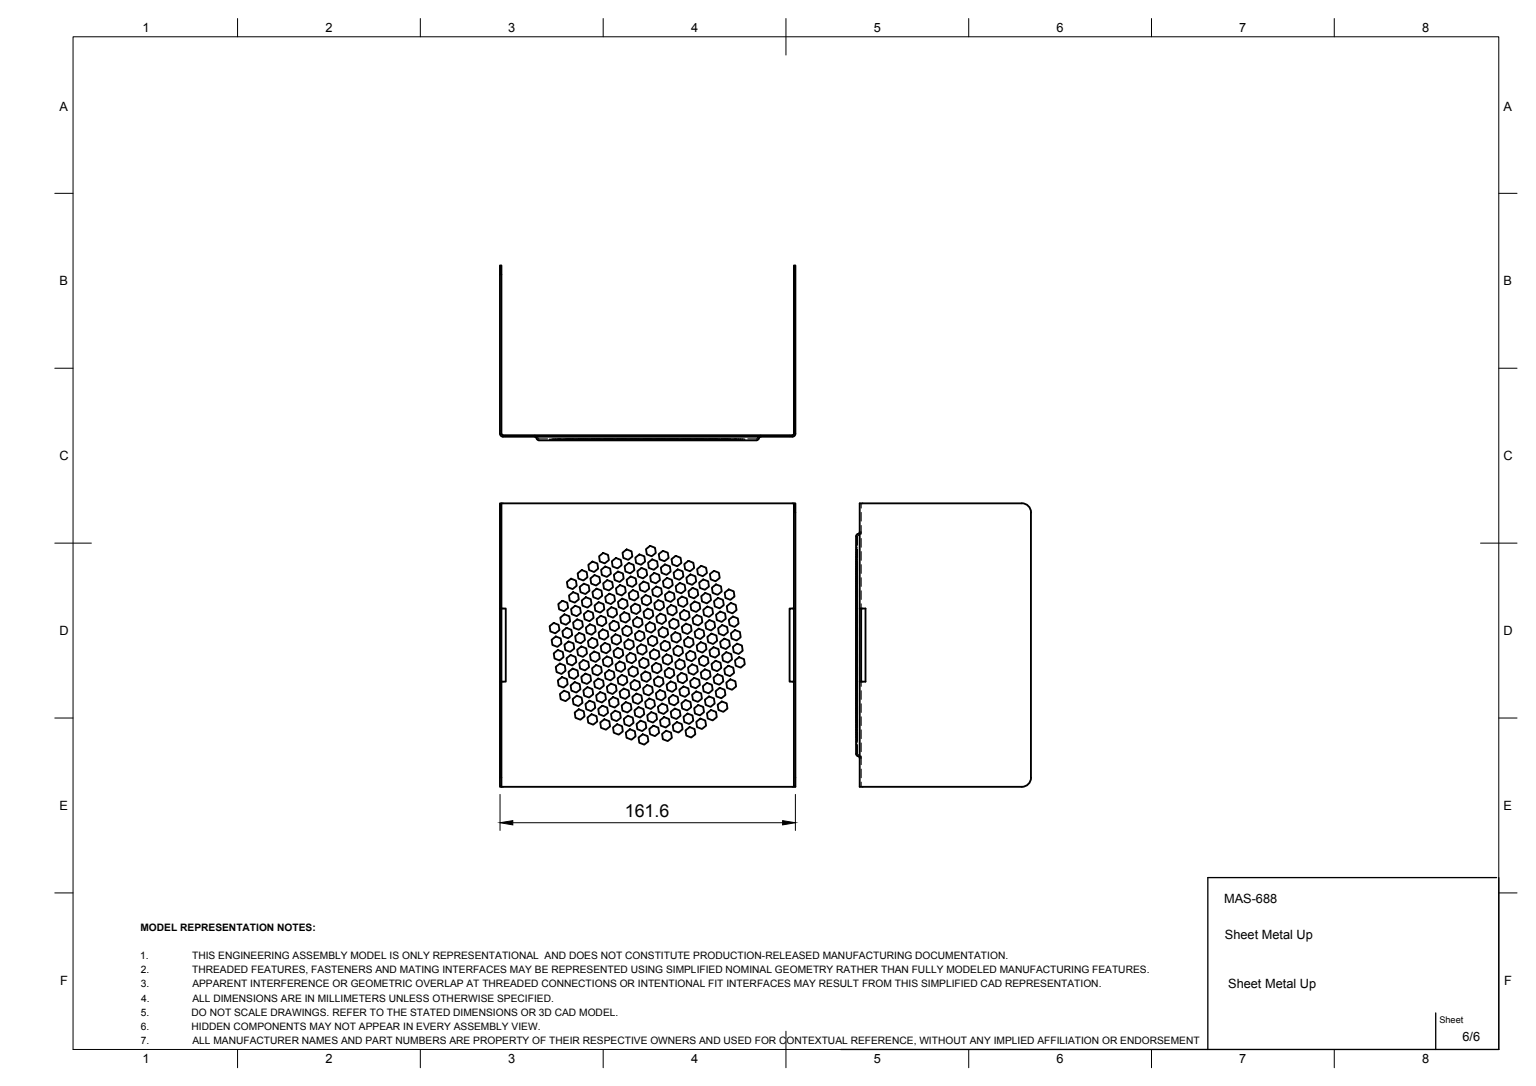
ISO-10303-21;
HEADER;
/* Generated by software containing ST-Developer
 * from STEP Tools, Inc. (www.steptools.com) 
 */

FILE_DESCRIPTION(
/* description */ ('STEP AP214'),
/* implementation_level */ '2;1');

FILE_NAME(
/* name */ 'Sheet Metal Up.step',
/* time_stamp */ '2026-11-14T03:58:36-08:00',
/* author */ (''),
/* organization */ (''),
/* preprocessor_version */ 'ST-DEVELOPER v20.2',
/* originating_system */ 'Autodesk Translation Framework v15.17.0.0',
/* authorisation */ '');

FILE_SCHEMA (('AUTOMOTIVE_DESIGN { 1 0 10303 214 3 1 1 }'));
ENDSEC;

DATA;
#10=MECHANICAL_DESIGN_GEOMETRIC_PRESENTATION_REPRESENTATION('',(#44),#65304);
#36=SHAPE_REPRESENTATION_RELATIONSHIP('SRR','None',#65327,#40);
#40=ADVANCED_BREP_SHAPE_REPRESENTATION('',(#47),#65303);
#44=STYLED_ITEM('',(#65356),#47);
#47=MANIFOLD_SOLID_BREP('Body1',#39937);
#255=FACE_BOUND('',#5203,.T.);
#256=FACE_BOUND('',#5205,.T.);
#257=FACE_BOUND('',#5251,.T.);
#258=FACE_BOUND('',#5252,.T.);
#259=FACE_BOUND('',#5253,.T.);
#260=FACE_BOUND('',#5254,.T.);
#261=FACE_BOUND('',#5255,.T.);
#262=FACE_BOUND('',#5256,.T.);
#263=FACE_BOUND('',#5257,.T.);
#264=FACE_BOUND('',#5258,.T.);
#265=FACE_BOUND('',#5259,.T.);
#266=FACE_BOUND('',#5260,.T.);
#267=FACE_BOUND('',#5261,.T.);
#268=FACE_BOUND('',#5262,.T.);
#269=FACE_BOUND('',#5263,.T.);
#270=FACE_BOUND('',#5264,.T.);
#271=FACE_BOUND('',#5265,.T.);
#272=FACE_BOUND('',#5266,.T.);
#273=FACE_BOUND('',#5267,.T.);
#274=FACE_BOUND('',#5268,.T.);
#275=FACE_BOUND('',#5269,.T.);
#276=FACE_BOUND('',#5270,.T.);
#277=FACE_BOUND('',#5271,.T.);
#278=FACE_BOUND('',#5272,.T.);
#279=FACE_BOUND('',#5273,.T.);
#280=FACE_BOUND('',#5274,.T.);
#281=FACE_BOUND('',#5275,.T.);
#282=FACE_BOUND('',#5276,.T.);
#283=FACE_BOUND('',#5277,.T.);
#284=FACE_BOUND('',#5278,.T.);
#285=FACE_BOUND('',#5279,.T.);
#286=FACE_BOUND('',#5280,.T.);
#287=FACE_BOUND('',#5281,.T.);
#288=FACE_BOUND('',#5282,.T.);
#289=FACE_BOUND('',#5283,.T.);
#290=FACE_BOUND('',#5284,.T.);
#291=FACE_BOUND('',#5285,.T.);
#292=FACE_BOUND('',#5286,.T.);
#293=FACE_BOUND('',#5287,.T.);
#294=FACE_BOUND('',#5288,.T.);
#295=FACE_BOUND('',#5289,.T.);
#296=FACE_BOUND('',#5290,.T.);
#297=FACE_BOUND('',#5291,.T.);
#298=FACE_BOUND('',#5292,.T.);
#299=FACE_BOUND('',#5293,.T.);
#300=FACE_BOUND('',#5294,.T.);
#301=FACE_BOUND('',#5295,.T.);
#302=FACE_BOUND('',#5296,.T.);
#303=FACE_BOUND('',#5297,.T.);
#304=FACE_BOUND('',#5298,.T.);
#305=FACE_BOUND('',#5299,.T.);
#306=FACE_BOUND('',#5300,.T.);
#307=FACE_BOUND('',#5301,.T.);
#308=FACE_BOUND('',#5302,.T.);
#309=FACE_BOUND('',#5303,.T.);
#310=FACE_BOUND('',#5304,.T.);
#311=FACE_BOUND('',#5305,.T.);
#312=FACE_BOUND('',#5306,.T.);
#313=FACE_BOUND('',#5307,.T.);
#314=FACE_BOUND('',#5308,.T.);
#315=FACE_BOUND('',#5309,.T.);
#316=FACE_BOUND('',#5310,.T.);
#317=FACE_BOUND('',#5311,.T.);
#318=FACE_BOUND('',#5312,.T.);
#319=FACE_BOUND('',#5313,.T.);
#320=FACE_BOUND('',#5314,.T.);
#321=FACE_BOUND('',#5315,.T.);
#322=FACE_BOUND('',#5316,.T.);
#323=FACE_BOUND('',#5317,.T.);
#324=FACE_BOUND('',#5318,.T.);
#325=FACE_BOUND('',#5319,.T.);
#326=FACE_BOUND('',#5320,.T.);
#327=FACE_BOUND('',#5321,.T.);
#328=FACE_BOUND('',#5322,.T.);
#329=FACE_BOUND('',#5323,.T.);
#330=FACE_BOUND('',#5324,.T.);
#331=FACE_BOUND('',#5325,.T.);
#332=FACE_BOUND('',#5326,.T.);
#333=FACE_BOUND('',#5327,.T.);
#334=FACE_BOUND('',#5328,.T.);
#335=FACE_BOUND('',#5329,.T.);
#336=FACE_BOUND('',#5330,.T.);
#337=FACE_BOUND('',#5331,.T.);
#338=FACE_BOUND('',#5332,.T.);
#339=FACE_BOUND('',#5333,.T.);
#340=FACE_BOUND('',#5334,.T.);
#341=FACE_BOUND('',#5335,.T.);
#342=FACE_BOUND('',#5336,.T.);
#343=FACE_BOUND('',#5337,.T.);
#344=FACE_BOUND('',#5338,.T.);
#345=FACE_BOUND('',#5339,.T.);
#346=FACE_BOUND('',#5340,.T.);
#347=FACE_BOUND('',#5341,.T.);
#348=FACE_BOUND('',#5342,.T.);
#349=FACE_BOUND('',#5343,.T.);
#350=FACE_BOUND('',#5344,.T.);
#351=FACE_BOUND('',#5345,.T.);
#352=FACE_BOUND('',#5346,.T.);
#353=FACE_BOUND('',#5347,.T.);
#354=FACE_BOUND('',#5348,.T.);
#355=FACE_BOUND('',#5349,.T.);
#356=FACE_BOUND('',#5350,.T.);
#357=FACE_BOUND('',#5351,.T.);
#358=FACE_BOUND('',#5352,.T.);
#359=FACE_BOUND('',#5353,.T.);
#360=FACE_BOUND('',#5354,.T.);
#361=FACE_BOUND('',#5355,.T.);
#362=FACE_BOUND('',#5356,.T.);
#363=FACE_BOUND('',#5357,.T.);
#364=FACE_BOUND('',#5358,.T.);
#365=FACE_BOUND('',#5359,.T.);
#366=FACE_BOUND('',#5360,.T.);
#367=FACE_BOUND('',#5361,.T.);
#368=FACE_BOUND('',#5362,.T.);
#369=FACE_BOUND('',#5363,.T.);
#370=FACE_BOUND('',#5364,.T.);
#371=FACE_BOUND('',#5365,.T.);
#372=FACE_BOUND('',#5366,.T.);
#373=FACE_BOUND('',#5367,.T.);
#374=FACE_BOUND('',#5368,.T.);
#375=FACE_BOUND('',#5369,.T.);
#376=FACE_BOUND('',#5370,.T.);
#377=FACE_BOUND('',#5371,.T.);
#378=FACE_BOUND('',#5372,.T.);
#379=FACE_BOUND('',#5373,.T.);
#380=FACE_BOUND('',#5374,.T.);
#381=FACE_BOUND('',#5375,.T.);
#382=FACE_BOUND('',#5376,.T.);
#383=FACE_BOUND('',#5377,.T.);
#384=FACE_BOUND('',#5378,.T.);
#385=FACE_BOUND('',#5379,.T.);
#386=FACE_BOUND('',#5380,.T.);
#387=FACE_BOUND('',#5381,.T.);
#388=FACE_BOUND('',#5382,.T.);
#389=FACE_BOUND('',#5383,.T.);
#390=FACE_BOUND('',#5384,.T.);
#391=FACE_BOUND('',#5385,.T.);
#392=FACE_BOUND('',#5386,.T.);
#393=FACE_BOUND('',#5387,.T.);
#394=FACE_BOUND('',#5388,.T.);
#395=FACE_BOUND('',#5389,.T.);
#396=FACE_BOUND('',#5390,.T.);
#397=FACE_BOUND('',#5391,.T.);
#398=FACE_BOUND('',#5392,.T.);
#399=FACE_BOUND('',#5393,.T.);
#400=FACE_BOUND('',#5394,.T.);
#401=FACE_BOUND('',#5395,.T.);
#402=FACE_BOUND('',#5396,.T.);
#403=FACE_BOUND('',#5397,.T.);
#404=FACE_BOUND('',#5398,.T.);
#405=FACE_BOUND('',#5399,.T.);
#406=FACE_BOUND('',#5400,.T.);
#407=FACE_BOUND('',#5401,.T.);
#408=FACE_BOUND('',#5402,.T.);
#409=FACE_BOUND('',#5403,.T.);
#410=FACE_BOUND('',#5404,.T.);
#411=FACE_BOUND('',#5405,.T.);
#412=FACE_BOUND('',#5406,.T.);
#413=FACE_BOUND('',#5407,.T.);
#414=FACE_BOUND('',#5408,.T.);
#415=FACE_BOUND('',#5409,.T.);
#416=FACE_BOUND('',#5410,.T.);
#417=FACE_BOUND('',#5411,.T.);
#418=FACE_BOUND('',#5412,.T.);
#419=FACE_BOUND('',#5413,.T.);
#420=FACE_BOUND('',#5414,.T.);
#421=FACE_BOUND('',#5415,.T.);
#422=FACE_BOUND('',#5416,.T.);
#423=FACE_BOUND('',#5417,.T.);
#424=FACE_BOUND('',#5418,.T.);
#425=FACE_BOUND('',#5419,.T.);
#426=FACE_BOUND('',#5420,.T.);
#427=FACE_BOUND('',#5421,.T.);
#428=FACE_BOUND('',#5422,.T.);
#429=FACE_BOUND('',#5423,.T.);
#430=FACE_BOUND('',#5424,.T.);
#431=FACE_BOUND('',#5425,.T.);
#432=FACE_BOUND('',#5426,.T.);
#433=FACE_BOUND('',#5427,.T.);
#434=FACE_BOUND('',#5428,.T.);
#435=FACE_BOUND('',#5429,.T.);
#436=FACE_BOUND('',#5430,.T.);
#437=FACE_BOUND('',#5431,.T.);
#438=FACE_BOUND('',#5432,.T.);
#439=FACE_BOUND('',#5433,.T.);
#440=FACE_BOUND('',#5434,.T.);
#441=FACE_BOUND('',#5435,.T.);
#442=FACE_BOUND('',#5436,.T.);
#443=FACE_BOUND('',#5438,.T.);
#444=FACE_BOUND('',#5439,.T.);
#445=FACE_BOUND('',#5440,.T.);
#446=FACE_BOUND('',#5441,.T.);
#447=FACE_BOUND('',#5442,.T.);
#448=FACE_BOUND('',#5443,.T.);
#449=FACE_BOUND('',#5444,.T.);
#450=FACE_BOUND('',#5445,.T.);
#451=FACE_BOUND('',#5446,.T.);
#452=FACE_BOUND('',#5447,.T.);
#453=FACE_BOUND('',#5448,.T.);
#454=FACE_BOUND('',#5449,.T.);
#455=FACE_BOUND('',#5450,.T.);
#456=FACE_BOUND('',#5451,.T.);
#457=FACE_BOUND('',#5452,.T.);
#458=FACE_BOUND('',#5453,.T.);
#459=FACE_BOUND('',#5454,.T.);
#460=FACE_BOUND('',#5455,.T.);
#461=FACE_BOUND('',#5456,.T.);
#462=FACE_BOUND('',#5457,.T.);
#463=FACE_BOUND('',#5458,.T.);
#464=FACE_BOUND('',#5459,.T.);
#465=FACE_BOUND('',#5460,.T.);
#466=FACE_BOUND('',#5461,.T.);
#467=FACE_BOUND('',#5462,.T.);
#468=FACE_BOUND('',#5463,.T.);
#469=FACE_BOUND('',#5464,.T.);
#470=FACE_BOUND('',#5465,.T.);
#471=FACE_BOUND('',#5466,.T.);
#472=FACE_BOUND('',#5467,.T.);
#473=FACE_BOUND('',#5468,.T.);
#474=FACE_BOUND('',#5469,.T.);
#475=FACE_BOUND('',#5470,.T.);
#476=FACE_BOUND('',#5471,.T.);
#477=FACE_BOUND('',#5472,.T.);
#478=FACE_BOUND('',#5473,.T.);
#479=FACE_BOUND('',#5474,.T.);
#480=FACE_BOUND('',#5475,.T.);
#481=FACE_BOUND('',#5476,.T.);
#482=FACE_BOUND('',#5477,.T.);
#483=FACE_BOUND('',#5478,.T.);
#484=FACE_BOUND('',#5479,.T.);
#485=FACE_BOUND('',#5480,.T.);
#486=FACE_BOUND('',#5481,.T.);
#487=FACE_BOUND('',#5482,.T.);
#488=FACE_BOUND('',#5483,.T.);
#489=FACE_BOUND('',#5484,.T.);
#490=FACE_BOUND('',#5485,.T.);
#491=FACE_BOUND('',#5486,.T.);
#492=FACE_BOUND('',#5487,.T.);
#493=FACE_BOUND('',#5488,.T.);
#494=FACE_BOUND('',#5489,.T.);
#495=FACE_BOUND('',#5490,.T.);
#496=FACE_BOUND('',#5491,.T.);
#497=FACE_BOUND('',#5492,.T.);
#498=FACE_BOUND('',#5493,.T.);
#499=FACE_BOUND('',#5494,.T.);
#500=FACE_BOUND('',#5495,.T.);
#501=FACE_BOUND('',#5496,.T.);
#502=FACE_BOUND('',#5497,.T.);
#503=FACE_BOUND('',#5498,.T.);
#504=FACE_BOUND('',#5499,.T.);
#505=FACE_BOUND('',#5500,.T.);
#506=FACE_BOUND('',#5501,.T.);
#507=FACE_BOUND('',#5502,.T.);
#508=FACE_BOUND('',#5503,.T.);
#509=FACE_BOUND('',#5504,.T.);
#510=FACE_BOUND('',#5505,.T.);
#511=FACE_BOUND('',#5506,.T.);
#512=FACE_BOUND('',#5507,.T.);
#513=FACE_BOUND('',#5508,.T.);
#514=FACE_BOUND('',#5509,.T.);
#515=FACE_BOUND('',#5510,.T.);
#516=FACE_BOUND('',#5511,.T.);
#517=FACE_BOUND('',#5512,.T.);
#518=FACE_BOUND('',#5513,.T.);
#519=FACE_BOUND('',#5514,.T.);
#520=FACE_BOUND('',#5515,.T.);
#521=FACE_BOUND('',#5516,.T.);
#522=FACE_BOUND('',#5517,.T.);
#523=FACE_BOUND('',#5518,.T.);
#524=FACE_BOUND('',#5519,.T.);
#525=FACE_BOUND('',#5520,.T.);
#526=FACE_BOUND('',#5521,.T.);
#527=FACE_BOUND('',#5522,.T.);
#528=FACE_BOUND('',#5523,.T.);
#529=FACE_BOUND('',#5524,.T.);
#530=FACE_BOUND('',#5525,.T.);
#531=FACE_BOUND('',#5526,.T.);
#532=FACE_BOUND('',#5527,.T.);
#533=FACE_BOUND('',#5528,.T.);
#534=FACE_BOUND('',#5529,.T.);
#535=FACE_BOUND('',#5530,.T.);
#536=FACE_BOUND('',#5531,.T.);
#537=FACE_BOUND('',#5532,.T.);
#538=FACE_BOUND('',#5533,.T.);
#539=FACE_BOUND('',#5534,.T.);
#540=FACE_BOUND('',#5535,.T.);
#541=FACE_BOUND('',#5536,.T.);
#542=FACE_BOUND('',#5537,.T.);
#543=FACE_BOUND('',#5538,.T.);
#544=FACE_BOUND('',#5539,.T.);
#545=FACE_BOUND('',#5540,.T.);
#546=FACE_BOUND('',#5541,.T.);
#547=FACE_BOUND('',#5542,.T.);
#548=FACE_BOUND('',#5543,.T.);
#549=FACE_BOUND('',#5544,.T.);
#550=FACE_BOUND('',#5545,.T.);
#551=FACE_BOUND('',#5546,.T.);
#552=FACE_BOUND('',#5547,.T.);
#553=FACE_BOUND('',#5548,.T.);
#554=FACE_BOUND('',#5549,.T.);
#555=FACE_BOUND('',#5550,.T.);
#556=FACE_BOUND('',#5551,.T.);
#557=FACE_BOUND('',#5552,.T.);
#558=FACE_BOUND('',#5553,.T.);
#559=FACE_BOUND('',#5554,.T.);
#560=FACE_BOUND('',#5555,.T.);
#561=FACE_BOUND('',#5556,.T.);
#562=FACE_BOUND('',#5557,.T.);
#563=FACE_BOUND('',#5558,.T.);
#564=FACE_BOUND('',#5559,.T.);
#565=FACE_BOUND('',#5560,.T.);
#566=FACE_BOUND('',#5561,.T.);
#567=FACE_BOUND('',#5562,.T.);
#568=FACE_BOUND('',#5563,.T.);
#569=FACE_BOUND('',#5564,.T.);
#570=FACE_BOUND('',#5565,.T.);
#571=FACE_BOUND('',#5566,.T.);
#572=FACE_BOUND('',#5567,.T.);
#573=FACE_BOUND('',#5568,.T.);
#574=FACE_BOUND('',#5569,.T.);
#575=FACE_BOUND('',#5570,.T.);
#576=FACE_BOUND('',#5571,.T.);
#577=FACE_BOUND('',#5572,.T.);
#578=FACE_BOUND('',#5573,.T.);
#579=FACE_BOUND('',#5574,.T.);
#580=FACE_BOUND('',#5575,.T.);
#581=FACE_BOUND('',#5576,.T.);
#582=FACE_BOUND('',#5577,.T.);
#583=FACE_BOUND('',#5578,.T.);
#584=FACE_BOUND('',#5579,.T.);
#585=FACE_BOUND('',#5580,.T.);
#586=FACE_BOUND('',#5581,.T.);
#587=FACE_BOUND('',#5582,.T.);
#588=FACE_BOUND('',#5583,.T.);
#589=FACE_BOUND('',#5584,.T.);
#590=FACE_BOUND('',#5585,.T.);
#591=FACE_BOUND('',#5586,.T.);
#592=FACE_BOUND('',#5587,.T.);
#593=FACE_BOUND('',#5588,.T.);
#594=FACE_BOUND('',#5589,.T.);
#595=FACE_BOUND('',#5590,.T.);
#596=FACE_BOUND('',#5591,.T.);
#597=FACE_BOUND('',#5592,.T.);
#598=FACE_BOUND('',#5593,.T.);
#599=FACE_BOUND('',#5594,.T.);
#600=FACE_BOUND('',#5595,.T.);
#601=FACE_BOUND('',#5596,.T.);
#602=FACE_BOUND('',#5597,.T.);
#603=FACE_BOUND('',#5598,.T.);
#604=FACE_BOUND('',#5599,.T.);
#605=FACE_BOUND('',#5600,.T.);
#606=FACE_BOUND('',#5601,.T.);
#607=FACE_BOUND('',#5602,.T.);
#608=FACE_BOUND('',#5603,.T.);
#609=FACE_BOUND('',#5604,.T.);
#610=FACE_BOUND('',#5605,.T.);
#611=FACE_BOUND('',#5606,.T.);
#612=FACE_BOUND('',#5607,.T.);
#613=FACE_BOUND('',#5608,.T.);
#614=FACE_BOUND('',#5609,.T.);
#615=FACE_BOUND('',#5610,.T.);
#616=FACE_BOUND('',#5611,.T.);
#617=FACE_BOUND('',#5612,.T.);
#618=FACE_BOUND('',#5613,.T.);
#619=FACE_BOUND('',#5614,.T.);
#620=FACE_BOUND('',#5615,.T.);
#621=FACE_BOUND('',#5616,.T.);
#622=FACE_BOUND('',#5617,.T.);
#623=FACE_BOUND('',#5618,.T.);
#624=FACE_BOUND('',#5619,.T.);
#625=FACE_BOUND('',#5620,.T.);
#626=FACE_BOUND('',#5621,.T.);
#627=FACE_BOUND('',#5622,.T.);
#628=FACE_BOUND('',#5623,.T.);
#1029=PLANE('',#41322);
#1030=PLANE('',#41323);
#1031=PLANE('',#41324);
#1032=PLANE('',#41325);
#1033=PLANE('',#41326);
#1034=PLANE('',#41327);
#1035=PLANE('',#41328);
#1036=PLANE('',#41329);
#1037=PLANE('',#41330);
#1038=PLANE('',#41331);
#1039=PLANE('',#41332);
#1040=PLANE('',#41335);
#1041=PLANE('',#41340);
#1042=PLANE('',#41343);
#1043=PLANE('',#41351);
#1044=PLANE('',#41355);
#1045=PLANE('',#41356);
#1046=PLANE('',#41357);
#1047=PLANE('',#41358);
#1048=PLANE('',#41359);
#1049=PLANE('',#41360);
#1050=PLANE('',#41361);
#1051=PLANE('',#41362);
#1052=PLANE('',#41365);
#1053=PLANE('',#41370);
#1054=PLANE('',#41373);
#1055=PLANE('',#41381);
#1056=PLANE('',#41385);
#1057=PLANE('',#41386);
#1058=PLANE('',#41387);
#1059=PLANE('',#41388);
#1060=PLANE('',#41389);
#1061=PLANE('',#41390);
#1062=PLANE('',#41391);
#1063=PLANE('',#41392);
#1064=PLANE('',#41393);
#1065=PLANE('',#41394);
#1066=PLANE('',#41395);
#1067=PLANE('',#41396);
#1068=PLANE('',#41397);
#1069=PLANE('',#41398);
#1070=PLANE('',#41399);
#1071=PLANE('',#41400);
#1072=PLANE('',#41401);
#1073=PLANE('',#41402);
#1074=PLANE('',#41403);
#1075=PLANE('',#41404);
#1076=PLANE('',#41405);
#1077=PLANE('',#41406);
#1078=PLANE('',#41407);
#1079=PLANE('',#41408);
#1080=PLANE('',#41409);
#1081=PLANE('',#41410);
#1082=PLANE('',#41411);
#1083=PLANE('',#41412);
#1084=PLANE('',#41413);
#1085=PLANE('',#41414);
#1086=PLANE('',#41415);
#1087=PLANE('',#41416);
#1088=PLANE('',#41417);
#1089=PLANE('',#41418);
#1090=PLANE('',#41419);
#1091=PLANE('',#41420);
#1092=PLANE('',#41421);
#1093=PLANE('',#41422);
#1094=PLANE('',#41423);
#1095=PLANE('',#41424);
#1096=PLANE('',#41425);
#1097=PLANE('',#41426);
#1098=PLANE('',#41427);
#1099=PLANE('',#41428);
#1100=PLANE('',#41429);
#1101=PLANE('',#41430);
#1102=PLANE('',#41431);
#1103=PLANE('',#41432);
#1104=PLANE('',#41433);
#1105=PLANE('',#41434);
#1106=PLANE('',#41435);
#1107=PLANE('',#41436);
#1108=PLANE('',#41437);
#1109=PLANE('',#41438);
#1110=PLANE('',#41439);
#1111=PLANE('',#41440);
#1112=PLANE('',#41441);
#1113=PLANE('',#41442);
#1114=PLANE('',#41443);
#1115=PLANE('',#41444);
#1116=PLANE('',#41445);
#1117=PLANE('',#41446);
#1118=PLANE('',#41447);
#1119=PLANE('',#41448);
#1120=PLANE('',#41449);
#1121=PLANE('',#41450);
#1122=PLANE('',#41451);
#1123=PLANE('',#41452);
#1124=PLANE('',#41453);
#1125=PLANE('',#41454);
#1126=PLANE('',#41455);
#1127=PLANE('',#41456);
#1128=PLANE('',#41457);
#1129=PLANE('',#41458);
#1130=PLANE('',#41459);
#1131=PLANE('',#41460);
#1132=PLANE('',#41461);
#1133=PLANE('',#41462);
#1134=PLANE('',#41463);
#1135=PLANE('',#41464);
#1136=PLANE('',#41465);
#1137=PLANE('',#41466);
#1138=PLANE('',#41467);
#1139=PLANE('',#41468);
#1140=PLANE('',#41469);
#1141=PLANE('',#41470);
#1142=PLANE('',#41471);
#1143=PLANE('',#41472);
#1144=PLANE('',#41473);
#1145=PLANE('',#41474);
#1146=PLANE('',#41475);
#1147=PLANE('',#41476);
#1148=PLANE('',#41477);
#1149=PLANE('',#41478);
#1150=PLANE('',#41479);
#1151=PLANE('',#41480);
#1152=PLANE('',#41481);
#1153=PLANE('',#41482);
#1154=PLANE('',#41483);
#1155=PLANE('',#41484);
#1156=PLANE('',#41485);
#1157=PLANE('',#41486);
#1158=PLANE('',#41487);
#1159=PLANE('',#41488);
#1160=PLANE('',#41489);
#1161=PLANE('',#41490);
#1162=PLANE('',#41491);
#1163=PLANE('',#41492);
#1164=PLANE('',#41493);
#1165=PLANE('',#41494);
#1166=PLANE('',#41495);
#1167=PLANE('',#41496);
#1168=PLANE('',#41497);
#1169=PLANE('',#41498);
#1170=PLANE('',#41499);
#1171=PLANE('',#41500);
#1172=PLANE('',#41501);
#1173=PLANE('',#41502);
#1174=PLANE('',#41503);
#1175=PLANE('',#41504);
#1176=PLANE('',#41505);
#1177=PLANE('',#41506);
#1178=PLANE('',#41507);
#1179=PLANE('',#41508);
#1180=PLANE('',#41509);
#1181=PLANE('',#41510);
#1182=PLANE('',#41511);
#1183=PLANE('',#41512);
#1184=PLANE('',#41513);
#1185=PLANE('',#41514);
#1186=PLANE('',#41515);
#1187=PLANE('',#41516);
#1188=PLANE('',#41517);
#1189=PLANE('',#41518);
#1190=PLANE('',#41519);
#1191=PLANE('',#41520);
#1192=PLANE('',#41521);
#1193=PLANE('',#41522);
#1194=PLANE('',#41523);
#1195=PLANE('',#41524);
#1196=PLANE('',#41525);
#1197=PLANE('',#41526);
#1198=PLANE('',#41527);
#1199=PLANE('',#41528);
#1200=PLANE('',#41529);
#1201=PLANE('',#41530);
#1202=PLANE('',#41531);
#1203=PLANE('',#41532);
#1204=PLANE('',#41533);
#1205=PLANE('',#41534);
#1206=PLANE('',#41535);
#1207=PLANE('',#41536);
#1208=PLANE('',#41537);
#1209=PLANE('',#41538);
#1210=PLANE('',#41539);
#1211=PLANE('',#41540);
#1212=PLANE('',#41541);
#1213=PLANE('',#41542);
#1214=PLANE('',#41543);
#1215=PLANE('',#41544);
#1216=PLANE('',#41545);
#1217=PLANE('',#41546);
#1218=PLANE('',#41547);
#1219=PLANE('',#41548);
#1220=PLANE('',#41549);
#1221=PLANE('',#41550);
#1222=PLANE('',#41551);
#1223=PLANE('',#41552);
#1224=PLANE('',#41553);
#1225=PLANE('',#41554);
#1226=PLANE('',#41555);
#1227=PLANE('',#41556);
#1228=PLANE('',#41557);
#1229=PLANE('',#41558);
#1230=PLANE('',#41559);
#1231=PLANE('',#41560);
#1232=PLANE('',#41561);
#1233=PLANE('',#41562);
#1234=PLANE('',#41563);
#1235=PLANE('',#41564);
#1236=PLANE('',#41565);
#1237=PLANE('',#41566);
#1238=PLANE('',#41567);
#1239=PLANE('',#41568);
#1240=PLANE('',#41569);
#1241=PLANE('',#41570);
#1242=PLANE('',#41571);
#1243=PLANE('',#41572);
#1244=PLANE('',#41573);
#1245=PLANE('',#41574);
#1246=PLANE('',#41575);
#1247=PLANE('',#41576);
#1248=PLANE('',#41577);
#1249=PLANE('',#41578);
#1250=PLANE('',#41579);
#1251=PLANE('',#41580);
#1252=PLANE('',#41581);
#1253=PLANE('',#41582);
#1254=PLANE('',#41583);
#1255=PLANE('',#41584);
#1256=PLANE('',#41585);
#1257=PLANE('',#41586);
#1258=PLANE('',#41587);
#1259=PLANE('',#41588);
#1260=PLANE('',#41589);
#1261=PLANE('',#41590);
#1262=PLANE('',#41591);
#1263=PLANE('',#41592);
#1264=PLANE('',#41593);
#1265=PLANE('',#41594);
#1266=PLANE('',#41595);
#1267=PLANE('',#41596);
#1268=PLANE('',#41597);
#1269=PLANE('',#41598);
#1270=PLANE('',#41599);
#1271=PLANE('',#41600);
#1272=PLANE('',#41601);
#1273=PLANE('',#41602);
#1274=PLANE('',#41603);
#1275=PLANE('',#41604);
#1276=PLANE('',#41605);
#1277=PLANE('',#41606);
#1278=PLANE('',#41607);
#1279=PLANE('',#41608);
#1280=PLANE('',#41609);
#1281=PLANE('',#41610);
#1282=PLANE('',#41611);
#1283=PLANE('',#41612);
#1284=PLANE('',#41613);
#1285=PLANE('',#41614);
#1286=PLANE('',#41615);
#1287=PLANE('',#41616);
#1288=PLANE('',#41617);
#1289=PLANE('',#41618);
#1290=PLANE('',#41619);
#1291=PLANE('',#41620);
#1292=PLANE('',#41621);
#1293=PLANE('',#41622);
#1294=PLANE('',#41623);
#1295=PLANE('',#41624);
#1296=PLANE('',#41625);
#1297=PLANE('',#41626);
#1298=PLANE('',#41627);
#1299=PLANE('',#41628);
#1300=PLANE('',#41629);
#1301=PLANE('',#41630);
#1302=PLANE('',#41631);
#1303=PLANE('',#41632);
#1304=PLANE('',#41633);
#1305=PLANE('',#41634);
#1306=PLANE('',#41635);
#1307=PLANE('',#41636);
#1308=PLANE('',#41637);
#1309=PLANE('',#41638);
#1310=PLANE('',#41639);
#1311=PLANE('',#41640);
#1312=PLANE('',#41641);
#1313=PLANE('',#41642);
#1314=PLANE('',#41643);
#1315=PLANE('',#41644);
#1316=PLANE('',#41645);
#1317=PLANE('',#41646);
#1318=PLANE('',#41647);
#1319=PLANE('',#41648);
#1320=PLANE('',#41649);
#1321=PLANE('',#41650);
#1322=PLANE('',#41651);
#1323=PLANE('',#41652);
#1324=PLANE('',#41653);
#1325=PLANE('',#41654);
#1326=PLANE('',#41655);
#1327=PLANE('',#41656);
#1328=PLANE('',#41657);
#1329=PLANE('',#41658);
#1330=PLANE('',#41659);
#1331=PLANE('',#41660);
#1332=PLANE('',#41661);
#1333=PLANE('',#41662);
#1334=PLANE('',#41663);
#1335=PLANE('',#41664);
#1336=PLANE('',#41665);
#1337=PLANE('',#41666);
#1338=PLANE('',#41667);
#1339=PLANE('',#41668);
#1340=PLANE('',#41669);
#1341=PLANE('',#41670);
#1342=PLANE('',#41671);
#1343=PLANE('',#41672);
#1344=PLANE('',#41673);
#1345=PLANE('',#41674);
#1346=PLANE('',#41675);
#1347=PLANE('',#41676);
#1348=PLANE('',#41677);
#1349=PLANE('',#41678);
#1350=PLANE('',#41679);
#1351=PLANE('',#41680);
#1352=PLANE('',#41681);
#1353=PLANE('',#41682);
#1354=PLANE('',#41683);
#1355=PLANE('',#41684);
#1356=PLANE('',#41685);
#1357=PLANE('',#41686);
#1358=PLANE('',#41687);
#1359=PLANE('',#41688);
#1360=PLANE('',#41689);
#1361=PLANE('',#41690);
#1362=PLANE('',#41691);
#1363=PLANE('',#41692);
#1364=PLANE('',#41693);
#1365=PLANE('',#41694);
#1366=PLANE('',#41695);
#1367=PLANE('',#41696);
#1368=PLANE('',#41697);
#1369=PLANE('',#41698);
#1370=PLANE('',#41699);
#1371=PLANE('',#41700);
#1372=PLANE('',#41701);
#1373=PLANE('',#41702);
#1374=PLANE('',#41703);
#1375=PLANE('',#41704);
#1376=PLANE('',#41705);
#1377=PLANE('',#41706);
#1378=PLANE('',#41707);
#1379=PLANE('',#41708);
#1380=PLANE('',#41709);
#1381=PLANE('',#41710);
#1382=PLANE('',#41711);
#1383=PLANE('',#41712);
#1384=PLANE('',#41713);
#1385=PLANE('',#41714);
#1386=PLANE('',#41715);
#1387=PLANE('',#41716);
#1388=PLANE('',#41717);
#1389=PLANE('',#41718);
#1390=PLANE('',#41719);
#1391=PLANE('',#41720);
#1392=PLANE('',#41721);
#1393=PLANE('',#41722);
#1394=PLANE('',#41723);
#1395=PLANE('',#41724);
#1396=PLANE('',#41725);
#1397=PLANE('',#41726);
#1398=PLANE('',#41727);
#1399=PLANE('',#41728);
#1400=PLANE('',#41729);
#1401=PLANE('',#41730);
#1402=PLANE('',#41731);
#1403=PLANE('',#41732);
#1404=PLANE('',#41733);
#1405=PLANE('',#41734);
#1406=PLANE('',#41735);
#1407=PLANE('',#41736);
#1408=PLANE('',#41737);
#1409=PLANE('',#41738);
#1410=PLANE('',#41739);
#1411=PLANE('',#41740);
#1412=PLANE('',#41741);
#1413=PLANE('',#41742);
#1414=PLANE('',#41743);
#1415=PLANE('',#41744);
#1416=PLANE('',#41745);
#1417=PLANE('',#41746);
#1418=PLANE('',#41747);
#1419=PLANE('',#41748);
#1420=PLANE('',#41749);
#1421=PLANE('',#41750);
#1422=PLANE('',#41751);
#1423=PLANE('',#41752);
#1424=PLANE('',#41753);
#1425=PLANE('',#41754);
#1426=PLANE('',#41755);
#1427=PLANE('',#41756);
#1428=PLANE('',#41757);
#1429=PLANE('',#41758);
#1430=PLANE('',#41759);
#1431=PLANE('',#41760);
#1432=PLANE('',#41761);
#1433=PLANE('',#41762);
#1434=PLANE('',#41763);
#1435=PLANE('',#41764);
#1436=PLANE('',#41765);
#1437=PLANE('',#41766);
#1438=PLANE('',#41767);
#1439=PLANE('',#41768);
#1440=PLANE('',#41769);
#1441=PLANE('',#41770);
#1442=PLANE('',#41771);
#1443=PLANE('',#41772);
#1444=PLANE('',#41773);
#1445=PLANE('',#41774);
#1446=PLANE('',#41775);
#1447=PLANE('',#41776);
#1448=PLANE('',#41777);
#1449=PLANE('',#41778);
#1450=PLANE('',#41779);
#1451=PLANE('',#41780);
#1452=PLANE('',#41781);
#1453=PLANE('',#41782);
#1454=PLANE('',#41783);
#1455=PLANE('',#41784);
#1456=PLANE('',#41785);
#1457=PLANE('',#41786);
#1458=PLANE('',#41787);
#1459=PLANE('',#41788);
#1460=PLANE('',#41789);
#1461=PLANE('',#41790);
#1462=PLANE('',#41791);
#1463=PLANE('',#41792);
#1464=PLANE('',#41793);
#1465=PLANE('',#41794);
#1466=PLANE('',#41795);
#1467=PLANE('',#41796);
#1468=PLANE('',#41797);
#1469=PLANE('',#41798);
#1470=PLANE('',#41799);
#1471=PLANE('',#41800);
#1472=PLANE('',#41801);
#1473=PLANE('',#41802);
#1474=PLANE('',#41803);
#1475=PLANE('',#41804);
#1476=PLANE('',#41805);
#1477=PLANE('',#41806);
#1478=PLANE('',#41807);
#1479=PLANE('',#41808);
#1480=PLANE('',#41809);
#1481=PLANE('',#41810);
#1482=PLANE('',#41811);
#1483=PLANE('',#41812);
#1484=PLANE('',#41813);
#1485=PLANE('',#41814);
#1486=PLANE('',#41815);
#1487=PLANE('',#41816);
#1488=PLANE('',#41817);
#1489=PLANE('',#41818);
#1490=PLANE('',#41819);
#1491=PLANE('',#41820);
#1492=PLANE('',#41821);
#1493=PLANE('',#41822);
#1494=PLANE('',#41823);
#1495=PLANE('',#41824);
#1496=PLANE('',#41825);
#1497=PLANE('',#41826);
#1498=PLANE('',#41827);
#1499=PLANE('',#41828);
#1500=PLANE('',#41829);
#1501=PLANE('',#41830);
#1502=PLANE('',#41831);
#1503=PLANE('',#41832);
#1504=PLANE('',#41833);
#1505=PLANE('',#41834);
#1506=PLANE('',#41835);
#1507=PLANE('',#41836);
#1508=PLANE('',#41837);
#1509=PLANE('',#41838);
#1510=PLANE('',#41839);
#1511=PLANE('',#41840);
#1512=PLANE('',#41841);
#1513=PLANE('',#41842);
#1514=PLANE('',#41843);
#1515=PLANE('',#41844);
#1516=PLANE('',#41845);
#1517=PLANE('',#41846);
#1518=PLANE('',#41847);
#1519=PLANE('',#41848);
#1520=PLANE('',#41849);
#1521=PLANE('',#41850);
#1522=PLANE('',#41851);
#1523=PLANE('',#41852);
#1524=PLANE('',#41853);
#1525=PLANE('',#41854);
#1526=PLANE('',#41855);
#1527=PLANE('',#41856);
#1528=PLANE('',#41857);
#1529=PLANE('',#41858);
#1530=PLANE('',#41859);
#1531=PLANE('',#41860);
#1532=PLANE('',#41861);
#1533=PLANE('',#41862);
#1534=PLANE('',#41863);
#1535=PLANE('',#41864);
#1536=PLANE('',#41865);
#1537=PLANE('',#41866);
#1538=PLANE('',#41867);
#1539=PLANE('',#41868);
#1540=PLANE('',#41869);
#1541=PLANE('',#41870);
#1542=PLANE('',#41871);
#1543=PLANE('',#41872);
#1544=PLANE('',#41873);
#1545=PLANE('',#41874);
#1546=PLANE('',#41875);
#1547=PLANE('',#41876);
#1548=PLANE('',#41877);
#1549=PLANE('',#41878);
#1550=PLANE('',#41879);
#1551=PLANE('',#41880);
#1552=PLANE('',#41881);
#1553=PLANE('',#41882);
#1554=PLANE('',#41883);
#1555=PLANE('',#41884);
#1556=PLANE('',#41885);
#1557=PLANE('',#41886);
#1558=PLANE('',#41887);
#1559=PLANE('',#41888);
#1560=PLANE('',#41889);
#1561=PLANE('',#41890);
#1562=PLANE('',#41891);
#1563=PLANE('',#41892);
#1564=PLANE('',#41893);
#1565=PLANE('',#41894);
#1566=PLANE('',#41895);
#1567=PLANE('',#41896);
#1568=PLANE('',#41897);
#1569=PLANE('',#41898);
#1570=PLANE('',#41899);
#1571=PLANE('',#41900);
#1572=PLANE('',#41901);
#1573=PLANE('',#41902);
#1574=PLANE('',#41903);
#1575=PLANE('',#41904);
#1576=PLANE('',#41905);
#1577=PLANE('',#41906);
#1578=PLANE('',#41907);
#1579=PLANE('',#41908);
#1580=PLANE('',#41909);
#1581=PLANE('',#41910);
#1582=PLANE('',#41911);
#1583=PLANE('',#41912);
#1584=PLANE('',#41913);
#1585=PLANE('',#41914);
#1586=PLANE('',#41915);
#1587=PLANE('',#41916);
#1588=PLANE('',#41917);
#1589=PLANE('',#41918);
#1590=PLANE('',#41919);
#1591=PLANE('',#41920);
#1592=PLANE('',#41921);
#1593=PLANE('',#41922);
#1594=PLANE('',#41923);
#1595=PLANE('',#41924);
#1596=PLANE('',#41925);
#1597=PLANE('',#41926);
#1598=PLANE('',#41927);
#1599=PLANE('',#41928);
#1600=PLANE('',#41929);
#1601=PLANE('',#41930);
#1602=PLANE('',#41931);
#1603=PLANE('',#41932);
#1604=PLANE('',#41933);
#1605=PLANE('',#41934);
#1606=PLANE('',#41935);
#1607=PLANE('',#41936);
#1608=PLANE('',#41937);
#1609=PLANE('',#41938);
#1610=PLANE('',#41939);
#1611=PLANE('',#41940);
#1612=PLANE('',#41941);
#1613=PLANE('',#41942);
#1614=PLANE('',#41943);
#1615=PLANE('',#41944);
#1616=PLANE('',#41945);
#1617=PLANE('',#41946);
#1618=PLANE('',#41947);
#1619=PLANE('',#41948);
#1620=PLANE('',#41949);
#1621=PLANE('',#41950);
#1622=PLANE('',#41951);
#1623=PLANE('',#41952);
#1624=PLANE('',#41953);
#1625=PLANE('',#41954);
#1626=PLANE('',#41955);
#1627=PLANE('',#41956);
#1628=PLANE('',#41957);
#1629=PLANE('',#41958);
#1630=PLANE('',#41959);
#1631=PLANE('',#41960);
#1632=PLANE('',#41961);
#1633=PLANE('',#41962);
#1634=PLANE('',#41963);
#1635=PLANE('',#41964);
#1636=PLANE('',#41965);
#1637=PLANE('',#41966);
#1638=PLANE('',#41967);
#1639=PLANE('',#41968);
#1640=PLANE('',#41969);
#1641=PLANE('',#41970);
#1642=PLANE('',#41971);
#1643=PLANE('',#41972);
#1644=PLANE('',#41973);
#1645=PLANE('',#41974);
#1646=PLANE('',#41975);
#1647=PLANE('',#41976);
#1648=PLANE('',#41977);
#1649=PLANE('',#41978);
#1650=PLANE('',#41979);
#1651=PLANE('',#41980);
#1652=PLANE('',#41981);
#1653=PLANE('',#41982);
#1654=PLANE('',#41983);
#1655=PLANE('',#41984);
#1656=PLANE('',#41985);
#1657=PLANE('',#41986);
#1658=PLANE('',#41987);
#1659=PLANE('',#41988);
#1660=PLANE('',#41989);
#1661=PLANE('',#41990);
#1662=PLANE('',#41991);
#1663=PLANE('',#41992);
#1664=PLANE('',#41993);
#1665=PLANE('',#41994);
#1666=PLANE('',#41995);
#1667=PLANE('',#41996);
#1668=PLANE('',#41997);
#1669=PLANE('',#41998);
#1670=PLANE('',#41999);
#1671=PLANE('',#42000);
#1672=PLANE('',#42001);
#1673=PLANE('',#42002);
#1674=PLANE('',#42003);
#1675=PLANE('',#42004);
#1676=PLANE('',#42005);
#1677=PLANE('',#42006);
#1678=PLANE('',#42007);
#1679=PLANE('',#42008);
#1680=PLANE('',#42009);
#1681=PLANE('',#42010);
#1682=PLANE('',#42011);
#1683=PLANE('',#42012);
#1684=PLANE('',#42013);
#1685=PLANE('',#42014);
#1686=PLANE('',#42015);
#1687=PLANE('',#42016);
#1688=PLANE('',#42017);
#1689=PLANE('',#42018);
#1690=PLANE('',#42019);
#1691=PLANE('',#42020);
#1692=PLANE('',#42021);
#1693=PLANE('',#42022);
#1694=PLANE('',#42023);
#1695=PLANE('',#42024);
#1696=PLANE('',#42025);
#1697=PLANE('',#42026);
#1698=PLANE('',#42027);
#1699=PLANE('',#42028);
#1700=PLANE('',#42029);
#1701=PLANE('',#42030);
#1702=PLANE('',#42031);
#1703=PLANE('',#42032);
#1704=PLANE('',#42033);
#1705=PLANE('',#42034);
#1706=PLANE('',#42035);
#1707=PLANE('',#42036);
#1708=PLANE('',#42037);
#1709=PLANE('',#42038);
#1710=PLANE('',#42039);
#1711=PLANE('',#42040);
#1712=PLANE('',#42041);
#1713=PLANE('',#42042);
#1714=PLANE('',#42043);
#1715=PLANE('',#42044);
#1716=PLANE('',#42045);
#1717=PLANE('',#42046);
#1718=PLANE('',#42047);
#1719=PLANE('',#42048);
#1720=PLANE('',#42049);
#1721=PLANE('',#42050);
#1722=PLANE('',#42051);
#1723=PLANE('',#42052);
#1724=PLANE('',#42053);
#1725=PLANE('',#42054);
#1726=PLANE('',#42055);
#1727=PLANE('',#42056);
#1728=PLANE('',#42057);
#1729=PLANE('',#42058);
#1730=PLANE('',#42059);
#1731=PLANE('',#42060);
#1732=PLANE('',#42061);
#1733=PLANE('',#42062);
#1734=PLANE('',#42063);
#1735=PLANE('',#42064);
#1736=PLANE('',#42065);
#1737=PLANE('',#42066);
#1738=PLANE('',#42067);
#1739=PLANE('',#42068);
#1740=PLANE('',#42069);
#1741=PLANE('',#42070);
#1742=PLANE('',#42071);
#1743=PLANE('',#42072);
#1744=PLANE('',#42073);
#1745=PLANE('',#42074);
#1746=PLANE('',#42075);
#1747=PLANE('',#42076);
#1748=PLANE('',#42077);
#1749=PLANE('',#42078);
#1750=PLANE('',#42079);
#1751=PLANE('',#42080);
#1752=PLANE('',#42081);
#1753=PLANE('',#42082);
#1754=PLANE('',#42083);
#1755=PLANE('',#42084);
#1756=PLANE('',#42085);
#1757=PLANE('',#42086);
#1758=PLANE('',#42087);
#1759=PLANE('',#42088);
#1760=PLANE('',#42089);
#1761=PLANE('',#42090);
#1762=PLANE('',#42091);
#1763=PLANE('',#42092);
#1764=PLANE('',#42093);
#1765=PLANE('',#42094);
#1766=PLANE('',#42095);
#1767=PLANE('',#42096);
#1768=PLANE('',#42097);
#1769=PLANE('',#42098);
#1770=PLANE('',#42099);
#1771=PLANE('',#42100);
#1772=PLANE('',#42101);
#1773=PLANE('',#42102);
#1774=PLANE('',#42103);
#1775=PLANE('',#42104);
#1776=PLANE('',#42105);
#1777=PLANE('',#42106);
#1778=PLANE('',#42107);
#1779=PLANE('',#42108);
#1780=PLANE('',#42109);
#1781=PLANE('',#42110);
#1782=PLANE('',#42111);
#1783=PLANE('',#42112);
#1784=PLANE('',#42113);
#1785=PLANE('',#42114);
#1786=PLANE('',#42115);
#1787=PLANE('',#42116);
#1788=PLANE('',#42117);
#1789=PLANE('',#42118);
#1790=PLANE('',#42119);
#1791=PLANE('',#42120);
#1792=PLANE('',#42121);
#1793=PLANE('',#42122);
#1794=PLANE('',#42123);
#1795=PLANE('',#42124);
#1796=PLANE('',#42125);
#1797=PLANE('',#42126);
#1798=PLANE('',#42127);
#1799=PLANE('',#42128);
#1800=PLANE('',#42129);
#1801=PLANE('',#42130);
#1802=PLANE('',#42131);
#1803=PLANE('',#42132);
#1804=PLANE('',#42133);
#1805=PLANE('',#42134);
#1806=PLANE('',#42135);
#1807=PLANE('',#42136);
#1808=PLANE('',#42137);
#1809=PLANE('',#42138);
#1810=PLANE('',#42139);
#1811=PLANE('',#42140);
#1812=PLANE('',#42141);
#1813=PLANE('',#42142);
#1814=PLANE('',#42143);
#1815=PLANE('',#42144);
#1816=PLANE('',#42145);
#1817=PLANE('',#42146);
#1818=PLANE('',#42147);
#1819=PLANE('',#42148);
#1820=PLANE('',#42149);
#1821=PLANE('',#42150);
#1822=PLANE('',#42151);
#1823=PLANE('',#42152);
#1824=PLANE('',#42153);
#1825=PLANE('',#42154);
#1826=PLANE('',#42155);
#1827=PLANE('',#42156);
#1828=PLANE('',#42157);
#1829=PLANE('',#42158);
#1830=PLANE('',#42159);
#1831=PLANE('',#42160);
#1832=PLANE('',#42161);
#1833=PLANE('',#42162);
#1834=PLANE('',#42163);
#1835=PLANE('',#42164);
#1836=PLANE('',#42165);
#1837=PLANE('',#42166);
#1838=PLANE('',#42167);
#1839=PLANE('',#42168);
#1840=PLANE('',#42169);
#1841=PLANE('',#42170);
#1842=PLANE('',#42171);
#1843=PLANE('',#42172);
#1844=PLANE('',#42173);
#1845=PLANE('',#42174);
#1846=PLANE('',#42175);
#1847=PLANE('',#42176);
#1848=PLANE('',#42177);
#1849=PLANE('',#42178);
#1850=PLANE('',#42179);
#1851=PLANE('',#42180);
#1852=PLANE('',#42181);
#1853=PLANE('',#42182);
#1854=PLANE('',#42183);
#1855=PLANE('',#42184);
#1856=PLANE('',#42185);
#1857=PLANE('',#42186);
#1858=PLANE('',#42187);
#1859=PLANE('',#42188);
#1860=PLANE('',#42189);
#1861=PLANE('',#42190);
#1862=PLANE('',#42191);
#1863=PLANE('',#42192);
#1864=PLANE('',#42193);
#1865=PLANE('',#42194);
#1866=PLANE('',#42195);
#1867=PLANE('',#42196);
#1868=PLANE('',#42197);
#1869=PLANE('',#42198);
#1870=PLANE('',#42199);
#1871=PLANE('',#42200);
#1872=PLANE('',#42201);
#1873=PLANE('',#42202);
#1874=PLANE('',#42203);
#1875=PLANE('',#42204);
#1876=PLANE('',#42205);
#1877=PLANE('',#42206);
#1878=PLANE('',#42207);
#1879=PLANE('',#42208);
#1880=PLANE('',#42209);
#1881=PLANE('',#42210);
#1882=PLANE('',#42211);
#1883=PLANE('',#42212);
#1884=PLANE('',#42213);
#1885=PLANE('',#42214);
#1886=PLANE('',#42215);
#1887=PLANE('',#42216);
#1888=PLANE('',#42217);
#1889=PLANE('',#42218);
#1890=PLANE('',#42219);
#1891=PLANE('',#42220);
#1892=PLANE('',#42221);
#1893=PLANE('',#42222);
#1894=PLANE('',#42223);
#1895=PLANE('',#42224);
#1896=PLANE('',#42225);
#1897=PLANE('',#42226);
#1898=PLANE('',#42227);
#1899=PLANE('',#42228);
#1900=PLANE('',#42229);
#1901=PLANE('',#42230);
#1902=PLANE('',#42231);
#1903=PLANE('',#42232);
#1904=PLANE('',#42233);
#1905=PLANE('',#42234);
#1906=PLANE('',#42235);
#1907=PLANE('',#42236);
#1908=PLANE('',#42237);
#1909=PLANE('',#42238);
#1910=PLANE('',#42239);
#1911=PLANE('',#42240);
#1912=PLANE('',#42241);
#1913=PLANE('',#42242);
#1914=PLANE('',#42243);
#1915=PLANE('',#42244);
#1916=PLANE('',#42245);
#1917=PLANE('',#42246);
#1918=PLANE('',#42247);
#1919=PLANE('',#42248);
#1920=PLANE('',#42249);
#1921=PLANE('',#42250);
#1922=PLANE('',#42251);
#1923=PLANE('',#42252);
#1924=PLANE('',#42253);
#1925=PLANE('',#42254);
#1926=PLANE('',#42255);
#1927=PLANE('',#42256);
#1928=PLANE('',#42257);
#1929=PLANE('',#42258);
#1930=PLANE('',#42259);
#1931=PLANE('',#42260);
#1932=PLANE('',#42261);
#1933=PLANE('',#42262);
#1934=PLANE('',#42263);
#1935=PLANE('',#42264);
#1936=PLANE('',#42265);
#1937=PLANE('',#42266);
#1938=PLANE('',#42267);
#1939=PLANE('',#42268);
#1940=PLANE('',#42269);
#1941=PLANE('',#42270);
#1942=PLANE('',#42271);
#1943=PLANE('',#42272);
#1944=PLANE('',#42273);
#1945=PLANE('',#42274);
#1946=PLANE('',#42275);
#1947=PLANE('',#42276);
#1948=PLANE('',#42277);
#1949=PLANE('',#42278);
#1950=PLANE('',#42279);
#1951=PLANE('',#42280);
#1952=PLANE('',#42281);
#1953=PLANE('',#42282);
#1954=PLANE('',#42283);
#1955=PLANE('',#42284);
#1956=PLANE('',#42285);
#1957=PLANE('',#42286);
#1958=PLANE('',#42287);
#1959=PLANE('',#42288);
#1960=PLANE('',#42289);
#1961=PLANE('',#42290);
#1962=PLANE('',#42291);
#1963=PLANE('',#42292);
#1964=PLANE('',#42293);
#1965=PLANE('',#42294);
#1966=PLANE('',#42295);
#1967=PLANE('',#42296);
#1968=PLANE('',#42297);
#1969=PLANE('',#42298);
#1970=PLANE('',#42299);
#1971=PLANE('',#42300);
#1972=PLANE('',#42301);
#1973=PLANE('',#42302);
#1974=PLANE('',#42303);
#1975=PLANE('',#42304);
#1976=PLANE('',#42305);
#1977=PLANE('',#42306);
#1978=PLANE('',#42307);
#1979=PLANE('',#42308);
#1980=PLANE('',#42309);
#1981=PLANE('',#42310);
#1982=PLANE('',#42311);
#1983=PLANE('',#42312);
#1984=PLANE('',#42313);
#1985=PLANE('',#42314);
#1986=PLANE('',#42315);
#1987=PLANE('',#42316);
#1988=PLANE('',#42317);
#1989=PLANE('',#42318);
#1990=PLANE('',#42319);
#1991=PLANE('',#42320);
#1992=PLANE('',#42321);
#1993=PLANE('',#42322);
#1994=PLANE('',#42323);
#1995=PLANE('',#42324);
#1996=PLANE('',#42325);
#1997=PLANE('',#42326);
#1998=PLANE('',#42327);
#1999=PLANE('',#42328);
#2000=PLANE('',#42329);
#2001=PLANE('',#42330);
#2002=PLANE('',#42331);
#2003=PLANE('',#42332);
#2004=PLANE('',#42333);
#2005=PLANE('',#42334);
#2006=PLANE('',#42335);
#2007=PLANE('',#42336);
#2008=PLANE('',#42337);
#2009=PLANE('',#42338);
#2010=PLANE('',#42339);
#2011=PLANE('',#42340);
#2012=PLANE('',#42341);
#2013=PLANE('',#42342);
#2014=PLANE('',#42343);
#2015=PLANE('',#42344);
#2016=PLANE('',#42345);
#2017=PLANE('',#42346);
#2018=PLANE('',#42347);
#2019=PLANE('',#42348);
#2020=PLANE('',#42349);
#2021=PLANE('',#42350);
#2022=PLANE('',#42351);
#2023=PLANE('',#42352);
#2024=PLANE('',#42353);
#2025=PLANE('',#42354);
#2026=PLANE('',#42355);
#2027=PLANE('',#42356);
#2028=PLANE('',#42357);
#2029=PLANE('',#42358);
#2030=PLANE('',#42359);
#2031=PLANE('',#42360);
#2032=PLANE('',#42361);
#2033=PLANE('',#42362);
#2034=PLANE('',#42363);
#2035=PLANE('',#42364);
#2036=PLANE('',#42365);
#2037=PLANE('',#42366);
#2038=PLANE('',#42367);
#2039=PLANE('',#42368);
#2040=PLANE('',#42369);
#2041=PLANE('',#42370);
#2042=PLANE('',#42371);
#2043=PLANE('',#42372);
#2044=PLANE('',#42373);
#2045=PLANE('',#42374);
#2046=PLANE('',#42375);
#2047=PLANE('',#42376);
#2048=PLANE('',#42377);
#2049=PLANE('',#42378);
#2050=PLANE('',#42379);
#2051=PLANE('',#42380);
#2052=PLANE('',#42381);
#2053=PLANE('',#42382);
#2054=PLANE('',#42383);
#2055=PLANE('',#42384);
#2056=PLANE('',#42385);
#2057=PLANE('',#42386);
#2058=PLANE('',#42387);
#2059=PLANE('',#42388);
#2060=PLANE('',#42389);
#2061=PLANE('',#42390);
#2062=PLANE('',#42391);
#2063=PLANE('',#42392);
#2064=PLANE('',#42393);
#2065=PLANE('',#42394);
#2066=PLANE('',#42395);
#2067=PLANE('',#42396);
#2068=PLANE('',#42397);
#2069=PLANE('',#42398);
#2070=PLANE('',#42399);
#2071=PLANE('',#42400);
#2072=PLANE('',#42401);
#2073=PLANE('',#42402);
#2074=PLANE('',#42403);
#2075=PLANE('',#42404);
#2076=PLANE('',#42405);
#2077=PLANE('',#42406);
#2078=PLANE('',#42407);
#2079=PLANE('',#42408);
#2080=PLANE('',#42409);
#2081=PLANE('',#42410);
#2082=PLANE('',#42411);
#2083=PLANE('',#42412);
#2084=PLANE('',#42413);
#2085=PLANE('',#42414);
#2086=PLANE('',#42415);
#2087=PLANE('',#42416);
#2088=PLANE('',#42417);
#2089=PLANE('',#42418);
#2090=PLANE('',#42419);
#2091=PLANE('',#42420);
#2092=PLANE('',#42421);
#2093=PLANE('',#42422);
#2094=PLANE('',#42423);
#2095=PLANE('',#42424);
#2096=PLANE('',#42425);
#2097=PLANE('',#42426);
#2098=PLANE('',#42427);
#2099=PLANE('',#42428);
#2100=PLANE('',#42429);
#2101=PLANE('',#42430);
#2102=PLANE('',#42431);
#2103=PLANE('',#42432);
#2104=PLANE('',#42433);
#2105=PLANE('',#42434);
#2106=PLANE('',#42435);
#2107=PLANE('',#42436);
#2108=PLANE('',#42437);
#2109=PLANE('',#42438);
#2110=PLANE('',#42439);
#2111=PLANE('',#42440);
#2112=PLANE('',#42441);
#2113=PLANE('',#42442);
#2114=PLANE('',#42443);
#2115=PLANE('',#42444);
#2116=PLANE('',#42445);
#2117=PLANE('',#42446);
#2118=PLANE('',#42447);
#2119=PLANE('',#42448);
#2120=PLANE('',#42449);
#2121=PLANE('',#42450);
#2122=PLANE('',#42451);
#2123=PLANE('',#42452);
#2124=PLANE('',#42453);
#2125=PLANE('',#42454);
#2126=PLANE('',#42455);
#2127=PLANE('',#42456);
#2128=PLANE('',#42457);
#2129=PLANE('',#42458);
#2130=PLANE('',#42459);
#2131=PLANE('',#42460);
#2132=PLANE('',#42461);
#2133=PLANE('',#42462);
#2134=PLANE('',#42463);
#2135=PLANE('',#42464);
#2136=PLANE('',#42465);
#2137=PLANE('',#42466);
#2138=PLANE('',#42467);
#2139=PLANE('',#42468);
#2140=PLANE('',#42469);
#2141=PLANE('',#42470);
#2142=PLANE('',#42471);
#2143=PLANE('',#42472);
#2144=PLANE('',#42473);
#2145=PLANE('',#42474);
#2146=PLANE('',#42475);
#2147=PLANE('',#42476);
#2148=PLANE('',#42477);
#2149=PLANE('',#42478);
#2150=PLANE('',#42479);
#2151=PLANE('',#42480);
#2152=PLANE('',#42481);
#2153=PLANE('',#42482);
#2154=PLANE('',#42483);
#2155=PLANE('',#42484);
#2156=PLANE('',#42485);
#2157=PLANE('',#42486);
#2158=PLANE('',#42487);
#2159=PLANE('',#42488);
#2160=PLANE('',#42489);
#2161=PLANE('',#42490);
#2162=PLANE('',#42491);
#2163=PLANE('',#42492);
#2164=PLANE('',#42493);
#2165=PLANE('',#42494);
#2166=PLANE('',#42495);
#2167=PLANE('',#42496);
#2168=PLANE('',#42497);
#2169=PLANE('',#42498);
#2170=PLANE('',#42499);
#2171=PLANE('',#42500);
#2172=PLANE('',#42501);
#2173=PLANE('',#42502);
#2174=PLANE('',#42503);
#2175=PLANE('',#42504);
#2176=PLANE('',#42505);
#2177=PLANE('',#42506);
#2178=PLANE('',#42507);
#2179=PLANE('',#42508);
#2180=PLANE('',#42509);
#2189=TOROIDAL_SURFACE('',#41308,59.5,0.5);
#2190=TOROIDAL_SURFACE('',#41312,61.9494897427832,1.2);
#2191=TOROIDAL_SURFACE('',#41316,59.5,1.3);
#2192=TOROIDAL_SURFACE('',#41319,61.9494897427832,2.);
#3077=FACE_OUTER_BOUND('',#5198,.T.);
#3078=FACE_OUTER_BOUND('',#5199,.T.);
#3079=FACE_OUTER_BOUND('',#5200,.T.);
#3080=FACE_OUTER_BOUND('',#5201,.T.);
#3081=FACE_OUTER_BOUND('',#5202,.T.);
#3082=FACE_OUTER_BOUND('',#5204,.T.);
#3083=FACE_OUTER_BOUND('',#5206,.T.);
#3084=FACE_OUTER_BOUND('',#5207,.T.);
#3085=FACE_OUTER_BOUND('',#5208,.T.);
#3086=FACE_OUTER_BOUND('',#5209,.T.);
#3087=FACE_OUTER_BOUND('',#5210,.T.);
#3088=FACE_OUTER_BOUND('',#5211,.T.);
#3089=FACE_OUTER_BOUND('',#5212,.T.);
#3090=FACE_OUTER_BOUND('',#5213,.T.);
#3091=FACE_OUTER_BOUND('',#5214,.T.);
#3092=FACE_OUTER_BOUND('',#5215,.T.);
#3093=FACE_OUTER_BOUND('',#5216,.T.);
#3094=FACE_OUTER_BOUND('',#5217,.T.);
#3095=FACE_OUTER_BOUND('',#5218,.T.);
#3096=FACE_OUTER_BOUND('',#5219,.T.);
#3097=FACE_OUTER_BOUND('',#5220,.T.);
#3098=FACE_OUTER_BOUND('',#5221,.T.);
#3099=FACE_OUTER_BOUND('',#5222,.T.);
#3100=FACE_OUTER_BOUND('',#5223,.T.);
#3101=FACE_OUTER_BOUND('',#5224,.T.);
#3102=FACE_OUTER_BOUND('',#5225,.T.);
#3103=FACE_OUTER_BOUND('',#5226,.T.);
#3104=FACE_OUTER_BOUND('',#5227,.T.);
#3105=FACE_OUTER_BOUND('',#5228,.T.);
#3106=FACE_OUTER_BOUND('',#5229,.T.);
#3107=FACE_OUTER_BOUND('',#5230,.T.);
#3108=FACE_OUTER_BOUND('',#5231,.T.);
#3109=FACE_OUTER_BOUND('',#5232,.T.);
#3110=FACE_OUTER_BOUND('',#5233,.T.);
#3111=FACE_OUTER_BOUND('',#5234,.T.);
#3112=FACE_OUTER_BOUND('',#5235,.T.);
#3113=FACE_OUTER_BOUND('',#5236,.T.);
#3114=FACE_OUTER_BOUND('',#5237,.T.);
#3115=FACE_OUTER_BOUND('',#5238,.T.);
#3116=FACE_OUTER_BOUND('',#5239,.T.);
#3117=FACE_OUTER_BOUND('',#5240,.T.);
#3118=FACE_OUTER_BOUND('',#5241,.T.);
#3119=FACE_OUTER_BOUND('',#5242,.T.);
#3120=FACE_OUTER_BOUND('',#5243,.T.);
#3121=FACE_OUTER_BOUND('',#5244,.T.);
#3122=FACE_OUTER_BOUND('',#5245,.T.);
#3123=FACE_OUTER_BOUND('',#5246,.T.);
#3124=FACE_OUTER_BOUND('',#5247,.T.);
#3125=FACE_OUTER_BOUND('',#5248,.T.);
#3126=FACE_OUTER_BOUND('',#5249,.T.);
#3127=FACE_OUTER_BOUND('',#5250,.T.);
#3128=FACE_OUTER_BOUND('',#5437,.T.);
#3129=FACE_OUTER_BOUND('',#5624,.T.);
#3130=FACE_OUTER_BOUND('',#5625,.T.);
#3131=FACE_OUTER_BOUND('',#5626,.T.);
#3132=FACE_OUTER_BOUND('',#5627,.T.);
#3133=FACE_OUTER_BOUND('',#5628,.T.);
#3134=FACE_OUTER_BOUND('',#5629,.T.);
#3135=FACE_OUTER_BOUND('',#5630,.T.);
#3136=FACE_OUTER_BOUND('',#5631,.T.);
#3137=FACE_OUTER_BOUND('',#5632,.T.);
#3138=FACE_OUTER_BOUND('',#5633,.T.);
#3139=FACE_OUTER_BOUND('',#5634,.T.);
#3140=FACE_OUTER_BOUND('',#5635,.T.);
#3141=FACE_OUTER_BOUND('',#5636,.T.);
#3142=FACE_OUTER_BOUND('',#5637,.T.);
#3143=FACE_OUTER_BOUND('',#5638,.T.);
#3144=FACE_OUTER_BOUND('',#5639,.T.);
#3145=FACE_OUTER_BOUND('',#5640,.T.);
#3146=FACE_OUTER_BOUND('',#5641,.T.);
#3147=FACE_OUTER_BOUND('',#5642,.T.);
#3148=FACE_OUTER_BOUND('',#5643,.T.);
#3149=FACE_OUTER_BOUND('',#5644,.T.);
#3150=FACE_OUTER_BOUND('',#5645,.T.);
#3151=FACE_OUTER_BOUND('',#5646,.T.);
#3152=FACE_OUTER_BOUND('',#5647,.T.);
#3153=FACE_OUTER_BOUND('',#5648,.T.);
#3154=FACE_OUTER_BOUND('',#5649,.T.);
#3155=FACE_OUTER_BOUND('',#5650,.T.);
#3156=FACE_OUTER_BOUND('',#5651,.T.);
#3157=FACE_OUTER_BOUND('',#5652,.T.);
#3158=FACE_OUTER_BOUND('',#5653,.T.);
#3159=FACE_OUTER_BOUND('',#5654,.T.);
#3160=FACE_OUTER_BOUND('',#5655,.T.);
#3161=FACE_OUTER_BOUND('',#5656,.T.);
#3162=FACE_OUTER_BOUND('',#5657,.T.);
#3163=FACE_OUTER_BOUND('',#5658,.T.);
#3164=FACE_OUTER_BOUND('',#5659,.T.);
#3165=FACE_OUTER_BOUND('',#5660,.T.);
#3166=FACE_OUTER_BOUND('',#5661,.T.);
#3167=FACE_OUTER_BOUND('',#5662,.T.);
#3168=FACE_OUTER_BOUND('',#5663,.T.);
#3169=FACE_OUTER_BOUND('',#5664,.T.);
#3170=FACE_OUTER_BOUND('',#5665,.T.);
#3171=FACE_OUTER_BOUND('',#5666,.T.);
#3172=FACE_OUTER_BOUND('',#5667,.T.);
#3173=FACE_OUTER_BOUND('',#5668,.T.);
#3174=FACE_OUTER_BOUND('',#5669,.T.);
#3175=FACE_OUTER_BOUND('',#5670,.T.);
#3176=FACE_OUTER_BOUND('',#5671,.T.);
#3177=FACE_OUTER_BOUND('',#5672,.T.);
#3178=FACE_OUTER_BOUND('',#5673,.T.);
#3179=FACE_OUTER_BOUND('',#5674,.T.);
#3180=FACE_OUTER_BOUND('',#5675,.T.);
#3181=FACE_OUTER_BOUND('',#5676,.T.);
#3182=FACE_OUTER_BOUND('',#5677,.T.);
#3183=FACE_OUTER_BOUND('',#5678,.T.);
#3184=FACE_OUTER_BOUND('',#5679,.T.);
#3185=FACE_OUTER_BOUND('',#5680,.T.);
#3186=FACE_OUTER_BOUND('',#5681,.T.);
#3187=FACE_OUTER_BOUND('',#5682,.T.);
#3188=FACE_OUTER_BOUND('',#5683,.T.);
#3189=FACE_OUTER_BOUND('',#5684,.T.);
#3190=FACE_OUTER_BOUND('',#5685,.T.);
#3191=FACE_OUTER_BOUND('',#5686,.T.);
#3192=FACE_OUTER_BOUND('',#5687,.T.);
#3193=FACE_OUTER_BOUND('',#5688,.T.);
#3194=FACE_OUTER_BOUND('',#5689,.T.);
#3195=FACE_OUTER_BOUND('',#5690,.T.);
#3196=FACE_OUTER_BOUND('',#5691,.T.);
#3197=FACE_OUTER_BOUND('',#5692,.T.);
#3198=FACE_OUTER_BOUND('',#5693,.T.);
#3199=FACE_OUTER_BOUND('',#5694,.T.);
#3200=FACE_OUTER_BOUND('',#5695,.T.);
#3201=FACE_OUTER_BOUND('',#5696,.T.);
#3202=FACE_OUTER_BOUND('',#5697,.T.);
#3203=FACE_OUTER_BOUND('',#5698,.T.);
#3204=FACE_OUTER_BOUND('',#5699,.T.);
#3205=FACE_OUTER_BOUND('',#5700,.T.);
#3206=FACE_OUTER_BOUND('',#5701,.T.);
#3207=FACE_OUTER_BOUND('',#5702,.T.);
#3208=FACE_OUTER_BOUND('',#5703,.T.);
#3209=FACE_OUTER_BOUND('',#5704,.T.);
#3210=FACE_OUTER_BOUND('',#5705,.T.);
#3211=FACE_OUTER_BOUND('',#5706,.T.);
#3212=FACE_OUTER_BOUND('',#5707,.T.);
#3213=FACE_OUTER_BOUND('',#5708,.T.);
#3214=FACE_OUTER_BOUND('',#5709,.T.);
#3215=FACE_OUTER_BOUND('',#5710,.T.);
#3216=FACE_OUTER_BOUND('',#5711,.T.);
#3217=FACE_OUTER_BOUND('',#5712,.T.);
#3218=FACE_OUTER_BOUND('',#5713,.T.);
#3219=FACE_OUTER_BOUND('',#5714,.T.);
#3220=FACE_OUTER_BOUND('',#5715,.T.);
#3221=FACE_OUTER_BOUND('',#5716,.T.);
#3222=FACE_OUTER_BOUND('',#5717,.T.);
#3223=FACE_OUTER_BOUND('',#5718,.T.);
#3224=FACE_OUTER_BOUND('',#5719,.T.);
#3225=FACE_OUTER_BOUND('',#5720,.T.);
#3226=FACE_OUTER_BOUND('',#5721,.T.);
#3227=FACE_OUTER_BOUND('',#5722,.T.);
#3228=FACE_OUTER_BOUND('',#5723,.T.);
#3229=FACE_OUTER_BOUND('',#5724,.T.);
#3230=FACE_OUTER_BOUND('',#5725,.T.);
#3231=FACE_OUTER_BOUND('',#5726,.T.);
#3232=FACE_OUTER_BOUND('',#5727,.T.);
#3233=FACE_OUTER_BOUND('',#5728,.T.);
#3234=FACE_OUTER_BOUND('',#5729,.T.);
#3235=FACE_OUTER_BOUND('',#5730,.T.);
#3236=FACE_OUTER_BOUND('',#5731,.T.);
#3237=FACE_OUTER_BOUND('',#5732,.T.);
#3238=FACE_OUTER_BOUND('',#5733,.T.);
#3239=FACE_OUTER_BOUND('',#5734,.T.);
#3240=FACE_OUTER_BOUND('',#5735,.T.);
#3241=FACE_OUTER_BOUND('',#5736,.T.);
#3242=FACE_OUTER_BOUND('',#5737,.T.);
#3243=FACE_OUTER_BOUND('',#5738,.T.);
#3244=FACE_OUTER_BOUND('',#5739,.T.);
#3245=FACE_OUTER_BOUND('',#5740,.T.);
#3246=FACE_OUTER_BOUND('',#5741,.T.);
#3247=FACE_OUTER_BOUND('',#5742,.T.);
#3248=FACE_OUTER_BOUND('',#5743,.T.);
#3249=FACE_OUTER_BOUND('',#5744,.T.);
#3250=FACE_OUTER_BOUND('',#5745,.T.);
#3251=FACE_OUTER_BOUND('',#5746,.T.);
#3252=FACE_OUTER_BOUND('',#5747,.T.);
#3253=FACE_OUTER_BOUND('',#5748,.T.);
#3254=FACE_OUTER_BOUND('',#5749,.T.);
#3255=FACE_OUTER_BOUND('',#5750,.T.);
#3256=FACE_OUTER_BOUND('',#5751,.T.);
#3257=FACE_OUTER_BOUND('',#5752,.T.);
#3258=FACE_OUTER_BOUND('',#5753,.T.);
#3259=FACE_OUTER_BOUND('',#5754,.T.);
#3260=FACE_OUTER_BOUND('',#5755,.T.);
#3261=FACE_OUTER_BOUND('',#5756,.T.);
#3262=FACE_OUTER_BOUND('',#5757,.T.);
#3263=FACE_OUTER_BOUND('',#5758,.T.);
#3264=FACE_OUTER_BOUND('',#5759,.T.);
#3265=FACE_OUTER_BOUND('',#5760,.T.);
#3266=FACE_OUTER_BOUND('',#5761,.T.);
#3267=FACE_OUTER_BOUND('',#5762,.T.);
#3268=FACE_OUTER_BOUND('',#5763,.T.);
#3269=FACE_OUTER_BOUND('',#5764,.T.);
#3270=FACE_OUTER_BOUND('',#5765,.T.);
#3271=FACE_OUTER_BOUND('',#5766,.T.);
#3272=FACE_OUTER_BOUND('',#5767,.T.);
#3273=FACE_OUTER_BOUND('',#5768,.T.);
#3274=FACE_OUTER_BOUND('',#5769,.T.);
#3275=FACE_OUTER_BOUND('',#5770,.T.);
#3276=FACE_OUTER_BOUND('',#5771,.T.);
#3277=FACE_OUTER_BOUND('',#5772,.T.);
#3278=FACE_OUTER_BOUND('',#5773,.T.);
#3279=FACE_OUTER_BOUND('',#5774,.T.);
#3280=FACE_OUTER_BOUND('',#5775,.T.);
#3281=FACE_OUTER_BOUND('',#5776,.T.);
#3282=FACE_OUTER_BOUND('',#5777,.T.);
#3283=FACE_OUTER_BOUND('',#5778,.T.);
#3284=FACE_OUTER_BOUND('',#5779,.T.);
#3285=FACE_OUTER_BOUND('',#5780,.T.);
#3286=FACE_OUTER_BOUND('',#5781,.T.);
#3287=FACE_OUTER_BOUND('',#5782,.T.);
#3288=FACE_OUTER_BOUND('',#5783,.T.);
#3289=FACE_OUTER_BOUND('',#5784,.T.);
#3290=FACE_OUTER_BOUND('',#5785,.T.);
#3291=FACE_OUTER_BOUND('',#5786,.T.);
#3292=FACE_OUTER_BOUND('',#5787,.T.);
#3293=FACE_OUTER_BOUND('',#5788,.T.);
#3294=FACE_OUTER_BOUND('',#5789,.T.);
#3295=FACE_OUTER_BOUND('',#5790,.T.);
#3296=FACE_OUTER_BOUND('',#5791,.T.);
#3297=FACE_OUTER_BOUND('',#5792,.T.);
#3298=FACE_OUTER_BOUND('',#5793,.T.);
#3299=FACE_OUTER_BOUND('',#5794,.T.);
#3300=FACE_OUTER_BOUND('',#5795,.T.);
#3301=FACE_OUTER_BOUND('',#5796,.T.);
#3302=FACE_OUTER_BOUND('',#5797,.T.);
#3303=FACE_OUTER_BOUND('',#5798,.T.);
#3304=FACE_OUTER_BOUND('',#5799,.T.);
#3305=FACE_OUTER_BOUND('',#5800,.T.);
#3306=FACE_OUTER_BOUND('',#5801,.T.);
#3307=FACE_OUTER_BOUND('',#5802,.T.);
#3308=FACE_OUTER_BOUND('',#5803,.T.);
#3309=FACE_OUTER_BOUND('',#5804,.T.);
#3310=FACE_OUTER_BOUND('',#5805,.T.);
#3311=FACE_OUTER_BOUND('',#5806,.T.);
#3312=FACE_OUTER_BOUND('',#5807,.T.);
#3313=FACE_OUTER_BOUND('',#5808,.T.);
#3314=FACE_OUTER_BOUND('',#5809,.T.);
#3315=FACE_OUTER_BOUND('',#5810,.T.);
#3316=FACE_OUTER_BOUND('',#5811,.T.);
#3317=FACE_OUTER_BOUND('',#5812,.T.);
#3318=FACE_OUTER_BOUND('',#5813,.T.);
#3319=FACE_OUTER_BOUND('',#5814,.T.);
#3320=FACE_OUTER_BOUND('',#5815,.T.);
#3321=FACE_OUTER_BOUND('',#5816,.T.);
#3322=FACE_OUTER_BOUND('',#5817,.T.);
#3323=FACE_OUTER_BOUND('',#5818,.T.);
#3324=FACE_OUTER_BOUND('',#5819,.T.);
#3325=FACE_OUTER_BOUND('',#5820,.T.);
#3326=FACE_OUTER_BOUND('',#5821,.T.);
#3327=FACE_OUTER_BOUND('',#5822,.T.);
#3328=FACE_OUTER_BOUND('',#5823,.T.);
#3329=FACE_OUTER_BOUND('',#5824,.T.);
#3330=FACE_OUTER_BOUND('',#5825,.T.);
#3331=FACE_OUTER_BOUND('',#5826,.T.);
#3332=FACE_OUTER_BOUND('',#5827,.T.);
#3333=FACE_OUTER_BOUND('',#5828,.T.);
#3334=FACE_OUTER_BOUND('',#5829,.T.);
#3335=FACE_OUTER_BOUND('',#5830,.T.);
#3336=FACE_OUTER_BOUND('',#5831,.T.);
#3337=FACE_OUTER_BOUND('',#5832,.T.);
#3338=FACE_OUTER_BOUND('',#5833,.T.);
#3339=FACE_OUTER_BOUND('',#5834,.T.);
#3340=FACE_OUTER_BOUND('',#5835,.T.);
#3341=FACE_OUTER_BOUND('',#5836,.T.);
#3342=FACE_OUTER_BOUND('',#5837,.T.);
#3343=FACE_OUTER_BOUND('',#5838,.T.);
#3344=FACE_OUTER_BOUND('',#5839,.T.);
#3345=FACE_OUTER_BOUND('',#5840,.T.);
#3346=FACE_OUTER_BOUND('',#5841,.T.);
#3347=FACE_OUTER_BOUND('',#5842,.T.);
#3348=FACE_OUTER_BOUND('',#5843,.T.);
#3349=FACE_OUTER_BOUND('',#5844,.T.);
#3350=FACE_OUTER_BOUND('',#5845,.T.);
#3351=FACE_OUTER_BOUND('',#5846,.T.);
#3352=FACE_OUTER_BOUND('',#5847,.T.);
#3353=FACE_OUTER_BOUND('',#5848,.T.);
#3354=FACE_OUTER_BOUND('',#5849,.T.);
#3355=FACE_OUTER_BOUND('',#5850,.T.);
#3356=FACE_OUTER_BOUND('',#5851,.T.);
#3357=FACE_OUTER_BOUND('',#5852,.T.);
#3358=FACE_OUTER_BOUND('',#5853,.T.);
#3359=FACE_OUTER_BOUND('',#5854,.T.);
#3360=FACE_OUTER_BOUND('',#5855,.T.);
#3361=FACE_OUTER_BOUND('',#5856,.T.);
#3362=FACE_OUTER_BOUND('',#5857,.T.);
#3363=FACE_OUTER_BOUND('',#5858,.T.);
#3364=FACE_OUTER_BOUND('',#5859,.T.);
#3365=FACE_OUTER_BOUND('',#5860,.T.);
#3366=FACE_OUTER_BOUND('',#5861,.T.);
#3367=FACE_OUTER_BOUND('',#5862,.T.);
#3368=FACE_OUTER_BOUND('',#5863,.T.);
#3369=FACE_OUTER_BOUND('',#5864,.T.);
#3370=FACE_OUTER_BOUND('',#5865,.T.);
#3371=FACE_OUTER_BOUND('',#5866,.T.);
#3372=FACE_OUTER_BOUND('',#5867,.T.);
#3373=FACE_OUTER_BOUND('',#5868,.T.);
#3374=FACE_OUTER_BOUND('',#5869,.T.);
#3375=FACE_OUTER_BOUND('',#5870,.T.);
#3376=FACE_OUTER_BOUND('',#5871,.T.);
#3377=FACE_OUTER_BOUND('',#5872,.T.);
#3378=FACE_OUTER_BOUND('',#5873,.T.);
#3379=FACE_OUTER_BOUND('',#5874,.T.);
#3380=FACE_OUTER_BOUND('',#5875,.T.);
#3381=FACE_OUTER_BOUND('',#5876,.T.);
#3382=FACE_OUTER_BOUND('',#5877,.T.);
#3383=FACE_OUTER_BOUND('',#5878,.T.);
#3384=FACE_OUTER_BOUND('',#5879,.T.);
#3385=FACE_OUTER_BOUND('',#5880,.T.);
#3386=FACE_OUTER_BOUND('',#5881,.T.);
#3387=FACE_OUTER_BOUND('',#5882,.T.);
#3388=FACE_OUTER_BOUND('',#5883,.T.);
#3389=FACE_OUTER_BOUND('',#5884,.T.);
#3390=FACE_OUTER_BOUND('',#5885,.T.);
#3391=FACE_OUTER_BOUND('',#5886,.T.);
#3392=FACE_OUTER_BOUND('',#5887,.T.);
#3393=FACE_OUTER_BOUND('',#5888,.T.);
#3394=FACE_OUTER_BOUND('',#5889,.T.);
#3395=FACE_OUTER_BOUND('',#5890,.T.);
#3396=FACE_OUTER_BOUND('',#5891,.T.);
#3397=FACE_OUTER_BOUND('',#5892,.T.);
#3398=FACE_OUTER_BOUND('',#5893,.T.);
#3399=FACE_OUTER_BOUND('',#5894,.T.);
#3400=FACE_OUTER_BOUND('',#5895,.T.);
#3401=FACE_OUTER_BOUND('',#5896,.T.);
#3402=FACE_OUTER_BOUND('',#5897,.T.);
#3403=FACE_OUTER_BOUND('',#5898,.T.);
#3404=FACE_OUTER_BOUND('',#5899,.T.);
#3405=FACE_OUTER_BOUND('',#5900,.T.);
#3406=FACE_OUTER_BOUND('',#5901,.T.);
#3407=FACE_OUTER_BOUND('',#5902,.T.);
#3408=FACE_OUTER_BOUND('',#5903,.T.);
#3409=FACE_OUTER_BOUND('',#5904,.T.);
#3410=FACE_OUTER_BOUND('',#5905,.T.);
#3411=FACE_OUTER_BOUND('',#5906,.T.);
#3412=FACE_OUTER_BOUND('',#5907,.T.);
#3413=FACE_OUTER_BOUND('',#5908,.T.);
#3414=FACE_OUTER_BOUND('',#5909,.T.);
#3415=FACE_OUTER_BOUND('',#5910,.T.);
#3416=FACE_OUTER_BOUND('',#5911,.T.);
#3417=FACE_OUTER_BOUND('',#5912,.T.);
#3418=FACE_OUTER_BOUND('',#5913,.T.);
#3419=FACE_OUTER_BOUND('',#5914,.T.);
#3420=FACE_OUTER_BOUND('',#5915,.T.);
#3421=FACE_OUTER_BOUND('',#5916,.T.);
#3422=FACE_OUTER_BOUND('',#5917,.T.);
#3423=FACE_OUTER_BOUND('',#5918,.T.);
#3424=FACE_OUTER_BOUND('',#5919,.T.);
#3425=FACE_OUTER_BOUND('',#5920,.T.);
#3426=FACE_OUTER_BOUND('',#5921,.T.);
#3427=FACE_OUTER_BOUND('',#5922,.T.);
#3428=FACE_OUTER_BOUND('',#5923,.T.);
#3429=FACE_OUTER_BOUND('',#5924,.T.);
#3430=FACE_OUTER_BOUND('',#5925,.T.);
#3431=FACE_OUTER_BOUND('',#5926,.T.);
#3432=FACE_OUTER_BOUND('',#5927,.T.);
#3433=FACE_OUTER_BOUND('',#5928,.T.);
#3434=FACE_OUTER_BOUND('',#5929,.T.);
#3435=FACE_OUTER_BOUND('',#5930,.T.);
#3436=FACE_OUTER_BOUND('',#5931,.T.);
#3437=FACE_OUTER_BOUND('',#5932,.T.);
#3438=FACE_OUTER_BOUND('',#5933,.T.);
#3439=FACE_OUTER_BOUND('',#5934,.T.);
#3440=FACE_OUTER_BOUND('',#5935,.T.);
#3441=FACE_OUTER_BOUND('',#5936,.T.);
#3442=FACE_OUTER_BOUND('',#5937,.T.);
#3443=FACE_OUTER_BOUND('',#5938,.T.);
#3444=FACE_OUTER_BOUND('',#5939,.T.);
#3445=FACE_OUTER_BOUND('',#5940,.T.);
#3446=FACE_OUTER_BOUND('',#5941,.T.);
#3447=FACE_OUTER_BOUND('',#5942,.T.);
#3448=FACE_OUTER_BOUND('',#5943,.T.);
#3449=FACE_OUTER_BOUND('',#5944,.T.);
#3450=FACE_OUTER_BOUND('',#5945,.T.);
#3451=FACE_OUTER_BOUND('',#5946,.T.);
#3452=FACE_OUTER_BOUND('',#5947,.T.);
#3453=FACE_OUTER_BOUND('',#5948,.T.);
#3454=FACE_OUTER_BOUND('',#5949,.T.);
#3455=FACE_OUTER_BOUND('',#5950,.T.);
#3456=FACE_OUTER_BOUND('',#5951,.T.);
#3457=FACE_OUTER_BOUND('',#5952,.T.);
#3458=FACE_OUTER_BOUND('',#5953,.T.);
#3459=FACE_OUTER_BOUND('',#5954,.T.);
#3460=FACE_OUTER_BOUND('',#5955,.T.);
#3461=FACE_OUTER_BOUND('',#5956,.T.);
#3462=FACE_OUTER_BOUND('',#5957,.T.);
#3463=FACE_OUTER_BOUND('',#5958,.T.);
#3464=FACE_OUTER_BOUND('',#5959,.T.);
#3465=FACE_OUTER_BOUND('',#5960,.T.);
#3466=FACE_OUTER_BOUND('',#5961,.T.);
#3467=FACE_OUTER_BOUND('',#5962,.T.);
#3468=FACE_OUTER_BOUND('',#5963,.T.);
#3469=FACE_OUTER_BOUND('',#5964,.T.);
#3470=FACE_OUTER_BOUND('',#5965,.T.);
#3471=FACE_OUTER_BOUND('',#5966,.T.);
#3472=FACE_OUTER_BOUND('',#5967,.T.);
#3473=FACE_OUTER_BOUND('',#5968,.T.);
#3474=FACE_OUTER_BOUND('',#5969,.T.);
#3475=FACE_OUTER_BOUND('',#5970,.T.);
#3476=FACE_OUTER_BOUND('',#5971,.T.);
#3477=FACE_OUTER_BOUND('',#5972,.T.);
#3478=FACE_OUTER_BOUND('',#5973,.T.);
#3479=FACE_OUTER_BOUND('',#5974,.T.);
#3480=FACE_OUTER_BOUND('',#5975,.T.);
#3481=FACE_OUTER_BOUND('',#5976,.T.);
#3482=FACE_OUTER_BOUND('',#5977,.T.);
#3483=FACE_OUTER_BOUND('',#5978,.T.);
#3484=FACE_OUTER_BOUND('',#5979,.T.);
#3485=FACE_OUTER_BOUND('',#5980,.T.);
#3486=FACE_OUTER_BOUND('',#5981,.T.);
#3487=FACE_OUTER_BOUND('',#5982,.T.);
#3488=FACE_OUTER_BOUND('',#5983,.T.);
#3489=FACE_OUTER_BOUND('',#5984,.T.);
#3490=FACE_OUTER_BOUND('',#5985,.T.);
#3491=FACE_OUTER_BOUND('',#5986,.T.);
#3492=FACE_OUTER_BOUND('',#5987,.T.);
#3493=FACE_OUTER_BOUND('',#5988,.T.);
#3494=FACE_OUTER_BOUND('',#5989,.T.);
#3495=FACE_OUTER_BOUND('',#5990,.T.);
#3496=FACE_OUTER_BOUND('',#5991,.T.);
#3497=FACE_OUTER_BOUND('',#5992,.T.);
#3498=FACE_OUTER_BOUND('',#5993,.T.);
#3499=FACE_OUTER_BOUND('',#5994,.T.);
#3500=FACE_OUTER_BOUND('',#5995,.T.);
#3501=FACE_OUTER_BOUND('',#5996,.T.);
#3502=FACE_OUTER_BOUND('',#5997,.T.);
#3503=FACE_OUTER_BOUND('',#5998,.T.);
#3504=FACE_OUTER_BOUND('',#5999,.T.);
#3505=FACE_OUTER_BOUND('',#6000,.T.);
#3506=FACE_OUTER_BOUND('',#6001,.T.);
#3507=FACE_OUTER_BOUND('',#6002,.T.);
#3508=FACE_OUTER_BOUND('',#6003,.T.);
#3509=FACE_OUTER_BOUND('',#6004,.T.);
#3510=FACE_OUTER_BOUND('',#6005,.T.);
#3511=FACE_OUTER_BOUND('',#6006,.T.);
#3512=FACE_OUTER_BOUND('',#6007,.T.);
#3513=FACE_OUTER_BOUND('',#6008,.T.);
#3514=FACE_OUTER_BOUND('',#6009,.T.);
#3515=FACE_OUTER_BOUND('',#6010,.T.);
#3516=FACE_OUTER_BOUND('',#6011,.T.);
#3517=FACE_OUTER_BOUND('',#6012,.T.);
#3518=FACE_OUTER_BOUND('',#6013,.T.);
#3519=FACE_OUTER_BOUND('',#6014,.T.);
#3520=FACE_OUTER_BOUND('',#6015,.T.);
#3521=FACE_OUTER_BOUND('',#6016,.T.);
#3522=FACE_OUTER_BOUND('',#6017,.T.);
#3523=FACE_OUTER_BOUND('',#6018,.T.);
#3524=FACE_OUTER_BOUND('',#6019,.T.);
#3525=FACE_OUTER_BOUND('',#6020,.T.);
#3526=FACE_OUTER_BOUND('',#6021,.T.);
#3527=FACE_OUTER_BOUND('',#6022,.T.);
#3528=FACE_OUTER_BOUND('',#6023,.T.);
#3529=FACE_OUTER_BOUND('',#6024,.T.);
#3530=FACE_OUTER_BOUND('',#6025,.T.);
#3531=FACE_OUTER_BOUND('',#6026,.T.);
#3532=FACE_OUTER_BOUND('',#6027,.T.);
#3533=FACE_OUTER_BOUND('',#6028,.T.);
#3534=FACE_OUTER_BOUND('',#6029,.T.);
#3535=FACE_OUTER_BOUND('',#6030,.T.);
#3536=FACE_OUTER_BOUND('',#6031,.T.);
#3537=FACE_OUTER_BOUND('',#6032,.T.);
#3538=FACE_OUTER_BOUND('',#6033,.T.);
#3539=FACE_OUTER_BOUND('',#6034,.T.);
#3540=FACE_OUTER_BOUND('',#6035,.T.);
#3541=FACE_OUTER_BOUND('',#6036,.T.);
#3542=FACE_OUTER_BOUND('',#6037,.T.);
#3543=FACE_OUTER_BOUND('',#6038,.T.);
#3544=FACE_OUTER_BOUND('',#6039,.T.);
#3545=FACE_OUTER_BOUND('',#6040,.T.);
#3546=FACE_OUTER_BOUND('',#6041,.T.);
#3547=FACE_OUTER_BOUND('',#6042,.T.);
#3548=FACE_OUTER_BOUND('',#6043,.T.);
#3549=FACE_OUTER_BOUND('',#6044,.T.);
#3550=FACE_OUTER_BOUND('',#6045,.T.);
#3551=FACE_OUTER_BOUND('',#6046,.T.);
#3552=FACE_OUTER_BOUND('',#6047,.T.);
#3553=FACE_OUTER_BOUND('',#6048,.T.);
#3554=FACE_OUTER_BOUND('',#6049,.T.);
#3555=FACE_OUTER_BOUND('',#6050,.T.);
#3556=FACE_OUTER_BOUND('',#6051,.T.);
#3557=FACE_OUTER_BOUND('',#6052,.T.);
#3558=FACE_OUTER_BOUND('',#6053,.T.);
#3559=FACE_OUTER_BOUND('',#6054,.T.);
#3560=FACE_OUTER_BOUND('',#6055,.T.);
#3561=FACE_OUTER_BOUND('',#6056,.T.);
#3562=FACE_OUTER_BOUND('',#6057,.T.);
#3563=FACE_OUTER_BOUND('',#6058,.T.);
#3564=FACE_OUTER_BOUND('',#6059,.T.);
#3565=FACE_OUTER_BOUND('',#6060,.T.);
#3566=FACE_OUTER_BOUND('',#6061,.T.);
#3567=FACE_OUTER_BOUND('',#6062,.T.);
#3568=FACE_OUTER_BOUND('',#6063,.T.);
#3569=FACE_OUTER_BOUND('',#6064,.T.);
#3570=FACE_OUTER_BOUND('',#6065,.T.);
#3571=FACE_OUTER_BOUND('',#6066,.T.);
#3572=FACE_OUTER_BOUND('',#6067,.T.);
#3573=FACE_OUTER_BOUND('',#6068,.T.);
#3574=FACE_OUTER_BOUND('',#6069,.T.);
#3575=FACE_OUTER_BOUND('',#6070,.T.);
#3576=FACE_OUTER_BOUND('',#6071,.T.);
#3577=FACE_OUTER_BOUND('',#6072,.T.);
#3578=FACE_OUTER_BOUND('',#6073,.T.);
#3579=FACE_OUTER_BOUND('',#6074,.T.);
#3580=FACE_OUTER_BOUND('',#6075,.T.);
#3581=FACE_OUTER_BOUND('',#6076,.T.);
#3582=FACE_OUTER_BOUND('',#6077,.T.);
#3583=FACE_OUTER_BOUND('',#6078,.T.);
#3584=FACE_OUTER_BOUND('',#6079,.T.);
#3585=FACE_OUTER_BOUND('',#6080,.T.);
#3586=FACE_OUTER_BOUND('',#6081,.T.);
#3587=FACE_OUTER_BOUND('',#6082,.T.);
#3588=FACE_OUTER_BOUND('',#6083,.T.);
#3589=FACE_OUTER_BOUND('',#6084,.T.);
#3590=FACE_OUTER_BOUND('',#6085,.T.);
#3591=FACE_OUTER_BOUND('',#6086,.T.);
#3592=FACE_OUTER_BOUND('',#6087,.T.);
#3593=FACE_OUTER_BOUND('',#6088,.T.);
#3594=FACE_OUTER_BOUND('',#6089,.T.);
#3595=FACE_OUTER_BOUND('',#6090,.T.);
#3596=FACE_OUTER_BOUND('',#6091,.T.);
#3597=FACE_OUTER_BOUND('',#6092,.T.);
#3598=FACE_OUTER_BOUND('',#6093,.T.);
#3599=FACE_OUTER_BOUND('',#6094,.T.);
#3600=FACE_OUTER_BOUND('',#6095,.T.);
#3601=FACE_OUTER_BOUND('',#6096,.T.);
#3602=FACE_OUTER_BOUND('',#6097,.T.);
#3603=FACE_OUTER_BOUND('',#6098,.T.);
#3604=FACE_OUTER_BOUND('',#6099,.T.);
#3605=FACE_OUTER_BOUND('',#6100,.T.);
#3606=FACE_OUTER_BOUND('',#6101,.T.);
#3607=FACE_OUTER_BOUND('',#6102,.T.);
#3608=FACE_OUTER_BOUND('',#6103,.T.);
#3609=FACE_OUTER_BOUND('',#6104,.T.);
#3610=FACE_OUTER_BOUND('',#6105,.T.);
#3611=FACE_OUTER_BOUND('',#6106,.T.);
#3612=FACE_OUTER_BOUND('',#6107,.T.);
#3613=FACE_OUTER_BOUND('',#6108,.T.);
#3614=FACE_OUTER_BOUND('',#6109,.T.);
#3615=FACE_OUTER_BOUND('',#6110,.T.);
#3616=FACE_OUTER_BOUND('',#6111,.T.);
#3617=FACE_OUTER_BOUND('',#6112,.T.);
#3618=FACE_OUTER_BOUND('',#6113,.T.);
#3619=FACE_OUTER_BOUND('',#6114,.T.);
#3620=FACE_OUTER_BOUND('',#6115,.T.);
#3621=FACE_OUTER_BOUND('',#6116,.T.);
#3622=FACE_OUTER_BOUND('',#6117,.T.);
#3623=FACE_OUTER_BOUND('',#6118,.T.);
#3624=FACE_OUTER_BOUND('',#6119,.T.);
#3625=FACE_OUTER_BOUND('',#6120,.T.);
#3626=FACE_OUTER_BOUND('',#6121,.T.);
#3627=FACE_OUTER_BOUND('',#6122,.T.);
#3628=FACE_OUTER_BOUND('',#6123,.T.);
#3629=FACE_OUTER_BOUND('',#6124,.T.);
#3630=FACE_OUTER_BOUND('',#6125,.T.);
#3631=FACE_OUTER_BOUND('',#6126,.T.);
#3632=FACE_OUTER_BOUND('',#6127,.T.);
#3633=FACE_OUTER_BOUND('',#6128,.T.);
#3634=FACE_OUTER_BOUND('',#6129,.T.);
#3635=FACE_OUTER_BOUND('',#6130,.T.);
#3636=FACE_OUTER_BOUND('',#6131,.T.);
#3637=FACE_OUTER_BOUND('',#6132,.T.);
#3638=FACE_OUTER_BOUND('',#6133,.T.);
#3639=FACE_OUTER_BOUND('',#6134,.T.);
#3640=FACE_OUTER_BOUND('',#6135,.T.);
#3641=FACE_OUTER_BOUND('',#6136,.T.);
#3642=FACE_OUTER_BOUND('',#6137,.T.);
#3643=FACE_OUTER_BOUND('',#6138,.T.);
#3644=FACE_OUTER_BOUND('',#6139,.T.);
#3645=FACE_OUTER_BOUND('',#6140,.T.);
#3646=FACE_OUTER_BOUND('',#6141,.T.);
#3647=FACE_OUTER_BOUND('',#6142,.T.);
#3648=FACE_OUTER_BOUND('',#6143,.T.);
#3649=FACE_OUTER_BOUND('',#6144,.T.);
#3650=FACE_OUTER_BOUND('',#6145,.T.);
#3651=FACE_OUTER_BOUND('',#6146,.T.);
#3652=FACE_OUTER_BOUND('',#6147,.T.);
#3653=FACE_OUTER_BOUND('',#6148,.T.);
#3654=FACE_OUTER_BOUND('',#6149,.T.);
#3655=FACE_OUTER_BOUND('',#6150,.T.);
#3656=FACE_OUTER_BOUND('',#6151,.T.);
#3657=FACE_OUTER_BOUND('',#6152,.T.);
#3658=FACE_OUTER_BOUND('',#6153,.T.);
#3659=FACE_OUTER_BOUND('',#6154,.T.);
#3660=FACE_OUTER_BOUND('',#6155,.T.);
#3661=FACE_OUTER_BOUND('',#6156,.T.);
#3662=FACE_OUTER_BOUND('',#6157,.T.);
#3663=FACE_OUTER_BOUND('',#6158,.T.);
#3664=FACE_OUTER_BOUND('',#6159,.T.);
#3665=FACE_OUTER_BOUND('',#6160,.T.);
#3666=FACE_OUTER_BOUND('',#6161,.T.);
#3667=FACE_OUTER_BOUND('',#6162,.T.);
#3668=FACE_OUTER_BOUND('',#6163,.T.);
#3669=FACE_OUTER_BOUND('',#6164,.T.);
#3670=FACE_OUTER_BOUND('',#6165,.T.);
#3671=FACE_OUTER_BOUND('',#6166,.T.);
#3672=FACE_OUTER_BOUND('',#6167,.T.);
#3673=FACE_OUTER_BOUND('',#6168,.T.);
#3674=FACE_OUTER_BOUND('',#6169,.T.);
#3675=FACE_OUTER_BOUND('',#6170,.T.);
#3676=FACE_OUTER_BOUND('',#6171,.T.);
#3677=FACE_OUTER_BOUND('',#6172,.T.);
#3678=FACE_OUTER_BOUND('',#6173,.T.);
#3679=FACE_OUTER_BOUND('',#6174,.T.);
#3680=FACE_OUTER_BOUND('',#6175,.T.);
#3681=FACE_OUTER_BOUND('',#6176,.T.);
#3682=FACE_OUTER_BOUND('',#6177,.T.);
#3683=FACE_OUTER_BOUND('',#6178,.T.);
#3684=FACE_OUTER_BOUND('',#6179,.T.);
#3685=FACE_OUTER_BOUND('',#6180,.T.);
#3686=FACE_OUTER_BOUND('',#6181,.T.);
#3687=FACE_OUTER_BOUND('',#6182,.T.);
#3688=FACE_OUTER_BOUND('',#6183,.T.);
#3689=FACE_OUTER_BOUND('',#6184,.T.);
#3690=FACE_OUTER_BOUND('',#6185,.T.);
#3691=FACE_OUTER_BOUND('',#6186,.T.);
#3692=FACE_OUTER_BOUND('',#6187,.T.);
#3693=FACE_OUTER_BOUND('',#6188,.T.);
#3694=FACE_OUTER_BOUND('',#6189,.T.);
#3695=FACE_OUTER_BOUND('',#6190,.T.);
#3696=FACE_OUTER_BOUND('',#6191,.T.);
#3697=FACE_OUTER_BOUND('',#6192,.T.);
#3698=FACE_OUTER_BOUND('',#6193,.T.);
#3699=FACE_OUTER_BOUND('',#6194,.T.);
#3700=FACE_OUTER_BOUND('',#6195,.T.);
#3701=FACE_OUTER_BOUND('',#6196,.T.);
#3702=FACE_OUTER_BOUND('',#6197,.T.);
#3703=FACE_OUTER_BOUND('',#6198,.T.);
#3704=FACE_OUTER_BOUND('',#6199,.T.);
#3705=FACE_OUTER_BOUND('',#6200,.T.);
#3706=FACE_OUTER_BOUND('',#6201,.T.);
#3707=FACE_OUTER_BOUND('',#6202,.T.);
#3708=FACE_OUTER_BOUND('',#6203,.T.);
#3709=FACE_OUTER_BOUND('',#6204,.T.);
#3710=FACE_OUTER_BOUND('',#6205,.T.);
#3711=FACE_OUTER_BOUND('',#6206,.T.);
#3712=FACE_OUTER_BOUND('',#6207,.T.);
#3713=FACE_OUTER_BOUND('',#6208,.T.);
#3714=FACE_OUTER_BOUND('',#6209,.T.);
#3715=FACE_OUTER_BOUND('',#6210,.T.);
#3716=FACE_OUTER_BOUND('',#6211,.T.);
#3717=FACE_OUTER_BOUND('',#6212,.T.);
#3718=FACE_OUTER_BOUND('',#6213,.T.);
#3719=FACE_OUTER_BOUND('',#6214,.T.);
#3720=FACE_OUTER_BOUND('',#6215,.T.);
#3721=FACE_OUTER_BOUND('',#6216,.T.);
#3722=FACE_OUTER_BOUND('',#6217,.T.);
#3723=FACE_OUTER_BOUND('',#6218,.T.);
#3724=FACE_OUTER_BOUND('',#6219,.T.);
#3725=FACE_OUTER_BOUND('',#6220,.T.);
#3726=FACE_OUTER_BOUND('',#6221,.T.);
#3727=FACE_OUTER_BOUND('',#6222,.T.);
#3728=FACE_OUTER_BOUND('',#6223,.T.);
#3729=FACE_OUTER_BOUND('',#6224,.T.);
#3730=FACE_OUTER_BOUND('',#6225,.T.);
#3731=FACE_OUTER_BOUND('',#6226,.T.);
#3732=FACE_OUTER_BOUND('',#6227,.T.);
#3733=FACE_OUTER_BOUND('',#6228,.T.);
#3734=FACE_OUTER_BOUND('',#6229,.T.);
#3735=FACE_OUTER_BOUND('',#6230,.T.);
#3736=FACE_OUTER_BOUND('',#6231,.T.);
#3737=FACE_OUTER_BOUND('',#6232,.T.);
#3738=FACE_OUTER_BOUND('',#6233,.T.);
#3739=FACE_OUTER_BOUND('',#6234,.T.);
#3740=FACE_OUTER_BOUND('',#6235,.T.);
#3741=FACE_OUTER_BOUND('',#6236,.T.);
#3742=FACE_OUTER_BOUND('',#6237,.T.);
#3743=FACE_OUTER_BOUND('',#6238,.T.);
#3744=FACE_OUTER_BOUND('',#6239,.T.);
#3745=FACE_OUTER_BOUND('',#6240,.T.);
#3746=FACE_OUTER_BOUND('',#6241,.T.);
#3747=FACE_OUTER_BOUND('',#6242,.T.);
#3748=FACE_OUTER_BOUND('',#6243,.T.);
#3749=FACE_OUTER_BOUND('',#6244,.T.);
#3750=FACE_OUTER_BOUND('',#6245,.T.);
#3751=FACE_OUTER_BOUND('',#6246,.T.);
#3752=FACE_OUTER_BOUND('',#6247,.T.);
#3753=FACE_OUTER_BOUND('',#6248,.T.);
#3754=FACE_OUTER_BOUND('',#6249,.T.);
#3755=FACE_OUTER_BOUND('',#6250,.T.);
#3756=FACE_OUTER_BOUND('',#6251,.T.);
#3757=FACE_OUTER_BOUND('',#6252,.T.);
#3758=FACE_OUTER_BOUND('',#6253,.T.);
#3759=FACE_OUTER_BOUND('',#6254,.T.);
#3760=FACE_OUTER_BOUND('',#6255,.T.);
#3761=FACE_OUTER_BOUND('',#6256,.T.);
#3762=FACE_OUTER_BOUND('',#6257,.T.);
#3763=FACE_OUTER_BOUND('',#6258,.T.);
#3764=FACE_OUTER_BOUND('',#6259,.T.);
#3765=FACE_OUTER_BOUND('',#6260,.T.);
#3766=FACE_OUTER_BOUND('',#6261,.T.);
#3767=FACE_OUTER_BOUND('',#6262,.T.);
#3768=FACE_OUTER_BOUND('',#6263,.T.);
#3769=FACE_OUTER_BOUND('',#6264,.T.);
#3770=FACE_OUTER_BOUND('',#6265,.T.);
#3771=FACE_OUTER_BOUND('',#6266,.T.);
#3772=FACE_OUTER_BOUND('',#6267,.T.);
#3773=FACE_OUTER_BOUND('',#6268,.T.);
#3774=FACE_OUTER_BOUND('',#6269,.T.);
#3775=FACE_OUTER_BOUND('',#6270,.T.);
#3776=FACE_OUTER_BOUND('',#6271,.T.);
#3777=FACE_OUTER_BOUND('',#6272,.T.);
#3778=FACE_OUTER_BOUND('',#6273,.T.);
#3779=FACE_OUTER_BOUND('',#6274,.T.);
#3780=FACE_OUTER_BOUND('',#6275,.T.);
#3781=FACE_OUTER_BOUND('',#6276,.T.);
#3782=FACE_OUTER_BOUND('',#6277,.T.);
#3783=FACE_OUTER_BOUND('',#6278,.T.);
#3784=FACE_OUTER_BOUND('',#6279,.T.);
#3785=FACE_OUTER_BOUND('',#6280,.T.);
#3786=FACE_OUTER_BOUND('',#6281,.T.);
#3787=FACE_OUTER_BOUND('',#6282,.T.);
#3788=FACE_OUTER_BOUND('',#6283,.T.);
#3789=FACE_OUTER_BOUND('',#6284,.T.);
#3790=FACE_OUTER_BOUND('',#6285,.T.);
#3791=FACE_OUTER_BOUND('',#6286,.T.);
#3792=FACE_OUTER_BOUND('',#6287,.T.);
#3793=FACE_OUTER_BOUND('',#6288,.T.);
#3794=FACE_OUTER_BOUND('',#6289,.T.);
#3795=FACE_OUTER_BOUND('',#6290,.T.);
#3796=FACE_OUTER_BOUND('',#6291,.T.);
#3797=FACE_OUTER_BOUND('',#6292,.T.);
#3798=FACE_OUTER_BOUND('',#6293,.T.);
#3799=FACE_OUTER_BOUND('',#6294,.T.);
#3800=FACE_OUTER_BOUND('',#6295,.T.);
#3801=FACE_OUTER_BOUND('',#6296,.T.);
#3802=FACE_OUTER_BOUND('',#6297,.T.);
#3803=FACE_OUTER_BOUND('',#6298,.T.);
#3804=FACE_OUTER_BOUND('',#6299,.T.);
#3805=FACE_OUTER_BOUND('',#6300,.T.);
#3806=FACE_OUTER_BOUND('',#6301,.T.);
#3807=FACE_OUTER_BOUND('',#6302,.T.);
#3808=FACE_OUTER_BOUND('',#6303,.T.);
#3809=FACE_OUTER_BOUND('',#6304,.T.);
#3810=FACE_OUTER_BOUND('',#6305,.T.);
#3811=FACE_OUTER_BOUND('',#6306,.T.);
#3812=FACE_OUTER_BOUND('',#6307,.T.);
#3813=FACE_OUTER_BOUND('',#6308,.T.);
#3814=FACE_OUTER_BOUND('',#6309,.T.);
#3815=FACE_OUTER_BOUND('',#6310,.T.);
#3816=FACE_OUTER_BOUND('',#6311,.T.);
#3817=FACE_OUTER_BOUND('',#6312,.T.);
#3818=FACE_OUTER_BOUND('',#6313,.T.);
#3819=FACE_OUTER_BOUND('',#6314,.T.);
#3820=FACE_OUTER_BOUND('',#6315,.T.);
#3821=FACE_OUTER_BOUND('',#6316,.T.);
#3822=FACE_OUTER_BOUND('',#6317,.T.);
#3823=FACE_OUTER_BOUND('',#6318,.T.);
#3824=FACE_OUTER_BOUND('',#6319,.T.);
#3825=FACE_OUTER_BOUND('',#6320,.T.);
#3826=FACE_OUTER_BOUND('',#6321,.T.);
#3827=FACE_OUTER_BOUND('',#6322,.T.);
#3828=FACE_OUTER_BOUND('',#6323,.T.);
#3829=FACE_OUTER_BOUND('',#6324,.T.);
#3830=FACE_OUTER_BOUND('',#6325,.T.);
#3831=FACE_OUTER_BOUND('',#6326,.T.);
#3832=FACE_OUTER_BOUND('',#6327,.T.);
#3833=FACE_OUTER_BOUND('',#6328,.T.);
#3834=FACE_OUTER_BOUND('',#6329,.T.);
#3835=FACE_OUTER_BOUND('',#6330,.T.);
#3836=FACE_OUTER_BOUND('',#6331,.T.);
#3837=FACE_OUTER_BOUND('',#6332,.T.);
#3838=FACE_OUTER_BOUND('',#6333,.T.);
#3839=FACE_OUTER_BOUND('',#6334,.T.);
#3840=FACE_OUTER_BOUND('',#6335,.T.);
#3841=FACE_OUTER_BOUND('',#6336,.T.);
#3842=FACE_OUTER_BOUND('',#6337,.T.);
#3843=FACE_OUTER_BOUND('',#6338,.T.);
#3844=FACE_OUTER_BOUND('',#6339,.T.);
#3845=FACE_OUTER_BOUND('',#6340,.T.);
#3846=FACE_OUTER_BOUND('',#6341,.T.);
#3847=FACE_OUTER_BOUND('',#6342,.T.);
#3848=FACE_OUTER_BOUND('',#6343,.T.);
#3849=FACE_OUTER_BOUND('',#6344,.T.);
#3850=FACE_OUTER_BOUND('',#6345,.T.);
#3851=FACE_OUTER_BOUND('',#6346,.T.);
#3852=FACE_OUTER_BOUND('',#6347,.T.);
#3853=FACE_OUTER_BOUND('',#6348,.T.);
#3854=FACE_OUTER_BOUND('',#6349,.T.);
#3855=FACE_OUTER_BOUND('',#6350,.T.);
#3856=FACE_OUTER_BOUND('',#6351,.T.);
#3857=FACE_OUTER_BOUND('',#6352,.T.);
#3858=FACE_OUTER_BOUND('',#6353,.T.);
#3859=FACE_OUTER_BOUND('',#6354,.T.);
#3860=FACE_OUTER_BOUND('',#6355,.T.);
#3861=FACE_OUTER_BOUND('',#6356,.T.);
#3862=FACE_OUTER_BOUND('',#6357,.T.);
#3863=FACE_OUTER_BOUND('',#6358,.T.);
#3864=FACE_OUTER_BOUND('',#6359,.T.);
#3865=FACE_OUTER_BOUND('',#6360,.T.);
#3866=FACE_OUTER_BOUND('',#6361,.T.);
#3867=FACE_OUTER_BOUND('',#6362,.T.);
#3868=FACE_OUTER_BOUND('',#6363,.T.);
#3869=FACE_OUTER_BOUND('',#6364,.T.);
#3870=FACE_OUTER_BOUND('',#6365,.T.);
#3871=FACE_OUTER_BOUND('',#6366,.T.);
#3872=FACE_OUTER_BOUND('',#6367,.T.);
#3873=FACE_OUTER_BOUND('',#6368,.T.);
#3874=FACE_OUTER_BOUND('',#6369,.T.);
#3875=FACE_OUTER_BOUND('',#6370,.T.);
#3876=FACE_OUTER_BOUND('',#6371,.T.);
#3877=FACE_OUTER_BOUND('',#6372,.T.);
#3878=FACE_OUTER_BOUND('',#6373,.T.);
#3879=FACE_OUTER_BOUND('',#6374,.T.);
#3880=FACE_OUTER_BOUND('',#6375,.T.);
#3881=FACE_OUTER_BOUND('',#6376,.T.);
#3882=FACE_OUTER_BOUND('',#6377,.T.);
#3883=FACE_OUTER_BOUND('',#6378,.T.);
#3884=FACE_OUTER_BOUND('',#6379,.T.);
#3885=FACE_OUTER_BOUND('',#6380,.T.);
#3886=FACE_OUTER_BOUND('',#6381,.T.);
#3887=FACE_OUTER_BOUND('',#6382,.T.);
#3888=FACE_OUTER_BOUND('',#6383,.T.);
#3889=FACE_OUTER_BOUND('',#6384,.T.);
#3890=FACE_OUTER_BOUND('',#6385,.T.);
#3891=FACE_OUTER_BOUND('',#6386,.T.);
#3892=FACE_OUTER_BOUND('',#6387,.T.);
#3893=FACE_OUTER_BOUND('',#6388,.T.);
#3894=FACE_OUTER_BOUND('',#6389,.T.);
#3895=FACE_OUTER_BOUND('',#6390,.T.);
#3896=FACE_OUTER_BOUND('',#6391,.T.);
#3897=FACE_OUTER_BOUND('',#6392,.T.);
#3898=FACE_OUTER_BOUND('',#6393,.T.);
#3899=FACE_OUTER_BOUND('',#6394,.T.);
#3900=FACE_OUTER_BOUND('',#6395,.T.);
#3901=FACE_OUTER_BOUND('',#6396,.T.);
#3902=FACE_OUTER_BOUND('',#6397,.T.);
#3903=FACE_OUTER_BOUND('',#6398,.T.);
#3904=FACE_OUTER_BOUND('',#6399,.T.);
#3905=FACE_OUTER_BOUND('',#6400,.T.);
#3906=FACE_OUTER_BOUND('',#6401,.T.);
#3907=FACE_OUTER_BOUND('',#6402,.T.);
#3908=FACE_OUTER_BOUND('',#6403,.T.);
#3909=FACE_OUTER_BOUND('',#6404,.T.);
#3910=FACE_OUTER_BOUND('',#6405,.T.);
#3911=FACE_OUTER_BOUND('',#6406,.T.);
#3912=FACE_OUTER_BOUND('',#6407,.T.);
#3913=FACE_OUTER_BOUND('',#6408,.T.);
#3914=FACE_OUTER_BOUND('',#6409,.T.);
#3915=FACE_OUTER_BOUND('',#6410,.T.);
#3916=FACE_OUTER_BOUND('',#6411,.T.);
#3917=FACE_OUTER_BOUND('',#6412,.T.);
#3918=FACE_OUTER_BOUND('',#6413,.T.);
#3919=FACE_OUTER_BOUND('',#6414,.T.);
#3920=FACE_OUTER_BOUND('',#6415,.T.);
#3921=FACE_OUTER_BOUND('',#6416,.T.);
#3922=FACE_OUTER_BOUND('',#6417,.T.);
#3923=FACE_OUTER_BOUND('',#6418,.T.);
#3924=FACE_OUTER_BOUND('',#6419,.T.);
#3925=FACE_OUTER_BOUND('',#6420,.T.);
#3926=FACE_OUTER_BOUND('',#6421,.T.);
#3927=FACE_OUTER_BOUND('',#6422,.T.);
#3928=FACE_OUTER_BOUND('',#6423,.T.);
#3929=FACE_OUTER_BOUND('',#6424,.T.);
#3930=FACE_OUTER_BOUND('',#6425,.T.);
#3931=FACE_OUTER_BOUND('',#6426,.T.);
#3932=FACE_OUTER_BOUND('',#6427,.T.);
#3933=FACE_OUTER_BOUND('',#6428,.T.);
#3934=FACE_OUTER_BOUND('',#6429,.T.);
#3935=FACE_OUTER_BOUND('',#6430,.T.);
#3936=FACE_OUTER_BOUND('',#6431,.T.);
#3937=FACE_OUTER_BOUND('',#6432,.T.);
#3938=FACE_OUTER_BOUND('',#6433,.T.);
#3939=FACE_OUTER_BOUND('',#6434,.T.);
#3940=FACE_OUTER_BOUND('',#6435,.T.);
#3941=FACE_OUTER_BOUND('',#6436,.T.);
#3942=FACE_OUTER_BOUND('',#6437,.T.);
#3943=FACE_OUTER_BOUND('',#6438,.T.);
#3944=FACE_OUTER_BOUND('',#6439,.T.);
#3945=FACE_OUTER_BOUND('',#6440,.T.);
#3946=FACE_OUTER_BOUND('',#6441,.T.);
#3947=FACE_OUTER_BOUND('',#6442,.T.);
#3948=FACE_OUTER_BOUND('',#6443,.T.);
#3949=FACE_OUTER_BOUND('',#6444,.T.);
#3950=FACE_OUTER_BOUND('',#6445,.T.);
#3951=FACE_OUTER_BOUND('',#6446,.T.);
#3952=FACE_OUTER_BOUND('',#6447,.T.);
#3953=FACE_OUTER_BOUND('',#6448,.T.);
#3954=FACE_OUTER_BOUND('',#6449,.T.);
#3955=FACE_OUTER_BOUND('',#6450,.T.);
#3956=FACE_OUTER_BOUND('',#6451,.T.);
#3957=FACE_OUTER_BOUND('',#6452,.T.);
#3958=FACE_OUTER_BOUND('',#6453,.T.);
#3959=FACE_OUTER_BOUND('',#6454,.T.);
#3960=FACE_OUTER_BOUND('',#6455,.T.);
#3961=FACE_OUTER_BOUND('',#6456,.T.);
#3962=FACE_OUTER_BOUND('',#6457,.T.);
#3963=FACE_OUTER_BOUND('',#6458,.T.);
#3964=FACE_OUTER_BOUND('',#6459,.T.);
#3965=FACE_OUTER_BOUND('',#6460,.T.);
#3966=FACE_OUTER_BOUND('',#6461,.T.);
#3967=FACE_OUTER_BOUND('',#6462,.T.);
#3968=FACE_OUTER_BOUND('',#6463,.T.);
#3969=FACE_OUTER_BOUND('',#6464,.T.);
#3970=FACE_OUTER_BOUND('',#6465,.T.);
#3971=FACE_OUTER_BOUND('',#6466,.T.);
#3972=FACE_OUTER_BOUND('',#6467,.T.);
#3973=FACE_OUTER_BOUND('',#6468,.T.);
#3974=FACE_OUTER_BOUND('',#6469,.T.);
#3975=FACE_OUTER_BOUND('',#6470,.T.);
#3976=FACE_OUTER_BOUND('',#6471,.T.);
#3977=FACE_OUTER_BOUND('',#6472,.T.);
#3978=FACE_OUTER_BOUND('',#6473,.T.);
#3979=FACE_OUTER_BOUND('',#6474,.T.);
#3980=FACE_OUTER_BOUND('',#6475,.T.);
#3981=FACE_OUTER_BOUND('',#6476,.T.);
#3982=FACE_OUTER_BOUND('',#6477,.T.);
#3983=FACE_OUTER_BOUND('',#6478,.T.);
#3984=FACE_OUTER_BOUND('',#6479,.T.);
#3985=FACE_OUTER_BOUND('',#6480,.T.);
#3986=FACE_OUTER_BOUND('',#6481,.T.);
#3987=FACE_OUTER_BOUND('',#6482,.T.);
#3988=FACE_OUTER_BOUND('',#6483,.T.);
#3989=FACE_OUTER_BOUND('',#6484,.T.);
#3990=FACE_OUTER_BOUND('',#6485,.T.);
#3991=FACE_OUTER_BOUND('',#6486,.T.);
#3992=FACE_OUTER_BOUND('',#6487,.T.);
#3993=FACE_OUTER_BOUND('',#6488,.T.);
#3994=FACE_OUTER_BOUND('',#6489,.T.);
#3995=FACE_OUTER_BOUND('',#6490,.T.);
#3996=FACE_OUTER_BOUND('',#6491,.T.);
#3997=FACE_OUTER_BOUND('',#6492,.T.);
#3998=FACE_OUTER_BOUND('',#6493,.T.);
#3999=FACE_OUTER_BOUND('',#6494,.T.);
#4000=FACE_OUTER_BOUND('',#6495,.T.);
#4001=FACE_OUTER_BOUND('',#6496,.T.);
#4002=FACE_OUTER_BOUND('',#6497,.T.);
#4003=FACE_OUTER_BOUND('',#6498,.T.);
#4004=FACE_OUTER_BOUND('',#6499,.T.);
#4005=FACE_OUTER_BOUND('',#6500,.T.);
#4006=FACE_OUTER_BOUND('',#6501,.T.);
#4007=FACE_OUTER_BOUND('',#6502,.T.);
#4008=FACE_OUTER_BOUND('',#6503,.T.);
#4009=FACE_OUTER_BOUND('',#6504,.T.);
#4010=FACE_OUTER_BOUND('',#6505,.T.);
#4011=FACE_OUTER_BOUND('',#6506,.T.);
#4012=FACE_OUTER_BOUND('',#6507,.T.);
#4013=FACE_OUTER_BOUND('',#6508,.T.);
#4014=FACE_OUTER_BOUND('',#6509,.T.);
#4015=FACE_OUTER_BOUND('',#6510,.T.);
#4016=FACE_OUTER_BOUND('',#6511,.T.);
#4017=FACE_OUTER_BOUND('',#6512,.T.);
#4018=FACE_OUTER_BOUND('',#6513,.T.);
#4019=FACE_OUTER_BOUND('',#6514,.T.);
#4020=FACE_OUTER_BOUND('',#6515,.T.);
#4021=FACE_OUTER_BOUND('',#6516,.T.);
#4022=FACE_OUTER_BOUND('',#6517,.T.);
#4023=FACE_OUTER_BOUND('',#6518,.T.);
#4024=FACE_OUTER_BOUND('',#6519,.T.);
#4025=FACE_OUTER_BOUND('',#6520,.T.);
#4026=FACE_OUTER_BOUND('',#6521,.T.);
#4027=FACE_OUTER_BOUND('',#6522,.T.);
#4028=FACE_OUTER_BOUND('',#6523,.T.);
#4029=FACE_OUTER_BOUND('',#6524,.T.);
#4030=FACE_OUTER_BOUND('',#6525,.T.);
#4031=FACE_OUTER_BOUND('',#6526,.T.);
#4032=FACE_OUTER_BOUND('',#6527,.T.);
#4033=FACE_OUTER_BOUND('',#6528,.T.);
#4034=FACE_OUTER_BOUND('',#6529,.T.);
#4035=FACE_OUTER_BOUND('',#6530,.T.);
#4036=FACE_OUTER_BOUND('',#6531,.T.);
#4037=FACE_OUTER_BOUND('',#6532,.T.);
#4038=FACE_OUTER_BOUND('',#6533,.T.);
#4039=FACE_OUTER_BOUND('',#6534,.T.);
#4040=FACE_OUTER_BOUND('',#6535,.T.);
#4041=FACE_OUTER_BOUND('',#6536,.T.);
#4042=FACE_OUTER_BOUND('',#6537,.T.);
#4043=FACE_OUTER_BOUND('',#6538,.T.);
#4044=FACE_OUTER_BOUND('',#6539,.T.);
#4045=FACE_OUTER_BOUND('',#6540,.T.);
#4046=FACE_OUTER_BOUND('',#6541,.T.);
#4047=FACE_OUTER_BOUND('',#6542,.T.);
#4048=FACE_OUTER_BOUND('',#6543,.T.);
#4049=FACE_OUTER_BOUND('',#6544,.T.);
#4050=FACE_OUTER_BOUND('',#6545,.T.);
#4051=FACE_OUTER_BOUND('',#6546,.T.);
#4052=FACE_OUTER_BOUND('',#6547,.T.);
#4053=FACE_OUTER_BOUND('',#6548,.T.);
#4054=FACE_OUTER_BOUND('',#6549,.T.);
#4055=FACE_OUTER_BOUND('',#6550,.T.);
#4056=FACE_OUTER_BOUND('',#6551,.T.);
#4057=FACE_OUTER_BOUND('',#6552,.T.);
#4058=FACE_OUTER_BOUND('',#6553,.T.);
#4059=FACE_OUTER_BOUND('',#6554,.T.);
#4060=FACE_OUTER_BOUND('',#6555,.T.);
#4061=FACE_OUTER_BOUND('',#6556,.T.);
#4062=FACE_OUTER_BOUND('',#6557,.T.);
#4063=FACE_OUTER_BOUND('',#6558,.T.);
#4064=FACE_OUTER_BOUND('',#6559,.T.);
#4065=FACE_OUTER_BOUND('',#6560,.T.);
#4066=FACE_OUTER_BOUND('',#6561,.T.);
#4067=FACE_OUTER_BOUND('',#6562,.T.);
#4068=FACE_OUTER_BOUND('',#6563,.T.);
#4069=FACE_OUTER_BOUND('',#6564,.T.);
#4070=FACE_OUTER_BOUND('',#6565,.T.);
#4071=FACE_OUTER_BOUND('',#6566,.T.);
#4072=FACE_OUTER_BOUND('',#6567,.T.);
#4073=FACE_OUTER_BOUND('',#6568,.T.);
#4074=FACE_OUTER_BOUND('',#6569,.T.);
#4075=FACE_OUTER_BOUND('',#6570,.T.);
#4076=FACE_OUTER_BOUND('',#6571,.T.);
#4077=FACE_OUTER_BOUND('',#6572,.T.);
#4078=FACE_OUTER_BOUND('',#6573,.T.);
#4079=FACE_OUTER_BOUND('',#6574,.T.);
#4080=FACE_OUTER_BOUND('',#6575,.T.);
#4081=FACE_OUTER_BOUND('',#6576,.T.);
#4082=FACE_OUTER_BOUND('',#6577,.T.);
#4083=FACE_OUTER_BOUND('',#6578,.T.);
#4084=FACE_OUTER_BOUND('',#6579,.T.);
#4085=FACE_OUTER_BOUND('',#6580,.T.);
#4086=FACE_OUTER_BOUND('',#6581,.T.);
#4087=FACE_OUTER_BOUND('',#6582,.T.);
#4088=FACE_OUTER_BOUND('',#6583,.T.);
#4089=FACE_OUTER_BOUND('',#6584,.T.);
#4090=FACE_OUTER_BOUND('',#6585,.T.);
#4091=FACE_OUTER_BOUND('',#6586,.T.);
#4092=FACE_OUTER_BOUND('',#6587,.T.);
#4093=FACE_OUTER_BOUND('',#6588,.T.);
#4094=FACE_OUTER_BOUND('',#6589,.T.);
#4095=FACE_OUTER_BOUND('',#6590,.T.);
#4096=FACE_OUTER_BOUND('',#6591,.T.);
#4097=FACE_OUTER_BOUND('',#6592,.T.);
#4098=FACE_OUTER_BOUND('',#6593,.T.);
#4099=FACE_OUTER_BOUND('',#6594,.T.);
#4100=FACE_OUTER_BOUND('',#6595,.T.);
#4101=FACE_OUTER_BOUND('',#6596,.T.);
#4102=FACE_OUTER_BOUND('',#6597,.T.);
#4103=FACE_OUTER_BOUND('',#6598,.T.);
#4104=FACE_OUTER_BOUND('',#6599,.T.);
#4105=FACE_OUTER_BOUND('',#6600,.T.);
#4106=FACE_OUTER_BOUND('',#6601,.T.);
#4107=FACE_OUTER_BOUND('',#6602,.T.);
#4108=FACE_OUTER_BOUND('',#6603,.T.);
#4109=FACE_OUTER_BOUND('',#6604,.T.);
#4110=FACE_OUTER_BOUND('',#6605,.T.);
#4111=FACE_OUTER_BOUND('',#6606,.T.);
#4112=FACE_OUTER_BOUND('',#6607,.T.);
#4113=FACE_OUTER_BOUND('',#6608,.T.);
#4114=FACE_OUTER_BOUND('',#6609,.T.);
#4115=FACE_OUTER_BOUND('',#6610,.T.);
#4116=FACE_OUTER_BOUND('',#6611,.T.);
#4117=FACE_OUTER_BOUND('',#6612,.T.);
#4118=FACE_OUTER_BOUND('',#6613,.T.);
#4119=FACE_OUTER_BOUND('',#6614,.T.);
#4120=FACE_OUTER_BOUND('',#6615,.T.);
#4121=FACE_OUTER_BOUND('',#6616,.T.);
#4122=FACE_OUTER_BOUND('',#6617,.T.);
#4123=FACE_OUTER_BOUND('',#6618,.T.);
#4124=FACE_OUTER_BOUND('',#6619,.T.);
#4125=FACE_OUTER_BOUND('',#6620,.T.);
#4126=FACE_OUTER_BOUND('',#6621,.T.);
#4127=FACE_OUTER_BOUND('',#6622,.T.);
#4128=FACE_OUTER_BOUND('',#6623,.T.);
#4129=FACE_OUTER_BOUND('',#6624,.T.);
#4130=FACE_OUTER_BOUND('',#6625,.T.);
#4131=FACE_OUTER_BOUND('',#6626,.T.);
#4132=FACE_OUTER_BOUND('',#6627,.T.);
#4133=FACE_OUTER_BOUND('',#6628,.T.);
#4134=FACE_OUTER_BOUND('',#6629,.T.);
#4135=FACE_OUTER_BOUND('',#6630,.T.);
#4136=FACE_OUTER_BOUND('',#6631,.T.);
#4137=FACE_OUTER_BOUND('',#6632,.T.);
#4138=FACE_OUTER_BOUND('',#6633,.T.);
#4139=FACE_OUTER_BOUND('',#6634,.T.);
#4140=FACE_OUTER_BOUND('',#6635,.T.);
#4141=FACE_OUTER_BOUND('',#6636,.T.);
#4142=FACE_OUTER_BOUND('',#6637,.T.);
#4143=FACE_OUTER_BOUND('',#6638,.T.);
#4144=FACE_OUTER_BOUND('',#6639,.T.);
#4145=FACE_OUTER_BOUND('',#6640,.T.);
#4146=FACE_OUTER_BOUND('',#6641,.T.);
#4147=FACE_OUTER_BOUND('',#6642,.T.);
#4148=FACE_OUTER_BOUND('',#6643,.T.);
#4149=FACE_OUTER_BOUND('',#6644,.T.);
#4150=FACE_OUTER_BOUND('',#6645,.T.);
#4151=FACE_OUTER_BOUND('',#6646,.T.);
#4152=FACE_OUTER_BOUND('',#6647,.T.);
#4153=FACE_OUTER_BOUND('',#6648,.T.);
#4154=FACE_OUTER_BOUND('',#6649,.T.);
#4155=FACE_OUTER_BOUND('',#6650,.T.);
#4156=FACE_OUTER_BOUND('',#6651,.T.);
#4157=FACE_OUTER_BOUND('',#6652,.T.);
#4158=FACE_OUTER_BOUND('',#6653,.T.);
#4159=FACE_OUTER_BOUND('',#6654,.T.);
#4160=FACE_OUTER_BOUND('',#6655,.T.);
#4161=FACE_OUTER_BOUND('',#6656,.T.);
#4162=FACE_OUTER_BOUND('',#6657,.T.);
#4163=FACE_OUTER_BOUND('',#6658,.T.);
#4164=FACE_OUTER_BOUND('',#6659,.T.);
#4165=FACE_OUTER_BOUND('',#6660,.T.);
#4166=FACE_OUTER_BOUND('',#6661,.T.);
#4167=FACE_OUTER_BOUND('',#6662,.T.);
#4168=FACE_OUTER_BOUND('',#6663,.T.);
#4169=FACE_OUTER_BOUND('',#6664,.T.);
#4170=FACE_OUTER_BOUND('',#6665,.T.);
#4171=FACE_OUTER_BOUND('',#6666,.T.);
#4172=FACE_OUTER_BOUND('',#6667,.T.);
#4173=FACE_OUTER_BOUND('',#6668,.T.);
#4174=FACE_OUTER_BOUND('',#6669,.T.);
#4175=FACE_OUTER_BOUND('',#6670,.T.);
#4176=FACE_OUTER_BOUND('',#6671,.T.);
#4177=FACE_OUTER_BOUND('',#6672,.T.);
#4178=FACE_OUTER_BOUND('',#6673,.T.);
#4179=FACE_OUTER_BOUND('',#6674,.T.);
#4180=FACE_OUTER_BOUND('',#6675,.T.);
#4181=FACE_OUTER_BOUND('',#6676,.T.);
#4182=FACE_OUTER_BOUND('',#6677,.T.);
#4183=FACE_OUTER_BOUND('',#6678,.T.);
#4184=FACE_OUTER_BOUND('',#6679,.T.);
#4185=FACE_OUTER_BOUND('',#6680,.T.);
#4186=FACE_OUTER_BOUND('',#6681,.T.);
#4187=FACE_OUTER_BOUND('',#6682,.T.);
#4188=FACE_OUTER_BOUND('',#6683,.T.);
#4189=FACE_OUTER_BOUND('',#6684,.T.);
#4190=FACE_OUTER_BOUND('',#6685,.T.);
#4191=FACE_OUTER_BOUND('',#6686,.T.);
#4192=FACE_OUTER_BOUND('',#6687,.T.);
#4193=FACE_OUTER_BOUND('',#6688,.T.);
#4194=FACE_OUTER_BOUND('',#6689,.T.);
#4195=FACE_OUTER_BOUND('',#6690,.T.);
#4196=FACE_OUTER_BOUND('',#6691,.T.);
#4197=FACE_OUTER_BOUND('',#6692,.T.);
#4198=FACE_OUTER_BOUND('',#6693,.T.);
#4199=FACE_OUTER_BOUND('',#6694,.T.);
#4200=FACE_OUTER_BOUND('',#6695,.T.);
#4201=FACE_OUTER_BOUND('',#6696,.T.);
#4202=FACE_OUTER_BOUND('',#6697,.T.);
#4203=FACE_OUTER_BOUND('',#6698,.T.);
#4204=FACE_OUTER_BOUND('',#6699,.T.);
#4205=FACE_OUTER_BOUND('',#6700,.T.);
#4206=FACE_OUTER_BOUND('',#6701,.T.);
#4207=FACE_OUTER_BOUND('',#6702,.T.);
#4208=FACE_OUTER_BOUND('',#6703,.T.);
#4209=FACE_OUTER_BOUND('',#6704,.T.);
#4210=FACE_OUTER_BOUND('',#6705,.T.);
#4211=FACE_OUTER_BOUND('',#6706,.T.);
#4212=FACE_OUTER_BOUND('',#6707,.T.);
#4213=FACE_OUTER_BOUND('',#6708,.T.);
#4214=FACE_OUTER_BOUND('',#6709,.T.);
#4215=FACE_OUTER_BOUND('',#6710,.T.);
#4216=FACE_OUTER_BOUND('',#6711,.T.);
#4217=FACE_OUTER_BOUND('',#6712,.T.);
#4218=FACE_OUTER_BOUND('',#6713,.T.);
#4219=FACE_OUTER_BOUND('',#6714,.T.);
#4220=FACE_OUTER_BOUND('',#6715,.T.);
#4221=FACE_OUTER_BOUND('',#6716,.T.);
#4222=FACE_OUTER_BOUND('',#6717,.T.);
#4223=FACE_OUTER_BOUND('',#6718,.T.);
#4224=FACE_OUTER_BOUND('',#6719,.T.);
#4225=FACE_OUTER_BOUND('',#6720,.T.);
#4226=FACE_OUTER_BOUND('',#6721,.T.);
#4227=FACE_OUTER_BOUND('',#6722,.T.);
#4228=FACE_OUTER_BOUND('',#6723,.T.);
#4229=FACE_OUTER_BOUND('',#6724,.T.);
#4230=FACE_OUTER_BOUND('',#6725,.T.);
#4231=FACE_OUTER_BOUND('',#6726,.T.);
#4232=FACE_OUTER_BOUND('',#6727,.T.);
#4233=FACE_OUTER_BOUND('',#6728,.T.);
#4234=FACE_OUTER_BOUND('',#6729,.T.);
#4235=FACE_OUTER_BOUND('',#6730,.T.);
#4236=FACE_OUTER_BOUND('',#6731,.T.);
#4237=FACE_OUTER_BOUND('',#6732,.T.);
#4238=FACE_OUTER_BOUND('',#6733,.T.);
#4239=FACE_OUTER_BOUND('',#6734,.T.);
#4240=FACE_OUTER_BOUND('',#6735,.T.);
#4241=FACE_OUTER_BOUND('',#6736,.T.);
#4242=FACE_OUTER_BOUND('',#6737,.T.);
#4243=FACE_OUTER_BOUND('',#6738,.T.);
#4244=FACE_OUTER_BOUND('',#6739,.T.);
#5198=EDGE_LOOP('',(#30779,#30780,#30781,#30782));
#5199=EDGE_LOOP('',(#30783,#30784,#30785,#30786));
#5200=EDGE_LOOP('',(#30787,#30788,#30789,#30790));
#5201=EDGE_LOOP('',(#30791,#30792,#30793,#30794));
#5202=EDGE_LOOP('',(#30795,#30796,#30797,#30798,#30799,#30800,#30801,#30802,
#30803,#30804,#30805,#30806));
#5203=EDGE_LOOP('',(#30807));
#5204=EDGE_LOOP('',(#30808,#30809,#30810,#30811,#30812,#30813,#30814,#30815,
#30816,#30817,#30818,#30819));
#5205=EDGE_LOOP('',(#30820));
#5206=EDGE_LOOP('',(#30821,#30822,#30823,#30824));
#5207=EDGE_LOOP('',(#30825,#30826,#30827,#30828));
#5208=EDGE_LOOP('',(#30829,#30830,#30831,#30832));
#5209=EDGE_LOOP('',(#30833,#30834,#30835,#30836));
#5210=EDGE_LOOP('',(#30837,#30838,#30839,#30840));
#5211=EDGE_LOOP('',(#30841,#30842,#30843,#30844));
#5212=EDGE_LOOP('',(#30845,#30846,#30847,#30848));
#5213=EDGE_LOOP('',(#30849,#30850,#30851,#30852));
#5214=EDGE_LOOP('',(#30853,#30854,#30855,#30856));
#5215=EDGE_LOOP('',(#30857,#30858,#30859,#30860));
#5216=EDGE_LOOP('',(#30861,#30862,#30863,#30864));
#5217=EDGE_LOOP('',(#30865,#30866,#30867,#30868));
#5218=EDGE_LOOP('',(#30869,#30870,#30871,#30872));
#5219=EDGE_LOOP('',(#30873,#30874,#30875,#30876));
#5220=EDGE_LOOP('',(#30877,#30878,#30879,#30880));
#5221=EDGE_LOOP('',(#30881,#30882,#30883,#30884));
#5222=EDGE_LOOP('',(#30885,#30886,#30887,#30888));
#5223=EDGE_LOOP('',(#30889,#30890,#30891,#30892));
#5224=EDGE_LOOP('',(#30893,#30894,#30895,#30896));
#5225=EDGE_LOOP('',(#30897,#30898,#30899,#30900));
#5226=EDGE_LOOP('',(#30901,#30902,#30903,#30904,#30905,#30906,#30907,#30908,
#30909,#30910));
#5227=EDGE_LOOP('',(#30911,#30912,#30913,#30914));
#5228=EDGE_LOOP('',(#30915,#30916,#30917,#30918,#30919,#30920,#30921,#30922,
#30923,#30924));
#5229=EDGE_LOOP('',(#30925,#30926,#30927,#30928));
#5230=EDGE_LOOP('',(#30929,#30930,#30931,#30932));
#5231=EDGE_LOOP('',(#30933,#30934,#30935,#30936));
#5232=EDGE_LOOP('',(#30937,#30938,#30939,#30940));
#5233=EDGE_LOOP('',(#30941,#30942,#30943,#30944));
#5234=EDGE_LOOP('',(#30945,#30946,#30947,#30948));
#5235=EDGE_LOOP('',(#30949,#30950,#30951,#30952));
#5236=EDGE_LOOP('',(#30953,#30954,#30955,#30956));
#5237=EDGE_LOOP('',(#30957,#30958,#30959,#30960));
#5238=EDGE_LOOP('',(#30961,#30962,#30963,#30964));
#5239=EDGE_LOOP('',(#30965,#30966,#30967,#30968));
#5240=EDGE_LOOP('',(#30969,#30970,#30971,#30972));
#5241=EDGE_LOOP('',(#30973,#30974,#30975,#30976));
#5242=EDGE_LOOP('',(#30977,#30978,#30979,#30980));
#5243=EDGE_LOOP('',(#30981,#30982,#30983,#30984));
#5244=EDGE_LOOP('',(#30985,#30986,#30987,#30988,#30989,#30990,#30991,#30992,
#30993,#30994));
#5245=EDGE_LOOP('',(#30995,#30996,#30997,#30998));
#5246=EDGE_LOOP('',(#30999,#31000,#31001,#31002,#31003,#31004,#31005,#31006,
#31007,#31008));
#5247=EDGE_LOOP('',(#31009,#31010,#31011,#31012));
#5248=EDGE_LOOP('',(#31013,#31014,#31015,#31016));
#5249=EDGE_LOOP('',(#31017,#31018,#31019,#31020));
#5250=EDGE_LOOP('',(#31021));
#5251=EDGE_LOOP('',(#31022,#31023,#31024,#31025,#31026,#31027));
#5252=EDGE_LOOP('',(#31028,#31029,#31030,#31031,#31032,#31033));
#5253=EDGE_LOOP('',(#31034,#31035,#31036,#31037,#31038,#31039));
#5254=EDGE_LOOP('',(#31040,#31041,#31042,#31043,#31044,#31045));
#5255=EDGE_LOOP('',(#31046,#31047,#31048,#31049,#31050,#31051));
#5256=EDGE_LOOP('',(#31052,#31053,#31054,#31055,#31056,#31057));
#5257=EDGE_LOOP('',(#31058,#31059,#31060,#31061,#31062,#31063));
#5258=EDGE_LOOP('',(#31064,#31065,#31066,#31067,#31068,#31069));
#5259=EDGE_LOOP('',(#31070,#31071,#31072,#31073,#31074,#31075));
#5260=EDGE_LOOP('',(#31076,#31077,#31078,#31079,#31080,#31081));
#5261=EDGE_LOOP('',(#31082,#31083,#31084,#31085,#31086,#31087));
#5262=EDGE_LOOP('',(#31088,#31089,#31090,#31091,#31092,#31093));
#5263=EDGE_LOOP('',(#31094,#31095,#31096,#31097,#31098,#31099));
#5264=EDGE_LOOP('',(#31100,#31101,#31102,#31103,#31104,#31105));
#5265=EDGE_LOOP('',(#31106,#31107,#31108,#31109,#31110,#31111));
#5266=EDGE_LOOP('',(#31112,#31113,#31114,#31115,#31116,#31117));
#5267=EDGE_LOOP('',(#31118,#31119,#31120,#31121,#31122,#31123));
#5268=EDGE_LOOP('',(#31124,#31125,#31126,#31127,#31128,#31129));
#5269=EDGE_LOOP('',(#31130,#31131,#31132,#31133,#31134,#31135));
#5270=EDGE_LOOP('',(#31136,#31137,#31138,#31139,#31140,#31141));
#5271=EDGE_LOOP('',(#31142,#31143,#31144,#31145,#31146,#31147));
#5272=EDGE_LOOP('',(#31148,#31149,#31150,#31151,#31152,#31153));
#5273=EDGE_LOOP('',(#31154,#31155,#31156,#31157,#31158,#31159));
#5274=EDGE_LOOP('',(#31160,#31161,#31162,#31163,#31164,#31165));
#5275=EDGE_LOOP('',(#31166,#31167,#31168,#31169,#31170,#31171));
#5276=EDGE_LOOP('',(#31172,#31173,#31174,#31175,#31176,#31177));
#5277=EDGE_LOOP('',(#31178,#31179,#31180,#31181,#31182,#31183));
#5278=EDGE_LOOP('',(#31184,#31185,#31186,#31187,#31188,#31189));
#5279=EDGE_LOOP('',(#31190,#31191,#31192,#31193,#31194,#31195));
#5280=EDGE_LOOP('',(#31196,#31197,#31198,#31199,#31200,#31201));
#5281=EDGE_LOOP('',(#31202,#31203,#31204,#31205,#31206,#31207));
#5282=EDGE_LOOP('',(#31208,#31209,#31210,#31211,#31212,#31213));
#5283=EDGE_LOOP('',(#31214,#31215,#31216,#31217,#31218,#31219));
#5284=EDGE_LOOP('',(#31220,#31221,#31222,#31223,#31224,#31225));
#5285=EDGE_LOOP('',(#31226,#31227,#31228,#31229,#31230,#31231));
#5286=EDGE_LOOP('',(#31232,#31233,#31234,#31235,#31236,#31237));
#5287=EDGE_LOOP('',(#31238,#31239,#31240,#31241,#31242,#31243));
#5288=EDGE_LOOP('',(#31244,#31245,#31246,#31247,#31248,#31249));
#5289=EDGE_LOOP('',(#31250,#31251,#31252,#31253,#31254,#31255));
#5290=EDGE_LOOP('',(#31256,#31257,#31258,#31259,#31260,#31261));
#5291=EDGE_LOOP('',(#31262,#31263,#31264,#31265,#31266,#31267));
#5292=EDGE_LOOP('',(#31268,#31269,#31270,#31271,#31272,#31273));
#5293=EDGE_LOOP('',(#31274,#31275,#31276,#31277,#31278,#31279));
#5294=EDGE_LOOP('',(#31280,#31281,#31282,#31283,#31284,#31285));
#5295=EDGE_LOOP('',(#31286,#31287,#31288,#31289,#31290,#31291));
#5296=EDGE_LOOP('',(#31292,#31293,#31294,#31295,#31296,#31297));
#5297=EDGE_LOOP('',(#31298,#31299,#31300,#31301,#31302,#31303));
#5298=EDGE_LOOP('',(#31304,#31305,#31306,#31307,#31308,#31309));
#5299=EDGE_LOOP('',(#31310,#31311,#31312,#31313,#31314,#31315));
#5300=EDGE_LOOP('',(#31316,#31317,#31318,#31319,#31320,#31321));
#5301=EDGE_LOOP('',(#31322,#31323,#31324,#31325,#31326,#31327));
#5302=EDGE_LOOP('',(#31328,#31329,#31330,#31331,#31332,#31333));
#5303=EDGE_LOOP('',(#31334,#31335,#31336,#31337,#31338,#31339));
#5304=EDGE_LOOP('',(#31340,#31341,#31342,#31343,#31344,#31345));
#5305=EDGE_LOOP('',(#31346,#31347,#31348,#31349,#31350,#31351));
#5306=EDGE_LOOP('',(#31352,#31353,#31354,#31355,#31356,#31357));
#5307=EDGE_LOOP('',(#31358,#31359,#31360,#31361,#31362,#31363));
#5308=EDGE_LOOP('',(#31364,#31365,#31366,#31367,#31368,#31369));
#5309=EDGE_LOOP('',(#31370,#31371,#31372,#31373,#31374,#31375));
#5310=EDGE_LOOP('',(#31376,#31377,#31378,#31379,#31380,#31381));
#5311=EDGE_LOOP('',(#31382,#31383,#31384,#31385,#31386,#31387));
#5312=EDGE_LOOP('',(#31388,#31389,#31390,#31391,#31392,#31393));
#5313=EDGE_LOOP('',(#31394,#31395,#31396,#31397,#31398,#31399));
#5314=EDGE_LOOP('',(#31400,#31401,#31402,#31403,#31404,#31405));
#5315=EDGE_LOOP('',(#31406,#31407,#31408,#31409,#31410,#31411));
#5316=EDGE_LOOP('',(#31412,#31413,#31414,#31415,#31416,#31417));
#5317=EDGE_LOOP('',(#31418,#31419,#31420,#31421,#31422,#31423));
#5318=EDGE_LOOP('',(#31424,#31425,#31426,#31427,#31428,#31429));
#5319=EDGE_LOOP('',(#31430,#31431,#31432,#31433,#31434,#31435));
#5320=EDGE_LOOP('',(#31436,#31437,#31438,#31439,#31440,#31441));
#5321=EDGE_LOOP('',(#31442,#31443,#31444,#31445,#31446,#31447));
#5322=EDGE_LOOP('',(#31448,#31449,#31450,#31451,#31452,#31453));
#5323=EDGE_LOOP('',(#31454,#31455,#31456,#31457,#31458,#31459));
#5324=EDGE_LOOP('',(#31460,#31461,#31462,#31463,#31464,#31465));
#5325=EDGE_LOOP('',(#31466,#31467,#31468,#31469,#31470,#31471));
#5326=EDGE_LOOP('',(#31472,#31473,#31474,#31475,#31476,#31477));
#5327=EDGE_LOOP('',(#31478,#31479,#31480,#31481,#31482,#31483));
#5328=EDGE_LOOP('',(#31484,#31485,#31486,#31487,#31488,#31489));
#5329=EDGE_LOOP('',(#31490,#31491,#31492,#31493,#31494,#31495));
#5330=EDGE_LOOP('',(#31496,#31497,#31498,#31499,#31500,#31501));
#5331=EDGE_LOOP('',(#31502,#31503,#31504,#31505,#31506,#31507));
#5332=EDGE_LOOP('',(#31508,#31509,#31510,#31511,#31512,#31513));
#5333=EDGE_LOOP('',(#31514,#31515,#31516,#31517,#31518,#31519));
#5334=EDGE_LOOP('',(#31520,#31521,#31522,#31523,#31524,#31525));
#5335=EDGE_LOOP('',(#31526,#31527,#31528,#31529,#31530,#31531));
#5336=EDGE_LOOP('',(#31532,#31533,#31534,#31535,#31536,#31537));
#5337=EDGE_LOOP('',(#31538,#31539,#31540,#31541,#31542,#31543));
#5338=EDGE_LOOP('',(#31544,#31545,#31546,#31547,#31548,#31549));
#5339=EDGE_LOOP('',(#31550,#31551,#31552,#31553,#31554,#31555));
#5340=EDGE_LOOP('',(#31556,#31557,#31558,#31559,#31560,#31561));
#5341=EDGE_LOOP('',(#31562,#31563,#31564,#31565,#31566,#31567));
#5342=EDGE_LOOP('',(#31568,#31569,#31570,#31571,#31572,#31573));
#5343=EDGE_LOOP('',(#31574,#31575,#31576,#31577,#31578,#31579));
#5344=EDGE_LOOP('',(#31580,#31581,#31582,#31583,#31584,#31585));
#5345=EDGE_LOOP('',(#31586,#31587,#31588,#31589,#31590,#31591));
#5346=EDGE_LOOP('',(#31592,#31593,#31594,#31595,#31596,#31597));
#5347=EDGE_LOOP('',(#31598,#31599,#31600,#31601,#31602,#31603));
#5348=EDGE_LOOP('',(#31604,#31605,#31606,#31607,#31608,#31609));
#5349=EDGE_LOOP('',(#31610,#31611,#31612,#31613,#31614,#31615));
#5350=EDGE_LOOP('',(#31616,#31617,#31618,#31619,#31620,#31621));
#5351=EDGE_LOOP('',(#31622,#31623,#31624,#31625,#31626,#31627));
#5352=EDGE_LOOP('',(#31628,#31629,#31630,#31631,#31632,#31633));
#5353=EDGE_LOOP('',(#31634,#31635,#31636,#31637,#31638,#31639));
#5354=EDGE_LOOP('',(#31640,#31641,#31642,#31643,#31644,#31645));
#5355=EDGE_LOOP('',(#31646,#31647,#31648,#31649,#31650,#31651));
#5356=EDGE_LOOP('',(#31652,#31653,#31654,#31655,#31656,#31657));
#5357=EDGE_LOOP('',(#31658,#31659,#31660,#31661,#31662,#31663));
#5358=EDGE_LOOP('',(#31664,#31665,#31666,#31667,#31668,#31669));
#5359=EDGE_LOOP('',(#31670,#31671,#31672,#31673,#31674,#31675));
#5360=EDGE_LOOP('',(#31676,#31677,#31678,#31679,#31680,#31681));
#5361=EDGE_LOOP('',(#31682,#31683,#31684,#31685,#31686,#31687));
#5362=EDGE_LOOP('',(#31688,#31689,#31690,#31691,#31692,#31693));
#5363=EDGE_LOOP('',(#31694,#31695,#31696,#31697,#31698,#31699));
#5364=EDGE_LOOP('',(#31700,#31701,#31702,#31703,#31704,#31705));
#5365=EDGE_LOOP('',(#31706,#31707,#31708,#31709,#31710,#31711));
#5366=EDGE_LOOP('',(#31712,#31713,#31714,#31715,#31716,#31717));
#5367=EDGE_LOOP('',(#31718,#31719,#31720,#31721,#31722,#31723));
#5368=EDGE_LOOP('',(#31724,#31725,#31726,#31727,#31728,#31729));
#5369=EDGE_LOOP('',(#31730,#31731,#31732,#31733,#31734,#31735));
#5370=EDGE_LOOP('',(#31736,#31737,#31738,#31739,#31740,#31741));
#5371=EDGE_LOOP('',(#31742,#31743,#31744,#31745,#31746,#31747));
#5372=EDGE_LOOP('',(#31748,#31749,#31750,#31751,#31752,#31753));
#5373=EDGE_LOOP('',(#31754,#31755,#31756,#31757,#31758,#31759));
#5374=EDGE_LOOP('',(#31760,#31761,#31762,#31763,#31764,#31765));
#5375=EDGE_LOOP('',(#31766,#31767,#31768,#31769,#31770,#31771));
#5376=EDGE_LOOP('',(#31772,#31773,#31774,#31775,#31776,#31777));
#5377=EDGE_LOOP('',(#31778,#31779,#31780,#31781,#31782,#31783));
#5378=EDGE_LOOP('',(#31784,#31785,#31786,#31787,#31788,#31789));
#5379=EDGE_LOOP('',(#31790,#31791,#31792,#31793,#31794,#31795));
#5380=EDGE_LOOP('',(#31796,#31797,#31798,#31799,#31800,#31801));
#5381=EDGE_LOOP('',(#31802,#31803,#31804,#31805,#31806,#31807));
#5382=EDGE_LOOP('',(#31808,#31809,#31810,#31811,#31812,#31813));
#5383=EDGE_LOOP('',(#31814,#31815,#31816,#31817,#31818,#31819));
#5384=EDGE_LOOP('',(#31820,#31821,#31822,#31823,#31824,#31825));
#5385=EDGE_LOOP('',(#31826,#31827,#31828,#31829,#31830,#31831));
#5386=EDGE_LOOP('',(#31832,#31833,#31834,#31835,#31836,#31837));
#5387=EDGE_LOOP('',(#31838,#31839,#31840,#31841,#31842,#31843));
#5388=EDGE_LOOP('',(#31844,#31845,#31846,#31847,#31848,#31849));
#5389=EDGE_LOOP('',(#31850,#31851,#31852,#31853,#31854,#31855));
#5390=EDGE_LOOP('',(#31856,#31857,#31858,#31859,#31860,#31861));
#5391=EDGE_LOOP('',(#31862,#31863,#31864,#31865,#31866,#31867));
#5392=EDGE_LOOP('',(#31868,#31869,#31870,#31871,#31872,#31873));
#5393=EDGE_LOOP('',(#31874,#31875,#31876,#31877,#31878,#31879));
#5394=EDGE_LOOP('',(#31880,#31881,#31882,#31883,#31884,#31885));
#5395=EDGE_LOOP('',(#31886,#31887,#31888,#31889,#31890,#31891));
#5396=EDGE_LOOP('',(#31892,#31893,#31894,#31895,#31896,#31897));
#5397=EDGE_LOOP('',(#31898,#31899,#31900,#31901,#31902,#31903));
#5398=EDGE_LOOP('',(#31904,#31905,#31906,#31907,#31908,#31909));
#5399=EDGE_LOOP('',(#31910,#31911,#31912,#31913,#31914,#31915));
#5400=EDGE_LOOP('',(#31916,#31917,#31918,#31919,#31920,#31921));
#5401=EDGE_LOOP('',(#31922,#31923,#31924,#31925,#31926,#31927));
#5402=EDGE_LOOP('',(#31928,#31929,#31930,#31931,#31932,#31933));
#5403=EDGE_LOOP('',(#31934,#31935,#31936,#31937,#31938,#31939));
#5404=EDGE_LOOP('',(#31940,#31941,#31942,#31943,#31944,#31945));
#5405=EDGE_LOOP('',(#31946,#31947,#31948,#31949,#31950,#31951));
#5406=EDGE_LOOP('',(#31952,#31953,#31954,#31955,#31956,#31957));
#5407=EDGE_LOOP('',(#31958,#31959,#31960,#31961,#31962,#31963));
#5408=EDGE_LOOP('',(#31964,#31965,#31966,#31967,#31968,#31969));
#5409=EDGE_LOOP('',(#31970,#31971,#31972,#31973,#31974,#31975));
#5410=EDGE_LOOP('',(#31976,#31977,#31978,#31979,#31980,#31981));
#5411=EDGE_LOOP('',(#31982,#31983,#31984,#31985,#31986,#31987));
#5412=EDGE_LOOP('',(#31988,#31989,#31990,#31991,#31992,#31993));
#5413=EDGE_LOOP('',(#31994,#31995,#31996,#31997,#31998,#31999));
#5414=EDGE_LOOP('',(#32000,#32001,#32002,#32003,#32004,#32005));
#5415=EDGE_LOOP('',(#32006,#32007,#32008,#32009,#32010,#32011));
#5416=EDGE_LOOP('',(#32012,#32013,#32014,#32015,#32016,#32017));
#5417=EDGE_LOOP('',(#32018,#32019,#32020,#32021,#32022,#32023));
#5418=EDGE_LOOP('',(#32024,#32025,#32026,#32027,#32028,#32029));
#5419=EDGE_LOOP('',(#32030,#32031,#32032,#32033,#32034,#32035));
#5420=EDGE_LOOP('',(#32036,#32037,#32038,#32039,#32040,#32041));
#5421=EDGE_LOOP('',(#32042,#32043,#32044,#32045,#32046,#32047));
#5422=EDGE_LOOP('',(#32048,#32049,#32050,#32051,#32052,#32053));
#5423=EDGE_LOOP('',(#32054,#32055,#32056,#32057,#32058,#32059));
#5424=EDGE_LOOP('',(#32060,#32061,#32062,#32063,#32064,#32065));
#5425=EDGE_LOOP('',(#32066,#32067,#32068,#32069,#32070,#32071));
#5426=EDGE_LOOP('',(#32072,#32073,#32074,#32075,#32076,#32077));
#5427=EDGE_LOOP('',(#32078,#32079,#32080,#32081,#32082,#32083));
#5428=EDGE_LOOP('',(#32084,#32085,#32086,#32087,#32088,#32089));
#5429=EDGE_LOOP('',(#32090,#32091,#32092,#32093,#32094,#32095));
#5430=EDGE_LOOP('',(#32096,#32097,#32098,#32099,#32100,#32101));
#5431=EDGE_LOOP('',(#32102,#32103,#32104,#32105,#32106,#32107));
#5432=EDGE_LOOP('',(#32108,#32109,#32110,#32111,#32112,#32113));
#5433=EDGE_LOOP('',(#32114,#32115,#32116,#32117,#32118,#32119));
#5434=EDGE_LOOP('',(#32120,#32121,#32122,#32123,#32124,#32125));
#5435=EDGE_LOOP('',(#32126,#32127,#32128,#32129,#32130,#32131));
#5436=EDGE_LOOP('',(#32132,#32133,#32134,#32135,#32136,#32137));
#5437=EDGE_LOOP('',(#32138));
#5438=EDGE_LOOP('',(#32139,#32140,#32141,#32142,#32143,#32144));
#5439=EDGE_LOOP('',(#32145,#32146,#32147,#32148,#32149,#32150));
#5440=EDGE_LOOP('',(#32151,#32152,#32153,#32154,#32155,#32156));
#5441=EDGE_LOOP('',(#32157,#32158,#32159,#32160,#32161,#32162));
#5442=EDGE_LOOP('',(#32163,#32164,#32165,#32166,#32167,#32168));
#5443=EDGE_LOOP('',(#32169,#32170,#32171,#32172,#32173,#32174));
#5444=EDGE_LOOP('',(#32175,#32176,#32177,#32178,#32179,#32180));
#5445=EDGE_LOOP('',(#32181,#32182,#32183,#32184,#32185,#32186));
#5446=EDGE_LOOP('',(#32187,#32188,#32189,#32190,#32191,#32192));
#5447=EDGE_LOOP('',(#32193,#32194,#32195,#32196,#32197,#32198));
#5448=EDGE_LOOP('',(#32199,#32200,#32201,#32202,#32203,#32204));
#5449=EDGE_LOOP('',(#32205,#32206,#32207,#32208,#32209,#32210));
#5450=EDGE_LOOP('',(#32211,#32212,#32213,#32214,#32215,#32216));
#5451=EDGE_LOOP('',(#32217,#32218,#32219,#32220,#32221,#32222));
#5452=EDGE_LOOP('',(#32223,#32224,#32225,#32226,#32227,#32228));
#5453=EDGE_LOOP('',(#32229,#32230,#32231,#32232,#32233,#32234));
#5454=EDGE_LOOP('',(#32235,#32236,#32237,#32238,#32239,#32240));
#5455=EDGE_LOOP('',(#32241,#32242,#32243,#32244,#32245,#32246));
#5456=EDGE_LOOP('',(#32247,#32248,#32249,#32250,#32251,#32252));
#5457=EDGE_LOOP('',(#32253,#32254,#32255,#32256,#32257,#32258));
#5458=EDGE_LOOP('',(#32259,#32260,#32261,#32262,#32263,#32264));
#5459=EDGE_LOOP('',(#32265,#32266,#32267,#32268,#32269,#32270));
#5460=EDGE_LOOP('',(#32271,#32272,#32273,#32274,#32275,#32276));
#5461=EDGE_LOOP('',(#32277,#32278,#32279,#32280,#32281,#32282));
#5462=EDGE_LOOP('',(#32283,#32284,#32285,#32286,#32287,#32288));
#5463=EDGE_LOOP('',(#32289,#32290,#32291,#32292,#32293,#32294));
#5464=EDGE_LOOP('',(#32295,#32296,#32297,#32298,#32299,#32300));
#5465=EDGE_LOOP('',(#32301,#32302,#32303,#32304,#32305,#32306));
#5466=EDGE_LOOP('',(#32307,#32308,#32309,#32310,#32311,#32312));
#5467=EDGE_LOOP('',(#32313,#32314,#32315,#32316,#32317,#32318));
#5468=EDGE_LOOP('',(#32319,#32320,#32321,#32322,#32323,#32324));
#5469=EDGE_LOOP('',(#32325,#32326,#32327,#32328,#32329,#32330));
#5470=EDGE_LOOP('',(#32331,#32332,#32333,#32334,#32335,#32336));
#5471=EDGE_LOOP('',(#32337,#32338,#32339,#32340,#32341,#32342));
#5472=EDGE_LOOP('',(#32343,#32344,#32345,#32346,#32347,#32348));
#5473=EDGE_LOOP('',(#32349,#32350,#32351,#32352,#32353,#32354));
#5474=EDGE_LOOP('',(#32355,#32356,#32357,#32358,#32359,#32360));
#5475=EDGE_LOOP('',(#32361,#32362,#32363,#32364,#32365,#32366));
#5476=EDGE_LOOP('',(#32367,#32368,#32369,#32370,#32371,#32372));
#5477=EDGE_LOOP('',(#32373,#32374,#32375,#32376,#32377,#32378));
#5478=EDGE_LOOP('',(#32379,#32380,#32381,#32382,#32383,#32384));
#5479=EDGE_LOOP('',(#32385,#32386,#32387,#32388,#32389,#32390));
#5480=EDGE_LOOP('',(#32391,#32392,#32393,#32394,#32395,#32396));
#5481=EDGE_LOOP('',(#32397,#32398,#32399,#32400,#32401,#32402));
#5482=EDGE_LOOP('',(#32403,#32404,#32405,#32406,#32407,#32408));
#5483=EDGE_LOOP('',(#32409,#32410,#32411,#32412,#32413,#32414));
#5484=EDGE_LOOP('',(#32415,#32416,#32417,#32418,#32419,#32420));
#5485=EDGE_LOOP('',(#32421,#32422,#32423,#32424,#32425,#32426));
#5486=EDGE_LOOP('',(#32427,#32428,#32429,#32430,#32431,#32432));
#5487=EDGE_LOOP('',(#32433,#32434,#32435,#32436,#32437,#32438));
#5488=EDGE_LOOP('',(#32439,#32440,#32441,#32442,#32443,#32444));
#5489=EDGE_LOOP('',(#32445,#32446,#32447,#32448,#32449,#32450));
#5490=EDGE_LOOP('',(#32451,#32452,#32453,#32454,#32455,#32456));
#5491=EDGE_LOOP('',(#32457,#32458,#32459,#32460,#32461,#32462));
#5492=EDGE_LOOP('',(#32463,#32464,#32465,#32466,#32467,#32468));
#5493=EDGE_LOOP('',(#32469,#32470,#32471,#32472,#32473,#32474));
#5494=EDGE_LOOP('',(#32475,#32476,#32477,#32478,#32479,#32480));
#5495=EDGE_LOOP('',(#32481,#32482,#32483,#32484,#32485,#32486));
#5496=EDGE_LOOP('',(#32487,#32488,#32489,#32490,#32491,#32492));
#5497=EDGE_LOOP('',(#32493,#32494,#32495,#32496,#32497,#32498));
#5498=EDGE_LOOP('',(#32499,#32500,#32501,#32502,#32503,#32504));
#5499=EDGE_LOOP('',(#32505,#32506,#32507,#32508,#32509,#32510));
#5500=EDGE_LOOP('',(#32511,#32512,#32513,#32514,#32515,#32516));
#5501=EDGE_LOOP('',(#32517,#32518,#32519,#32520,#32521,#32522));
#5502=EDGE_LOOP('',(#32523,#32524,#32525,#32526,#32527,#32528));
#5503=EDGE_LOOP('',(#32529,#32530,#32531,#32532,#32533,#32534));
#5504=EDGE_LOOP('',(#32535,#32536,#32537,#32538,#32539,#32540));
#5505=EDGE_LOOP('',(#32541,#32542,#32543,#32544,#32545,#32546));
#5506=EDGE_LOOP('',(#32547,#32548,#32549,#32550,#32551,#32552));
#5507=EDGE_LOOP('',(#32553,#32554,#32555,#32556,#32557,#32558));
#5508=EDGE_LOOP('',(#32559,#32560,#32561,#32562,#32563,#32564));
#5509=EDGE_LOOP('',(#32565,#32566,#32567,#32568,#32569,#32570));
#5510=EDGE_LOOP('',(#32571,#32572,#32573,#32574,#32575,#32576));
#5511=EDGE_LOOP('',(#32577,#32578,#32579,#32580,#32581,#32582));
#5512=EDGE_LOOP('',(#32583,#32584,#32585,#32586,#32587,#32588));
#5513=EDGE_LOOP('',(#32589,#32590,#32591,#32592,#32593,#32594));
#5514=EDGE_LOOP('',(#32595,#32596,#32597,#32598,#32599,#32600));
#5515=EDGE_LOOP('',(#32601,#32602,#32603,#32604,#32605,#32606));
#5516=EDGE_LOOP('',(#32607,#32608,#32609,#32610,#32611,#32612));
#5517=EDGE_LOOP('',(#32613,#32614,#32615,#32616,#32617,#32618));
#5518=EDGE_LOOP('',(#32619,#32620,#32621,#32622,#32623,#32624));
#5519=EDGE_LOOP('',(#32625,#32626,#32627,#32628,#32629,#32630));
#5520=EDGE_LOOP('',(#32631,#32632,#32633,#32634,#32635,#32636));
#5521=EDGE_LOOP('',(#32637,#32638,#32639,#32640,#32641,#32642));
#5522=EDGE_LOOP('',(#32643,#32644,#32645,#32646,#32647,#32648));
#5523=EDGE_LOOP('',(#32649,#32650,#32651,#32652,#32653,#32654));
#5524=EDGE_LOOP('',(#32655,#32656,#32657,#32658,#32659,#32660));
#5525=EDGE_LOOP('',(#32661,#32662,#32663,#32664,#32665,#32666));
#5526=EDGE_LOOP('',(#32667,#32668,#32669,#32670,#32671,#32672));
#5527=EDGE_LOOP('',(#32673,#32674,#32675,#32676,#32677,#32678));
#5528=EDGE_LOOP('',(#32679,#32680,#32681,#32682,#32683,#32684));
#5529=EDGE_LOOP('',(#32685,#32686,#32687,#32688,#32689,#32690));
#5530=EDGE_LOOP('',(#32691,#32692,#32693,#32694,#32695,#32696));
#5531=EDGE_LOOP('',(#32697,#32698,#32699,#32700,#32701,#32702));
#5532=EDGE_LOOP('',(#32703,#32704,#32705,#32706,#32707,#32708));
#5533=EDGE_LOOP('',(#32709,#32710,#32711,#32712,#32713,#32714));
#5534=EDGE_LOOP('',(#32715,#32716,#32717,#32718,#32719,#32720));
#5535=EDGE_LOOP('',(#32721,#32722,#32723,#32724,#32725,#32726));
#5536=EDGE_LOOP('',(#32727,#32728,#32729,#32730,#32731,#32732));
#5537=EDGE_LOOP('',(#32733,#32734,#32735,#32736,#32737,#32738));
#5538=EDGE_LOOP('',(#32739,#32740,#32741,#32742,#32743,#32744));
#5539=EDGE_LOOP('',(#32745,#32746,#32747,#32748,#32749,#32750));
#5540=EDGE_LOOP('',(#32751,#32752,#32753,#32754,#32755,#32756));
#5541=EDGE_LOOP('',(#32757,#32758,#32759,#32760,#32761,#32762));
#5542=EDGE_LOOP('',(#32763,#32764,#32765,#32766,#32767,#32768));
#5543=EDGE_LOOP('',(#32769,#32770,#32771,#32772,#32773,#32774));
#5544=EDGE_LOOP('',(#32775,#32776,#32777,#32778,#32779,#32780));
#5545=EDGE_LOOP('',(#32781,#32782,#32783,#32784,#32785,#32786));
#5546=EDGE_LOOP('',(#32787,#32788,#32789,#32790,#32791,#32792));
#5547=EDGE_LOOP('',(#32793,#32794,#32795,#32796,#32797,#32798));
#5548=EDGE_LOOP('',(#32799,#32800,#32801,#32802,#32803,#32804));
#5549=EDGE_LOOP('',(#32805,#32806,#32807,#32808,#32809,#32810));
#5550=EDGE_LOOP('',(#32811,#32812,#32813,#32814,#32815,#32816));
#5551=EDGE_LOOP('',(#32817,#32818,#32819,#32820,#32821,#32822));
#5552=EDGE_LOOP('',(#32823,#32824,#32825,#32826,#32827,#32828));
#5553=EDGE_LOOP('',(#32829,#32830,#32831,#32832,#32833,#32834));
#5554=EDGE_LOOP('',(#32835,#32836,#32837,#32838,#32839,#32840));
#5555=EDGE_LOOP('',(#32841,#32842,#32843,#32844,#32845,#32846));
#5556=EDGE_LOOP('',(#32847,#32848,#32849,#32850,#32851,#32852));
#5557=EDGE_LOOP('',(#32853,#32854,#32855,#32856,#32857,#32858));
#5558=EDGE_LOOP('',(#32859,#32860,#32861,#32862,#32863,#32864));
#5559=EDGE_LOOP('',(#32865,#32866,#32867,#32868,#32869,#32870));
#5560=EDGE_LOOP('',(#32871,#32872,#32873,#32874,#32875,#32876));
#5561=EDGE_LOOP('',(#32877,#32878,#32879,#32880,#32881,#32882));
#5562=EDGE_LOOP('',(#32883,#32884,#32885,#32886,#32887,#32888));
#5563=EDGE_LOOP('',(#32889,#32890,#32891,#32892,#32893,#32894));
#5564=EDGE_LOOP('',(#32895,#32896,#32897,#32898,#32899,#32900));
#5565=EDGE_LOOP('',(#32901,#32902,#32903,#32904,#32905,#32906));
#5566=EDGE_LOOP('',(#32907,#32908,#32909,#32910,#32911,#32912));
#5567=EDGE_LOOP('',(#32913,#32914,#32915,#32916,#32917,#32918));
#5568=EDGE_LOOP('',(#32919,#32920,#32921,#32922,#32923,#32924));
#5569=EDGE_LOOP('',(#32925,#32926,#32927,#32928,#32929,#32930));
#5570=EDGE_LOOP('',(#32931,#32932,#32933,#32934,#32935,#32936));
#5571=EDGE_LOOP('',(#32937,#32938,#32939,#32940,#32941,#32942));
#5572=EDGE_LOOP('',(#32943,#32944,#32945,#32946,#32947,#32948));
#5573=EDGE_LOOP('',(#32949,#32950,#32951,#32952,#32953,#32954));
#5574=EDGE_LOOP('',(#32955,#32956,#32957,#32958,#32959,#32960));
#5575=EDGE_LOOP('',(#32961,#32962,#32963,#32964,#32965,#32966));
#5576=EDGE_LOOP('',(#32967,#32968,#32969,#32970,#32971,#32972));
#5577=EDGE_LOOP('',(#32973,#32974,#32975,#32976,#32977,#32978));
#5578=EDGE_LOOP('',(#32979,#32980,#32981,#32982,#32983,#32984));
#5579=EDGE_LOOP('',(#32985,#32986,#32987,#32988,#32989,#32990));
#5580=EDGE_LOOP('',(#32991,#32992,#32993,#32994,#32995,#32996));
#5581=EDGE_LOOP('',(#32997,#32998,#32999,#33000,#33001,#33002));
#5582=EDGE_LOOP('',(#33003,#33004,#33005,#33006,#33007,#33008));
#5583=EDGE_LOOP('',(#33009,#33010,#33011,#33012,#33013,#33014));
#5584=EDGE_LOOP('',(#33015,#33016,#33017,#33018,#33019,#33020));
#5585=EDGE_LOOP('',(#33021,#33022,#33023,#33024,#33025,#33026));
#5586=EDGE_LOOP('',(#33027,#33028,#33029,#33030,#33031,#33032));
#5587=EDGE_LOOP('',(#33033,#33034,#33035,#33036,#33037,#33038));
#5588=EDGE_LOOP('',(#33039,#33040,#33041,#33042,#33043,#33044));
#5589=EDGE_LOOP('',(#33045,#33046,#33047,#33048,#33049,#33050));
#5590=EDGE_LOOP('',(#33051,#33052,#33053,#33054,#33055,#33056));
#5591=EDGE_LOOP('',(#33057,#33058,#33059,#33060,#33061,#33062));
#5592=EDGE_LOOP('',(#33063,#33064,#33065,#33066,#33067,#33068));
#5593=EDGE_LOOP('',(#33069,#33070,#33071,#33072,#33073,#33074));
#5594=EDGE_LOOP('',(#33075,#33076,#33077,#33078,#33079,#33080));
#5595=EDGE_LOOP('',(#33081,#33082,#33083,#33084,#33085,#33086));
#5596=EDGE_LOOP('',(#33087,#33088,#33089,#33090,#33091,#33092));
#5597=EDGE_LOOP('',(#33093,#33094,#33095,#33096,#33097,#33098));
#5598=EDGE_LOOP('',(#33099,#33100,#33101,#33102,#33103,#33104));
#5599=EDGE_LOOP('',(#33105,#33106,#33107,#33108,#33109,#33110));
#5600=EDGE_LOOP('',(#33111,#33112,#33113,#33114,#33115,#33116));
#5601=EDGE_LOOP('',(#33117,#33118,#33119,#33120,#33121,#33122));
#5602=EDGE_LOOP('',(#33123,#33124,#33125,#33126,#33127,#33128));
#5603=EDGE_LOOP('',(#33129,#33130,#33131,#33132,#33133,#33134));
#5604=EDGE_LOOP('',(#33135,#33136,#33137,#33138,#33139,#33140));
#5605=EDGE_LOOP('',(#33141,#33142,#33143,#33144,#33145,#33146));
#5606=EDGE_LOOP('',(#33147,#33148,#33149,#33150,#33151,#33152));
#5607=EDGE_LOOP('',(#33153,#33154,#33155,#33156,#33157,#33158));
#5608=EDGE_LOOP('',(#33159,#33160,#33161,#33162,#33163,#33164));
#5609=EDGE_LOOP('',(#33165,#33166,#33167,#33168,#33169,#33170));
#5610=EDGE_LOOP('',(#33171,#33172,#33173,#33174,#33175,#33176));
#5611=EDGE_LOOP('',(#33177,#33178,#33179,#33180,#33181,#33182));
#5612=EDGE_LOOP('',(#33183,#33184,#33185,#33186,#33187,#33188));
#5613=EDGE_LOOP('',(#33189,#33190,#33191,#33192,#33193,#33194));
#5614=EDGE_LOOP('',(#33195,#33196,#33197,#33198,#33199,#33200));
#5615=EDGE_LOOP('',(#33201,#33202,#33203,#33204,#33205,#33206));
#5616=EDGE_LOOP('',(#33207,#33208,#33209,#33210,#33211,#33212));
#5617=EDGE_LOOP('',(#33213,#33214,#33215,#33216,#33217,#33218));
#5618=EDGE_LOOP('',(#33219,#33220,#33221,#33222,#33223,#33224));
#5619=EDGE_LOOP('',(#33225,#33226,#33227,#33228,#33229,#33230));
#5620=EDGE_LOOP('',(#33231,#33232,#33233,#33234,#33235,#33236));
#5621=EDGE_LOOP('',(#33237,#33238,#33239,#33240,#33241,#33242));
#5622=EDGE_LOOP('',(#33243,#33244,#33245,#33246,#33247,#33248));
#5623=EDGE_LOOP('',(#33249,#33250,#33251,#33252,#33253,#33254));
#5624=EDGE_LOOP('',(#33255,#33256,#33257,#33258));
#5625=EDGE_LOOP('',(#33259,#33260,#33261,#33262));
#5626=EDGE_LOOP('',(#33263,#33264,#33265,#33266));
#5627=EDGE_LOOP('',(#33267,#33268,#33269,#33270));
#5628=EDGE_LOOP('',(#33271,#33272,#33273,#33274));
#5629=EDGE_LOOP('',(#33275,#33276,#33277,#33278));
#5630=EDGE_LOOP('',(#33279,#33280,#33281,#33282));
#5631=EDGE_LOOP('',(#33283,#33284,#33285,#33286));
#5632=EDGE_LOOP('',(#33287,#33288,#33289,#33290));
#5633=EDGE_LOOP('',(#33291,#33292,#33293,#33294));
#5634=EDGE_LOOP('',(#33295,#33296,#33297,#33298));
#5635=EDGE_LOOP('',(#33299,#33300,#33301,#33302));
#5636=EDGE_LOOP('',(#33303,#33304,#33305,#33306));
#5637=EDGE_LOOP('',(#33307,#33308,#33309,#33310));
#5638=EDGE_LOOP('',(#33311,#33312,#33313,#33314));
#5639=EDGE_LOOP('',(#33315,#33316,#33317,#33318));
#5640=EDGE_LOOP('',(#33319,#33320,#33321,#33322));
#5641=EDGE_LOOP('',(#33323,#33324,#33325,#33326));
#5642=EDGE_LOOP('',(#33327,#33328,#33329,#33330));
#5643=EDGE_LOOP('',(#33331,#33332,#33333,#33334));
#5644=EDGE_LOOP('',(#33335,#33336,#33337,#33338));
#5645=EDGE_LOOP('',(#33339,#33340,#33341,#33342));
#5646=EDGE_LOOP('',(#33343,#33344,#33345,#33346));
#5647=EDGE_LOOP('',(#33347,#33348,#33349,#33350));
#5648=EDGE_LOOP('',(#33351,#33352,#33353,#33354));
#5649=EDGE_LOOP('',(#33355,#33356,#33357,#33358));
#5650=EDGE_LOOP('',(#33359,#33360,#33361,#33362));
#5651=EDGE_LOOP('',(#33363,#33364,#33365,#33366));
#5652=EDGE_LOOP('',(#33367,#33368,#33369,#33370));
#5653=EDGE_LOOP('',(#33371,#33372,#33373,#33374));
#5654=EDGE_LOOP('',(#33375,#33376,#33377,#33378));
#5655=EDGE_LOOP('',(#33379,#33380,#33381,#33382));
#5656=EDGE_LOOP('',(#33383,#33384,#33385,#33386));
#5657=EDGE_LOOP('',(#33387,#33388,#33389,#33390));
#5658=EDGE_LOOP('',(#33391,#33392,#33393,#33394));
#5659=EDGE_LOOP('',(#33395,#33396,#33397,#33398));
#5660=EDGE_LOOP('',(#33399,#33400,#33401,#33402));
#5661=EDGE_LOOP('',(#33403,#33404,#33405,#33406));
#5662=EDGE_LOOP('',(#33407,#33408,#33409,#33410));
#5663=EDGE_LOOP('',(#33411,#33412,#33413,#33414));
#5664=EDGE_LOOP('',(#33415,#33416,#33417,#33418));
#5665=EDGE_LOOP('',(#33419,#33420,#33421,#33422));
#5666=EDGE_LOOP('',(#33423,#33424,#33425,#33426));
#5667=EDGE_LOOP('',(#33427,#33428,#33429,#33430));
#5668=EDGE_LOOP('',(#33431,#33432,#33433,#33434));
#5669=EDGE_LOOP('',(#33435,#33436,#33437,#33438));
#5670=EDGE_LOOP('',(#33439,#33440,#33441,#33442));
#5671=EDGE_LOOP('',(#33443,#33444,#33445,#33446));
#5672=EDGE_LOOP('',(#33447,#33448,#33449,#33450));
#5673=EDGE_LOOP('',(#33451,#33452,#33453,#33454));
#5674=EDGE_LOOP('',(#33455,#33456,#33457,#33458));
#5675=EDGE_LOOP('',(#33459,#33460,#33461,#33462));
#5676=EDGE_LOOP('',(#33463,#33464,#33465,#33466));
#5677=EDGE_LOOP('',(#33467,#33468,#33469,#33470));
#5678=EDGE_LOOP('',(#33471,#33472,#33473,#33474));
#5679=EDGE_LOOP('',(#33475,#33476,#33477,#33478));
#5680=EDGE_LOOP('',(#33479,#33480,#33481,#33482));
#5681=EDGE_LOOP('',(#33483,#33484,#33485,#33486));
#5682=EDGE_LOOP('',(#33487,#33488,#33489,#33490));
#5683=EDGE_LOOP('',(#33491,#33492,#33493,#33494));
#5684=EDGE_LOOP('',(#33495,#33496,#33497,#33498));
#5685=EDGE_LOOP('',(#33499,#33500,#33501,#33502));
#5686=EDGE_LOOP('',(#33503,#33504,#33505,#33506));
#5687=EDGE_LOOP('',(#33507,#33508,#33509,#33510));
#5688=EDGE_LOOP('',(#33511,#33512,#33513,#33514));
#5689=EDGE_LOOP('',(#33515,#33516,#33517,#33518));
#5690=EDGE_LOOP('',(#33519,#33520,#33521,#33522));
#5691=EDGE_LOOP('',(#33523,#33524,#33525,#33526));
#5692=EDGE_LOOP('',(#33527,#33528,#33529,#33530));
#5693=EDGE_LOOP('',(#33531,#33532,#33533,#33534));
#5694=EDGE_LOOP('',(#33535,#33536,#33537,#33538));
#5695=EDGE_LOOP('',(#33539,#33540,#33541,#33542));
#5696=EDGE_LOOP('',(#33543,#33544,#33545,#33546));
#5697=EDGE_LOOP('',(#33547,#33548,#33549,#33550));
#5698=EDGE_LOOP('',(#33551,#33552,#33553,#33554));
#5699=EDGE_LOOP('',(#33555,#33556,#33557,#33558));
#5700=EDGE_LOOP('',(#33559,#33560,#33561,#33562));
#5701=EDGE_LOOP('',(#33563,#33564,#33565,#33566));
#5702=EDGE_LOOP('',(#33567,#33568,#33569,#33570));
#5703=EDGE_LOOP('',(#33571,#33572,#33573,#33574));
#5704=EDGE_LOOP('',(#33575,#33576,#33577,#33578));
#5705=EDGE_LOOP('',(#33579,#33580,#33581,#33582));
#5706=EDGE_LOOP('',(#33583,#33584,#33585,#33586));
#5707=EDGE_LOOP('',(#33587,#33588,#33589,#33590));
#5708=EDGE_LOOP('',(#33591,#33592,#33593,#33594));
#5709=EDGE_LOOP('',(#33595,#33596,#33597,#33598));
#5710=EDGE_LOOP('',(#33599,#33600,#33601,#33602));
#5711=EDGE_LOOP('',(#33603,#33604,#33605,#33606));
#5712=EDGE_LOOP('',(#33607,#33608,#33609,#33610));
#5713=EDGE_LOOP('',(#33611,#33612,#33613,#33614));
#5714=EDGE_LOOP('',(#33615,#33616,#33617,#33618));
#5715=EDGE_LOOP('',(#33619,#33620,#33621,#33622));
#5716=EDGE_LOOP('',(#33623,#33624,#33625,#33626));
#5717=EDGE_LOOP('',(#33627,#33628,#33629,#33630));
#5718=EDGE_LOOP('',(#33631,#33632,#33633,#33634));
#5719=EDGE_LOOP('',(#33635,#33636,#33637,#33638));
#5720=EDGE_LOOP('',(#33639,#33640,#33641,#33642));
#5721=EDGE_LOOP('',(#33643,#33644,#33645,#33646));
#5722=EDGE_LOOP('',(#33647,#33648,#33649,#33650));
#5723=EDGE_LOOP('',(#33651,#33652,#33653,#33654));
#5724=EDGE_LOOP('',(#33655,#33656,#33657,#33658));
#5725=EDGE_LOOP('',(#33659,#33660,#33661,#33662));
#5726=EDGE_LOOP('',(#33663,#33664,#33665,#33666));
#5727=EDGE_LOOP('',(#33667,#33668,#33669,#33670));
#5728=EDGE_LOOP('',(#33671,#33672,#33673,#33674));
#5729=EDGE_LOOP('',(#33675,#33676,#33677,#33678));
#5730=EDGE_LOOP('',(#33679,#33680,#33681,#33682));
#5731=EDGE_LOOP('',(#33683,#33684,#33685,#33686));
#5732=EDGE_LOOP('',(#33687,#33688,#33689,#33690));
#5733=EDGE_LOOP('',(#33691,#33692,#33693,#33694));
#5734=EDGE_LOOP('',(#33695,#33696,#33697,#33698));
#5735=EDGE_LOOP('',(#33699,#33700,#33701,#33702));
#5736=EDGE_LOOP('',(#33703,#33704,#33705,#33706));
#5737=EDGE_LOOP('',(#33707,#33708,#33709,#33710));
#5738=EDGE_LOOP('',(#33711,#33712,#33713,#33714));
#5739=EDGE_LOOP('',(#33715,#33716,#33717,#33718));
#5740=EDGE_LOOP('',(#33719,#33720,#33721,#33722));
#5741=EDGE_LOOP('',(#33723,#33724,#33725,#33726));
#5742=EDGE_LOOP('',(#33727,#33728,#33729,#33730));
#5743=EDGE_LOOP('',(#33731,#33732,#33733,#33734));
#5744=EDGE_LOOP('',(#33735,#33736,#33737,#33738));
#5745=EDGE_LOOP('',(#33739,#33740,#33741,#33742));
#5746=EDGE_LOOP('',(#33743,#33744,#33745,#33746));
#5747=EDGE_LOOP('',(#33747,#33748,#33749,#33750));
#5748=EDGE_LOOP('',(#33751,#33752,#33753,#33754));
#5749=EDGE_LOOP('',(#33755,#33756,#33757,#33758));
#5750=EDGE_LOOP('',(#33759,#33760,#33761,#33762));
#5751=EDGE_LOOP('',(#33763,#33764,#33765,#33766));
#5752=EDGE_LOOP('',(#33767,#33768,#33769,#33770));
#5753=EDGE_LOOP('',(#33771,#33772,#33773,#33774));
#5754=EDGE_LOOP('',(#33775,#33776,#33777,#33778));
#5755=EDGE_LOOP('',(#33779,#33780,#33781,#33782));
#5756=EDGE_LOOP('',(#33783,#33784,#33785,#33786));
#5757=EDGE_LOOP('',(#33787,#33788,#33789,#33790));
#5758=EDGE_LOOP('',(#33791,#33792,#33793,#33794));
#5759=EDGE_LOOP('',(#33795,#33796,#33797,#33798));
#5760=EDGE_LOOP('',(#33799,#33800,#33801,#33802));
#5761=EDGE_LOOP('',(#33803,#33804,#33805,#33806));
#5762=EDGE_LOOP('',(#33807,#33808,#33809,#33810));
#5763=EDGE_LOOP('',(#33811,#33812,#33813,#33814));
#5764=EDGE_LOOP('',(#33815,#33816,#33817,#33818));
#5765=EDGE_LOOP('',(#33819,#33820,#33821,#33822));
#5766=EDGE_LOOP('',(#33823,#33824,#33825,#33826));
#5767=EDGE_LOOP('',(#33827,#33828,#33829,#33830));
#5768=EDGE_LOOP('',(#33831,#33832,#33833,#33834));
#5769=EDGE_LOOP('',(#33835,#33836,#33837,#33838));
#5770=EDGE_LOOP('',(#33839,#33840,#33841,#33842));
#5771=EDGE_LOOP('',(#33843,#33844,#33845,#33846));
#5772=EDGE_LOOP('',(#33847,#33848,#33849,#33850));
#5773=EDGE_LOOP('',(#33851,#33852,#33853,#33854));
#5774=EDGE_LOOP('',(#33855,#33856,#33857,#33858));
#5775=EDGE_LOOP('',(#33859,#33860,#33861,#33862));
#5776=EDGE_LOOP('',(#33863,#33864,#33865,#33866));
#5777=EDGE_LOOP('',(#33867,#33868,#33869,#33870));
#5778=EDGE_LOOP('',(#33871,#33872,#33873,#33874));
#5779=EDGE_LOOP('',(#33875,#33876,#33877,#33878));
#5780=EDGE_LOOP('',(#33879,#33880,#33881,#33882));
#5781=EDGE_LOOP('',(#33883,#33884,#33885,#33886));
#5782=EDGE_LOOP('',(#33887,#33888,#33889,#33890));
#5783=EDGE_LOOP('',(#33891,#33892,#33893,#33894));
#5784=EDGE_LOOP('',(#33895,#33896,#33897,#33898));
#5785=EDGE_LOOP('',(#33899,#33900,#33901,#33902));
#5786=EDGE_LOOP('',(#33903,#33904,#33905,#33906));
#5787=EDGE_LOOP('',(#33907,#33908,#33909,#33910));
#5788=EDGE_LOOP('',(#33911,#33912,#33913,#33914));
#5789=EDGE_LOOP('',(#33915,#33916,#33917,#33918));
#5790=EDGE_LOOP('',(#33919,#33920,#33921,#33922));
#5791=EDGE_LOOP('',(#33923,#33924,#33925,#33926));
#5792=EDGE_LOOP('',(#33927,#33928,#33929,#33930));
#5793=EDGE_LOOP('',(#33931,#33932,#33933,#33934));
#5794=EDGE_LOOP('',(#33935,#33936,#33937,#33938));
#5795=EDGE_LOOP('',(#33939,#33940,#33941,#33942));
#5796=EDGE_LOOP('',(#33943,#33944,#33945,#33946));
#5797=EDGE_LOOP('',(#33947,#33948,#33949,#33950));
#5798=EDGE_LOOP('',(#33951,#33952,#33953,#33954));
#5799=EDGE_LOOP('',(#33955,#33956,#33957,#33958));
#5800=EDGE_LOOP('',(#33959,#33960,#33961,#33962));
#5801=EDGE_LOOP('',(#33963,#33964,#33965,#33966));
#5802=EDGE_LOOP('',(#33967,#33968,#33969,#33970));
#5803=EDGE_LOOP('',(#33971,#33972,#33973,#33974));
#5804=EDGE_LOOP('',(#33975,#33976,#33977,#33978));
#5805=EDGE_LOOP('',(#33979,#33980,#33981,#33982));
#5806=EDGE_LOOP('',(#33983,#33984,#33985,#33986));
#5807=EDGE_LOOP('',(#33987,#33988,#33989,#33990));
#5808=EDGE_LOOP('',(#33991,#33992,#33993,#33994));
#5809=EDGE_LOOP('',(#33995,#33996,#33997,#33998));
#5810=EDGE_LOOP('',(#33999,#34000,#34001,#34002));
#5811=EDGE_LOOP('',(#34003,#34004,#34005,#34006));
#5812=EDGE_LOOP('',(#34007,#34008,#34009,#34010));
#5813=EDGE_LOOP('',(#34011,#34012,#34013,#34014));
#5814=EDGE_LOOP('',(#34015,#34016,#34017,#34018));
#5815=EDGE_LOOP('',(#34019,#34020,#34021,#34022));
#5816=EDGE_LOOP('',(#34023,#34024,#34025,#34026));
#5817=EDGE_LOOP('',(#34027,#34028,#34029,#34030));
#5818=EDGE_LOOP('',(#34031,#34032,#34033,#34034));
#5819=EDGE_LOOP('',(#34035,#34036,#34037,#34038));
#5820=EDGE_LOOP('',(#34039,#34040,#34041,#34042));
#5821=EDGE_LOOP('',(#34043,#34044,#34045,#34046));
#5822=EDGE_LOOP('',(#34047,#34048,#34049,#34050));
#5823=EDGE_LOOP('',(#34051,#34052,#34053,#34054));
#5824=EDGE_LOOP('',(#34055,#34056,#34057,#34058));
#5825=EDGE_LOOP('',(#34059,#34060,#34061,#34062));
#5826=EDGE_LOOP('',(#34063,#34064,#34065,#34066));
#5827=EDGE_LOOP('',(#34067,#34068,#34069,#34070));
#5828=EDGE_LOOP('',(#34071,#34072,#34073,#34074));
#5829=EDGE_LOOP('',(#34075,#34076,#34077,#34078));
#5830=EDGE_LOOP('',(#34079,#34080,#34081,#34082));
#5831=EDGE_LOOP('',(#34083,#34084,#34085,#34086));
#5832=EDGE_LOOP('',(#34087,#34088,#34089,#34090));
#5833=EDGE_LOOP('',(#34091,#34092,#34093,#34094));
#5834=EDGE_LOOP('',(#34095,#34096,#34097,#34098));
#5835=EDGE_LOOP('',(#34099,#34100,#34101,#34102));
#5836=EDGE_LOOP('',(#34103,#34104,#34105,#34106));
#5837=EDGE_LOOP('',(#34107,#34108,#34109,#34110));
#5838=EDGE_LOOP('',(#34111,#34112,#34113,#34114));
#5839=EDGE_LOOP('',(#34115,#34116,#34117,#34118));
#5840=EDGE_LOOP('',(#34119,#34120,#34121,#34122));
#5841=EDGE_LOOP('',(#34123,#34124,#34125,#34126));
#5842=EDGE_LOOP('',(#34127,#34128,#34129,#34130));
#5843=EDGE_LOOP('',(#34131,#34132,#34133,#34134));
#5844=EDGE_LOOP('',(#34135,#34136,#34137,#34138));
#5845=EDGE_LOOP('',(#34139,#34140,#34141,#34142));
#5846=EDGE_LOOP('',(#34143,#34144,#34145,#34146));
#5847=EDGE_LOOP('',(#34147,#34148,#34149,#34150));
#5848=EDGE_LOOP('',(#34151,#34152,#34153,#34154));
#5849=EDGE_LOOP('',(#34155,#34156,#34157,#34158));
#5850=EDGE_LOOP('',(#34159,#34160,#34161,#34162));
#5851=EDGE_LOOP('',(#34163,#34164,#34165,#34166));
#5852=EDGE_LOOP('',(#34167,#34168,#34169,#34170));
#5853=EDGE_LOOP('',(#34171,#34172,#34173,#34174));
#5854=EDGE_LOOP('',(#34175,#34176,#34177,#34178));
#5855=EDGE_LOOP('',(#34179,#34180,#34181,#34182));
#5856=EDGE_LOOP('',(#34183,#34184,#34185,#34186));
#5857=EDGE_LOOP('',(#34187,#34188,#34189,#34190));
#5858=EDGE_LOOP('',(#34191,#34192,#34193,#34194));
#5859=EDGE_LOOP('',(#34195,#34196,#34197,#34198));
#5860=EDGE_LOOP('',(#34199,#34200,#34201,#34202));
#5861=EDGE_LOOP('',(#34203,#34204,#34205,#34206));
#5862=EDGE_LOOP('',(#34207,#34208,#34209,#34210));
#5863=EDGE_LOOP('',(#34211,#34212,#34213,#34214));
#5864=EDGE_LOOP('',(#34215,#34216,#34217,#34218));
#5865=EDGE_LOOP('',(#34219,#34220,#34221,#34222));
#5866=EDGE_LOOP('',(#34223,#34224,#34225,#34226));
#5867=EDGE_LOOP('',(#34227,#34228,#34229,#34230));
#5868=EDGE_LOOP('',(#34231,#34232,#34233,#34234));
#5869=EDGE_LOOP('',(#34235,#34236,#34237,#34238));
#5870=EDGE_LOOP('',(#34239,#34240,#34241,#34242));
#5871=EDGE_LOOP('',(#34243,#34244,#34245,#34246));
#5872=EDGE_LOOP('',(#34247,#34248,#34249,#34250));
#5873=EDGE_LOOP('',(#34251,#34252,#34253,#34254));
#5874=EDGE_LOOP('',(#34255,#34256,#34257,#34258));
#5875=EDGE_LOOP('',(#34259,#34260,#34261,#34262));
#5876=EDGE_LOOP('',(#34263,#34264,#34265,#34266));
#5877=EDGE_LOOP('',(#34267,#34268,#34269,#34270));
#5878=EDGE_LOOP('',(#34271,#34272,#34273,#34274));
#5879=EDGE_LOOP('',(#34275,#34276,#34277,#34278));
#5880=EDGE_LOOP('',(#34279,#34280,#34281,#34282));
#5881=EDGE_LOOP('',(#34283,#34284,#34285,#34286));
#5882=EDGE_LOOP('',(#34287,#34288,#34289,#34290));
#5883=EDGE_LOOP('',(#34291,#34292,#34293,#34294));
#5884=EDGE_LOOP('',(#34295,#34296,#34297,#34298));
#5885=EDGE_LOOP('',(#34299,#34300,#34301,#34302));
#5886=EDGE_LOOP('',(#34303,#34304,#34305,#34306));
#5887=EDGE_LOOP('',(#34307,#34308,#34309,#34310));
#5888=EDGE_LOOP('',(#34311,#34312,#34313,#34314));
#5889=EDGE_LOOP('',(#34315,#34316,#34317,#34318));
#5890=EDGE_LOOP('',(#34319,#34320,#34321,#34322));
#5891=EDGE_LOOP('',(#34323,#34324,#34325,#34326));
#5892=EDGE_LOOP('',(#34327,#34328,#34329,#34330));
#5893=EDGE_LOOP('',(#34331,#34332,#34333,#34334));
#5894=EDGE_LOOP('',(#34335,#34336,#34337,#34338));
#5895=EDGE_LOOP('',(#34339,#34340,#34341,#34342));
#5896=EDGE_LOOP('',(#34343,#34344,#34345,#34346));
#5897=EDGE_LOOP('',(#34347,#34348,#34349,#34350));
#5898=EDGE_LOOP('',(#34351,#34352,#34353,#34354));
#5899=EDGE_LOOP('',(#34355,#34356,#34357,#34358));
#5900=EDGE_LOOP('',(#34359,#34360,#34361,#34362));
#5901=EDGE_LOOP('',(#34363,#34364,#34365,#34366));
#5902=EDGE_LOOP('',(#34367,#34368,#34369,#34370));
#5903=EDGE_LOOP('',(#34371,#34372,#34373,#34374));
#5904=EDGE_LOOP('',(#34375,#34376,#34377,#34378));
#5905=EDGE_LOOP('',(#34379,#34380,#34381,#34382));
#5906=EDGE_LOOP('',(#34383,#34384,#34385,#34386));
#5907=EDGE_LOOP('',(#34387,#34388,#34389,#34390));
#5908=EDGE_LOOP('',(#34391,#34392,#34393,#34394));
#5909=EDGE_LOOP('',(#34395,#34396,#34397,#34398));
#5910=EDGE_LOOP('',(#34399,#34400,#34401,#34402));
#5911=EDGE_LOOP('',(#34403,#34404,#34405,#34406));
#5912=EDGE_LOOP('',(#34407,#34408,#34409,#34410));
#5913=EDGE_LOOP('',(#34411,#34412,#34413,#34414));
#5914=EDGE_LOOP('',(#34415,#34416,#34417,#34418));
#5915=EDGE_LOOP('',(#34419,#34420,#34421,#34422));
#5916=EDGE_LOOP('',(#34423,#34424,#34425,#34426));
#5917=EDGE_LOOP('',(#34427,#34428,#34429,#34430));
#5918=EDGE_LOOP('',(#34431,#34432,#34433,#34434));
#5919=EDGE_LOOP('',(#34435,#34436,#34437,#34438));
#5920=EDGE_LOOP('',(#34439,#34440,#34441,#34442));
#5921=EDGE_LOOP('',(#34443,#34444,#34445,#34446));
#5922=EDGE_LOOP('',(#34447,#34448,#34449,#34450));
#5923=EDGE_LOOP('',(#34451,#34452,#34453,#34454));
#5924=EDGE_LOOP('',(#34455,#34456,#34457,#34458));
#5925=EDGE_LOOP('',(#34459,#34460,#34461,#34462));
#5926=EDGE_LOOP('',(#34463,#34464,#34465,#34466));
#5927=EDGE_LOOP('',(#34467,#34468,#34469,#34470));
#5928=EDGE_LOOP('',(#34471,#34472,#34473,#34474));
#5929=EDGE_LOOP('',(#34475,#34476,#34477,#34478));
#5930=EDGE_LOOP('',(#34479,#34480,#34481,#34482));
#5931=EDGE_LOOP('',(#34483,#34484,#34485,#34486));
#5932=EDGE_LOOP('',(#34487,#34488,#34489,#34490));
#5933=EDGE_LOOP('',(#34491,#34492,#34493,#34494));
#5934=EDGE_LOOP('',(#34495,#34496,#34497,#34498));
#5935=EDGE_LOOP('',(#34499,#34500,#34501,#34502));
#5936=EDGE_LOOP('',(#34503,#34504,#34505,#34506));
#5937=EDGE_LOOP('',(#34507,#34508,#34509,#34510));
#5938=EDGE_LOOP('',(#34511,#34512,#34513,#34514));
#5939=EDGE_LOOP('',(#34515,#34516,#34517,#34518));
#5940=EDGE_LOOP('',(#34519,#34520,#34521,#34522));
#5941=EDGE_LOOP('',(#34523,#34524,#34525,#34526));
#5942=EDGE_LOOP('',(#34527,#34528,#34529,#34530));
#5943=EDGE_LOOP('',(#34531,#34532,#34533,#34534));
#5944=EDGE_LOOP('',(#34535,#34536,#34537,#34538));
#5945=EDGE_LOOP('',(#34539,#34540,#34541,#34542));
#5946=EDGE_LOOP('',(#34543,#34544,#34545,#34546));
#5947=EDGE_LOOP('',(#34547,#34548,#34549,#34550));
#5948=EDGE_LOOP('',(#34551,#34552,#34553,#34554));
#5949=EDGE_LOOP('',(#34555,#34556,#34557,#34558));
#5950=EDGE_LOOP('',(#34559,#34560,#34561,#34562));
#5951=EDGE_LOOP('',(#34563,#34564,#34565,#34566));
#5952=EDGE_LOOP('',(#34567,#34568,#34569,#34570));
#5953=EDGE_LOOP('',(#34571,#34572,#34573,#34574));
#5954=EDGE_LOOP('',(#34575,#34576,#34577,#34578));
#5955=EDGE_LOOP('',(#34579,#34580,#34581,#34582));
#5956=EDGE_LOOP('',(#34583,#34584,#34585,#34586));
#5957=EDGE_LOOP('',(#34587,#34588,#34589,#34590));
#5958=EDGE_LOOP('',(#34591,#34592,#34593,#34594));
#5959=EDGE_LOOP('',(#34595,#34596,#34597,#34598));
#5960=EDGE_LOOP('',(#34599,#34600,#34601,#34602));
#5961=EDGE_LOOP('',(#34603,#34604,#34605,#34606));
#5962=EDGE_LOOP('',(#34607,#34608,#34609,#34610));
#5963=EDGE_LOOP('',(#34611,#34612,#34613,#34614));
#5964=EDGE_LOOP('',(#34615,#34616,#34617,#34618));
#5965=EDGE_LOOP('',(#34619,#34620,#34621,#34622));
#5966=EDGE_LOOP('',(#34623,#34624,#34625,#34626));
#5967=EDGE_LOOP('',(#34627,#34628,#34629,#34630));
#5968=EDGE_LOOP('',(#34631,#34632,#34633,#34634));
#5969=EDGE_LOOP('',(#34635,#34636,#34637,#34638));
#5970=EDGE_LOOP('',(#34639,#34640,#34641,#34642));
#5971=EDGE_LOOP('',(#34643,#34644,#34645,#34646));
#5972=EDGE_LOOP('',(#34647,#34648,#34649,#34650));
#5973=EDGE_LOOP('',(#34651,#34652,#34653,#34654));
#5974=EDGE_LOOP('',(#34655,#34656,#34657,#34658));
#5975=EDGE_LOOP('',(#34659,#34660,#34661,#34662));
#5976=EDGE_LOOP('',(#34663,#34664,#34665,#34666));
#5977=EDGE_LOOP('',(#34667,#34668,#34669,#34670));
#5978=EDGE_LOOP('',(#34671,#34672,#34673,#34674));
#5979=EDGE_LOOP('',(#34675,#34676,#34677,#34678));
#5980=EDGE_LOOP('',(#34679,#34680,#34681,#34682));
#5981=EDGE_LOOP('',(#34683,#34684,#34685,#34686));
#5982=EDGE_LOOP('',(#34687,#34688,#34689,#34690));
#5983=EDGE_LOOP('',(#34691,#34692,#34693,#34694));
#5984=EDGE_LOOP('',(#34695,#34696,#34697,#34698));
#5985=EDGE_LOOP('',(#34699,#34700,#34701,#34702));
#5986=EDGE_LOOP('',(#34703,#34704,#34705,#34706));
#5987=EDGE_LOOP('',(#34707,#34708,#34709,#34710));
#5988=EDGE_LOOP('',(#34711,#34712,#34713,#34714));
#5989=EDGE_LOOP('',(#34715,#34716,#34717,#34718));
#5990=EDGE_LOOP('',(#34719,#34720,#34721,#34722));
#5991=EDGE_LOOP('',(#34723,#34724,#34725,#34726));
#5992=EDGE_LOOP('',(#34727,#34728,#34729,#34730));
#5993=EDGE_LOOP('',(#34731,#34732,#34733,#34734));
#5994=EDGE_LOOP('',(#34735,#34736,#34737,#34738));
#5995=EDGE_LOOP('',(#34739,#34740,#34741,#34742));
#5996=EDGE_LOOP('',(#34743,#34744,#34745,#34746));
#5997=EDGE_LOOP('',(#34747,#34748,#34749,#34750));
#5998=EDGE_LOOP('',(#34751,#34752,#34753,#34754));
#5999=EDGE_LOOP('',(#34755,#34756,#34757,#34758));
#6000=EDGE_LOOP('',(#34759,#34760,#34761,#34762));
#6001=EDGE_LOOP('',(#34763,#34764,#34765,#34766));
#6002=EDGE_LOOP('',(#34767,#34768,#34769,#34770));
#6003=EDGE_LOOP('',(#34771,#34772,#34773,#34774));
#6004=EDGE_LOOP('',(#34775,#34776,#34777,#34778));
#6005=EDGE_LOOP('',(#34779,#34780,#34781,#34782));
#6006=EDGE_LOOP('',(#34783,#34784,#34785,#34786));
#6007=EDGE_LOOP('',(#34787,#34788,#34789,#34790));
#6008=EDGE_LOOP('',(#34791,#34792,#34793,#34794));
#6009=EDGE_LOOP('',(#34795,#34796,#34797,#34798));
#6010=EDGE_LOOP('',(#34799,#34800,#34801,#34802));
#6011=EDGE_LOOP('',(#34803,#34804,#34805,#34806));
#6012=EDGE_LOOP('',(#34807,#34808,#34809,#34810));
#6013=EDGE_LOOP('',(#34811,#34812,#34813,#34814));
#6014=EDGE_LOOP('',(#34815,#34816,#34817,#34818));
#6015=EDGE_LOOP('',(#34819,#34820,#34821,#34822));
#6016=EDGE_LOOP('',(#34823,#34824,#34825,#34826));
#6017=EDGE_LOOP('',(#34827,#34828,#34829,#34830));
#6018=EDGE_LOOP('',(#34831,#34832,#34833,#34834));
#6019=EDGE_LOOP('',(#34835,#34836,#34837,#34838));
#6020=EDGE_LOOP('',(#34839,#34840,#34841,#34842));
#6021=EDGE_LOOP('',(#34843,#34844,#34845,#34846));
#6022=EDGE_LOOP('',(#34847,#34848,#34849,#34850));
#6023=EDGE_LOOP('',(#34851,#34852,#34853,#34854));
#6024=EDGE_LOOP('',(#34855,#34856,#34857,#34858));
#6025=EDGE_LOOP('',(#34859,#34860,#34861,#34862));
#6026=EDGE_LOOP('',(#34863,#34864,#34865,#34866));
#6027=EDGE_LOOP('',(#34867,#34868,#34869,#34870));
#6028=EDGE_LOOP('',(#34871,#34872,#34873,#34874));
#6029=EDGE_LOOP('',(#34875,#34876,#34877,#34878));
#6030=EDGE_LOOP('',(#34879,#34880,#34881,#34882));
#6031=EDGE_LOOP('',(#34883,#34884,#34885,#34886));
#6032=EDGE_LOOP('',(#34887,#34888,#34889,#34890));
#6033=EDGE_LOOP('',(#34891,#34892,#34893,#34894));
#6034=EDGE_LOOP('',(#34895,#34896,#34897,#34898));
#6035=EDGE_LOOP('',(#34899,#34900,#34901,#34902));
#6036=EDGE_LOOP('',(#34903,#34904,#34905,#34906));
#6037=EDGE_LOOP('',(#34907,#34908,#34909,#34910));
#6038=EDGE_LOOP('',(#34911,#34912,#34913,#34914));
#6039=EDGE_LOOP('',(#34915,#34916,#34917,#34918));
#6040=EDGE_LOOP('',(#34919,#34920,#34921,#34922));
#6041=EDGE_LOOP('',(#34923,#34924,#34925,#34926));
#6042=EDGE_LOOP('',(#34927,#34928,#34929,#34930));
#6043=EDGE_LOOP('',(#34931,#34932,#34933,#34934));
#6044=EDGE_LOOP('',(#34935,#34936,#34937,#34938));
#6045=EDGE_LOOP('',(#34939,#34940,#34941,#34942));
#6046=EDGE_LOOP('',(#34943,#34944,#34945,#34946));
#6047=EDGE_LOOP('',(#34947,#34948,#34949,#34950));
#6048=EDGE_LOOP('',(#34951,#34952,#34953,#34954));
#6049=EDGE_LOOP('',(#34955,#34956,#34957,#34958));
#6050=EDGE_LOOP('',(#34959,#34960,#34961,#34962));
#6051=EDGE_LOOP('',(#34963,#34964,#34965,#34966));
#6052=EDGE_LOOP('',(#34967,#34968,#34969,#34970));
#6053=EDGE_LOOP('',(#34971,#34972,#34973,#34974));
#6054=EDGE_LOOP('',(#34975,#34976,#34977,#34978));
#6055=EDGE_LOOP('',(#34979,#34980,#34981,#34982));
#6056=EDGE_LOOP('',(#34983,#34984,#34985,#34986));
#6057=EDGE_LOOP('',(#34987,#34988,#34989,#34990));
#6058=EDGE_LOOP('',(#34991,#34992,#34993,#34994));
#6059=EDGE_LOOP('',(#34995,#34996,#34997,#34998));
#6060=EDGE_LOOP('',(#34999,#35000,#35001,#35002));
#6061=EDGE_LOOP('',(#35003,#35004,#35005,#35006));
#6062=EDGE_LOOP('',(#35007,#35008,#35009,#35010));
#6063=EDGE_LOOP('',(#35011,#35012,#35013,#35014));
#6064=EDGE_LOOP('',(#35015,#35016,#35017,#35018));
#6065=EDGE_LOOP('',(#35019,#35020,#35021,#35022));
#6066=EDGE_LOOP('',(#35023,#35024,#35025,#35026));
#6067=EDGE_LOOP('',(#35027,#35028,#35029,#35030));
#6068=EDGE_LOOP('',(#35031,#35032,#35033,#35034));
#6069=EDGE_LOOP('',(#35035,#35036,#35037,#35038));
#6070=EDGE_LOOP('',(#35039,#35040,#35041,#35042));
#6071=EDGE_LOOP('',(#35043,#35044,#35045,#35046));
#6072=EDGE_LOOP('',(#35047,#35048,#35049,#35050));
#6073=EDGE_LOOP('',(#35051,#35052,#35053,#35054));
#6074=EDGE_LOOP('',(#35055,#35056,#35057,#35058));
#6075=EDGE_LOOP('',(#35059,#35060,#35061,#35062));
#6076=EDGE_LOOP('',(#35063,#35064,#35065,#35066));
#6077=EDGE_LOOP('',(#35067,#35068,#35069,#35070));
#6078=EDGE_LOOP('',(#35071,#35072,#35073,#35074));
#6079=EDGE_LOOP('',(#35075,#35076,#35077,#35078));
#6080=EDGE_LOOP('',(#35079,#35080,#35081,#35082));
#6081=EDGE_LOOP('',(#35083,#35084,#35085,#35086));
#6082=EDGE_LOOP('',(#35087,#35088,#35089,#35090));
#6083=EDGE_LOOP('',(#35091,#35092,#35093,#35094));
#6084=EDGE_LOOP('',(#35095,#35096,#35097,#35098));
#6085=EDGE_LOOP('',(#35099,#35100,#35101,#35102));
#6086=EDGE_LOOP('',(#35103,#35104,#35105,#35106));
#6087=EDGE_LOOP('',(#35107,#35108,#35109,#35110));
#6088=EDGE_LOOP('',(#35111,#35112,#35113,#35114));
#6089=EDGE_LOOP('',(#35115,#35116,#35117,#35118));
#6090=EDGE_LOOP('',(#35119,#35120,#35121,#35122));
#6091=EDGE_LOOP('',(#35123,#35124,#35125,#35126));
#6092=EDGE_LOOP('',(#35127,#35128,#35129,#35130));
#6093=EDGE_LOOP('',(#35131,#35132,#35133,#35134));
#6094=EDGE_LOOP('',(#35135,#35136,#35137,#35138));
#6095=EDGE_LOOP('',(#35139,#35140,#35141,#35142));
#6096=EDGE_LOOP('',(#35143,#35144,#35145,#35146));
#6097=EDGE_LOOP('',(#35147,#35148,#35149,#35150));
#6098=EDGE_LOOP('',(#35151,#35152,#35153,#35154));
#6099=EDGE_LOOP('',(#35155,#35156,#35157,#35158));
#6100=EDGE_LOOP('',(#35159,#35160,#35161,#35162));
#6101=EDGE_LOOP('',(#35163,#35164,#35165,#35166));
#6102=EDGE_LOOP('',(#35167,#35168,#35169,#35170));
#6103=EDGE_LOOP('',(#35171,#35172,#35173,#35174));
#6104=EDGE_LOOP('',(#35175,#35176,#35177,#35178));
#6105=EDGE_LOOP('',(#35179,#35180,#35181,#35182));
#6106=EDGE_LOOP('',(#35183,#35184,#35185,#35186));
#6107=EDGE_LOOP('',(#35187,#35188,#35189,#35190));
#6108=EDGE_LOOP('',(#35191,#35192,#35193,#35194));
#6109=EDGE_LOOP('',(#35195,#35196,#35197,#35198));
#6110=EDGE_LOOP('',(#35199,#35200,#35201,#35202));
#6111=EDGE_LOOP('',(#35203,#35204,#35205,#35206));
#6112=EDGE_LOOP('',(#35207,#35208,#35209,#35210));
#6113=EDGE_LOOP('',(#35211,#35212,#35213,#35214));
#6114=EDGE_LOOP('',(#35215,#35216,#35217,#35218));
#6115=EDGE_LOOP('',(#35219,#35220,#35221,#35222));
#6116=EDGE_LOOP('',(#35223,#35224,#35225,#35226));
#6117=EDGE_LOOP('',(#35227,#35228,#35229,#35230));
#6118=EDGE_LOOP('',(#35231,#35232,#35233,#35234));
#6119=EDGE_LOOP('',(#35235,#35236,#35237,#35238));
#6120=EDGE_LOOP('',(#35239,#35240,#35241,#35242));
#6121=EDGE_LOOP('',(#35243,#35244,#35245,#35246));
#6122=EDGE_LOOP('',(#35247,#35248,#35249,#35250));
#6123=EDGE_LOOP('',(#35251,#35252,#35253,#35254));
#6124=EDGE_LOOP('',(#35255,#35256,#35257,#35258));
#6125=EDGE_LOOP('',(#35259,#35260,#35261,#35262));
#6126=EDGE_LOOP('',(#35263,#35264,#35265,#35266));
#6127=EDGE_LOOP('',(#35267,#35268,#35269,#35270));
#6128=EDGE_LOOP('',(#35271,#35272,#35273,#35274));
#6129=EDGE_LOOP('',(#35275,#35276,#35277,#35278));
#6130=EDGE_LOOP('',(#35279,#35280,#35281,#35282));
#6131=EDGE_LOOP('',(#35283,#35284,#35285,#35286));
#6132=EDGE_LOOP('',(#35287,#35288,#35289,#35290));
#6133=EDGE_LOOP('',(#35291,#35292,#35293,#35294));
#6134=EDGE_LOOP('',(#35295,#35296,#35297,#35298));
#6135=EDGE_LOOP('',(#35299,#35300,#35301,#35302));
#6136=EDGE_LOOP('',(#35303,#35304,#35305,#35306));
#6137=EDGE_LOOP('',(#35307,#35308,#35309,#35310));
#6138=EDGE_LOOP('',(#35311,#35312,#35313,#35314));
#6139=EDGE_LOOP('',(#35315,#35316,#35317,#35318));
#6140=EDGE_LOOP('',(#35319,#35320,#35321,#35322));
#6141=EDGE_LOOP('',(#35323,#35324,#35325,#35326));
#6142=EDGE_LOOP('',(#35327,#35328,#35329,#35330));
#6143=EDGE_LOOP('',(#35331,#35332,#35333,#35334));
#6144=EDGE_LOOP('',(#35335,#35336,#35337,#35338));
#6145=EDGE_LOOP('',(#35339,#35340,#35341,#35342));
#6146=EDGE_LOOP('',(#35343,#35344,#35345,#35346));
#6147=EDGE_LOOP('',(#35347,#35348,#35349,#35350));
#6148=EDGE_LOOP('',(#35351,#35352,#35353,#35354));
#6149=EDGE_LOOP('',(#35355,#35356,#35357,#35358));
#6150=EDGE_LOOP('',(#35359,#35360,#35361,#35362));
#6151=EDGE_LOOP('',(#35363,#35364,#35365,#35366));
#6152=EDGE_LOOP('',(#35367,#35368,#35369,#35370));
#6153=EDGE_LOOP('',(#35371,#35372,#35373,#35374));
#6154=EDGE_LOOP('',(#35375,#35376,#35377,#35378));
#6155=EDGE_LOOP('',(#35379,#35380,#35381,#35382));
#6156=EDGE_LOOP('',(#35383,#35384,#35385,#35386));
#6157=EDGE_LOOP('',(#35387,#35388,#35389,#35390));
#6158=EDGE_LOOP('',(#35391,#35392,#35393,#35394));
#6159=EDGE_LOOP('',(#35395,#35396,#35397,#35398));
#6160=EDGE_LOOP('',(#35399,#35400,#35401,#35402));
#6161=EDGE_LOOP('',(#35403,#35404,#35405,#35406));
#6162=EDGE_LOOP('',(#35407,#35408,#35409,#35410));
#6163=EDGE_LOOP('',(#35411,#35412,#35413,#35414));
#6164=EDGE_LOOP('',(#35415,#35416,#35417,#35418));
#6165=EDGE_LOOP('',(#35419,#35420,#35421,#35422));
#6166=EDGE_LOOP('',(#35423,#35424,#35425,#35426));
#6167=EDGE_LOOP('',(#35427,#35428,#35429,#35430));
#6168=EDGE_LOOP('',(#35431,#35432,#35433,#35434));
#6169=EDGE_LOOP('',(#35435,#35436,#35437,#35438));
#6170=EDGE_LOOP('',(#35439,#35440,#35441,#35442));
#6171=EDGE_LOOP('',(#35443,#35444,#35445,#35446));
#6172=EDGE_LOOP('',(#35447,#35448,#35449,#35450));
#6173=EDGE_LOOP('',(#35451,#35452,#35453,#35454));
#6174=EDGE_LOOP('',(#35455,#35456,#35457,#35458));
#6175=EDGE_LOOP('',(#35459,#35460,#35461,#35462));
#6176=EDGE_LOOP('',(#35463,#35464,#35465,#35466));
#6177=EDGE_LOOP('',(#35467,#35468,#35469,#35470));
#6178=EDGE_LOOP('',(#35471,#35472,#35473,#35474));
#6179=EDGE_LOOP('',(#35475,#35476,#35477,#35478));
#6180=EDGE_LOOP('',(#35479,#35480,#35481,#35482));
#6181=EDGE_LOOP('',(#35483,#35484,#35485,#35486));
#6182=EDGE_LOOP('',(#35487,#35488,#35489,#35490));
#6183=EDGE_LOOP('',(#35491,#35492,#35493,#35494));
#6184=EDGE_LOOP('',(#35495,#35496,#35497,#35498));
#6185=EDGE_LOOP('',(#35499,#35500,#35501,#35502));
#6186=EDGE_LOOP('',(#35503,#35504,#35505,#35506));
#6187=EDGE_LOOP('',(#35507,#35508,#35509,#35510));
#6188=EDGE_LOOP('',(#35511,#35512,#35513,#35514));
#6189=EDGE_LOOP('',(#35515,#35516,#35517,#35518));
#6190=EDGE_LOOP('',(#35519,#35520,#35521,#35522));
#6191=EDGE_LOOP('',(#35523,#35524,#35525,#35526));
#6192=EDGE_LOOP('',(#35527,#35528,#35529,#35530));
#6193=EDGE_LOOP('',(#35531,#35532,#35533,#35534));
#6194=EDGE_LOOP('',(#35535,#35536,#35537,#35538));
#6195=EDGE_LOOP('',(#35539,#35540,#35541,#35542));
#6196=EDGE_LOOP('',(#35543,#35544,#35545,#35546));
#6197=EDGE_LOOP('',(#35547,#35548,#35549,#35550));
#6198=EDGE_LOOP('',(#35551,#35552,#35553,#35554));
#6199=EDGE_LOOP('',(#35555,#35556,#35557,#35558));
#6200=EDGE_LOOP('',(#35559,#35560,#35561,#35562));
#6201=EDGE_LOOP('',(#35563,#35564,#35565,#35566));
#6202=EDGE_LOOP('',(#35567,#35568,#35569,#35570));
#6203=EDGE_LOOP('',(#35571,#35572,#35573,#35574));
#6204=EDGE_LOOP('',(#35575,#35576,#35577,#35578));
#6205=EDGE_LOOP('',(#35579,#35580,#35581,#35582));
#6206=EDGE_LOOP('',(#35583,#35584,#35585,#35586));
#6207=EDGE_LOOP('',(#35587,#35588,#35589,#35590));
#6208=EDGE_LOOP('',(#35591,#35592,#35593,#35594));
#6209=EDGE_LOOP('',(#35595,#35596,#35597,#35598));
#6210=EDGE_LOOP('',(#35599,#35600,#35601,#35602));
#6211=EDGE_LOOP('',(#35603,#35604,#35605,#35606));
#6212=EDGE_LOOP('',(#35607,#35608,#35609,#35610));
#6213=EDGE_LOOP('',(#35611,#35612,#35613,#35614));
#6214=EDGE_LOOP('',(#35615,#35616,#35617,#35618));
#6215=EDGE_LOOP('',(#35619,#35620,#35621,#35622));
#6216=EDGE_LOOP('',(#35623,#35624,#35625,#35626));
#6217=EDGE_LOOP('',(#35627,#35628,#35629,#35630));
#6218=EDGE_LOOP('',(#35631,#35632,#35633,#35634));
#6219=EDGE_LOOP('',(#35635,#35636,#35637,#35638));
#6220=EDGE_LOOP('',(#35639,#35640,#35641,#35642));
#6221=EDGE_LOOP('',(#35643,#35644,#35645,#35646));
#6222=EDGE_LOOP('',(#35647,#35648,#35649,#35650));
#6223=EDGE_LOOP('',(#35651,#35652,#35653,#35654));
#6224=EDGE_LOOP('',(#35655,#35656,#35657,#35658));
#6225=EDGE_LOOP('',(#35659,#35660,#35661,#35662));
#6226=EDGE_LOOP('',(#35663,#35664,#35665,#35666));
#6227=EDGE_LOOP('',(#35667,#35668,#35669,#35670));
#6228=EDGE_LOOP('',(#35671,#35672,#35673,#35674));
#6229=EDGE_LOOP('',(#35675,#35676,#35677,#35678));
#6230=EDGE_LOOP('',(#35679,#35680,#35681,#35682));
#6231=EDGE_LOOP('',(#35683,#35684,#35685,#35686));
#6232=EDGE_LOOP('',(#35687,#35688,#35689,#35690));
#6233=EDGE_LOOP('',(#35691,#35692,#35693,#35694));
#6234=EDGE_LOOP('',(#35695,#35696,#35697,#35698));
#6235=EDGE_LOOP('',(#35699,#35700,#35701,#35702));
#6236=EDGE_LOOP('',(#35703,#35704,#35705,#35706));
#6237=EDGE_LOOP('',(#35707,#35708,#35709,#35710));
#6238=EDGE_LOOP('',(#35711,#35712,#35713,#35714));
#6239=EDGE_LOOP('',(#35715,#35716,#35717,#35718));
#6240=EDGE_LOOP('',(#35719,#35720,#35721,#35722));
#6241=EDGE_LOOP('',(#35723,#35724,#35725,#35726));
#6242=EDGE_LOOP('',(#35727,#35728,#35729,#35730));
#6243=EDGE_LOOP('',(#35731,#35732,#35733,#35734));
#6244=EDGE_LOOP('',(#35735,#35736,#35737,#35738));
#6245=EDGE_LOOP('',(#35739,#35740,#35741,#35742));
#6246=EDGE_LOOP('',(#35743,#35744,#35745,#35746));
#6247=EDGE_LOOP('',(#35747,#35748,#35749,#35750));
#6248=EDGE_LOOP('',(#35751,#35752,#35753,#35754));
#6249=EDGE_LOOP('',(#35755,#35756,#35757,#35758));
#6250=EDGE_LOOP('',(#35759,#35760,#35761,#35762));
#6251=EDGE_LOOP('',(#35763,#35764,#35765,#35766));
#6252=EDGE_LOOP('',(#35767,#35768,#35769,#35770));
#6253=EDGE_LOOP('',(#35771,#35772,#35773,#35774));
#6254=EDGE_LOOP('',(#35775,#35776,#35777,#35778));
#6255=EDGE_LOOP('',(#35779,#35780,#35781,#35782));
#6256=EDGE_LOOP('',(#35783,#35784,#35785,#35786));
#6257=EDGE_LOOP('',(#35787,#35788,#35789,#35790));
#6258=EDGE_LOOP('',(#35791,#35792,#35793,#35794));
#6259=EDGE_LOOP('',(#35795,#35796,#35797,#35798));
#6260=EDGE_LOOP('',(#35799,#35800,#35801,#35802));
#6261=EDGE_LOOP('',(#35803,#35804,#35805,#35806));
#6262=EDGE_LOOP('',(#35807,#35808,#35809,#35810));
#6263=EDGE_LOOP('',(#35811,#35812,#35813,#35814));
#6264=EDGE_LOOP('',(#35815,#35816,#35817,#35818));
#6265=EDGE_LOOP('',(#35819,#35820,#35821,#35822));
#6266=EDGE_LOOP('',(#35823,#35824,#35825,#35826));
#6267=EDGE_LOOP('',(#35827,#35828,#35829,#35830));
#6268=EDGE_LOOP('',(#35831,#35832,#35833,#35834));
#6269=EDGE_LOOP('',(#35835,#35836,#35837,#35838));
#6270=EDGE_LOOP('',(#35839,#35840,#35841,#35842));
#6271=EDGE_LOOP('',(#35843,#35844,#35845,#35846));
#6272=EDGE_LOOP('',(#35847,#35848,#35849,#35850));
#6273=EDGE_LOOP('',(#35851,#35852,#35853,#35854));
#6274=EDGE_LOOP('',(#35855,#35856,#35857,#35858));
#6275=EDGE_LOOP('',(#35859,#35860,#35861,#35862));
#6276=EDGE_LOOP('',(#35863,#35864,#35865,#35866));
#6277=EDGE_LOOP('',(#35867,#35868,#35869,#35870));
#6278=EDGE_LOOP('',(#35871,#35872,#35873,#35874));
#6279=EDGE_LOOP('',(#35875,#35876,#35877,#35878));
#6280=EDGE_LOOP('',(#35879,#35880,#35881,#35882));
#6281=EDGE_LOOP('',(#35883,#35884,#35885,#35886));
#6282=EDGE_LOOP('',(#35887,#35888,#35889,#35890));
#6283=EDGE_LOOP('',(#35891,#35892,#35893,#35894));
#6284=EDGE_LOOP('',(#35895,#35896,#35897,#35898));
#6285=EDGE_LOOP('',(#35899,#35900,#35901,#35902));
#6286=EDGE_LOOP('',(#35903,#35904,#35905,#35906));
#6287=EDGE_LOOP('',(#35907,#35908,#35909,#35910));
#6288=EDGE_LOOP('',(#35911,#35912,#35913,#35914));
#6289=EDGE_LOOP('',(#35915,#35916,#35917,#35918));
#6290=EDGE_LOOP('',(#35919,#35920,#35921,#35922));
#6291=EDGE_LOOP('',(#35923,#35924,#35925,#35926));
#6292=EDGE_LOOP('',(#35927,#35928,#35929,#35930));
#6293=EDGE_LOOP('',(#35931,#35932,#35933,#35934));
#6294=EDGE_LOOP('',(#35935,#35936,#35937,#35938));
#6295=EDGE_LOOP('',(#35939,#35940,#35941,#35942));
#6296=EDGE_LOOP('',(#35943,#35944,#35945,#35946));
#6297=EDGE_LOOP('',(#35947,#35948,#35949,#35950));
#6298=EDGE_LOOP('',(#35951,#35952,#35953,#35954));
#6299=EDGE_LOOP('',(#35955,#35956,#35957,#35958));
#6300=EDGE_LOOP('',(#35959,#35960,#35961,#35962));
#6301=EDGE_LOOP('',(#35963,#35964,#35965,#35966));
#6302=EDGE_LOOP('',(#35967,#35968,#35969,#35970));
#6303=EDGE_LOOP('',(#35971,#35972,#35973,#35974));
#6304=EDGE_LOOP('',(#35975,#35976,#35977,#35978));
#6305=EDGE_LOOP('',(#35979,#35980,#35981,#35982));
#6306=EDGE_LOOP('',(#35983,#35984,#35985,#35986));
#6307=EDGE_LOOP('',(#35987,#35988,#35989,#35990));
#6308=EDGE_LOOP('',(#35991,#35992,#35993,#35994));
#6309=EDGE_LOOP('',(#35995,#35996,#35997,#35998));
#6310=EDGE_LOOP('',(#35999,#36000,#36001,#36002));
#6311=EDGE_LOOP('',(#36003,#36004,#36005,#36006));
#6312=EDGE_LOOP('',(#36007,#36008,#36009,#36010));
#6313=EDGE_LOOP('',(#36011,#36012,#36013,#36014));
#6314=EDGE_LOOP('',(#36015,#36016,#36017,#36018));
#6315=EDGE_LOOP('',(#36019,#36020,#36021,#36022));
#6316=EDGE_LOOP('',(#36023,#36024,#36025,#36026));
#6317=EDGE_LOOP('',(#36027,#36028,#36029,#36030));
#6318=EDGE_LOOP('',(#36031,#36032,#36033,#36034));
#6319=EDGE_LOOP('',(#36035,#36036,#36037,#36038));
#6320=EDGE_LOOP('',(#36039,#36040,#36041,#36042));
#6321=EDGE_LOOP('',(#36043,#36044,#36045,#36046));
#6322=EDGE_LOOP('',(#36047,#36048,#36049,#36050));
#6323=EDGE_LOOP('',(#36051,#36052,#36053,#36054));
#6324=EDGE_LOOP('',(#36055,#36056,#36057,#36058));
#6325=EDGE_LOOP('',(#36059,#36060,#36061,#36062));
#6326=EDGE_LOOP('',(#36063,#36064,#36065,#36066));
#6327=EDGE_LOOP('',(#36067,#36068,#36069,#36070));
#6328=EDGE_LOOP('',(#36071,#36072,#36073,#36074));
#6329=EDGE_LOOP('',(#36075,#36076,#36077,#36078));
#6330=EDGE_LOOP('',(#36079,#36080,#36081,#36082));
#6331=EDGE_LOOP('',(#36083,#36084,#36085,#36086));
#6332=EDGE_LOOP('',(#36087,#36088,#36089,#36090));
#6333=EDGE_LOOP('',(#36091,#36092,#36093,#36094));
#6334=EDGE_LOOP('',(#36095,#36096,#36097,#36098));
#6335=EDGE_LOOP('',(#36099,#36100,#36101,#36102));
#6336=EDGE_LOOP('',(#36103,#36104,#36105,#36106));
#6337=EDGE_LOOP('',(#36107,#36108,#36109,#36110));
#6338=EDGE_LOOP('',(#36111,#36112,#36113,#36114));
#6339=EDGE_LOOP('',(#36115,#36116,#36117,#36118));
#6340=EDGE_LOOP('',(#36119,#36120,#36121,#36122));
#6341=EDGE_LOOP('',(#36123,#36124,#36125,#36126));
#6342=EDGE_LOOP('',(#36127,#36128,#36129,#36130));
#6343=EDGE_LOOP('',(#36131,#36132,#36133,#36134));
#6344=EDGE_LOOP('',(#36135,#36136,#36137,#36138));
#6345=EDGE_LOOP('',(#36139,#36140,#36141,#36142));
#6346=EDGE_LOOP('',(#36143,#36144,#36145,#36146));
#6347=EDGE_LOOP('',(#36147,#36148,#36149,#36150));
#6348=EDGE_LOOP('',(#36151,#36152,#36153,#36154));
#6349=EDGE_LOOP('',(#36155,#36156,#36157,#36158));
#6350=EDGE_LOOP('',(#36159,#36160,#36161,#36162));
#6351=EDGE_LOOP('',(#36163,#36164,#36165,#36166));
#6352=EDGE_LOOP('',(#36167,#36168,#36169,#36170));
#6353=EDGE_LOOP('',(#36171,#36172,#36173,#36174));
#6354=EDGE_LOOP('',(#36175,#36176,#36177,#36178));
#6355=EDGE_LOOP('',(#36179,#36180,#36181,#36182));
#6356=EDGE_LOOP('',(#36183,#36184,#36185,#36186));
#6357=EDGE_LOOP('',(#36187,#36188,#36189,#36190));
#6358=EDGE_LOOP('',(#36191,#36192,#36193,#36194));
#6359=EDGE_LOOP('',(#36195,#36196,#36197,#36198));
#6360=EDGE_LOOP('',(#36199,#36200,#36201,#36202));
#6361=EDGE_LOOP('',(#36203,#36204,#36205,#36206));
#6362=EDGE_LOOP('',(#36207,#36208,#36209,#36210));
#6363=EDGE_LOOP('',(#36211,#36212,#36213,#36214));
#6364=EDGE_LOOP('',(#36215,#36216,#36217,#36218));
#6365=EDGE_LOOP('',(#36219,#36220,#36221,#36222));
#6366=EDGE_LOOP('',(#36223,#36224,#36225,#36226));
#6367=EDGE_LOOP('',(#36227,#36228,#36229,#36230));
#6368=EDGE_LOOP('',(#36231,#36232,#36233,#36234));
#6369=EDGE_LOOP('',(#36235,#36236,#36237,#36238));
#6370=EDGE_LOOP('',(#36239,#36240,#36241,#36242));
#6371=EDGE_LOOP('',(#36243,#36244,#36245,#36246));
#6372=EDGE_LOOP('',(#36247,#36248,#36249,#36250));
#6373=EDGE_LOOP('',(#36251,#36252,#36253,#36254));
#6374=EDGE_LOOP('',(#36255,#36256,#36257,#36258));
#6375=EDGE_LOOP('',(#36259,#36260,#36261,#36262));
#6376=EDGE_LOOP('',(#36263,#36264,#36265,#36266));
#6377=EDGE_LOOP('',(#36267,#36268,#36269,#36270));
#6378=EDGE_LOOP('',(#36271,#36272,#36273,#36274));
#6379=EDGE_LOOP('',(#36275,#36276,#36277,#36278));
#6380=EDGE_LOOP('',(#36279,#36280,#36281,#36282));
#6381=EDGE_LOOP('',(#36283,#36284,#36285,#36286));
#6382=EDGE_LOOP('',(#36287,#36288,#36289,#36290));
#6383=EDGE_LOOP('',(#36291,#36292,#36293,#36294));
#6384=EDGE_LOOP('',(#36295,#36296,#36297,#36298));
#6385=EDGE_LOOP('',(#36299,#36300,#36301,#36302));
#6386=EDGE_LOOP('',(#36303,#36304,#36305,#36306));
#6387=EDGE_LOOP('',(#36307,#36308,#36309,#36310));
#6388=EDGE_LOOP('',(#36311,#36312,#36313,#36314));
#6389=EDGE_LOOP('',(#36315,#36316,#36317,#36318));
#6390=EDGE_LOOP('',(#36319,#36320,#36321,#36322));
#6391=EDGE_LOOP('',(#36323,#36324,#36325,#36326));
#6392=EDGE_LOOP('',(#36327,#36328,#36329,#36330));
#6393=EDGE_LOOP('',(#36331,#36332,#36333,#36334));
#6394=EDGE_LOOP('',(#36335,#36336,#36337,#36338));
#6395=EDGE_LOOP('',(#36339,#36340,#36341,#36342));
#6396=EDGE_LOOP('',(#36343,#36344,#36345,#36346));
#6397=EDGE_LOOP('',(#36347,#36348,#36349,#36350));
#6398=EDGE_LOOP('',(#36351,#36352,#36353,#36354));
#6399=EDGE_LOOP('',(#36355,#36356,#36357,#36358));
#6400=EDGE_LOOP('',(#36359,#36360,#36361,#36362));
#6401=EDGE_LOOP('',(#36363,#36364,#36365,#36366));
#6402=EDGE_LOOP('',(#36367,#36368,#36369,#36370));
#6403=EDGE_LOOP('',(#36371,#36372,#36373,#36374));
#6404=EDGE_LOOP('',(#36375,#36376,#36377,#36378));
#6405=EDGE_LOOP('',(#36379,#36380,#36381,#36382));
#6406=EDGE_LOOP('',(#36383,#36384,#36385,#36386));
#6407=EDGE_LOOP('',(#36387,#36388,#36389,#36390));
#6408=EDGE_LOOP('',(#36391,#36392,#36393,#36394));
#6409=EDGE_LOOP('',(#36395,#36396,#36397,#36398));
#6410=EDGE_LOOP('',(#36399,#36400,#36401,#36402));
#6411=EDGE_LOOP('',(#36403,#36404,#36405,#36406));
#6412=EDGE_LOOP('',(#36407,#36408,#36409,#36410));
#6413=EDGE_LOOP('',(#36411,#36412,#36413,#36414));
#6414=EDGE_LOOP('',(#36415,#36416,#36417,#36418));
#6415=EDGE_LOOP('',(#36419,#36420,#36421,#36422));
#6416=EDGE_LOOP('',(#36423,#36424,#36425,#36426));
#6417=EDGE_LOOP('',(#36427,#36428,#36429,#36430));
#6418=EDGE_LOOP('',(#36431,#36432,#36433,#36434));
#6419=EDGE_LOOP('',(#36435,#36436,#36437,#36438));
#6420=EDGE_LOOP('',(#36439,#36440,#36441,#36442));
#6421=EDGE_LOOP('',(#36443,#36444,#36445,#36446));
#6422=EDGE_LOOP('',(#36447,#36448,#36449,#36450));
#6423=EDGE_LOOP('',(#36451,#36452,#36453,#36454));
#6424=EDGE_LOOP('',(#36455,#36456,#36457,#36458));
#6425=EDGE_LOOP('',(#36459,#36460,#36461,#36462));
#6426=EDGE_LOOP('',(#36463,#36464,#36465,#36466));
#6427=EDGE_LOOP('',(#36467,#36468,#36469,#36470));
#6428=EDGE_LOOP('',(#36471,#36472,#36473,#36474));
#6429=EDGE_LOOP('',(#36475,#36476,#36477,#36478));
#6430=EDGE_LOOP('',(#36479,#36480,#36481,#36482));
#6431=EDGE_LOOP('',(#36483,#36484,#36485,#36486));
#6432=EDGE_LOOP('',(#36487,#36488,#36489,#36490));
#6433=EDGE_LOOP('',(#36491,#36492,#36493,#36494));
#6434=EDGE_LOOP('',(#36495,#36496,#36497,#36498));
#6435=EDGE_LOOP('',(#36499,#36500,#36501,#36502));
#6436=EDGE_LOOP('',(#36503,#36504,#36505,#36506));
#6437=EDGE_LOOP('',(#36507,#36508,#36509,#36510));
#6438=EDGE_LOOP('',(#36511,#36512,#36513,#36514));
#6439=EDGE_LOOP('',(#36515,#36516,#36517,#36518));
#6440=EDGE_LOOP('',(#36519,#36520,#36521,#36522));
#6441=EDGE_LOOP('',(#36523,#36524,#36525,#36526));
#6442=EDGE_LOOP('',(#36527,#36528,#36529,#36530));
#6443=EDGE_LOOP('',(#36531,#36532,#36533,#36534));
#6444=EDGE_LOOP('',(#36535,#36536,#36537,#36538));
#6445=EDGE_LOOP('',(#36539,#36540,#36541,#36542));
#6446=EDGE_LOOP('',(#36543,#36544,#36545,#36546));
#6447=EDGE_LOOP('',(#36547,#36548,#36549,#36550));
#6448=EDGE_LOOP('',(#36551,#36552,#36553,#36554));
#6449=EDGE_LOOP('',(#36555,#36556,#36557,#36558));
#6450=EDGE_LOOP('',(#36559,#36560,#36561,#36562));
#6451=EDGE_LOOP('',(#36563,#36564,#36565,#36566));
#6452=EDGE_LOOP('',(#36567,#36568,#36569,#36570));
#6453=EDGE_LOOP('',(#36571,#36572,#36573,#36574));
#6454=EDGE_LOOP('',(#36575,#36576,#36577,#36578));
#6455=EDGE_LOOP('',(#36579,#36580,#36581,#36582));
#6456=EDGE_LOOP('',(#36583,#36584,#36585,#36586));
#6457=EDGE_LOOP('',(#36587,#36588,#36589,#36590));
#6458=EDGE_LOOP('',(#36591,#36592,#36593,#36594));
#6459=EDGE_LOOP('',(#36595,#36596,#36597,#36598));
#6460=EDGE_LOOP('',(#36599,#36600,#36601,#36602));
#6461=EDGE_LOOP('',(#36603,#36604,#36605,#36606));
#6462=EDGE_LOOP('',(#36607,#36608,#36609,#36610));
#6463=EDGE_LOOP('',(#36611,#36612,#36613,#36614));
#6464=EDGE_LOOP('',(#36615,#36616,#36617,#36618));
#6465=EDGE_LOOP('',(#36619,#36620,#36621,#36622));
#6466=EDGE_LOOP('',(#36623,#36624,#36625,#36626));
#6467=EDGE_LOOP('',(#36627,#36628,#36629,#36630));
#6468=EDGE_LOOP('',(#36631,#36632,#36633,#36634));
#6469=EDGE_LOOP('',(#36635,#36636,#36637,#36638));
#6470=EDGE_LOOP('',(#36639,#36640,#36641,#36642));
#6471=EDGE_LOOP('',(#36643,#36644,#36645,#36646));
#6472=EDGE_LOOP('',(#36647,#36648,#36649,#36650));
#6473=EDGE_LOOP('',(#36651,#36652,#36653,#36654));
#6474=EDGE_LOOP('',(#36655,#36656,#36657,#36658));
#6475=EDGE_LOOP('',(#36659,#36660,#36661,#36662));
#6476=EDGE_LOOP('',(#36663,#36664,#36665,#36666));
#6477=EDGE_LOOP('',(#36667,#36668,#36669,#36670));
#6478=EDGE_LOOP('',(#36671,#36672,#36673,#36674));
#6479=EDGE_LOOP('',(#36675,#36676,#36677,#36678));
#6480=EDGE_LOOP('',(#36679,#36680,#36681,#36682));
#6481=EDGE_LOOP('',(#36683,#36684,#36685,#36686));
#6482=EDGE_LOOP('',(#36687,#36688,#36689,#36690));
#6483=EDGE_LOOP('',(#36691,#36692,#36693,#36694));
#6484=EDGE_LOOP('',(#36695,#36696,#36697,#36698));
#6485=EDGE_LOOP('',(#36699,#36700,#36701,#36702));
#6486=EDGE_LOOP('',(#36703,#36704,#36705,#36706));
#6487=EDGE_LOOP('',(#36707,#36708,#36709,#36710));
#6488=EDGE_LOOP('',(#36711,#36712,#36713,#36714));
#6489=EDGE_LOOP('',(#36715,#36716,#36717,#36718));
#6490=EDGE_LOOP('',(#36719,#36720,#36721,#36722));
#6491=EDGE_LOOP('',(#36723,#36724,#36725,#36726));
#6492=EDGE_LOOP('',(#36727,#36728,#36729,#36730));
#6493=EDGE_LOOP('',(#36731,#36732,#36733,#36734));
#6494=EDGE_LOOP('',(#36735,#36736,#36737,#36738));
#6495=EDGE_LOOP('',(#36739,#36740,#36741,#36742));
#6496=EDGE_LOOP('',(#36743,#36744,#36745,#36746));
#6497=EDGE_LOOP('',(#36747,#36748,#36749,#36750));
#6498=EDGE_LOOP('',(#36751,#36752,#36753,#36754));
#6499=EDGE_LOOP('',(#36755,#36756,#36757,#36758));
#6500=EDGE_LOOP('',(#36759,#36760,#36761,#36762));
#6501=EDGE_LOOP('',(#36763,#36764,#36765,#36766));
#6502=EDGE_LOOP('',(#36767,#36768,#36769,#36770));
#6503=EDGE_LOOP('',(#36771,#36772,#36773,#36774));
#6504=EDGE_LOOP('',(#36775,#36776,#36777,#36778));
#6505=EDGE_LOOP('',(#36779,#36780,#36781,#36782));
#6506=EDGE_LOOP('',(#36783,#36784,#36785,#36786));
#6507=EDGE_LOOP('',(#36787,#36788,#36789,#36790));
#6508=EDGE_LOOP('',(#36791,#36792,#36793,#36794));
#6509=EDGE_LOOP('',(#36795,#36796,#36797,#36798));
#6510=EDGE_LOOP('',(#36799,#36800,#36801,#36802));
#6511=EDGE_LOOP('',(#36803,#36804,#36805,#36806));
#6512=EDGE_LOOP('',(#36807,#36808,#36809,#36810));
#6513=EDGE_LOOP('',(#36811,#36812,#36813,#36814));
#6514=EDGE_LOOP('',(#36815,#36816,#36817,#36818));
#6515=EDGE_LOOP('',(#36819,#36820,#36821,#36822));
#6516=EDGE_LOOP('',(#36823,#36824,#36825,#36826));
#6517=EDGE_LOOP('',(#36827,#36828,#36829,#36830));
#6518=EDGE_LOOP('',(#36831,#36832,#36833,#36834));
#6519=EDGE_LOOP('',(#36835,#36836,#36837,#36838));
#6520=EDGE_LOOP('',(#36839,#36840,#36841,#36842));
#6521=EDGE_LOOP('',(#36843,#36844,#36845,#36846));
#6522=EDGE_LOOP('',(#36847,#36848,#36849,#36850));
#6523=EDGE_LOOP('',(#36851,#36852,#36853,#36854));
#6524=EDGE_LOOP('',(#36855,#36856,#36857,#36858));
#6525=EDGE_LOOP('',(#36859,#36860,#36861,#36862));
#6526=EDGE_LOOP('',(#36863,#36864,#36865,#36866));
#6527=EDGE_LOOP('',(#36867,#36868,#36869,#36870));
#6528=EDGE_LOOP('',(#36871,#36872,#36873,#36874));
#6529=EDGE_LOOP('',(#36875,#36876,#36877,#36878));
#6530=EDGE_LOOP('',(#36879,#36880,#36881,#36882));
#6531=EDGE_LOOP('',(#36883,#36884,#36885,#36886));
#6532=EDGE_LOOP('',(#36887,#36888,#36889,#36890));
#6533=EDGE_LOOP('',(#36891,#36892,#36893,#36894));
#6534=EDGE_LOOP('',(#36895,#36896,#36897,#36898));
#6535=EDGE_LOOP('',(#36899,#36900,#36901,#36902));
#6536=EDGE_LOOP('',(#36903,#36904,#36905,#36906));
#6537=EDGE_LOOP('',(#36907,#36908,#36909,#36910));
#6538=EDGE_LOOP('',(#36911,#36912,#36913,#36914));
#6539=EDGE_LOOP('',(#36915,#36916,#36917,#36918));
#6540=EDGE_LOOP('',(#36919,#36920,#36921,#36922));
#6541=EDGE_LOOP('',(#36923,#36924,#36925,#36926));
#6542=EDGE_LOOP('',(#36927,#36928,#36929,#36930));
#6543=EDGE_LOOP('',(#36931,#36932,#36933,#36934));
#6544=EDGE_LOOP('',(#36935,#36936,#36937,#36938));
#6545=EDGE_LOOP('',(#36939,#36940,#36941,#36942));
#6546=EDGE_LOOP('',(#36943,#36944,#36945,#36946));
#6547=EDGE_LOOP('',(#36947,#36948,#36949,#36950));
#6548=EDGE_LOOP('',(#36951,#36952,#36953,#36954));
#6549=EDGE_LOOP('',(#36955,#36956,#36957,#36958));
#6550=EDGE_LOOP('',(#36959,#36960,#36961,#36962));
#6551=EDGE_LOOP('',(#36963,#36964,#36965,#36966));
#6552=EDGE_LOOP('',(#36967,#36968,#36969,#36970));
#6553=EDGE_LOOP('',(#36971,#36972,#36973,#36974));
#6554=EDGE_LOOP('',(#36975,#36976,#36977,#36978));
#6555=EDGE_LOOP('',(#36979,#36980,#36981,#36982));
#6556=EDGE_LOOP('',(#36983,#36984,#36985,#36986));
#6557=EDGE_LOOP('',(#36987,#36988,#36989,#36990));
#6558=EDGE_LOOP('',(#36991,#36992,#36993,#36994));
#6559=EDGE_LOOP('',(#36995,#36996,#36997,#36998));
#6560=EDGE_LOOP('',(#36999,#37000,#37001,#37002));
#6561=EDGE_LOOP('',(#37003,#37004,#37005,#37006));
#6562=EDGE_LOOP('',(#37007,#37008,#37009,#37010));
#6563=EDGE_LOOP('',(#37011,#37012,#37013,#37014));
#6564=EDGE_LOOP('',(#37015,#37016,#37017,#37018));
#6565=EDGE_LOOP('',(#37019,#37020,#37021,#37022));
#6566=EDGE_LOOP('',(#37023,#37024,#37025,#37026));
#6567=EDGE_LOOP('',(#37027,#37028,#37029,#37030));
#6568=EDGE_LOOP('',(#37031,#37032,#37033,#37034));
#6569=EDGE_LOOP('',(#37035,#37036,#37037,#37038));
#6570=EDGE_LOOP('',(#37039,#37040,#37041,#37042));
#6571=EDGE_LOOP('',(#37043,#37044,#37045,#37046));
#6572=EDGE_LOOP('',(#37047,#37048,#37049,#37050));
#6573=EDGE_LOOP('',(#37051,#37052,#37053,#37054));
#6574=EDGE_LOOP('',(#37055,#37056,#37057,#37058));
#6575=EDGE_LOOP('',(#37059,#37060,#37061,#37062));
#6576=EDGE_LOOP('',(#37063,#37064,#37065,#37066));
#6577=EDGE_LOOP('',(#37067,#37068,#37069,#37070));
#6578=EDGE_LOOP('',(#37071,#37072,#37073,#37074));
#6579=EDGE_LOOP('',(#37075,#37076,#37077,#37078));
#6580=EDGE_LOOP('',(#37079,#37080,#37081,#37082));
#6581=EDGE_LOOP('',(#37083,#37084,#37085,#37086));
#6582=EDGE_LOOP('',(#37087,#37088,#37089,#37090));
#6583=EDGE_LOOP('',(#37091,#37092,#37093,#37094));
#6584=EDGE_LOOP('',(#37095,#37096,#37097,#37098));
#6585=EDGE_LOOP('',(#37099,#37100,#37101,#37102));
#6586=EDGE_LOOP('',(#37103,#37104,#37105,#37106));
#6587=EDGE_LOOP('',(#37107,#37108,#37109,#37110));
#6588=EDGE_LOOP('',(#37111,#37112,#37113,#37114));
#6589=EDGE_LOOP('',(#37115,#37116,#37117,#37118));
#6590=EDGE_LOOP('',(#37119,#37120,#37121,#37122));
#6591=EDGE_LOOP('',(#37123,#37124,#37125,#37126));
#6592=EDGE_LOOP('',(#37127,#37128,#37129,#37130));
#6593=EDGE_LOOP('',(#37131,#37132,#37133,#37134));
#6594=EDGE_LOOP('',(#37135,#37136,#37137,#37138));
#6595=EDGE_LOOP('',(#37139,#37140,#37141,#37142));
#6596=EDGE_LOOP('',(#37143,#37144,#37145,#37146));
#6597=EDGE_LOOP('',(#37147,#37148,#37149,#37150));
#6598=EDGE_LOOP('',(#37151,#37152,#37153,#37154));
#6599=EDGE_LOOP('',(#37155,#37156,#37157,#37158));
#6600=EDGE_LOOP('',(#37159,#37160,#37161,#37162));
#6601=EDGE_LOOP('',(#37163,#37164,#37165,#37166));
#6602=EDGE_LOOP('',(#37167,#37168,#37169,#37170));
#6603=EDGE_LOOP('',(#37171,#37172,#37173,#37174));
#6604=EDGE_LOOP('',(#37175,#37176,#37177,#37178));
#6605=EDGE_LOOP('',(#37179,#37180,#37181,#37182));
#6606=EDGE_LOOP('',(#37183,#37184,#37185,#37186));
#6607=EDGE_LOOP('',(#37187,#37188,#37189,#37190));
#6608=EDGE_LOOP('',(#37191,#37192,#37193,#37194));
#6609=EDGE_LOOP('',(#37195,#37196,#37197,#37198));
#6610=EDGE_LOOP('',(#37199,#37200,#37201,#37202));
#6611=EDGE_LOOP('',(#37203,#37204,#37205,#37206));
#6612=EDGE_LOOP('',(#37207,#37208,#37209,#37210));
#6613=EDGE_LOOP('',(#37211,#37212,#37213,#37214));
#6614=EDGE_LOOP('',(#37215,#37216,#37217,#37218));
#6615=EDGE_LOOP('',(#37219,#37220,#37221,#37222));
#6616=EDGE_LOOP('',(#37223,#37224,#37225,#37226));
#6617=EDGE_LOOP('',(#37227,#37228,#37229,#37230));
#6618=EDGE_LOOP('',(#37231,#37232,#37233,#37234));
#6619=EDGE_LOOP('',(#37235,#37236,#37237,#37238));
#6620=EDGE_LOOP('',(#37239,#37240,#37241,#37242));
#6621=EDGE_LOOP('',(#37243,#37244,#37245,#37246));
#6622=EDGE_LOOP('',(#37247,#37248,#37249,#37250));
#6623=EDGE_LOOP('',(#37251,#37252,#37253,#37254));
#6624=EDGE_LOOP('',(#37255,#37256,#37257,#37258));
#6625=EDGE_LOOP('',(#37259,#37260,#37261,#37262));
#6626=EDGE_LOOP('',(#37263,#37264,#37265,#37266));
#6627=EDGE_LOOP('',(#37267,#37268,#37269,#37270));
#6628=EDGE_LOOP('',(#37271,#37272,#37273,#37274));
#6629=EDGE_LOOP('',(#37275,#37276,#37277,#37278));
#6630=EDGE_LOOP('',(#37279,#37280,#37281,#37282));
#6631=EDGE_LOOP('',(#37283,#37284,#37285,#37286));
#6632=EDGE_LOOP('',(#37287,#37288,#37289,#37290));
#6633=EDGE_LOOP('',(#37291,#37292,#37293,#37294));
#6634=EDGE_LOOP('',(#37295,#37296,#37297,#37298));
#6635=EDGE_LOOP('',(#37299,#37300,#37301,#37302));
#6636=EDGE_LOOP('',(#37303,#37304,#37305,#37306));
#6637=EDGE_LOOP('',(#37307,#37308,#37309,#37310));
#6638=EDGE_LOOP('',(#37311,#37312,#37313,#37314));
#6639=EDGE_LOOP('',(#37315,#37316,#37317,#37318));
#6640=EDGE_LOOP('',(#37319,#37320,#37321,#37322));
#6641=EDGE_LOOP('',(#37323,#37324,#37325,#37326));
#6642=EDGE_LOOP('',(#37327,#37328,#37329,#37330));
#6643=EDGE_LOOP('',(#37331,#37332,#37333,#37334));
#6644=EDGE_LOOP('',(#37335,#37336,#37337,#37338));
#6645=EDGE_LOOP('',(#37339,#37340,#37341,#37342));
#6646=EDGE_LOOP('',(#37343,#37344,#37345,#37346));
#6647=EDGE_LOOP('',(#37347,#37348,#37349,#37350));
#6648=EDGE_LOOP('',(#37351,#37352,#37353,#37354));
#6649=EDGE_LOOP('',(#37355,#37356,#37357,#37358));
#6650=EDGE_LOOP('',(#37359,#37360,#37361,#37362));
#6651=EDGE_LOOP('',(#37363,#37364,#37365,#37366));
#6652=EDGE_LOOP('',(#37367,#37368,#37369,#37370));
#6653=EDGE_LOOP('',(#37371,#37372,#37373,#37374));
#6654=EDGE_LOOP('',(#37375,#37376,#37377,#37378));
#6655=EDGE_LOOP('',(#37379,#37380,#37381,#37382));
#6656=EDGE_LOOP('',(#37383,#37384,#37385,#37386));
#6657=EDGE_LOOP('',(#37387,#37388,#37389,#37390));
#6658=EDGE_LOOP('',(#37391,#37392,#37393,#37394));
#6659=EDGE_LOOP('',(#37395,#37396,#37397,#37398));
#6660=EDGE_LOOP('',(#37399,#37400,#37401,#37402));
#6661=EDGE_LOOP('',(#37403,#37404,#37405,#37406));
#6662=EDGE_LOOP('',(#37407,#37408,#37409,#37410));
#6663=EDGE_LOOP('',(#37411,#37412,#37413,#37414));
#6664=EDGE_LOOP('',(#37415,#37416,#37417,#37418));
#6665=EDGE_LOOP('',(#37419,#37420,#37421,#37422));
#6666=EDGE_LOOP('',(#37423,#37424,#37425,#37426));
#6667=EDGE_LOOP('',(#37427,#37428,#37429,#37430));
#6668=EDGE_LOOP('',(#37431,#37432,#37433,#37434));
#6669=EDGE_LOOP('',(#37435,#37436,#37437,#37438));
#6670=EDGE_LOOP('',(#37439,#37440,#37441,#37442));
#6671=EDGE_LOOP('',(#37443,#37444,#37445,#37446));
#6672=EDGE_LOOP('',(#37447,#37448,#37449,#37450));
#6673=EDGE_LOOP('',(#37451,#37452,#37453,#37454));
#6674=EDGE_LOOP('',(#37455,#37456,#37457,#37458));
#6675=EDGE_LOOP('',(#37459,#37460,#37461,#37462));
#6676=EDGE_LOOP('',(#37463,#37464,#37465,#37466));
#6677=EDGE_LOOP('',(#37467,#37468,#37469,#37470));
#6678=EDGE_LOOP('',(#37471,#37472,#37473,#37474));
#6679=EDGE_LOOP('',(#37475,#37476,#37477,#37478));
#6680=EDGE_LOOP('',(#37479,#37480,#37481,#37482));
#6681=EDGE_LOOP('',(#37483,#37484,#37485,#37486));
#6682=EDGE_LOOP('',(#37487,#37488,#37489,#37490));
#6683=EDGE_LOOP('',(#37491,#37492,#37493,#37494));
#6684=EDGE_LOOP('',(#37495,#37496,#37497,#37498));
#6685=EDGE_LOOP('',(#37499,#37500,#37501,#37502));
#6686=EDGE_LOOP('',(#37503,#37504,#37505,#37506));
#6687=EDGE_LOOP('',(#37507,#37508,#37509,#37510));
#6688=EDGE_LOOP('',(#37511,#37512,#37513,#37514));
#6689=EDGE_LOOP('',(#37515,#37516,#37517,#37518));
#6690=EDGE_LOOP('',(#37519,#37520,#37521,#37522));
#6691=EDGE_LOOP('',(#37523,#37524,#37525,#37526));
#6692=EDGE_LOOP('',(#37527,#37528,#37529,#37530));
#6693=EDGE_LOOP('',(#37531,#37532,#37533,#37534));
#6694=EDGE_LOOP('',(#37535,#37536,#37537,#37538));
#6695=EDGE_LOOP('',(#37539,#37540,#37541,#37542));
#6696=EDGE_LOOP('',(#37543,#37544,#37545,#37546));
#6697=EDGE_LOOP('',(#37547,#37548,#37549,#37550));
#6698=EDGE_LOOP('',(#37551,#37552,#37553,#37554));
#6699=EDGE_LOOP('',(#37555,#37556,#37557,#37558));
#6700=EDGE_LOOP('',(#37559,#37560,#37561,#37562));
#6701=EDGE_LOOP('',(#37563,#37564,#37565,#37566));
#6702=EDGE_LOOP('',(#37567,#37568,#37569,#37570));
#6703=EDGE_LOOP('',(#37571,#37572,#37573,#37574));
#6704=EDGE_LOOP('',(#37575,#37576,#37577,#37578));
#6705=EDGE_LOOP('',(#37579,#37580,#37581,#37582));
#6706=EDGE_LOOP('',(#37583,#37584,#37585,#37586));
#6707=EDGE_LOOP('',(#37587,#37588,#37589,#37590));
#6708=EDGE_LOOP('',(#37591,#37592,#37593,#37594));
#6709=EDGE_LOOP('',(#37595,#37596,#37597,#37598));
#6710=EDGE_LOOP('',(#37599,#37600,#37601,#37602));
#6711=EDGE_LOOP('',(#37603,#37604,#37605,#37606));
#6712=EDGE_LOOP('',(#37607,#37608,#37609,#37610));
#6713=EDGE_LOOP('',(#37611,#37612,#37613,#37614));
#6714=EDGE_LOOP('',(#37615,#37616,#37617,#37618));
#6715=EDGE_LOOP('',(#37619,#37620,#37621,#37622));
#6716=EDGE_LOOP('',(#37623,#37624,#37625,#37626));
#6717=EDGE_LOOP('',(#37627,#37628,#37629,#37630));
#6718=EDGE_LOOP('',(#37631,#37632,#37633,#37634));
#6719=EDGE_LOOP('',(#37635,#37636,#37637,#37638));
#6720=EDGE_LOOP('',(#37639,#37640,#37641,#37642));
#6721=EDGE_LOOP('',(#37643,#37644,#37645,#37646));
#6722=EDGE_LOOP('',(#37647,#37648,#37649,#37650));
#6723=EDGE_LOOP('',(#37651,#37652,#37653,#37654));
#6724=EDGE_LOOP('',(#37655,#37656,#37657,#37658));
#6725=EDGE_LOOP('',(#37659,#37660,#37661,#37662));
#6726=EDGE_LOOP('',(#37663,#37664,#37665,#37666));
#6727=EDGE_LOOP('',(#37667,#37668,#37669,#37670));
#6728=EDGE_LOOP('',(#37671,#37672,#37673,#37674));
#6729=EDGE_LOOP('',(#37675,#37676,#37677,#37678));
#6730=EDGE_LOOP('',(#37679,#37680,#37681,#37682));
#6731=EDGE_LOOP('',(#37683,#37684,#37685,#37686));
#6732=EDGE_LOOP('',(#37687,#37688,#37689,#37690));
#6733=EDGE_LOOP('',(#37691,#37692,#37693,#37694));
#6734=EDGE_LOOP('',(#37695,#37696,#37697,#37698));
#6735=EDGE_LOOP('',(#37699,#37700,#37701,#37702));
#6736=EDGE_LOOP('',(#37703,#37704,#37705,#37706));
#6737=EDGE_LOOP('',(#37707,#37708,#37709,#37710));
#6738=EDGE_LOOP('',(#37711,#37712,#37713,#37714));
#6739=EDGE_LOOP('',(#37715,#37716,#37717,#37718));
#8179=LINE('',#58372,#13054);
#8180=LINE('',#58374,#13055);
#8181=LINE('',#58376,#13056);
#8182=LINE('',#58378,#13057);
#8183=LINE('',#58380,#13058);
#8184=LINE('',#58382,#13059);
#8185=LINE('',#58384,#13060);
#8186=LINE('',#58386,#13061);
#8187=LINE('',#58388,#13062);
#8188=LINE('',#58390,#13063);
#8189=LINE('',#58392,#13064);
#8190=LINE('',#58393,#13065);
#8191=LINE('',#58397,#13066);
#8192=LINE('',#58399,#13067);
#8193=LINE('',#58401,#13068);
#8194=LINE('',#58403,#13069);
#8195=LINE('',#58405,#13070);
#8196=LINE('',#58407,#13071);
#8197=LINE('',#58409,#13072);
#8198=LINE('',#58411,#13073);
#8199=LINE('',#58413,#13074);
#8200=LINE('',#58415,#13075);
#8201=LINE('',#58417,#13076);
#8202=LINE('',#58418,#13077);
#8203=LINE('',#58420,#13078);
#8204=LINE('',#58421,#13079);
#8205=LINE('',#58423,#13080);
#8206=LINE('',#58424,#13081);
#8207=LINE('',#58426,#13082);
#8208=LINE('',#58427,#13083);
#8209=LINE('',#58429,#13084);
#8210=LINE('',#58430,#13085);
#8211=LINE('',#58433,#13086);
#8212=LINE('',#58434,#13087);
#8213=LINE('',#58436,#13088);
#8214=LINE('',#58438,#13089);
#8215=LINE('',#58442,#13090);
#8216=LINE('',#58449,#13091);
#8217=LINE('',#58452,#13092);
#8218=LINE('',#58454,#13093);
#8219=LINE('',#58459,#13094);
#8220=LINE('',#58464,#13095);
#8221=LINE('',#58468,#13096);
#8222=LINE('',#58470,#13097);
#8223=LINE('',#58476,#13098);
#8224=LINE('',#58479,#13099);
#8225=LINE('',#58483,#13100);
#8226=LINE('',#58485,#13101);
#8227=LINE('',#58487,#13102);
#8228=LINE('',#58488,#13103);
#8229=LINE('',#58494,#13104);
#8230=LINE('',#58497,#13105);
#8231=LINE('',#58499,#13106);
#8232=LINE('',#58500,#13107);
#8233=LINE('',#58502,#13108);
#8234=LINE('',#58503,#13109);
#8235=LINE('',#58504,#13110);
#8236=LINE('',#58505,#13111);
#8237=LINE('',#58507,#13112);
#8238=LINE('',#58509,#13113);
#8239=LINE('',#58510,#13114);
#8240=LINE('',#58511,#13115);
#8241=LINE('',#58518,#13116);
#8242=LINE('',#58525,#13117);
#8243=LINE('',#58528,#13118);
#8244=LINE('',#58530,#13119);
#8245=LINE('',#58535,#13120);
#8246=LINE('',#58540,#13121);
#8247=LINE('',#58544,#13122);
#8248=LINE('',#58546,#13123);
#8249=LINE('',#58552,#13124);
#8250=LINE('',#58555,#13125);
#8251=LINE('',#58559,#13126);
#8252=LINE('',#58561,#13127);
#8253=LINE('',#58563,#13128);
#8254=LINE('',#58564,#13129);
#8255=LINE('',#58570,#13130);
#8256=LINE('',#58573,#13131);
#8257=LINE('',#58575,#13132);
#8258=LINE('',#58576,#13133);
#8259=LINE('',#58578,#13134);
#8260=LINE('',#58579,#13135);
#8261=LINE('',#58580,#13136);
#8262=LINE('',#58581,#13137);
#8263=LINE('',#58583,#13138);
#8264=LINE('',#58585,#13139);
#8265=LINE('',#58586,#13140);
#8266=LINE('',#58587,#13141);
#8267=LINE('',#58594,#13142);
#8268=LINE('',#58596,#13143);
#8269=LINE('',#58598,#13144);
#8270=LINE('',#58600,#13145);
#8271=LINE('',#58602,#13146);
#8272=LINE('',#58603,#13147);
#8273=LINE('',#58606,#13148);
#8274=LINE('',#58608,#13149);
#8275=LINE('',#58610,#13150);
#8276=LINE('',#58612,#13151);
#8277=LINE('',#58614,#13152);
#8278=LINE('',#58615,#13153);
#8279=LINE('',#58618,#13154);
#8280=LINE('',#58620,#13155);
#8281=LINE('',#58622,#13156);
#8282=LINE('',#58624,#13157);
#8283=LINE('',#58626,#13158);
#8284=LINE('',#58627,#13159);
#8285=LINE('',#58630,#13160);
#8286=LINE('',#58632,#13161);
#8287=LINE('',#58634,#13162);
#8288=LINE('',#58636,#13163);
#8289=LINE('',#58638,#13164);
#8290=LINE('',#58639,#13165);
#8291=LINE('',#58642,#13166);
#8292=LINE('',#58644,#13167);
#8293=LINE('',#58646,#13168);
#8294=LINE('',#58648,#13169);
#8295=LINE('',#58650,#13170);
#8296=LINE('',#58651,#13171);
#8297=LINE('',#58654,#13172);
#8298=LINE('',#58656,#13173);
#8299=LINE('',#58658,#13174);
#8300=LINE('',#58660,#13175);
#8301=LINE('',#58662,#13176);
#8302=LINE('',#58663,#13177);
#8303=LINE('',#58666,#13178);
#8304=LINE('',#58668,#13179);
#8305=LINE('',#58670,#13180);
#8306=LINE('',#58672,#13181);
#8307=LINE('',#58674,#13182);
#8308=LINE('',#58675,#13183);
#8309=LINE('',#58678,#13184);
#8310=LINE('',#58680,#13185);
#8311=LINE('',#58682,#13186);
#8312=LINE('',#58684,#13187);
#8313=LINE('',#58686,#13188);
#8314=LINE('',#58687,#13189);
#8315=LINE('',#58690,#13190);
#8316=LINE('',#58692,#13191);
#8317=LINE('',#58694,#13192);
#8318=LINE('',#58696,#13193);
#8319=LINE('',#58698,#13194);
#8320=LINE('',#58699,#13195);
#8321=LINE('',#58702,#13196);
#8322=LINE('',#58704,#13197);
#8323=LINE('',#58706,#13198);
#8324=LINE('',#58708,#13199);
#8325=LINE('',#58710,#13200);
#8326=LINE('',#58711,#13201);
#8327=LINE('',#58714,#13202);
#8328=LINE('',#58716,#13203);
#8329=LINE('',#58718,#13204);
#8330=LINE('',#58720,#13205);
#8331=LINE('',#58722,#13206);
#8332=LINE('',#58723,#13207);
#8333=LINE('',#58726,#13208);
#8334=LINE('',#58728,#13209);
#8335=LINE('',#58730,#13210);
#8336=LINE('',#58732,#13211);
#8337=LINE('',#58734,#13212);
#8338=LINE('',#58735,#13213);
#8339=LINE('',#58738,#13214);
#8340=LINE('',#58740,#13215);
#8341=LINE('',#58742,#13216);
#8342=LINE('',#58744,#13217);
#8343=LINE('',#58746,#13218);
#8344=LINE('',#58747,#13219);
#8345=LINE('',#58750,#13220);
#8346=LINE('',#58752,#13221);
#8347=LINE('',#58754,#13222);
#8348=LINE('',#58756,#13223);
#8349=LINE('',#58758,#13224);
#8350=LINE('',#58759,#13225);
#8351=LINE('',#58762,#13226);
#8352=LINE('',#58764,#13227);
#8353=LINE('',#58766,#13228);
#8354=LINE('',#58768,#13229);
#8355=LINE('',#58770,#13230);
#8356=LINE('',#58771,#13231);
#8357=LINE('',#58774,#13232);
#8358=LINE('',#58776,#13233);
#8359=LINE('',#58778,#13234);
#8360=LINE('',#58780,#13235);
#8361=LINE('',#58782,#13236);
#8362=LINE('',#58783,#13237);
#8363=LINE('',#58786,#13238);
#8364=LINE('',#58788,#13239);
#8365=LINE('',#58790,#13240);
#8366=LINE('',#58792,#13241);
#8367=LINE('',#58794,#13242);
#8368=LINE('',#58795,#13243);
#8369=LINE('',#58798,#13244);
#8370=LINE('',#58800,#13245);
#8371=LINE('',#58802,#13246);
#8372=LINE('',#58804,#13247);
#8373=LINE('',#58806,#13248);
#8374=LINE('',#58807,#13249);
#8375=LINE('',#58810,#13250);
#8376=LINE('',#58812,#13251);
#8377=LINE('',#58814,#13252);
#8378=LINE('',#58816,#13253);
#8379=LINE('',#58818,#13254);
#8380=LINE('',#58819,#13255);
#8381=LINE('',#58822,#13256);
#8382=LINE('',#58824,#13257);
#8383=LINE('',#58826,#13258);
#8384=LINE('',#58828,#13259);
#8385=LINE('',#58830,#13260);
#8386=LINE('',#58831,#13261);
#8387=LINE('',#58834,#13262);
#8388=LINE('',#58836,#13263);
#8389=LINE('',#58838,#13264);
#8390=LINE('',#58840,#13265);
#8391=LINE('',#58842,#13266);
#8392=LINE('',#58843,#13267);
#8393=LINE('',#58846,#13268);
#8394=LINE('',#58848,#13269);
#8395=LINE('',#58850,#13270);
#8396=LINE('',#58852,#13271);
#8397=LINE('',#58854,#13272);
#8398=LINE('',#58855,#13273);
#8399=LINE('',#58858,#13274);
#8400=LINE('',#58860,#13275);
#8401=LINE('',#58862,#13276);
#8402=LINE('',#58864,#13277);
#8403=LINE('',#58866,#13278);
#8404=LINE('',#58867,#13279);
#8405=LINE('',#58870,#13280);
#8406=LINE('',#58872,#13281);
#8407=LINE('',#58874,#13282);
#8408=LINE('',#58876,#13283);
#8409=LINE('',#58878,#13284);
#8410=LINE('',#58879,#13285);
#8411=LINE('',#58882,#13286);
#8412=LINE('',#58884,#13287);
#8413=LINE('',#58886,#13288);
#8414=LINE('',#58888,#13289);
#8415=LINE('',#58890,#13290);
#8416=LINE('',#58891,#13291);
#8417=LINE('',#58894,#13292);
#8418=LINE('',#58896,#13293);
#8419=LINE('',#58898,#13294);
#8420=LINE('',#58900,#13295);
#8421=LINE('',#58902,#13296);
#8422=LINE('',#58903,#13297);
#8423=LINE('',#58906,#13298);
#8424=LINE('',#58908,#13299);
#8425=LINE('',#58910,#13300);
#8426=LINE('',#58912,#13301);
#8427=LINE('',#58914,#13302);
#8428=LINE('',#58915,#13303);
#8429=LINE('',#58918,#13304);
#8430=LINE('',#58920,#13305);
#8431=LINE('',#58922,#13306);
#8432=LINE('',#58924,#13307);
#8433=LINE('',#58926,#13308);
#8434=LINE('',#58927,#13309);
#8435=LINE('',#58930,#13310);
#8436=LINE('',#58932,#13311);
#8437=LINE('',#58934,#13312);
#8438=LINE('',#58936,#13313);
#8439=LINE('',#58938,#13314);
#8440=LINE('',#58939,#13315);
#8441=LINE('',#58942,#13316);
#8442=LINE('',#58944,#13317);
#8443=LINE('',#58946,#13318);
#8444=LINE('',#58948,#13319);
#8445=LINE('',#58950,#13320);
#8446=LINE('',#58951,#13321);
#8447=LINE('',#58954,#13322);
#8448=LINE('',#58956,#13323);
#8449=LINE('',#58958,#13324);
#8450=LINE('',#58960,#13325);
#8451=LINE('',#58962,#13326);
#8452=LINE('',#58963,#13327);
#8453=LINE('',#58966,#13328);
#8454=LINE('',#58968,#13329);
#8455=LINE('',#58970,#13330);
#8456=LINE('',#58972,#13331);
#8457=LINE('',#58974,#13332);
#8458=LINE('',#58975,#13333);
#8459=LINE('',#58978,#13334);
#8460=LINE('',#58980,#13335);
#8461=LINE('',#58982,#13336);
#8462=LINE('',#58984,#13337);
#8463=LINE('',#58986,#13338);
#8464=LINE('',#58987,#13339);
#8465=LINE('',#58990,#13340);
#8466=LINE('',#58992,#13341);
#8467=LINE('',#58994,#13342);
#8468=LINE('',#58996,#13343);
#8469=LINE('',#58998,#13344);
#8470=LINE('',#58999,#13345);
#8471=LINE('',#59002,#13346);
#8472=LINE('',#59004,#13347);
#8473=LINE('',#59006,#13348);
#8474=LINE('',#59008,#13349);
#8475=LINE('',#59010,#13350);
#8476=LINE('',#59011,#13351);
#8477=LINE('',#59014,#13352);
#8478=LINE('',#59016,#13353);
#8479=LINE('',#59018,#13354);
#8480=LINE('',#59020,#13355);
#8481=LINE('',#59022,#13356);
#8482=LINE('',#59023,#13357);
#8483=LINE('',#59026,#13358);
#8484=LINE('',#59028,#13359);
#8485=LINE('',#59030,#13360);
#8486=LINE('',#59032,#13361);
#8487=LINE('',#59034,#13362);
#8488=LINE('',#59035,#13363);
#8489=LINE('',#59038,#13364);
#8490=LINE('',#59040,#13365);
#8491=LINE('',#59042,#13366);
#8492=LINE('',#59044,#13367);
#8493=LINE('',#59046,#13368);
#8494=LINE('',#59047,#13369);
#8495=LINE('',#59050,#13370);
#8496=LINE('',#59052,#13371);
#8497=LINE('',#59054,#13372);
#8498=LINE('',#59056,#13373);
#8499=LINE('',#59058,#13374);
#8500=LINE('',#59059,#13375);
#8501=LINE('',#59062,#13376);
#8502=LINE('',#59064,#13377);
#8503=LINE('',#59066,#13378);
#8504=LINE('',#59068,#13379);
#8505=LINE('',#59070,#13380);
#8506=LINE('',#59071,#13381);
#8507=LINE('',#59074,#13382);
#8508=LINE('',#59076,#13383);
#8509=LINE('',#59078,#13384);
#8510=LINE('',#59080,#13385);
#8511=LINE('',#59082,#13386);
#8512=LINE('',#59083,#13387);
#8513=LINE('',#59086,#13388);
#8514=LINE('',#59088,#13389);
#8515=LINE('',#59090,#13390);
#8516=LINE('',#59092,#13391);
#8517=LINE('',#59094,#13392);
#8518=LINE('',#59095,#13393);
#8519=LINE('',#59098,#13394);
#8520=LINE('',#59100,#13395);
#8521=LINE('',#59102,#13396);
#8522=LINE('',#59104,#13397);
#8523=LINE('',#59106,#13398);
#8524=LINE('',#59107,#13399);
#8525=LINE('',#59110,#13400);
#8526=LINE('',#59112,#13401);
#8527=LINE('',#59114,#13402);
#8528=LINE('',#59116,#13403);
#8529=LINE('',#59118,#13404);
#8530=LINE('',#59119,#13405);
#8531=LINE('',#59122,#13406);
#8532=LINE('',#59124,#13407);
#8533=LINE('',#59126,#13408);
#8534=LINE('',#59128,#13409);
#8535=LINE('',#59130,#13410);
#8536=LINE('',#59131,#13411);
#8537=LINE('',#59134,#13412);
#8538=LINE('',#59136,#13413);
#8539=LINE('',#59138,#13414);
#8540=LINE('',#59140,#13415);
#8541=LINE('',#59142,#13416);
#8542=LINE('',#59143,#13417);
#8543=LINE('',#59146,#13418);
#8544=LINE('',#59148,#13419);
#8545=LINE('',#59150,#13420);
#8546=LINE('',#59152,#13421);
#8547=LINE('',#59154,#13422);
#8548=LINE('',#59155,#13423);
#8549=LINE('',#59158,#13424);
#8550=LINE('',#59160,#13425);
#8551=LINE('',#59162,#13426);
#8552=LINE('',#59164,#13427);
#8553=LINE('',#59166,#13428);
#8554=LINE('',#59167,#13429);
#8555=LINE('',#59170,#13430);
#8556=LINE('',#59172,#13431);
#8557=LINE('',#59174,#13432);
#8558=LINE('',#59176,#13433);
#8559=LINE('',#59178,#13434);
#8560=LINE('',#59179,#13435);
#8561=LINE('',#59182,#13436);
#8562=LINE('',#59184,#13437);
#8563=LINE('',#59186,#13438);
#8564=LINE('',#59188,#13439);
#8565=LINE('',#59190,#13440);
#8566=LINE('',#59191,#13441);
#8567=LINE('',#59194,#13442);
#8568=LINE('',#59196,#13443);
#8569=LINE('',#59198,#13444);
#8570=LINE('',#59200,#13445);
#8571=LINE('',#59202,#13446);
#8572=LINE('',#59203,#13447);
#8573=LINE('',#59206,#13448);
#8574=LINE('',#59208,#13449);
#8575=LINE('',#59210,#13450);
#8576=LINE('',#59212,#13451);
#8577=LINE('',#59214,#13452);
#8578=LINE('',#59215,#13453);
#8579=LINE('',#59218,#13454);
#8580=LINE('',#59220,#13455);
#8581=LINE('',#59222,#13456);
#8582=LINE('',#59224,#13457);
#8583=LINE('',#59226,#13458);
#8584=LINE('',#59227,#13459);
#8585=LINE('',#59230,#13460);
#8586=LINE('',#59232,#13461);
#8587=LINE('',#59234,#13462);
#8588=LINE('',#59236,#13463);
#8589=LINE('',#59238,#13464);
#8590=LINE('',#59239,#13465);
#8591=LINE('',#59242,#13466);
#8592=LINE('',#59244,#13467);
#8593=LINE('',#59246,#13468);
#8594=LINE('',#59248,#13469);
#8595=LINE('',#59250,#13470);
#8596=LINE('',#59251,#13471);
#8597=LINE('',#59254,#13472);
#8598=LINE('',#59256,#13473);
#8599=LINE('',#59258,#13474);
#8600=LINE('',#59260,#13475);
#8601=LINE('',#59262,#13476);
#8602=LINE('',#59263,#13477);
#8603=LINE('',#59266,#13478);
#8604=LINE('',#59268,#13479);
#8605=LINE('',#59270,#13480);
#8606=LINE('',#59272,#13481);
#8607=LINE('',#59274,#13482);
#8608=LINE('',#59275,#13483);
#8609=LINE('',#59278,#13484);
#8610=LINE('',#59280,#13485);
#8611=LINE('',#59282,#13486);
#8612=LINE('',#59284,#13487);
#8613=LINE('',#59286,#13488);
#8614=LINE('',#59287,#13489);
#8615=LINE('',#59290,#13490);
#8616=LINE('',#59292,#13491);
#8617=LINE('',#59294,#13492);
#8618=LINE('',#59296,#13493);
#8619=LINE('',#59298,#13494);
#8620=LINE('',#59299,#13495);
#8621=LINE('',#59302,#13496);
#8622=LINE('',#59304,#13497);
#8623=LINE('',#59306,#13498);
#8624=LINE('',#59308,#13499);
#8625=LINE('',#59310,#13500);
#8626=LINE('',#59311,#13501);
#8627=LINE('',#59314,#13502);
#8628=LINE('',#59316,#13503);
#8629=LINE('',#59318,#13504);
#8630=LINE('',#59320,#13505);
#8631=LINE('',#59322,#13506);
#8632=LINE('',#59323,#13507);
#8633=LINE('',#59326,#13508);
#8634=LINE('',#59328,#13509);
#8635=LINE('',#59330,#13510);
#8636=LINE('',#59332,#13511);
#8637=LINE('',#59334,#13512);
#8638=LINE('',#59335,#13513);
#8639=LINE('',#59338,#13514);
#8640=LINE('',#59340,#13515);
#8641=LINE('',#59342,#13516);
#8642=LINE('',#59344,#13517);
#8643=LINE('',#59346,#13518);
#8644=LINE('',#59347,#13519);
#8645=LINE('',#59350,#13520);
#8646=LINE('',#59352,#13521);
#8647=LINE('',#59354,#13522);
#8648=LINE('',#59356,#13523);
#8649=LINE('',#59358,#13524);
#8650=LINE('',#59359,#13525);
#8651=LINE('',#59362,#13526);
#8652=LINE('',#59364,#13527);
#8653=LINE('',#59366,#13528);
#8654=LINE('',#59368,#13529);
#8655=LINE('',#59370,#13530);
#8656=LINE('',#59371,#13531);
#8657=LINE('',#59374,#13532);
#8658=LINE('',#59376,#13533);
#8659=LINE('',#59378,#13534);
#8660=LINE('',#59380,#13535);
#8661=LINE('',#59382,#13536);
#8662=LINE('',#59383,#13537);
#8663=LINE('',#59386,#13538);
#8664=LINE('',#59388,#13539);
#8665=LINE('',#59390,#13540);
#8666=LINE('',#59392,#13541);
#8667=LINE('',#59394,#13542);
#8668=LINE('',#59395,#13543);
#8669=LINE('',#59398,#13544);
#8670=LINE('',#59400,#13545);
#8671=LINE('',#59402,#13546);
#8672=LINE('',#59404,#13547);
#8673=LINE('',#59406,#13548);
#8674=LINE('',#59407,#13549);
#8675=LINE('',#59410,#13550);
#8676=LINE('',#59412,#13551);
#8677=LINE('',#59414,#13552);
#8678=LINE('',#59416,#13553);
#8679=LINE('',#59418,#13554);
#8680=LINE('',#59419,#13555);
#8681=LINE('',#59422,#13556);
#8682=LINE('',#59424,#13557);
#8683=LINE('',#59426,#13558);
#8684=LINE('',#59428,#13559);
#8685=LINE('',#59430,#13560);
#8686=LINE('',#59431,#13561);
#8687=LINE('',#59434,#13562);
#8688=LINE('',#59436,#13563);
#8689=LINE('',#59438,#13564);
#8690=LINE('',#59440,#13565);
#8691=LINE('',#59442,#13566);
#8692=LINE('',#59443,#13567);
#8693=LINE('',#59446,#13568);
#8694=LINE('',#59448,#13569);
#8695=LINE('',#59450,#13570);
#8696=LINE('',#59452,#13571);
#8697=LINE('',#59454,#13572);
#8698=LINE('',#59455,#13573);
#8699=LINE('',#59458,#13574);
#8700=LINE('',#59460,#13575);
#8701=LINE('',#59462,#13576);
#8702=LINE('',#59464,#13577);
#8703=LINE('',#59466,#13578);
#8704=LINE('',#59467,#13579);
#8705=LINE('',#59470,#13580);
#8706=LINE('',#59472,#13581);
#8707=LINE('',#59474,#13582);
#8708=LINE('',#59476,#13583);
#8709=LINE('',#59478,#13584);
#8710=LINE('',#59479,#13585);
#8711=LINE('',#59482,#13586);
#8712=LINE('',#59484,#13587);
#8713=LINE('',#59486,#13588);
#8714=LINE('',#59488,#13589);
#8715=LINE('',#59490,#13590);
#8716=LINE('',#59491,#13591);
#8717=LINE('',#59494,#13592);
#8718=LINE('',#59496,#13593);
#8719=LINE('',#59498,#13594);
#8720=LINE('',#59500,#13595);
#8721=LINE('',#59502,#13596);
#8722=LINE('',#59503,#13597);
#8723=LINE('',#59506,#13598);
#8724=LINE('',#59508,#13599);
#8725=LINE('',#59510,#13600);
#8726=LINE('',#59512,#13601);
#8727=LINE('',#59514,#13602);
#8728=LINE('',#59515,#13603);
#8729=LINE('',#59518,#13604);
#8730=LINE('',#59520,#13605);
#8731=LINE('',#59522,#13606);
#8732=LINE('',#59524,#13607);
#8733=LINE('',#59526,#13608);
#8734=LINE('',#59527,#13609);
#8735=LINE('',#59530,#13610);
#8736=LINE('',#59532,#13611);
#8737=LINE('',#59534,#13612);
#8738=LINE('',#59536,#13613);
#8739=LINE('',#59538,#13614);
#8740=LINE('',#59539,#13615);
#8741=LINE('',#59542,#13616);
#8742=LINE('',#59544,#13617);
#8743=LINE('',#59546,#13618);
#8744=LINE('',#59548,#13619);
#8745=LINE('',#59550,#13620);
#8746=LINE('',#59551,#13621);
#8747=LINE('',#59554,#13622);
#8748=LINE('',#59556,#13623);
#8749=LINE('',#59558,#13624);
#8750=LINE('',#59560,#13625);
#8751=LINE('',#59562,#13626);
#8752=LINE('',#59563,#13627);
#8753=LINE('',#59566,#13628);
#8754=LINE('',#59568,#13629);
#8755=LINE('',#59570,#13630);
#8756=LINE('',#59572,#13631);
#8757=LINE('',#59574,#13632);
#8758=LINE('',#59575,#13633);
#8759=LINE('',#59578,#13634);
#8760=LINE('',#59580,#13635);
#8761=LINE('',#59582,#13636);
#8762=LINE('',#59584,#13637);
#8763=LINE('',#59586,#13638);
#8764=LINE('',#59587,#13639);
#8765=LINE('',#59590,#13640);
#8766=LINE('',#59592,#13641);
#8767=LINE('',#59594,#13642);
#8768=LINE('',#59596,#13643);
#8769=LINE('',#59598,#13644);
#8770=LINE('',#59599,#13645);
#8771=LINE('',#59602,#13646);
#8772=LINE('',#59604,#13647);
#8773=LINE('',#59606,#13648);
#8774=LINE('',#59608,#13649);
#8775=LINE('',#59610,#13650);
#8776=LINE('',#59611,#13651);
#8777=LINE('',#59614,#13652);
#8778=LINE('',#59616,#13653);
#8779=LINE('',#59618,#13654);
#8780=LINE('',#59620,#13655);
#8781=LINE('',#59622,#13656);
#8782=LINE('',#59623,#13657);
#8783=LINE('',#59626,#13658);
#8784=LINE('',#59628,#13659);
#8785=LINE('',#59630,#13660);
#8786=LINE('',#59632,#13661);
#8787=LINE('',#59634,#13662);
#8788=LINE('',#59635,#13663);
#8789=LINE('',#59638,#13664);
#8790=LINE('',#59640,#13665);
#8791=LINE('',#59642,#13666);
#8792=LINE('',#59644,#13667);
#8793=LINE('',#59646,#13668);
#8794=LINE('',#59647,#13669);
#8795=LINE('',#59650,#13670);
#8796=LINE('',#59652,#13671);
#8797=LINE('',#59654,#13672);
#8798=LINE('',#59656,#13673);
#8799=LINE('',#59658,#13674);
#8800=LINE('',#59659,#13675);
#8801=LINE('',#59662,#13676);
#8802=LINE('',#59664,#13677);
#8803=LINE('',#59666,#13678);
#8804=LINE('',#59668,#13679);
#8805=LINE('',#59670,#13680);
#8806=LINE('',#59671,#13681);
#8807=LINE('',#59674,#13682);
#8808=LINE('',#59676,#13683);
#8809=LINE('',#59678,#13684);
#8810=LINE('',#59680,#13685);
#8811=LINE('',#59682,#13686);
#8812=LINE('',#59683,#13687);
#8813=LINE('',#59686,#13688);
#8814=LINE('',#59688,#13689);
#8815=LINE('',#59690,#13690);
#8816=LINE('',#59692,#13691);
#8817=LINE('',#59694,#13692);
#8818=LINE('',#59695,#13693);
#8819=LINE('',#59698,#13694);
#8820=LINE('',#59700,#13695);
#8821=LINE('',#59702,#13696);
#8822=LINE('',#59704,#13697);
#8823=LINE('',#59706,#13698);
#8824=LINE('',#59707,#13699);
#8825=LINE('',#59710,#13700);
#8826=LINE('',#59712,#13701);
#8827=LINE('',#59714,#13702);
#8828=LINE('',#59716,#13703);
#8829=LINE('',#59718,#13704);
#8830=LINE('',#59719,#13705);
#8831=LINE('',#59722,#13706);
#8832=LINE('',#59724,#13707);
#8833=LINE('',#59726,#13708);
#8834=LINE('',#59728,#13709);
#8835=LINE('',#59730,#13710);
#8836=LINE('',#59731,#13711);
#8837=LINE('',#59734,#13712);
#8838=LINE('',#59736,#13713);
#8839=LINE('',#59738,#13714);
#8840=LINE('',#59740,#13715);
#8841=LINE('',#59742,#13716);
#8842=LINE('',#59743,#13717);
#8843=LINE('',#59746,#13718);
#8844=LINE('',#59748,#13719);
#8845=LINE('',#59750,#13720);
#8846=LINE('',#59752,#13721);
#8847=LINE('',#59754,#13722);
#8848=LINE('',#59755,#13723);
#8849=LINE('',#59758,#13724);
#8850=LINE('',#59760,#13725);
#8851=LINE('',#59762,#13726);
#8852=LINE('',#59764,#13727);
#8853=LINE('',#59766,#13728);
#8854=LINE('',#59767,#13729);
#8855=LINE('',#59770,#13730);
#8856=LINE('',#59772,#13731);
#8857=LINE('',#59774,#13732);
#8858=LINE('',#59776,#13733);
#8859=LINE('',#59778,#13734);
#8860=LINE('',#59779,#13735);
#8861=LINE('',#59782,#13736);
#8862=LINE('',#59784,#13737);
#8863=LINE('',#59786,#13738);
#8864=LINE('',#59788,#13739);
#8865=LINE('',#59790,#13740);
#8866=LINE('',#59791,#13741);
#8867=LINE('',#59794,#13742);
#8868=LINE('',#59796,#13743);
#8869=LINE('',#59798,#13744);
#8870=LINE('',#59800,#13745);
#8871=LINE('',#59802,#13746);
#8872=LINE('',#59803,#13747);
#8873=LINE('',#59806,#13748);
#8874=LINE('',#59808,#13749);
#8875=LINE('',#59810,#13750);
#8876=LINE('',#59812,#13751);
#8877=LINE('',#59814,#13752);
#8878=LINE('',#59815,#13753);
#8879=LINE('',#59818,#13754);
#8880=LINE('',#59820,#13755);
#8881=LINE('',#59822,#13756);
#8882=LINE('',#59824,#13757);
#8883=LINE('',#59826,#13758);
#8884=LINE('',#59827,#13759);
#8885=LINE('',#59830,#13760);
#8886=LINE('',#59832,#13761);
#8887=LINE('',#59834,#13762);
#8888=LINE('',#59836,#13763);
#8889=LINE('',#59838,#13764);
#8890=LINE('',#59839,#13765);
#8891=LINE('',#59842,#13766);
#8892=LINE('',#59844,#13767);
#8893=LINE('',#59846,#13768);
#8894=LINE('',#59848,#13769);
#8895=LINE('',#59850,#13770);
#8896=LINE('',#59851,#13771);
#8897=LINE('',#59854,#13772);
#8898=LINE('',#59856,#13773);
#8899=LINE('',#59858,#13774);
#8900=LINE('',#59860,#13775);
#8901=LINE('',#59862,#13776);
#8902=LINE('',#59863,#13777);
#8903=LINE('',#59866,#13778);
#8904=LINE('',#59868,#13779);
#8905=LINE('',#59870,#13780);
#8906=LINE('',#59872,#13781);
#8907=LINE('',#59874,#13782);
#8908=LINE('',#59875,#13783);
#8909=LINE('',#59878,#13784);
#8910=LINE('',#59880,#13785);
#8911=LINE('',#59882,#13786);
#8912=LINE('',#59884,#13787);
#8913=LINE('',#59886,#13788);
#8914=LINE('',#59887,#13789);
#8915=LINE('',#59890,#13790);
#8916=LINE('',#59892,#13791);
#8917=LINE('',#59894,#13792);
#8918=LINE('',#59896,#13793);
#8919=LINE('',#59898,#13794);
#8920=LINE('',#59899,#13795);
#8921=LINE('',#59902,#13796);
#8922=LINE('',#59904,#13797);
#8923=LINE('',#59906,#13798);
#8924=LINE('',#59908,#13799);
#8925=LINE('',#59910,#13800);
#8926=LINE('',#59911,#13801);
#8927=LINE('',#59914,#13802);
#8928=LINE('',#59916,#13803);
#8929=LINE('',#59918,#13804);
#8930=LINE('',#59920,#13805);
#8931=LINE('',#59922,#13806);
#8932=LINE('',#59923,#13807);
#8933=LINE('',#59926,#13808);
#8934=LINE('',#59928,#13809);
#8935=LINE('',#59930,#13810);
#8936=LINE('',#59932,#13811);
#8937=LINE('',#59934,#13812);
#8938=LINE('',#59935,#13813);
#8939=LINE('',#59938,#13814);
#8940=LINE('',#59940,#13815);
#8941=LINE('',#59942,#13816);
#8942=LINE('',#59944,#13817);
#8943=LINE('',#59946,#13818);
#8944=LINE('',#59947,#13819);
#8945=LINE('',#59950,#13820);
#8946=LINE('',#59952,#13821);
#8947=LINE('',#59954,#13822);
#8948=LINE('',#59956,#13823);
#8949=LINE('',#59958,#13824);
#8950=LINE('',#59959,#13825);
#8951=LINE('',#59962,#13826);
#8952=LINE('',#59964,#13827);
#8953=LINE('',#59966,#13828);
#8954=LINE('',#59968,#13829);
#8955=LINE('',#59970,#13830);
#8956=LINE('',#59971,#13831);
#8957=LINE('',#59974,#13832);
#8958=LINE('',#59976,#13833);
#8959=LINE('',#59978,#13834);
#8960=LINE('',#59980,#13835);
#8961=LINE('',#59982,#13836);
#8962=LINE('',#59983,#13837);
#8963=LINE('',#59986,#13838);
#8964=LINE('',#59988,#13839);
#8965=LINE('',#59990,#13840);
#8966=LINE('',#59992,#13841);
#8967=LINE('',#59994,#13842);
#8968=LINE('',#59995,#13843);
#8969=LINE('',#59998,#13844);
#8970=LINE('',#60000,#13845);
#8971=LINE('',#60002,#13846);
#8972=LINE('',#60004,#13847);
#8973=LINE('',#60006,#13848);
#8974=LINE('',#60007,#13849);
#8975=LINE('',#60010,#13850);
#8976=LINE('',#60012,#13851);
#8977=LINE('',#60014,#13852);
#8978=LINE('',#60016,#13853);
#8979=LINE('',#60018,#13854);
#8980=LINE('',#60019,#13855);
#8981=LINE('',#60022,#13856);
#8982=LINE('',#60024,#13857);
#8983=LINE('',#60026,#13858);
#8984=LINE('',#60028,#13859);
#8985=LINE('',#60030,#13860);
#8986=LINE('',#60031,#13861);
#8987=LINE('',#60034,#13862);
#8988=LINE('',#60036,#13863);
#8989=LINE('',#60038,#13864);
#8990=LINE('',#60040,#13865);
#8991=LINE('',#60042,#13866);
#8992=LINE('',#60043,#13867);
#8993=LINE('',#60046,#13868);
#8994=LINE('',#60048,#13869);
#8995=LINE('',#60050,#13870);
#8996=LINE('',#60052,#13871);
#8997=LINE('',#60054,#13872);
#8998=LINE('',#60055,#13873);
#8999=LINE('',#60058,#13874);
#9000=LINE('',#60060,#13875);
#9001=LINE('',#60062,#13876);
#9002=LINE('',#60064,#13877);
#9003=LINE('',#60066,#13878);
#9004=LINE('',#60067,#13879);
#9005=LINE('',#60070,#13880);
#9006=LINE('',#60072,#13881);
#9007=LINE('',#60074,#13882);
#9008=LINE('',#60076,#13883);
#9009=LINE('',#60078,#13884);
#9010=LINE('',#60079,#13885);
#9011=LINE('',#60082,#13886);
#9012=LINE('',#60084,#13887);
#9013=LINE('',#60086,#13888);
#9014=LINE('',#60088,#13889);
#9015=LINE('',#60090,#13890);
#9016=LINE('',#60091,#13891);
#9017=LINE('',#60094,#13892);
#9018=LINE('',#60096,#13893);
#9019=LINE('',#60098,#13894);
#9020=LINE('',#60100,#13895);
#9021=LINE('',#60102,#13896);
#9022=LINE('',#60103,#13897);
#9023=LINE('',#60106,#13898);
#9024=LINE('',#60108,#13899);
#9025=LINE('',#60110,#13900);
#9026=LINE('',#60112,#13901);
#9027=LINE('',#60114,#13902);
#9028=LINE('',#60115,#13903);
#9029=LINE('',#60118,#13904);
#9030=LINE('',#60120,#13905);
#9031=LINE('',#60122,#13906);
#9032=LINE('',#60124,#13907);
#9033=LINE('',#60126,#13908);
#9034=LINE('',#60127,#13909);
#9035=LINE('',#60130,#13910);
#9036=LINE('',#60132,#13911);
#9037=LINE('',#60134,#13912);
#9038=LINE('',#60136,#13913);
#9039=LINE('',#60138,#13914);
#9040=LINE('',#60139,#13915);
#9041=LINE('',#60142,#13916);
#9042=LINE('',#60144,#13917);
#9043=LINE('',#60146,#13918);
#9044=LINE('',#60148,#13919);
#9045=LINE('',#60150,#13920);
#9046=LINE('',#60151,#13921);
#9047=LINE('',#60154,#13922);
#9048=LINE('',#60156,#13923);
#9049=LINE('',#60158,#13924);
#9050=LINE('',#60160,#13925);
#9051=LINE('',#60162,#13926);
#9052=LINE('',#60163,#13927);
#9053=LINE('',#60166,#13928);
#9054=LINE('',#60168,#13929);
#9055=LINE('',#60170,#13930);
#9056=LINE('',#60172,#13931);
#9057=LINE('',#60174,#13932);
#9058=LINE('',#60175,#13933);
#9059=LINE('',#60178,#13934);
#9060=LINE('',#60180,#13935);
#9061=LINE('',#60182,#13936);
#9062=LINE('',#60184,#13937);
#9063=LINE('',#60186,#13938);
#9064=LINE('',#60187,#13939);
#9065=LINE('',#60190,#13940);
#9066=LINE('',#60192,#13941);
#9067=LINE('',#60194,#13942);
#9068=LINE('',#60196,#13943);
#9069=LINE('',#60198,#13944);
#9070=LINE('',#60199,#13945);
#9071=LINE('',#60202,#13946);
#9072=LINE('',#60204,#13947);
#9073=LINE('',#60206,#13948);
#9074=LINE('',#60208,#13949);
#9075=LINE('',#60210,#13950);
#9076=LINE('',#60211,#13951);
#9077=LINE('',#60214,#13952);
#9078=LINE('',#60216,#13953);
#9079=LINE('',#60218,#13954);
#9080=LINE('',#60220,#13955);
#9081=LINE('',#60222,#13956);
#9082=LINE('',#60223,#13957);
#9083=LINE('',#60226,#13958);
#9084=LINE('',#60228,#13959);
#9085=LINE('',#60230,#13960);
#9086=LINE('',#60232,#13961);
#9087=LINE('',#60234,#13962);
#9088=LINE('',#60235,#13963);
#9089=LINE('',#60238,#13964);
#9090=LINE('',#60240,#13965);
#9091=LINE('',#60242,#13966);
#9092=LINE('',#60244,#13967);
#9093=LINE('',#60246,#13968);
#9094=LINE('',#60247,#13969);
#9095=LINE('',#60250,#13970);
#9096=LINE('',#60252,#13971);
#9097=LINE('',#60254,#13972);
#9098=LINE('',#60256,#13973);
#9099=LINE('',#60258,#13974);
#9100=LINE('',#60259,#13975);
#9101=LINE('',#60262,#13976);
#9102=LINE('',#60264,#13977);
#9103=LINE('',#60266,#13978);
#9104=LINE('',#60268,#13979);
#9105=LINE('',#60270,#13980);
#9106=LINE('',#60271,#13981);
#9107=LINE('',#60274,#13982);
#9108=LINE('',#60276,#13983);
#9109=LINE('',#60278,#13984);
#9110=LINE('',#60280,#13985);
#9111=LINE('',#60282,#13986);
#9112=LINE('',#60283,#13987);
#9113=LINE('',#60286,#13988);
#9114=LINE('',#60288,#13989);
#9115=LINE('',#60290,#13990);
#9116=LINE('',#60292,#13991);
#9117=LINE('',#60294,#13992);
#9118=LINE('',#60295,#13993);
#9119=LINE('',#60298,#13994);
#9120=LINE('',#60300,#13995);
#9121=LINE('',#60302,#13996);
#9122=LINE('',#60304,#13997);
#9123=LINE('',#60306,#13998);
#9124=LINE('',#60307,#13999);
#9125=LINE('',#60310,#14000);
#9126=LINE('',#60312,#14001);
#9127=LINE('',#60314,#14002);
#9128=LINE('',#60316,#14003);
#9129=LINE('',#60318,#14004);
#9130=LINE('',#60319,#14005);
#9131=LINE('',#60322,#14006);
#9132=LINE('',#60324,#14007);
#9133=LINE('',#60326,#14008);
#9134=LINE('',#60328,#14009);
#9135=LINE('',#60330,#14010);
#9136=LINE('',#60331,#14011);
#9137=LINE('',#60334,#14012);
#9138=LINE('',#60336,#14013);
#9139=LINE('',#60338,#14014);
#9140=LINE('',#60340,#14015);
#9141=LINE('',#60342,#14016);
#9142=LINE('',#60343,#14017);
#9143=LINE('',#60346,#14018);
#9144=LINE('',#60348,#14019);
#9145=LINE('',#60350,#14020);
#9146=LINE('',#60352,#14021);
#9147=LINE('',#60354,#14022);
#9148=LINE('',#60355,#14023);
#9149=LINE('',#60358,#14024);
#9150=LINE('',#60360,#14025);
#9151=LINE('',#60362,#14026);
#9152=LINE('',#60364,#14027);
#9153=LINE('',#60366,#14028);
#9154=LINE('',#60367,#14029);
#9155=LINE('',#60370,#14030);
#9156=LINE('',#60372,#14031);
#9157=LINE('',#60374,#14032);
#9158=LINE('',#60376,#14033);
#9159=LINE('',#60378,#14034);
#9160=LINE('',#60379,#14035);
#9161=LINE('',#60382,#14036);
#9162=LINE('',#60384,#14037);
#9163=LINE('',#60386,#14038);
#9164=LINE('',#60388,#14039);
#9165=LINE('',#60390,#14040);
#9166=LINE('',#60391,#14041);
#9167=LINE('',#60394,#14042);
#9168=LINE('',#60396,#14043);
#9169=LINE('',#60398,#14044);
#9170=LINE('',#60400,#14045);
#9171=LINE('',#60402,#14046);
#9172=LINE('',#60403,#14047);
#9173=LINE('',#60406,#14048);
#9174=LINE('',#60408,#14049);
#9175=LINE('',#60410,#14050);
#9176=LINE('',#60412,#14051);
#9177=LINE('',#60414,#14052);
#9178=LINE('',#60415,#14053);
#9179=LINE('',#60418,#14054);
#9180=LINE('',#60420,#14055);
#9181=LINE('',#60422,#14056);
#9182=LINE('',#60424,#14057);
#9183=LINE('',#60426,#14058);
#9184=LINE('',#60427,#14059);
#9185=LINE('',#60430,#14060);
#9186=LINE('',#60432,#14061);
#9187=LINE('',#60434,#14062);
#9188=LINE('',#60436,#14063);
#9189=LINE('',#60438,#14064);
#9190=LINE('',#60439,#14065);
#9191=LINE('',#60442,#14066);
#9192=LINE('',#60444,#14067);
#9193=LINE('',#60446,#14068);
#9194=LINE('',#60448,#14069);
#9195=LINE('',#60450,#14070);
#9196=LINE('',#60451,#14071);
#9197=LINE('',#60454,#14072);
#9198=LINE('',#60456,#14073);
#9199=LINE('',#60458,#14074);
#9200=LINE('',#60460,#14075);
#9201=LINE('',#60462,#14076);
#9202=LINE('',#60463,#14077);
#9203=LINE('',#60466,#14078);
#9204=LINE('',#60468,#14079);
#9205=LINE('',#60470,#14080);
#9206=LINE('',#60472,#14081);
#9207=LINE('',#60474,#14082);
#9208=LINE('',#60475,#14083);
#9209=LINE('',#60478,#14084);
#9210=LINE('',#60480,#14085);
#9211=LINE('',#60482,#14086);
#9212=LINE('',#60484,#14087);
#9213=LINE('',#60486,#14088);
#9214=LINE('',#60487,#14089);
#9215=LINE('',#60490,#14090);
#9216=LINE('',#60492,#14091);
#9217=LINE('',#60494,#14092);
#9218=LINE('',#60496,#14093);
#9219=LINE('',#60498,#14094);
#9220=LINE('',#60499,#14095);
#9221=LINE('',#60502,#14096);
#9222=LINE('',#60504,#14097);
#9223=LINE('',#60506,#14098);
#9224=LINE('',#60508,#14099);
#9225=LINE('',#60510,#14100);
#9226=LINE('',#60511,#14101);
#9227=LINE('',#60514,#14102);
#9228=LINE('',#60516,#14103);
#9229=LINE('',#60518,#14104);
#9230=LINE('',#60520,#14105);
#9231=LINE('',#60522,#14106);
#9232=LINE('',#60523,#14107);
#9233=LINE('',#60526,#14108);
#9234=LINE('',#60528,#14109);
#9235=LINE('',#60530,#14110);
#9236=LINE('',#60532,#14111);
#9237=LINE('',#60534,#14112);
#9238=LINE('',#60535,#14113);
#9239=LINE('',#60538,#14114);
#9240=LINE('',#60540,#14115);
#9241=LINE('',#60542,#14116);
#9242=LINE('',#60544,#14117);
#9243=LINE('',#60546,#14118);
#9244=LINE('',#60547,#14119);
#9245=LINE('',#60550,#14120);
#9246=LINE('',#60552,#14121);
#9247=LINE('',#60554,#14122);
#9248=LINE('',#60556,#14123);
#9249=LINE('',#60558,#14124);
#9250=LINE('',#60559,#14125);
#9251=LINE('',#60562,#14126);
#9252=LINE('',#60564,#14127);
#9253=LINE('',#60566,#14128);
#9254=LINE('',#60568,#14129);
#9255=LINE('',#60570,#14130);
#9256=LINE('',#60571,#14131);
#9257=LINE('',#60574,#14132);
#9258=LINE('',#60576,#14133);
#9259=LINE('',#60578,#14134);
#9260=LINE('',#60580,#14135);
#9261=LINE('',#60582,#14136);
#9262=LINE('',#60583,#14137);
#9263=LINE('',#60586,#14138);
#9264=LINE('',#60588,#14139);
#9265=LINE('',#60590,#14140);
#9266=LINE('',#60592,#14141);
#9267=LINE('',#60594,#14142);
#9268=LINE('',#60595,#14143);
#9269=LINE('',#60598,#14144);
#9270=LINE('',#60600,#14145);
#9271=LINE('',#60602,#14146);
#9272=LINE('',#60604,#14147);
#9273=LINE('',#60606,#14148);
#9274=LINE('',#60607,#14149);
#9275=LINE('',#60610,#14150);
#9276=LINE('',#60612,#14151);
#9277=LINE('',#60614,#14152);
#9278=LINE('',#60616,#14153);
#9279=LINE('',#60618,#14154);
#9280=LINE('',#60619,#14155);
#9281=LINE('',#60622,#14156);
#9282=LINE('',#60624,#14157);
#9283=LINE('',#60626,#14158);
#9284=LINE('',#60628,#14159);
#9285=LINE('',#60630,#14160);
#9286=LINE('',#60631,#14161);
#9287=LINE('',#60634,#14162);
#9288=LINE('',#60636,#14163);
#9289=LINE('',#60638,#14164);
#9290=LINE('',#60640,#14165);
#9291=LINE('',#60642,#14166);
#9292=LINE('',#60643,#14167);
#9293=LINE('',#60646,#14168);
#9294=LINE('',#60648,#14169);
#9295=LINE('',#60650,#14170);
#9296=LINE('',#60652,#14171);
#9297=LINE('',#60654,#14172);
#9298=LINE('',#60655,#14173);
#9299=LINE('',#60658,#14174);
#9300=LINE('',#60660,#14175);
#9301=LINE('',#60662,#14176);
#9302=LINE('',#60664,#14177);
#9303=LINE('',#60666,#14178);
#9304=LINE('',#60667,#14179);
#9305=LINE('',#60670,#14180);
#9306=LINE('',#60672,#14181);
#9307=LINE('',#60674,#14182);
#9308=LINE('',#60676,#14183);
#9309=LINE('',#60678,#14184);
#9310=LINE('',#60679,#14185);
#9311=LINE('',#60682,#14186);
#9312=LINE('',#60684,#14187);
#9313=LINE('',#60686,#14188);
#9314=LINE('',#60688,#14189);
#9315=LINE('',#60690,#14190);
#9316=LINE('',#60691,#14191);
#9317=LINE('',#60694,#14192);
#9318=LINE('',#60696,#14193);
#9319=LINE('',#60698,#14194);
#9320=LINE('',#60700,#14195);
#9321=LINE('',#60702,#14196);
#9322=LINE('',#60703,#14197);
#9323=LINE('',#60706,#14198);
#9324=LINE('',#60708,#14199);
#9325=LINE('',#60710,#14200);
#9326=LINE('',#60712,#14201);
#9327=LINE('',#60714,#14202);
#9328=LINE('',#60715,#14203);
#9329=LINE('',#60718,#14204);
#9330=LINE('',#60720,#14205);
#9331=LINE('',#60722,#14206);
#9332=LINE('',#60724,#14207);
#9333=LINE('',#60726,#14208);
#9334=LINE('',#60727,#14209);
#9335=LINE('',#60730,#14210);
#9336=LINE('',#60732,#14211);
#9337=LINE('',#60734,#14212);
#9338=LINE('',#60736,#14213);
#9339=LINE('',#60738,#14214);
#9340=LINE('',#60739,#14215);
#9341=LINE('',#60742,#14216);
#9342=LINE('',#60744,#14217);
#9343=LINE('',#60746,#14218);
#9344=LINE('',#60748,#14219);
#9345=LINE('',#60750,#14220);
#9346=LINE('',#60751,#14221);
#9347=LINE('',#60754,#14222);
#9348=LINE('',#60756,#14223);
#9349=LINE('',#60758,#14224);
#9350=LINE('',#60760,#14225);
#9351=LINE('',#60762,#14226);
#9352=LINE('',#60763,#14227);
#9353=LINE('',#60766,#14228);
#9354=LINE('',#60768,#14229);
#9355=LINE('',#60770,#14230);
#9356=LINE('',#60772,#14231);
#9357=LINE('',#60774,#14232);
#9358=LINE('',#60775,#14233);
#9359=LINE('',#60778,#14234);
#9360=LINE('',#60780,#14235);
#9361=LINE('',#60782,#14236);
#9362=LINE('',#60784,#14237);
#9363=LINE('',#60786,#14238);
#9364=LINE('',#60787,#14239);
#9365=LINE('',#60790,#14240);
#9366=LINE('',#60792,#14241);
#9367=LINE('',#60794,#14242);
#9368=LINE('',#60796,#14243);
#9369=LINE('',#60798,#14244);
#9370=LINE('',#60799,#14245);
#9371=LINE('',#60802,#14246);
#9372=LINE('',#60804,#14247);
#9373=LINE('',#60806,#14248);
#9374=LINE('',#60808,#14249);
#9375=LINE('',#60810,#14250);
#9376=LINE('',#60811,#14251);
#9377=LINE('',#60814,#14252);
#9378=LINE('',#60816,#14253);
#9379=LINE('',#60818,#14254);
#9380=LINE('',#60820,#14255);
#9381=LINE('',#60822,#14256);
#9382=LINE('',#60823,#14257);
#9383=LINE('',#60827,#14258);
#9384=LINE('',#60829,#14259);
#9385=LINE('',#60831,#14260);
#9386=LINE('',#60833,#14261);
#9387=LINE('',#60835,#14262);
#9388=LINE('',#60836,#14263);
#9389=LINE('',#60839,#14264);
#9390=LINE('',#60841,#14265);
#9391=LINE('',#60843,#14266);
#9392=LINE('',#60845,#14267);
#9393=LINE('',#60847,#14268);
#9394=LINE('',#60848,#14269);
#9395=LINE('',#60851,#14270);
#9396=LINE('',#60853,#14271);
#9397=LINE('',#60855,#14272);
#9398=LINE('',#60857,#14273);
#9399=LINE('',#60859,#14274);
#9400=LINE('',#60860,#14275);
#9401=LINE('',#60863,#14276);
#9402=LINE('',#60865,#14277);
#9403=LINE('',#60867,#14278);
#9404=LINE('',#60869,#14279);
#9405=LINE('',#60871,#14280);
#9406=LINE('',#60872,#14281);
#9407=LINE('',#60875,#14282);
#9408=LINE('',#60877,#14283);
#9409=LINE('',#60879,#14284);
#9410=LINE('',#60881,#14285);
#9411=LINE('',#60883,#14286);
#9412=LINE('',#60884,#14287);
#9413=LINE('',#60887,#14288);
#9414=LINE('',#60889,#14289);
#9415=LINE('',#60891,#14290);
#9416=LINE('',#60893,#14291);
#9417=LINE('',#60895,#14292);
#9418=LINE('',#60896,#14293);
#9419=LINE('',#60899,#14294);
#9420=LINE('',#60901,#14295);
#9421=LINE('',#60903,#14296);
#9422=LINE('',#60905,#14297);
#9423=LINE('',#60907,#14298);
#9424=LINE('',#60908,#14299);
#9425=LINE('',#60911,#14300);
#9426=LINE('',#60913,#14301);
#9427=LINE('',#60915,#14302);
#9428=LINE('',#60917,#14303);
#9429=LINE('',#60919,#14304);
#9430=LINE('',#60920,#14305);
#9431=LINE('',#60923,#14306);
#9432=LINE('',#60925,#14307);
#9433=LINE('',#60927,#14308);
#9434=LINE('',#60929,#14309);
#9435=LINE('',#60931,#14310);
#9436=LINE('',#60932,#14311);
#9437=LINE('',#60935,#14312);
#9438=LINE('',#60937,#14313);
#9439=LINE('',#60939,#14314);
#9440=LINE('',#60941,#14315);
#9441=LINE('',#60943,#14316);
#9442=LINE('',#60944,#14317);
#9443=LINE('',#60947,#14318);
#9444=LINE('',#60949,#14319);
#9445=LINE('',#60951,#14320);
#9446=LINE('',#60953,#14321);
#9447=LINE('',#60955,#14322);
#9448=LINE('',#60956,#14323);
#9449=LINE('',#60959,#14324);
#9450=LINE('',#60961,#14325);
#9451=LINE('',#60963,#14326);
#9452=LINE('',#60965,#14327);
#9453=LINE('',#60967,#14328);
#9454=LINE('',#60968,#14329);
#9455=LINE('',#60971,#14330);
#9456=LINE('',#60973,#14331);
#9457=LINE('',#60975,#14332);
#9458=LINE('',#60977,#14333);
#9459=LINE('',#60979,#14334);
#9460=LINE('',#60980,#14335);
#9461=LINE('',#60983,#14336);
#9462=LINE('',#60985,#14337);
#9463=LINE('',#60987,#14338);
#9464=LINE('',#60989,#14339);
#9465=LINE('',#60991,#14340);
#9466=LINE('',#60992,#14341);
#9467=LINE('',#60995,#14342);
#9468=LINE('',#60997,#14343);
#9469=LINE('',#60999,#14344);
#9470=LINE('',#61001,#14345);
#9471=LINE('',#61003,#14346);
#9472=LINE('',#61004,#14347);
#9473=LINE('',#61007,#14348);
#9474=LINE('',#61009,#14349);
#9475=LINE('',#61011,#14350);
#9476=LINE('',#61013,#14351);
#9477=LINE('',#61015,#14352);
#9478=LINE('',#61016,#14353);
#9479=LINE('',#61019,#14354);
#9480=LINE('',#61021,#14355);
#9481=LINE('',#61023,#14356);
#9482=LINE('',#61025,#14357);
#9483=LINE('',#61027,#14358);
#9484=LINE('',#61028,#14359);
#9485=LINE('',#61031,#14360);
#9486=LINE('',#61033,#14361);
#9487=LINE('',#61035,#14362);
#9488=LINE('',#61037,#14363);
#9489=LINE('',#61039,#14364);
#9490=LINE('',#61040,#14365);
#9491=LINE('',#61043,#14366);
#9492=LINE('',#61045,#14367);
#9493=LINE('',#61047,#14368);
#9494=LINE('',#61049,#14369);
#9495=LINE('',#61051,#14370);
#9496=LINE('',#61052,#14371);
#9497=LINE('',#61055,#14372);
#9498=LINE('',#61057,#14373);
#9499=LINE('',#61059,#14374);
#9500=LINE('',#61061,#14375);
#9501=LINE('',#61063,#14376);
#9502=LINE('',#61064,#14377);
#9503=LINE('',#61067,#14378);
#9504=LINE('',#61069,#14379);
#9505=LINE('',#61071,#14380);
#9506=LINE('',#61073,#14381);
#9507=LINE('',#61075,#14382);
#9508=LINE('',#61076,#14383);
#9509=LINE('',#61079,#14384);
#9510=LINE('',#61081,#14385);
#9511=LINE('',#61083,#14386);
#9512=LINE('',#61085,#14387);
#9513=LINE('',#61087,#14388);
#9514=LINE('',#61088,#14389);
#9515=LINE('',#61091,#14390);
#9516=LINE('',#61093,#14391);
#9517=LINE('',#61095,#14392);
#9518=LINE('',#61097,#14393);
#9519=LINE('',#61099,#14394);
#9520=LINE('',#61100,#14395);
#9521=LINE('',#61103,#14396);
#9522=LINE('',#61105,#14397);
#9523=LINE('',#61107,#14398);
#9524=LINE('',#61109,#14399);
#9525=LINE('',#61111,#14400);
#9526=LINE('',#61112,#14401);
#9527=LINE('',#61115,#14402);
#9528=LINE('',#61117,#14403);
#9529=LINE('',#61119,#14404);
#9530=LINE('',#61121,#14405);
#9531=LINE('',#61123,#14406);
#9532=LINE('',#61124,#14407);
#9533=LINE('',#61127,#14408);
#9534=LINE('',#61129,#14409);
#9535=LINE('',#61131,#14410);
#9536=LINE('',#61133,#14411);
#9537=LINE('',#61135,#14412);
#9538=LINE('',#61136,#14413);
#9539=LINE('',#61139,#14414);
#9540=LINE('',#61141,#14415);
#9541=LINE('',#61143,#14416);
#9542=LINE('',#61145,#14417);
#9543=LINE('',#61147,#14418);
#9544=LINE('',#61148,#14419);
#9545=LINE('',#61151,#14420);
#9546=LINE('',#61153,#14421);
#9547=LINE('',#61155,#14422);
#9548=LINE('',#61157,#14423);
#9549=LINE('',#61159,#14424);
#9550=LINE('',#61160,#14425);
#9551=LINE('',#61163,#14426);
#9552=LINE('',#61165,#14427);
#9553=LINE('',#61167,#14428);
#9554=LINE('',#61169,#14429);
#9555=LINE('',#61171,#14430);
#9556=LINE('',#61172,#14431);
#9557=LINE('',#61175,#14432);
#9558=LINE('',#61177,#14433);
#9559=LINE('',#61179,#14434);
#9560=LINE('',#61181,#14435);
#9561=LINE('',#61183,#14436);
#9562=LINE('',#61184,#14437);
#9563=LINE('',#61187,#14438);
#9564=LINE('',#61189,#14439);
#9565=LINE('',#61191,#14440);
#9566=LINE('',#61193,#14441);
#9567=LINE('',#61195,#14442);
#9568=LINE('',#61196,#14443);
#9569=LINE('',#61199,#14444);
#9570=LINE('',#61201,#14445);
#9571=LINE('',#61203,#14446);
#9572=LINE('',#61205,#14447);
#9573=LINE('',#61207,#14448);
#9574=LINE('',#61208,#14449);
#9575=LINE('',#61211,#14450);
#9576=LINE('',#61213,#14451);
#9577=LINE('',#61215,#14452);
#9578=LINE('',#61217,#14453);
#9579=LINE('',#61219,#14454);
#9580=LINE('',#61220,#14455);
#9581=LINE('',#61223,#14456);
#9582=LINE('',#61225,#14457);
#9583=LINE('',#61227,#14458);
#9584=LINE('',#61229,#14459);
#9585=LINE('',#61231,#14460);
#9586=LINE('',#61232,#14461);
#9587=LINE('',#61235,#14462);
#9588=LINE('',#61237,#14463);
#9589=LINE('',#61239,#14464);
#9590=LINE('',#61241,#14465);
#9591=LINE('',#61243,#14466);
#9592=LINE('',#61244,#14467);
#9593=LINE('',#61247,#14468);
#9594=LINE('',#61249,#14469);
#9595=LINE('',#61251,#14470);
#9596=LINE('',#61253,#14471);
#9597=LINE('',#61255,#14472);
#9598=LINE('',#61256,#14473);
#9599=LINE('',#61259,#14474);
#9600=LINE('',#61261,#14475);
#9601=LINE('',#61263,#14476);
#9602=LINE('',#61265,#14477);
#9603=LINE('',#61267,#14478);
#9604=LINE('',#61268,#14479);
#9605=LINE('',#61271,#14480);
#9606=LINE('',#61273,#14481);
#9607=LINE('',#61275,#14482);
#9608=LINE('',#61277,#14483);
#9609=LINE('',#61279,#14484);
#9610=LINE('',#61280,#14485);
#9611=LINE('',#61283,#14486);
#9612=LINE('',#61285,#14487);
#9613=LINE('',#61287,#14488);
#9614=LINE('',#61289,#14489);
#9615=LINE('',#61291,#14490);
#9616=LINE('',#61292,#14491);
#9617=LINE('',#61295,#14492);
#9618=LINE('',#61297,#14493);
#9619=LINE('',#61299,#14494);
#9620=LINE('',#61301,#14495);
#9621=LINE('',#61303,#14496);
#9622=LINE('',#61304,#14497);
#9623=LINE('',#61307,#14498);
#9624=LINE('',#61309,#14499);
#9625=LINE('',#61311,#14500);
#9626=LINE('',#61313,#14501);
#9627=LINE('',#61315,#14502);
#9628=LINE('',#61316,#14503);
#9629=LINE('',#61319,#14504);
#9630=LINE('',#61321,#14505);
#9631=LINE('',#61323,#14506);
#9632=LINE('',#61325,#14507);
#9633=LINE('',#61327,#14508);
#9634=LINE('',#61328,#14509);
#9635=LINE('',#61331,#14510);
#9636=LINE('',#61333,#14511);
#9637=LINE('',#61335,#14512);
#9638=LINE('',#61337,#14513);
#9639=LINE('',#61339,#14514);
#9640=LINE('',#61340,#14515);
#9641=LINE('',#61343,#14516);
#9642=LINE('',#61345,#14517);
#9643=LINE('',#61347,#14518);
#9644=LINE('',#61349,#14519);
#9645=LINE('',#61351,#14520);
#9646=LINE('',#61352,#14521);
#9647=LINE('',#61355,#14522);
#9648=LINE('',#61357,#14523);
#9649=LINE('',#61359,#14524);
#9650=LINE('',#61361,#14525);
#9651=LINE('',#61363,#14526);
#9652=LINE('',#61364,#14527);
#9653=LINE('',#61367,#14528);
#9654=LINE('',#61369,#14529);
#9655=LINE('',#61371,#14530);
#9656=LINE('',#61373,#14531);
#9657=LINE('',#61375,#14532);
#9658=LINE('',#61376,#14533);
#9659=LINE('',#61379,#14534);
#9660=LINE('',#61381,#14535);
#9661=LINE('',#61383,#14536);
#9662=LINE('',#61385,#14537);
#9663=LINE('',#61387,#14538);
#9664=LINE('',#61388,#14539);
#9665=LINE('',#61391,#14540);
#9666=LINE('',#61393,#14541);
#9667=LINE('',#61395,#14542);
#9668=LINE('',#61397,#14543);
#9669=LINE('',#61399,#14544);
#9670=LINE('',#61400,#14545);
#9671=LINE('',#61403,#14546);
#9672=LINE('',#61405,#14547);
#9673=LINE('',#61407,#14548);
#9674=LINE('',#61409,#14549);
#9675=LINE('',#61411,#14550);
#9676=LINE('',#61412,#14551);
#9677=LINE('',#61415,#14552);
#9678=LINE('',#61417,#14553);
#9679=LINE('',#61419,#14554);
#9680=LINE('',#61421,#14555);
#9681=LINE('',#61423,#14556);
#9682=LINE('',#61424,#14557);
#9683=LINE('',#61427,#14558);
#9684=LINE('',#61429,#14559);
#9685=LINE('',#61431,#14560);
#9686=LINE('',#61433,#14561);
#9687=LINE('',#61435,#14562);
#9688=LINE('',#61436,#14563);
#9689=LINE('',#61439,#14564);
#9690=LINE('',#61441,#14565);
#9691=LINE('',#61443,#14566);
#9692=LINE('',#61445,#14567);
#9693=LINE('',#61447,#14568);
#9694=LINE('',#61448,#14569);
#9695=LINE('',#61451,#14570);
#9696=LINE('',#61453,#14571);
#9697=LINE('',#61455,#14572);
#9698=LINE('',#61457,#14573);
#9699=LINE('',#61459,#14574);
#9700=LINE('',#61460,#14575);
#9701=LINE('',#61463,#14576);
#9702=LINE('',#61465,#14577);
#9703=LINE('',#61467,#14578);
#9704=LINE('',#61469,#14579);
#9705=LINE('',#61471,#14580);
#9706=LINE('',#61472,#14581);
#9707=LINE('',#61475,#14582);
#9708=LINE('',#61477,#14583);
#9709=LINE('',#61479,#14584);
#9710=LINE('',#61481,#14585);
#9711=LINE('',#61483,#14586);
#9712=LINE('',#61484,#14587);
#9713=LINE('',#61487,#14588);
#9714=LINE('',#61489,#14589);
#9715=LINE('',#61491,#14590);
#9716=LINE('',#61493,#14591);
#9717=LINE('',#61495,#14592);
#9718=LINE('',#61496,#14593);
#9719=LINE('',#61499,#14594);
#9720=LINE('',#61501,#14595);
#9721=LINE('',#61503,#14596);
#9722=LINE('',#61505,#14597);
#9723=LINE('',#61507,#14598);
#9724=LINE('',#61508,#14599);
#9725=LINE('',#61511,#14600);
#9726=LINE('',#61513,#14601);
#9727=LINE('',#61515,#14602);
#9728=LINE('',#61517,#14603);
#9729=LINE('',#61519,#14604);
#9730=LINE('',#61520,#14605);
#9731=LINE('',#61523,#14606);
#9732=LINE('',#61525,#14607);
#9733=LINE('',#61527,#14608);
#9734=LINE('',#61529,#14609);
#9735=LINE('',#61531,#14610);
#9736=LINE('',#61532,#14611);
#9737=LINE('',#61535,#14612);
#9738=LINE('',#61537,#14613);
#9739=LINE('',#61539,#14614);
#9740=LINE('',#61541,#14615);
#9741=LINE('',#61543,#14616);
#9742=LINE('',#61544,#14617);
#9743=LINE('',#61547,#14618);
#9744=LINE('',#61549,#14619);
#9745=LINE('',#61551,#14620);
#9746=LINE('',#61553,#14621);
#9747=LINE('',#61555,#14622);
#9748=LINE('',#61556,#14623);
#9749=LINE('',#61559,#14624);
#9750=LINE('',#61561,#14625);
#9751=LINE('',#61563,#14626);
#9752=LINE('',#61565,#14627);
#9753=LINE('',#61567,#14628);
#9754=LINE('',#61568,#14629);
#9755=LINE('',#61571,#14630);
#9756=LINE('',#61573,#14631);
#9757=LINE('',#61575,#14632);
#9758=LINE('',#61577,#14633);
#9759=LINE('',#61579,#14634);
#9760=LINE('',#61580,#14635);
#9761=LINE('',#61583,#14636);
#9762=LINE('',#61585,#14637);
#9763=LINE('',#61587,#14638);
#9764=LINE('',#61589,#14639);
#9765=LINE('',#61591,#14640);
#9766=LINE('',#61592,#14641);
#9767=LINE('',#61595,#14642);
#9768=LINE('',#61597,#14643);
#9769=LINE('',#61599,#14644);
#9770=LINE('',#61601,#14645);
#9771=LINE('',#61603,#14646);
#9772=LINE('',#61604,#14647);
#9773=LINE('',#61607,#14648);
#9774=LINE('',#61609,#14649);
#9775=LINE('',#61611,#14650);
#9776=LINE('',#61613,#14651);
#9777=LINE('',#61615,#14652);
#9778=LINE('',#61616,#14653);
#9779=LINE('',#61619,#14654);
#9780=LINE('',#61621,#14655);
#9781=LINE('',#61623,#14656);
#9782=LINE('',#61625,#14657);
#9783=LINE('',#61627,#14658);
#9784=LINE('',#61628,#14659);
#9785=LINE('',#61631,#14660);
#9786=LINE('',#61633,#14661);
#9787=LINE('',#61635,#14662);
#9788=LINE('',#61637,#14663);
#9789=LINE('',#61639,#14664);
#9790=LINE('',#61640,#14665);
#9791=LINE('',#61643,#14666);
#9792=LINE('',#61645,#14667);
#9793=LINE('',#61647,#14668);
#9794=LINE('',#61649,#14669);
#9795=LINE('',#61651,#14670);
#9796=LINE('',#61652,#14671);
#9797=LINE('',#61655,#14672);
#9798=LINE('',#61657,#14673);
#9799=LINE('',#61659,#14674);
#9800=LINE('',#61661,#14675);
#9801=LINE('',#61663,#14676);
#9802=LINE('',#61664,#14677);
#9803=LINE('',#61667,#14678);
#9804=LINE('',#61669,#14679);
#9805=LINE('',#61671,#14680);
#9806=LINE('',#61673,#14681);
#9807=LINE('',#61675,#14682);
#9808=LINE('',#61676,#14683);
#9809=LINE('',#61679,#14684);
#9810=LINE('',#61681,#14685);
#9811=LINE('',#61683,#14686);
#9812=LINE('',#61685,#14687);
#9813=LINE('',#61687,#14688);
#9814=LINE('',#61688,#14689);
#9815=LINE('',#61691,#14690);
#9816=LINE('',#61693,#14691);
#9817=LINE('',#61695,#14692);
#9818=LINE('',#61697,#14693);
#9819=LINE('',#61699,#14694);
#9820=LINE('',#61700,#14695);
#9821=LINE('',#61703,#14696);
#9822=LINE('',#61705,#14697);
#9823=LINE('',#61707,#14698);
#9824=LINE('',#61709,#14699);
#9825=LINE('',#61711,#14700);
#9826=LINE('',#61712,#14701);
#9827=LINE('',#61715,#14702);
#9828=LINE('',#61717,#14703);
#9829=LINE('',#61719,#14704);
#9830=LINE('',#61721,#14705);
#9831=LINE('',#61723,#14706);
#9832=LINE('',#61724,#14707);
#9833=LINE('',#61727,#14708);
#9834=LINE('',#61729,#14709);
#9835=LINE('',#61731,#14710);
#9836=LINE('',#61733,#14711);
#9837=LINE('',#61735,#14712);
#9838=LINE('',#61736,#14713);
#9839=LINE('',#61739,#14714);
#9840=LINE('',#61741,#14715);
#9841=LINE('',#61743,#14716);
#9842=LINE('',#61745,#14717);
#9843=LINE('',#61747,#14718);
#9844=LINE('',#61748,#14719);
#9845=LINE('',#61751,#14720);
#9846=LINE('',#61753,#14721);
#9847=LINE('',#61755,#14722);
#9848=LINE('',#61757,#14723);
#9849=LINE('',#61759,#14724);
#9850=LINE('',#61760,#14725);
#9851=LINE('',#61763,#14726);
#9852=LINE('',#61765,#14727);
#9853=LINE('',#61767,#14728);
#9854=LINE('',#61769,#14729);
#9855=LINE('',#61771,#14730);
#9856=LINE('',#61772,#14731);
#9857=LINE('',#61775,#14732);
#9858=LINE('',#61777,#14733);
#9859=LINE('',#61779,#14734);
#9860=LINE('',#61781,#14735);
#9861=LINE('',#61783,#14736);
#9862=LINE('',#61784,#14737);
#9863=LINE('',#61787,#14738);
#9864=LINE('',#61789,#14739);
#9865=LINE('',#61791,#14740);
#9866=LINE('',#61793,#14741);
#9867=LINE('',#61795,#14742);
#9868=LINE('',#61796,#14743);
#9869=LINE('',#61799,#14744);
#9870=LINE('',#61801,#14745);
#9871=LINE('',#61803,#14746);
#9872=LINE('',#61805,#14747);
#9873=LINE('',#61807,#14748);
#9874=LINE('',#61808,#14749);
#9875=LINE('',#61811,#14750);
#9876=LINE('',#61813,#14751);
#9877=LINE('',#61815,#14752);
#9878=LINE('',#61817,#14753);
#9879=LINE('',#61819,#14754);
#9880=LINE('',#61820,#14755);
#9881=LINE('',#61823,#14756);
#9882=LINE('',#61825,#14757);
#9883=LINE('',#61827,#14758);
#9884=LINE('',#61829,#14759);
#9885=LINE('',#61831,#14760);
#9886=LINE('',#61832,#14761);
#9887=LINE('',#61835,#14762);
#9888=LINE('',#61837,#14763);
#9889=LINE('',#61839,#14764);
#9890=LINE('',#61841,#14765);
#9891=LINE('',#61843,#14766);
#9892=LINE('',#61844,#14767);
#9893=LINE('',#61847,#14768);
#9894=LINE('',#61849,#14769);
#9895=LINE('',#61851,#14770);
#9896=LINE('',#61853,#14771);
#9897=LINE('',#61855,#14772);
#9898=LINE('',#61856,#14773);
#9899=LINE('',#61859,#14774);
#9900=LINE('',#61861,#14775);
#9901=LINE('',#61863,#14776);
#9902=LINE('',#61865,#14777);
#9903=LINE('',#61867,#14778);
#9904=LINE('',#61868,#14779);
#9905=LINE('',#61871,#14780);
#9906=LINE('',#61873,#14781);
#9907=LINE('',#61875,#14782);
#9908=LINE('',#61877,#14783);
#9909=LINE('',#61879,#14784);
#9910=LINE('',#61880,#14785);
#9911=LINE('',#61883,#14786);
#9912=LINE('',#61885,#14787);
#9913=LINE('',#61887,#14788);
#9914=LINE('',#61889,#14789);
#9915=LINE('',#61891,#14790);
#9916=LINE('',#61892,#14791);
#9917=LINE('',#61895,#14792);
#9918=LINE('',#61897,#14793);
#9919=LINE('',#61899,#14794);
#9920=LINE('',#61901,#14795);
#9921=LINE('',#61903,#14796);
#9922=LINE('',#61904,#14797);
#9923=LINE('',#61907,#14798);
#9924=LINE('',#61909,#14799);
#9925=LINE('',#61911,#14800);
#9926=LINE('',#61913,#14801);
#9927=LINE('',#61915,#14802);
#9928=LINE('',#61916,#14803);
#9929=LINE('',#61919,#14804);
#9930=LINE('',#61921,#14805);
#9931=LINE('',#61923,#14806);
#9932=LINE('',#61925,#14807);
#9933=LINE('',#61927,#14808);
#9934=LINE('',#61928,#14809);
#9935=LINE('',#61931,#14810);
#9936=LINE('',#61933,#14811);
#9937=LINE('',#61935,#14812);
#9938=LINE('',#61937,#14813);
#9939=LINE('',#61939,#14814);
#9940=LINE('',#61940,#14815);
#9941=LINE('',#61943,#14816);
#9942=LINE('',#61945,#14817);
#9943=LINE('',#61947,#14818);
#9944=LINE('',#61949,#14819);
#9945=LINE('',#61951,#14820);
#9946=LINE('',#61952,#14821);
#9947=LINE('',#61955,#14822);
#9948=LINE('',#61957,#14823);
#9949=LINE('',#61959,#14824);
#9950=LINE('',#61961,#14825);
#9951=LINE('',#61963,#14826);
#9952=LINE('',#61964,#14827);
#9953=LINE('',#61967,#14828);
#9954=LINE('',#61969,#14829);
#9955=LINE('',#61971,#14830);
#9956=LINE('',#61973,#14831);
#9957=LINE('',#61975,#14832);
#9958=LINE('',#61976,#14833);
#9959=LINE('',#61979,#14834);
#9960=LINE('',#61981,#14835);
#9961=LINE('',#61983,#14836);
#9962=LINE('',#61985,#14837);
#9963=LINE('',#61987,#14838);
#9964=LINE('',#61988,#14839);
#9965=LINE('',#61991,#14840);
#9966=LINE('',#61993,#14841);
#9967=LINE('',#61995,#14842);
#9968=LINE('',#61997,#14843);
#9969=LINE('',#61999,#14844);
#9970=LINE('',#62000,#14845);
#9971=LINE('',#62003,#14846);
#9972=LINE('',#62005,#14847);
#9973=LINE('',#62007,#14848);
#9974=LINE('',#62009,#14849);
#9975=LINE('',#62011,#14850);
#9976=LINE('',#62012,#14851);
#9977=LINE('',#62015,#14852);
#9978=LINE('',#62017,#14853);
#9979=LINE('',#62019,#14854);
#9980=LINE('',#62021,#14855);
#9981=LINE('',#62023,#14856);
#9982=LINE('',#62024,#14857);
#9983=LINE('',#62027,#14858);
#9984=LINE('',#62029,#14859);
#9985=LINE('',#62031,#14860);
#9986=LINE('',#62033,#14861);
#9987=LINE('',#62035,#14862);
#9988=LINE('',#62036,#14863);
#9989=LINE('',#62039,#14864);
#9990=LINE('',#62041,#14865);
#9991=LINE('',#62043,#14866);
#9992=LINE('',#62045,#14867);
#9993=LINE('',#62047,#14868);
#9994=LINE('',#62048,#14869);
#9995=LINE('',#62051,#14870);
#9996=LINE('',#62053,#14871);
#9997=LINE('',#62055,#14872);
#9998=LINE('',#62057,#14873);
#9999=LINE('',#62059,#14874);
#10000=LINE('',#62060,#14875);
#10001=LINE('',#62063,#14876);
#10002=LINE('',#62065,#14877);
#10003=LINE('',#62067,#14878);
#10004=LINE('',#62069,#14879);
#10005=LINE('',#62071,#14880);
#10006=LINE('',#62072,#14881);
#10007=LINE('',#62075,#14882);
#10008=LINE('',#62077,#14883);
#10009=LINE('',#62079,#14884);
#10010=LINE('',#62081,#14885);
#10011=LINE('',#62083,#14886);
#10012=LINE('',#62084,#14887);
#10013=LINE('',#62087,#14888);
#10014=LINE('',#62089,#14889);
#10015=LINE('',#62091,#14890);
#10016=LINE('',#62093,#14891);
#10017=LINE('',#62095,#14892);
#10018=LINE('',#62096,#14893);
#10019=LINE('',#62099,#14894);
#10020=LINE('',#62101,#14895);
#10021=LINE('',#62103,#14896);
#10022=LINE('',#62105,#14897);
#10023=LINE('',#62107,#14898);
#10024=LINE('',#62108,#14899);
#10025=LINE('',#62111,#14900);
#10026=LINE('',#62113,#14901);
#10027=LINE('',#62115,#14902);
#10028=LINE('',#62117,#14903);
#10029=LINE('',#62119,#14904);
#10030=LINE('',#62120,#14905);
#10031=LINE('',#62123,#14906);
#10032=LINE('',#62125,#14907);
#10033=LINE('',#62127,#14908);
#10034=LINE('',#62129,#14909);
#10035=LINE('',#62131,#14910);
#10036=LINE('',#62132,#14911);
#10037=LINE('',#62135,#14912);
#10038=LINE('',#62137,#14913);
#10039=LINE('',#62139,#14914);
#10040=LINE('',#62141,#14915);
#10041=LINE('',#62143,#14916);
#10042=LINE('',#62144,#14917);
#10043=LINE('',#62147,#14918);
#10044=LINE('',#62149,#14919);
#10045=LINE('',#62151,#14920);
#10046=LINE('',#62153,#14921);
#10047=LINE('',#62155,#14922);
#10048=LINE('',#62156,#14923);
#10049=LINE('',#62159,#14924);
#10050=LINE('',#62161,#14925);
#10051=LINE('',#62163,#14926);
#10052=LINE('',#62165,#14927);
#10053=LINE('',#62167,#14928);
#10054=LINE('',#62168,#14929);
#10055=LINE('',#62171,#14930);
#10056=LINE('',#62173,#14931);
#10057=LINE('',#62175,#14932);
#10058=LINE('',#62177,#14933);
#10059=LINE('',#62179,#14934);
#10060=LINE('',#62180,#14935);
#10061=LINE('',#62183,#14936);
#10062=LINE('',#62185,#14937);
#10063=LINE('',#62187,#14938);
#10064=LINE('',#62189,#14939);
#10065=LINE('',#62191,#14940);
#10066=LINE('',#62192,#14941);
#10067=LINE('',#62195,#14942);
#10068=LINE('',#62197,#14943);
#10069=LINE('',#62199,#14944);
#10070=LINE('',#62201,#14945);
#10071=LINE('',#62203,#14946);
#10072=LINE('',#62204,#14947);
#10073=LINE('',#62207,#14948);
#10074=LINE('',#62209,#14949);
#10075=LINE('',#62211,#14950);
#10076=LINE('',#62213,#14951);
#10077=LINE('',#62215,#14952);
#10078=LINE('',#62216,#14953);
#10079=LINE('',#62219,#14954);
#10080=LINE('',#62221,#14955);
#10081=LINE('',#62223,#14956);
#10082=LINE('',#62225,#14957);
#10083=LINE('',#62227,#14958);
#10084=LINE('',#62228,#14959);
#10085=LINE('',#62231,#14960);
#10086=LINE('',#62233,#14961);
#10087=LINE('',#62235,#14962);
#10088=LINE('',#62237,#14963);
#10089=LINE('',#62239,#14964);
#10090=LINE('',#62240,#14965);
#10091=LINE('',#62243,#14966);
#10092=LINE('',#62245,#14967);
#10093=LINE('',#62247,#14968);
#10094=LINE('',#62249,#14969);
#10095=LINE('',#62251,#14970);
#10096=LINE('',#62252,#14971);
#10097=LINE('',#62255,#14972);
#10098=LINE('',#62257,#14973);
#10099=LINE('',#62259,#14974);
#10100=LINE('',#62261,#14975);
#10101=LINE('',#62263,#14976);
#10102=LINE('',#62264,#14977);
#10103=LINE('',#62267,#14978);
#10104=LINE('',#62269,#14979);
#10105=LINE('',#62271,#14980);
#10106=LINE('',#62273,#14981);
#10107=LINE('',#62275,#14982);
#10108=LINE('',#62276,#14983);
#10109=LINE('',#62279,#14984);
#10110=LINE('',#62281,#14985);
#10111=LINE('',#62283,#14986);
#10112=LINE('',#62285,#14987);
#10113=LINE('',#62287,#14988);
#10114=LINE('',#62288,#14989);
#10115=LINE('',#62291,#14990);
#10116=LINE('',#62293,#14991);
#10117=LINE('',#62295,#14992);
#10118=LINE('',#62297,#14993);
#10119=LINE('',#62299,#14994);
#10120=LINE('',#62300,#14995);
#10121=LINE('',#62303,#14996);
#10122=LINE('',#62305,#14997);
#10123=LINE('',#62307,#14998);
#10124=LINE('',#62309,#14999);
#10125=LINE('',#62311,#15000);
#10126=LINE('',#62312,#15001);
#10127=LINE('',#62315,#15002);
#10128=LINE('',#62317,#15003);
#10129=LINE('',#62319,#15004);
#10130=LINE('',#62321,#15005);
#10131=LINE('',#62323,#15006);
#10132=LINE('',#62324,#15007);
#10133=LINE('',#62327,#15008);
#10134=LINE('',#62329,#15009);
#10135=LINE('',#62331,#15010);
#10136=LINE('',#62333,#15011);
#10137=LINE('',#62335,#15012);
#10138=LINE('',#62336,#15013);
#10139=LINE('',#62339,#15014);
#10140=LINE('',#62341,#15015);
#10141=LINE('',#62343,#15016);
#10142=LINE('',#62345,#15017);
#10143=LINE('',#62347,#15018);
#10144=LINE('',#62348,#15019);
#10145=LINE('',#62351,#15020);
#10146=LINE('',#62353,#15021);
#10147=LINE('',#62355,#15022);
#10148=LINE('',#62357,#15023);
#10149=LINE('',#62359,#15024);
#10150=LINE('',#62360,#15025);
#10151=LINE('',#62363,#15026);
#10152=LINE('',#62365,#15027);
#10153=LINE('',#62367,#15028);
#10154=LINE('',#62369,#15029);
#10155=LINE('',#62371,#15030);
#10156=LINE('',#62372,#15031);
#10157=LINE('',#62375,#15032);
#10158=LINE('',#62377,#15033);
#10159=LINE('',#62379,#15034);
#10160=LINE('',#62381,#15035);
#10161=LINE('',#62383,#15036);
#10162=LINE('',#62384,#15037);
#10163=LINE('',#62387,#15038);
#10164=LINE('',#62389,#15039);
#10165=LINE('',#62391,#15040);
#10166=LINE('',#62393,#15041);
#10167=LINE('',#62395,#15042);
#10168=LINE('',#62396,#15043);
#10169=LINE('',#62399,#15044);
#10170=LINE('',#62401,#15045);
#10171=LINE('',#62403,#15046);
#10172=LINE('',#62405,#15047);
#10173=LINE('',#62407,#15048);
#10174=LINE('',#62408,#15049);
#10175=LINE('',#62411,#15050);
#10176=LINE('',#62413,#15051);
#10177=LINE('',#62415,#15052);
#10178=LINE('',#62417,#15053);
#10179=LINE('',#62419,#15054);
#10180=LINE('',#62420,#15055);
#10181=LINE('',#62423,#15056);
#10182=LINE('',#62425,#15057);
#10183=LINE('',#62427,#15058);
#10184=LINE('',#62429,#15059);
#10185=LINE('',#62431,#15060);
#10186=LINE('',#62432,#15061);
#10187=LINE('',#62435,#15062);
#10188=LINE('',#62437,#15063);
#10189=LINE('',#62439,#15064);
#10190=LINE('',#62441,#15065);
#10191=LINE('',#62443,#15066);
#10192=LINE('',#62444,#15067);
#10193=LINE('',#62447,#15068);
#10194=LINE('',#62449,#15069);
#10195=LINE('',#62451,#15070);
#10196=LINE('',#62453,#15071);
#10197=LINE('',#62455,#15072);
#10198=LINE('',#62456,#15073);
#10199=LINE('',#62459,#15074);
#10200=LINE('',#62461,#15075);
#10201=LINE('',#62463,#15076);
#10202=LINE('',#62465,#15077);
#10203=LINE('',#62467,#15078);
#10204=LINE('',#62468,#15079);
#10205=LINE('',#62471,#15080);
#10206=LINE('',#62473,#15081);
#10207=LINE('',#62475,#15082);
#10208=LINE('',#62477,#15083);
#10209=LINE('',#62479,#15084);
#10210=LINE('',#62480,#15085);
#10211=LINE('',#62483,#15086);
#10212=LINE('',#62485,#15087);
#10213=LINE('',#62487,#15088);
#10214=LINE('',#62489,#15089);
#10215=LINE('',#62491,#15090);
#10216=LINE('',#62492,#15091);
#10217=LINE('',#62495,#15092);
#10218=LINE('',#62497,#15093);
#10219=LINE('',#62499,#15094);
#10220=LINE('',#62501,#15095);
#10221=LINE('',#62503,#15096);
#10222=LINE('',#62504,#15097);
#10223=LINE('',#62507,#15098);
#10224=LINE('',#62509,#15099);
#10225=LINE('',#62511,#15100);
#10226=LINE('',#62513,#15101);
#10227=LINE('',#62515,#15102);
#10228=LINE('',#62516,#15103);
#10229=LINE('',#62519,#15104);
#10230=LINE('',#62521,#15105);
#10231=LINE('',#62523,#15106);
#10232=LINE('',#62525,#15107);
#10233=LINE('',#62527,#15108);
#10234=LINE('',#62528,#15109);
#10235=LINE('',#62531,#15110);
#10236=LINE('',#62533,#15111);
#10237=LINE('',#62535,#15112);
#10238=LINE('',#62537,#15113);
#10239=LINE('',#62539,#15114);
#10240=LINE('',#62540,#15115);
#10241=LINE('',#62543,#15116);
#10242=LINE('',#62545,#15117);
#10243=LINE('',#62547,#15118);
#10244=LINE('',#62549,#15119);
#10245=LINE('',#62551,#15120);
#10246=LINE('',#62552,#15121);
#10247=LINE('',#62555,#15122);
#10248=LINE('',#62557,#15123);
#10249=LINE('',#62559,#15124);
#10250=LINE('',#62561,#15125);
#10251=LINE('',#62563,#15126);
#10252=LINE('',#62564,#15127);
#10253=LINE('',#62567,#15128);
#10254=LINE('',#62569,#15129);
#10255=LINE('',#62571,#15130);
#10256=LINE('',#62573,#15131);
#10257=LINE('',#62575,#15132);
#10258=LINE('',#62576,#15133);
#10259=LINE('',#62579,#15134);
#10260=LINE('',#62581,#15135);
#10261=LINE('',#62583,#15136);
#10262=LINE('',#62585,#15137);
#10263=LINE('',#62587,#15138);
#10264=LINE('',#62588,#15139);
#10265=LINE('',#62591,#15140);
#10266=LINE('',#62593,#15141);
#10267=LINE('',#62595,#15142);
#10268=LINE('',#62597,#15143);
#10269=LINE('',#62599,#15144);
#10270=LINE('',#62600,#15145);
#10271=LINE('',#62603,#15146);
#10272=LINE('',#62605,#15147);
#10273=LINE('',#62607,#15148);
#10274=LINE('',#62609,#15149);
#10275=LINE('',#62611,#15150);
#10276=LINE('',#62612,#15151);
#10277=LINE('',#62615,#15152);
#10278=LINE('',#62617,#15153);
#10279=LINE('',#62619,#15154);
#10280=LINE('',#62621,#15155);
#10281=LINE('',#62623,#15156);
#10282=LINE('',#62624,#15157);
#10283=LINE('',#62627,#15158);
#10284=LINE('',#62629,#15159);
#10285=LINE('',#62631,#15160);
#10286=LINE('',#62633,#15161);
#10287=LINE('',#62635,#15162);
#10288=LINE('',#62636,#15163);
#10289=LINE('',#62639,#15164);
#10290=LINE('',#62641,#15165);
#10291=LINE('',#62643,#15166);
#10292=LINE('',#62645,#15167);
#10293=LINE('',#62647,#15168);
#10294=LINE('',#62648,#15169);
#10295=LINE('',#62651,#15170);
#10296=LINE('',#62653,#15171);
#10297=LINE('',#62655,#15172);
#10298=LINE('',#62657,#15173);
#10299=LINE('',#62659,#15174);
#10300=LINE('',#62660,#15175);
#10301=LINE('',#62663,#15176);
#10302=LINE('',#62665,#15177);
#10303=LINE('',#62667,#15178);
#10304=LINE('',#62669,#15179);
#10305=LINE('',#62671,#15180);
#10306=LINE('',#62672,#15181);
#10307=LINE('',#62675,#15182);
#10308=LINE('',#62677,#15183);
#10309=LINE('',#62679,#15184);
#10310=LINE('',#62681,#15185);
#10311=LINE('',#62683,#15186);
#10312=LINE('',#62684,#15187);
#10313=LINE('',#62687,#15188);
#10314=LINE('',#62689,#15189);
#10315=LINE('',#62691,#15190);
#10316=LINE('',#62693,#15191);
#10317=LINE('',#62695,#15192);
#10318=LINE('',#62696,#15193);
#10319=LINE('',#62699,#15194);
#10320=LINE('',#62701,#15195);
#10321=LINE('',#62703,#15196);
#10322=LINE('',#62705,#15197);
#10323=LINE('',#62707,#15198);
#10324=LINE('',#62708,#15199);
#10325=LINE('',#62711,#15200);
#10326=LINE('',#62713,#15201);
#10327=LINE('',#62715,#15202);
#10328=LINE('',#62717,#15203);
#10329=LINE('',#62719,#15204);
#10330=LINE('',#62720,#15205);
#10331=LINE('',#62723,#15206);
#10332=LINE('',#62725,#15207);
#10333=LINE('',#62727,#15208);
#10334=LINE('',#62729,#15209);
#10335=LINE('',#62731,#15210);
#10336=LINE('',#62732,#15211);
#10337=LINE('',#62735,#15212);
#10338=LINE('',#62737,#15213);
#10339=LINE('',#62739,#15214);
#10340=LINE('',#62741,#15215);
#10341=LINE('',#62743,#15216);
#10342=LINE('',#62744,#15217);
#10343=LINE('',#62747,#15218);
#10344=LINE('',#62749,#15219);
#10345=LINE('',#62751,#15220);
#10346=LINE('',#62753,#15221);
#10347=LINE('',#62755,#15222);
#10348=LINE('',#62756,#15223);
#10349=LINE('',#62759,#15224);
#10350=LINE('',#62761,#15225);
#10351=LINE('',#62763,#15226);
#10352=LINE('',#62765,#15227);
#10353=LINE('',#62767,#15228);
#10354=LINE('',#62768,#15229);
#10355=LINE('',#62771,#15230);
#10356=LINE('',#62773,#15231);
#10357=LINE('',#62775,#15232);
#10358=LINE('',#62777,#15233);
#10359=LINE('',#62779,#15234);
#10360=LINE('',#62780,#15235);
#10361=LINE('',#62783,#15236);
#10362=LINE('',#62785,#15237);
#10363=LINE('',#62787,#15238);
#10364=LINE('',#62789,#15239);
#10365=LINE('',#62791,#15240);
#10366=LINE('',#62792,#15241);
#10367=LINE('',#62795,#15242);
#10368=LINE('',#62797,#15243);
#10369=LINE('',#62799,#15244);
#10370=LINE('',#62801,#15245);
#10371=LINE('',#62803,#15246);
#10372=LINE('',#62804,#15247);
#10373=LINE('',#62807,#15248);
#10374=LINE('',#62809,#15249);
#10375=LINE('',#62811,#15250);
#10376=LINE('',#62813,#15251);
#10377=LINE('',#62815,#15252);
#10378=LINE('',#62816,#15253);
#10379=LINE('',#62819,#15254);
#10380=LINE('',#62821,#15255);
#10381=LINE('',#62823,#15256);
#10382=LINE('',#62825,#15257);
#10383=LINE('',#62827,#15258);
#10384=LINE('',#62828,#15259);
#10385=LINE('',#62831,#15260);
#10386=LINE('',#62833,#15261);
#10387=LINE('',#62835,#15262);
#10388=LINE('',#62837,#15263);
#10389=LINE('',#62839,#15264);
#10390=LINE('',#62840,#15265);
#10391=LINE('',#62843,#15266);
#10392=LINE('',#62845,#15267);
#10393=LINE('',#62847,#15268);
#10394=LINE('',#62849,#15269);
#10395=LINE('',#62851,#15270);
#10396=LINE('',#62852,#15271);
#10397=LINE('',#62855,#15272);
#10398=LINE('',#62857,#15273);
#10399=LINE('',#62859,#15274);
#10400=LINE('',#62861,#15275);
#10401=LINE('',#62863,#15276);
#10402=LINE('',#62864,#15277);
#10403=LINE('',#62867,#15278);
#10404=LINE('',#62869,#15279);
#10405=LINE('',#62871,#15280);
#10406=LINE('',#62873,#15281);
#10407=LINE('',#62875,#15282);
#10408=LINE('',#62876,#15283);
#10409=LINE('',#62879,#15284);
#10410=LINE('',#62881,#15285);
#10411=LINE('',#62883,#15286);
#10412=LINE('',#62885,#15287);
#10413=LINE('',#62887,#15288);
#10414=LINE('',#62888,#15289);
#10415=LINE('',#62891,#15290);
#10416=LINE('',#62893,#15291);
#10417=LINE('',#62895,#15292);
#10418=LINE('',#62897,#15293);
#10419=LINE('',#62899,#15294);
#10420=LINE('',#62900,#15295);
#10421=LINE('',#62903,#15296);
#10422=LINE('',#62905,#15297);
#10423=LINE('',#62907,#15298);
#10424=LINE('',#62909,#15299);
#10425=LINE('',#62911,#15300);
#10426=LINE('',#62912,#15301);
#10427=LINE('',#62915,#15302);
#10428=LINE('',#62917,#15303);
#10429=LINE('',#62919,#15304);
#10430=LINE('',#62921,#15305);
#10431=LINE('',#62923,#15306);
#10432=LINE('',#62924,#15307);
#10433=LINE('',#62927,#15308);
#10434=LINE('',#62929,#15309);
#10435=LINE('',#62931,#15310);
#10436=LINE('',#62933,#15311);
#10437=LINE('',#62935,#15312);
#10438=LINE('',#62936,#15313);
#10439=LINE('',#62939,#15314);
#10440=LINE('',#62941,#15315);
#10441=LINE('',#62943,#15316);
#10442=LINE('',#62945,#15317);
#10443=LINE('',#62947,#15318);
#10444=LINE('',#62948,#15319);
#10445=LINE('',#62951,#15320);
#10446=LINE('',#62953,#15321);
#10447=LINE('',#62955,#15322);
#10448=LINE('',#62957,#15323);
#10449=LINE('',#62959,#15324);
#10450=LINE('',#62960,#15325);
#10451=LINE('',#62963,#15326);
#10452=LINE('',#62965,#15327);
#10453=LINE('',#62967,#15328);
#10454=LINE('',#62969,#15329);
#10455=LINE('',#62971,#15330);
#10456=LINE('',#62972,#15331);
#10457=LINE('',#62975,#15332);
#10458=LINE('',#62977,#15333);
#10459=LINE('',#62979,#15334);
#10460=LINE('',#62981,#15335);
#10461=LINE('',#62983,#15336);
#10462=LINE('',#62984,#15337);
#10463=LINE('',#62987,#15338);
#10464=LINE('',#62989,#15339);
#10465=LINE('',#62991,#15340);
#10466=LINE('',#62993,#15341);
#10467=LINE('',#62995,#15342);
#10468=LINE('',#62996,#15343);
#10469=LINE('',#62999,#15344);
#10470=LINE('',#63001,#15345);
#10471=LINE('',#63003,#15346);
#10472=LINE('',#63005,#15347);
#10473=LINE('',#63007,#15348);
#10474=LINE('',#63008,#15349);
#10475=LINE('',#63011,#15350);
#10476=LINE('',#63013,#15351);
#10477=LINE('',#63015,#15352);
#10478=LINE('',#63017,#15353);
#10479=LINE('',#63019,#15354);
#10480=LINE('',#63020,#15355);
#10481=LINE('',#63023,#15356);
#10482=LINE('',#63025,#15357);
#10483=LINE('',#63027,#15358);
#10484=LINE('',#63029,#15359);
#10485=LINE('',#63031,#15360);
#10486=LINE('',#63032,#15361);
#10487=LINE('',#63035,#15362);
#10488=LINE('',#63037,#15363);
#10489=LINE('',#63039,#15364);
#10490=LINE('',#63041,#15365);
#10491=LINE('',#63043,#15366);
#10492=LINE('',#63044,#15367);
#10493=LINE('',#63047,#15368);
#10494=LINE('',#63049,#15369);
#10495=LINE('',#63051,#15370);
#10496=LINE('',#63053,#15371);
#10497=LINE('',#63055,#15372);
#10498=LINE('',#63056,#15373);
#10499=LINE('',#63058,#15374);
#10500=LINE('',#63059,#15375);
#10501=LINE('',#63061,#15376);
#10502=LINE('',#63063,#15377);
#10503=LINE('',#63065,#15378);
#10504=LINE('',#63067,#15379);
#10505=LINE('',#63070,#15380);
#10506=LINE('',#63071,#15381);
#10507=LINE('',#63073,#15382);
#10508=LINE('',#63075,#15383);
#10509=LINE('',#63077,#15384);
#10510=LINE('',#63079,#15385);
#10511=LINE('',#63082,#15386);
#10512=LINE('',#63083,#15387);
#10513=LINE('',#63085,#15388);
#10514=LINE('',#63087,#15389);
#10515=LINE('',#63089,#15390);
#10516=LINE('',#63091,#15391);
#10517=LINE('',#63094,#15392);
#10518=LINE('',#63095,#15393);
#10519=LINE('',#63097,#15394);
#10520=LINE('',#63099,#15395);
#10521=LINE('',#63101,#15396);
#10522=LINE('',#63103,#15397);
#10523=LINE('',#63106,#15398);
#10524=LINE('',#63107,#15399);
#10525=LINE('',#63109,#15400);
#10526=LINE('',#63111,#15401);
#10527=LINE('',#63113,#15402);
#10528=LINE('',#63115,#15403);
#10529=LINE('',#63118,#15404);
#10530=LINE('',#63119,#15405);
#10531=LINE('',#63121,#15406);
#10532=LINE('',#63123,#15407);
#10533=LINE('',#63125,#15408);
#10534=LINE('',#63127,#15409);
#10535=LINE('',#63130,#15410);
#10536=LINE('',#63131,#15411);
#10537=LINE('',#63133,#15412);
#10538=LINE('',#63135,#15413);
#10539=LINE('',#63137,#15414);
#10540=LINE('',#63139,#15415);
#10541=LINE('',#63142,#15416);
#10542=LINE('',#63143,#15417);
#10543=LINE('',#63145,#15418);
#10544=LINE('',#63147,#15419);
#10545=LINE('',#63149,#15420);
#10546=LINE('',#63151,#15421);
#10547=LINE('',#63154,#15422);
#10548=LINE('',#63155,#15423);
#10549=LINE('',#63157,#15424);
#10550=LINE('',#63159,#15425);
#10551=LINE('',#63161,#15426);
#10552=LINE('',#63163,#15427);
#10553=LINE('',#63166,#15428);
#10554=LINE('',#63167,#15429);
#10555=LINE('',#63169,#15430);
#10556=LINE('',#63171,#15431);
#10557=LINE('',#63173,#15432);
#10558=LINE('',#63175,#15433);
#10559=LINE('',#63178,#15434);
#10560=LINE('',#63179,#15435);
#10561=LINE('',#63181,#15436);
#10562=LINE('',#63183,#15437);
#10563=LINE('',#63185,#15438);
#10564=LINE('',#63187,#15439);
#10565=LINE('',#63190,#15440);
#10566=LINE('',#63191,#15441);
#10567=LINE('',#63193,#15442);
#10568=LINE('',#63195,#15443);
#10569=LINE('',#63197,#15444);
#10570=LINE('',#63199,#15445);
#10571=LINE('',#63202,#15446);
#10572=LINE('',#63203,#15447);
#10573=LINE('',#63205,#15448);
#10574=LINE('',#63207,#15449);
#10575=LINE('',#63209,#15450);
#10576=LINE('',#63211,#15451);
#10577=LINE('',#63214,#15452);
#10578=LINE('',#63215,#15453);
#10579=LINE('',#63217,#15454);
#10580=LINE('',#63219,#15455);
#10581=LINE('',#63221,#15456);
#10582=LINE('',#63223,#15457);
#10583=LINE('',#63226,#15458);
#10584=LINE('',#63227,#15459);
#10585=LINE('',#63229,#15460);
#10586=LINE('',#63231,#15461);
#10587=LINE('',#63233,#15462);
#10588=LINE('',#63235,#15463);
#10589=LINE('',#63238,#15464);
#10590=LINE('',#63239,#15465);
#10591=LINE('',#63241,#15466);
#10592=LINE('',#63243,#15467);
#10593=LINE('',#63245,#15468);
#10594=LINE('',#63247,#15469);
#10595=LINE('',#63250,#15470);
#10596=LINE('',#63251,#15471);
#10597=LINE('',#63253,#15472);
#10598=LINE('',#63255,#15473);
#10599=LINE('',#63257,#15474);
#10600=LINE('',#63259,#15475);
#10601=LINE('',#63262,#15476);
#10602=LINE('',#63263,#15477);
#10603=LINE('',#63265,#15478);
#10604=LINE('',#63267,#15479);
#10605=LINE('',#63269,#15480);
#10606=LINE('',#63271,#15481);
#10607=LINE('',#63274,#15482);
#10608=LINE('',#63275,#15483);
#10609=LINE('',#63277,#15484);
#10610=LINE('',#63279,#15485);
#10611=LINE('',#63281,#15486);
#10612=LINE('',#63283,#15487);
#10613=LINE('',#63286,#15488);
#10614=LINE('',#63287,#15489);
#10615=LINE('',#63289,#15490);
#10616=LINE('',#63291,#15491);
#10617=LINE('',#63293,#15492);
#10618=LINE('',#63295,#15493);
#10619=LINE('',#63298,#15494);
#10620=LINE('',#63299,#15495);
#10621=LINE('',#63301,#15496);
#10622=LINE('',#63303,#15497);
#10623=LINE('',#63305,#15498);
#10624=LINE('',#63307,#15499);
#10625=LINE('',#63310,#15500);
#10626=LINE('',#63311,#15501);
#10627=LINE('',#63313,#15502);
#10628=LINE('',#63315,#15503);
#10629=LINE('',#63317,#15504);
#10630=LINE('',#63319,#15505);
#10631=LINE('',#63322,#15506);
#10632=LINE('',#63323,#15507);
#10633=LINE('',#63325,#15508);
#10634=LINE('',#63327,#15509);
#10635=LINE('',#63329,#15510);
#10636=LINE('',#63331,#15511);
#10637=LINE('',#63334,#15512);
#10638=LINE('',#63335,#15513);
#10639=LINE('',#63337,#15514);
#10640=LINE('',#63339,#15515);
#10641=LINE('',#63341,#15516);
#10642=LINE('',#63343,#15517);
#10643=LINE('',#63346,#15518);
#10644=LINE('',#63347,#15519);
#10645=LINE('',#63349,#15520);
#10646=LINE('',#63351,#15521);
#10647=LINE('',#63353,#15522);
#10648=LINE('',#63355,#15523);
#10649=LINE('',#63358,#15524);
#10650=LINE('',#63359,#15525);
#10651=LINE('',#63361,#15526);
#10652=LINE('',#63363,#15527);
#10653=LINE('',#63365,#15528);
#10654=LINE('',#63367,#15529);
#10655=LINE('',#63370,#15530);
#10656=LINE('',#63371,#15531);
#10657=LINE('',#63373,#15532);
#10658=LINE('',#63375,#15533);
#10659=LINE('',#63377,#15534);
#10660=LINE('',#63379,#15535);
#10661=LINE('',#63382,#15536);
#10662=LINE('',#63383,#15537);
#10663=LINE('',#63385,#15538);
#10664=LINE('',#63387,#15539);
#10665=LINE('',#63389,#15540);
#10666=LINE('',#63391,#15541);
#10667=LINE('',#63394,#15542);
#10668=LINE('',#63395,#15543);
#10669=LINE('',#63397,#15544);
#10670=LINE('',#63399,#15545);
#10671=LINE('',#63401,#15546);
#10672=LINE('',#63403,#15547);
#10673=LINE('',#63406,#15548);
#10674=LINE('',#63407,#15549);
#10675=LINE('',#63409,#15550);
#10676=LINE('',#63411,#15551);
#10677=LINE('',#63413,#15552);
#10678=LINE('',#63415,#15553);
#10679=LINE('',#63418,#15554);
#10680=LINE('',#63419,#15555);
#10681=LINE('',#63421,#15556);
#10682=LINE('',#63423,#15557);
#10683=LINE('',#63425,#15558);
#10684=LINE('',#63427,#15559);
#10685=LINE('',#63430,#15560);
#10686=LINE('',#63431,#15561);
#10687=LINE('',#63433,#15562);
#10688=LINE('',#63435,#15563);
#10689=LINE('',#63437,#15564);
#10690=LINE('',#63439,#15565);
#10691=LINE('',#63442,#15566);
#10692=LINE('',#63443,#15567);
#10693=LINE('',#63445,#15568);
#10694=LINE('',#63447,#15569);
#10695=LINE('',#63449,#15570);
#10696=LINE('',#63451,#15571);
#10697=LINE('',#63454,#15572);
#10698=LINE('',#63455,#15573);
#10699=LINE('',#63457,#15574);
#10700=LINE('',#63459,#15575);
#10701=LINE('',#63461,#15576);
#10702=LINE('',#63463,#15577);
#10703=LINE('',#63466,#15578);
#10704=LINE('',#63467,#15579);
#10705=LINE('',#63469,#15580);
#10706=LINE('',#63471,#15581);
#10707=LINE('',#63473,#15582);
#10708=LINE('',#63475,#15583);
#10709=LINE('',#63478,#15584);
#10710=LINE('',#63479,#15585);
#10711=LINE('',#63481,#15586);
#10712=LINE('',#63483,#15587);
#10713=LINE('',#63485,#15588);
#10714=LINE('',#63487,#15589);
#10715=LINE('',#63490,#15590);
#10716=LINE('',#63491,#15591);
#10717=LINE('',#63493,#15592);
#10718=LINE('',#63495,#15593);
#10719=LINE('',#63497,#15594);
#10720=LINE('',#63499,#15595);
#10721=LINE('',#63502,#15596);
#10722=LINE('',#63503,#15597);
#10723=LINE('',#63505,#15598);
#10724=LINE('',#63507,#15599);
#10725=LINE('',#63509,#15600);
#10726=LINE('',#63511,#15601);
#10727=LINE('',#63514,#15602);
#10728=LINE('',#63515,#15603);
#10729=LINE('',#63517,#15604);
#10730=LINE('',#63519,#15605);
#10731=LINE('',#63521,#15606);
#10732=LINE('',#63523,#15607);
#10733=LINE('',#63526,#15608);
#10734=LINE('',#63527,#15609);
#10735=LINE('',#63529,#15610);
#10736=LINE('',#63531,#15611);
#10737=LINE('',#63533,#15612);
#10738=LINE('',#63535,#15613);
#10739=LINE('',#63538,#15614);
#10740=LINE('',#63539,#15615);
#10741=LINE('',#63541,#15616);
#10742=LINE('',#63543,#15617);
#10743=LINE('',#63545,#15618);
#10744=LINE('',#63547,#15619);
#10745=LINE('',#63550,#15620);
#10746=LINE('',#63551,#15621);
#10747=LINE('',#63553,#15622);
#10748=LINE('',#63555,#15623);
#10749=LINE('',#63557,#15624);
#10750=LINE('',#63559,#15625);
#10751=LINE('',#63562,#15626);
#10752=LINE('',#63563,#15627);
#10753=LINE('',#63565,#15628);
#10754=LINE('',#63567,#15629);
#10755=LINE('',#63569,#15630);
#10756=LINE('',#63571,#15631);
#10757=LINE('',#63574,#15632);
#10758=LINE('',#63575,#15633);
#10759=LINE('',#63577,#15634);
#10760=LINE('',#63579,#15635);
#10761=LINE('',#63581,#15636);
#10762=LINE('',#63583,#15637);
#10763=LINE('',#63586,#15638);
#10764=LINE('',#63587,#15639);
#10765=LINE('',#63589,#15640);
#10766=LINE('',#63591,#15641);
#10767=LINE('',#63593,#15642);
#10768=LINE('',#63595,#15643);
#10769=LINE('',#63598,#15644);
#10770=LINE('',#63599,#15645);
#10771=LINE('',#63601,#15646);
#10772=LINE('',#63603,#15647);
#10773=LINE('',#63605,#15648);
#10774=LINE('',#63607,#15649);
#10775=LINE('',#63610,#15650);
#10776=LINE('',#63611,#15651);
#10777=LINE('',#63613,#15652);
#10778=LINE('',#63615,#15653);
#10779=LINE('',#63617,#15654);
#10780=LINE('',#63619,#15655);
#10781=LINE('',#63622,#15656);
#10782=LINE('',#63623,#15657);
#10783=LINE('',#63625,#15658);
#10784=LINE('',#63627,#15659);
#10785=LINE('',#63629,#15660);
#10786=LINE('',#63631,#15661);
#10787=LINE('',#63634,#15662);
#10788=LINE('',#63635,#15663);
#10789=LINE('',#63637,#15664);
#10790=LINE('',#63639,#15665);
#10791=LINE('',#63641,#15666);
#10792=LINE('',#63643,#15667);
#10793=LINE('',#63646,#15668);
#10794=LINE('',#63647,#15669);
#10795=LINE('',#63649,#15670);
#10796=LINE('',#63651,#15671);
#10797=LINE('',#63653,#15672);
#10798=LINE('',#63655,#15673);
#10799=LINE('',#63658,#15674);
#10800=LINE('',#63659,#15675);
#10801=LINE('',#63661,#15676);
#10802=LINE('',#63663,#15677);
#10803=LINE('',#63665,#15678);
#10804=LINE('',#63667,#15679);
#10805=LINE('',#63670,#15680);
#10806=LINE('',#63671,#15681);
#10807=LINE('',#63673,#15682);
#10808=LINE('',#63675,#15683);
#10809=LINE('',#63677,#15684);
#10810=LINE('',#63679,#15685);
#10811=LINE('',#63682,#15686);
#10812=LINE('',#63683,#15687);
#10813=LINE('',#63685,#15688);
#10814=LINE('',#63687,#15689);
#10815=LINE('',#63689,#15690);
#10816=LINE('',#63691,#15691);
#10817=LINE('',#63694,#15692);
#10818=LINE('',#63695,#15693);
#10819=LINE('',#63697,#15694);
#10820=LINE('',#63699,#15695);
#10821=LINE('',#63701,#15696);
#10822=LINE('',#63703,#15697);
#10823=LINE('',#63706,#15698);
#10824=LINE('',#63707,#15699);
#10825=LINE('',#63709,#15700);
#10826=LINE('',#63711,#15701);
#10827=LINE('',#63713,#15702);
#10828=LINE('',#63715,#15703);
#10829=LINE('',#63718,#15704);
#10830=LINE('',#63719,#15705);
#10831=LINE('',#63721,#15706);
#10832=LINE('',#63723,#15707);
#10833=LINE('',#63725,#15708);
#10834=LINE('',#63727,#15709);
#10835=LINE('',#63730,#15710);
#10836=LINE('',#63731,#15711);
#10837=LINE('',#63733,#15712);
#10838=LINE('',#63735,#15713);
#10839=LINE('',#63737,#15714);
#10840=LINE('',#63739,#15715);
#10841=LINE('',#63742,#15716);
#10842=LINE('',#63743,#15717);
#10843=LINE('',#63745,#15718);
#10844=LINE('',#63747,#15719);
#10845=LINE('',#63749,#15720);
#10846=LINE('',#63751,#15721);
#10847=LINE('',#63754,#15722);
#10848=LINE('',#63755,#15723);
#10849=LINE('',#63757,#15724);
#10850=LINE('',#63759,#15725);
#10851=LINE('',#63761,#15726);
#10852=LINE('',#63763,#15727);
#10853=LINE('',#63766,#15728);
#10854=LINE('',#63767,#15729);
#10855=LINE('',#63769,#15730);
#10856=LINE('',#63771,#15731);
#10857=LINE('',#63773,#15732);
#10858=LINE('',#63775,#15733);
#10859=LINE('',#63778,#15734);
#10860=LINE('',#63779,#15735);
#10861=LINE('',#63781,#15736);
#10862=LINE('',#63783,#15737);
#10863=LINE('',#63785,#15738);
#10864=LINE('',#63787,#15739);
#10865=LINE('',#63790,#15740);
#10866=LINE('',#63791,#15741);
#10867=LINE('',#63793,#15742);
#10868=LINE('',#63795,#15743);
#10869=LINE('',#63797,#15744);
#10870=LINE('',#63799,#15745);
#10871=LINE('',#63802,#15746);
#10872=LINE('',#63803,#15747);
#10873=LINE('',#63805,#15748);
#10874=LINE('',#63807,#15749);
#10875=LINE('',#63809,#15750);
#10876=LINE('',#63811,#15751);
#10877=LINE('',#63814,#15752);
#10878=LINE('',#63815,#15753);
#10879=LINE('',#63817,#15754);
#10880=LINE('',#63819,#15755);
#10881=LINE('',#63821,#15756);
#10882=LINE('',#63823,#15757);
#10883=LINE('',#63826,#15758);
#10884=LINE('',#63827,#15759);
#10885=LINE('',#63829,#15760);
#10886=LINE('',#63831,#15761);
#10887=LINE('',#63833,#15762);
#10888=LINE('',#63835,#15763);
#10889=LINE('',#63838,#15764);
#10890=LINE('',#63839,#15765);
#10891=LINE('',#63841,#15766);
#10892=LINE('',#63843,#15767);
#10893=LINE('',#63845,#15768);
#10894=LINE('',#63847,#15769);
#10895=LINE('',#63850,#15770);
#10896=LINE('',#63851,#15771);
#10897=LINE('',#63853,#15772);
#10898=LINE('',#63855,#15773);
#10899=LINE('',#63857,#15774);
#10900=LINE('',#63859,#15775);
#10901=LINE('',#63862,#15776);
#10902=LINE('',#63863,#15777);
#10903=LINE('',#63865,#15778);
#10904=LINE('',#63867,#15779);
#10905=LINE('',#63869,#15780);
#10906=LINE('',#63871,#15781);
#10907=LINE('',#63874,#15782);
#10908=LINE('',#63875,#15783);
#10909=LINE('',#63877,#15784);
#10910=LINE('',#63879,#15785);
#10911=LINE('',#63881,#15786);
#10912=LINE('',#63883,#15787);
#10913=LINE('',#63886,#15788);
#10914=LINE('',#63887,#15789);
#10915=LINE('',#63889,#15790);
#10916=LINE('',#63891,#15791);
#10917=LINE('',#63893,#15792);
#10918=LINE('',#63895,#15793);
#10919=LINE('',#63898,#15794);
#10920=LINE('',#63899,#15795);
#10921=LINE('',#63901,#15796);
#10922=LINE('',#63903,#15797);
#10923=LINE('',#63905,#15798);
#10924=LINE('',#63907,#15799);
#10925=LINE('',#63910,#15800);
#10926=LINE('',#63911,#15801);
#10927=LINE('',#63913,#15802);
#10928=LINE('',#63915,#15803);
#10929=LINE('',#63917,#15804);
#10930=LINE('',#63919,#15805);
#10931=LINE('',#63922,#15806);
#10932=LINE('',#63923,#15807);
#10933=LINE('',#63925,#15808);
#10934=LINE('',#63927,#15809);
#10935=LINE('',#63929,#15810);
#10936=LINE('',#63931,#15811);
#10937=LINE('',#63934,#15812);
#10938=LINE('',#63935,#15813);
#10939=LINE('',#63937,#15814);
#10940=LINE('',#63939,#15815);
#10941=LINE('',#63941,#15816);
#10942=LINE('',#63943,#15817);
#10943=LINE('',#63946,#15818);
#10944=LINE('',#63947,#15819);
#10945=LINE('',#63949,#15820);
#10946=LINE('',#63951,#15821);
#10947=LINE('',#63953,#15822);
#10948=LINE('',#63955,#15823);
#10949=LINE('',#63958,#15824);
#10950=LINE('',#63959,#15825);
#10951=LINE('',#63961,#15826);
#10952=LINE('',#63963,#15827);
#10953=LINE('',#63965,#15828);
#10954=LINE('',#63967,#15829);
#10955=LINE('',#63970,#15830);
#10956=LINE('',#63971,#15831);
#10957=LINE('',#63973,#15832);
#10958=LINE('',#63975,#15833);
#10959=LINE('',#63977,#15834);
#10960=LINE('',#63979,#15835);
#10961=LINE('',#63982,#15836);
#10962=LINE('',#63983,#15837);
#10963=LINE('',#63985,#15838);
#10964=LINE('',#63987,#15839);
#10965=LINE('',#63989,#15840);
#10966=LINE('',#63991,#15841);
#10967=LINE('',#63994,#15842);
#10968=LINE('',#63995,#15843);
#10969=LINE('',#63997,#15844);
#10970=LINE('',#63999,#15845);
#10971=LINE('',#64001,#15846);
#10972=LINE('',#64003,#15847);
#10973=LINE('',#64006,#15848);
#10974=LINE('',#64007,#15849);
#10975=LINE('',#64009,#15850);
#10976=LINE('',#64011,#15851);
#10977=LINE('',#64013,#15852);
#10978=LINE('',#64015,#15853);
#10979=LINE('',#64018,#15854);
#10980=LINE('',#64019,#15855);
#10981=LINE('',#64021,#15856);
#10982=LINE('',#64023,#15857);
#10983=LINE('',#64025,#15858);
#10984=LINE('',#64027,#15859);
#10985=LINE('',#64030,#15860);
#10986=LINE('',#64031,#15861);
#10987=LINE('',#64033,#15862);
#10988=LINE('',#64035,#15863);
#10989=LINE('',#64037,#15864);
#10990=LINE('',#64039,#15865);
#10991=LINE('',#64042,#15866);
#10992=LINE('',#64043,#15867);
#10993=LINE('',#64045,#15868);
#10994=LINE('',#64047,#15869);
#10995=LINE('',#64049,#15870);
#10996=LINE('',#64051,#15871);
#10997=LINE('',#64054,#15872);
#10998=LINE('',#64055,#15873);
#10999=LINE('',#64057,#15874);
#11000=LINE('',#64059,#15875);
#11001=LINE('',#64061,#15876);
#11002=LINE('',#64063,#15877);
#11003=LINE('',#64066,#15878);
#11004=LINE('',#64067,#15879);
#11005=LINE('',#64069,#15880);
#11006=LINE('',#64071,#15881);
#11007=LINE('',#64073,#15882);
#11008=LINE('',#64075,#15883);
#11009=LINE('',#64078,#15884);
#11010=LINE('',#64079,#15885);
#11011=LINE('',#64081,#15886);
#11012=LINE('',#64083,#15887);
#11013=LINE('',#64085,#15888);
#11014=LINE('',#64087,#15889);
#11015=LINE('',#64090,#15890);
#11016=LINE('',#64091,#15891);
#11017=LINE('',#64093,#15892);
#11018=LINE('',#64095,#15893);
#11019=LINE('',#64097,#15894);
#11020=LINE('',#64099,#15895);
#11021=LINE('',#64102,#15896);
#11022=LINE('',#64103,#15897);
#11023=LINE('',#64105,#15898);
#11024=LINE('',#64107,#15899);
#11025=LINE('',#64109,#15900);
#11026=LINE('',#64111,#15901);
#11027=LINE('',#64114,#15902);
#11028=LINE('',#64115,#15903);
#11029=LINE('',#64117,#15904);
#11030=LINE('',#64119,#15905);
#11031=LINE('',#64121,#15906);
#11032=LINE('',#64123,#15907);
#11033=LINE('',#64126,#15908);
#11034=LINE('',#64127,#15909);
#11035=LINE('',#64129,#15910);
#11036=LINE('',#64131,#15911);
#11037=LINE('',#64133,#15912);
#11038=LINE('',#64135,#15913);
#11039=LINE('',#64138,#15914);
#11040=LINE('',#64139,#15915);
#11041=LINE('',#64141,#15916);
#11042=LINE('',#64143,#15917);
#11043=LINE('',#64145,#15918);
#11044=LINE('',#64147,#15919);
#11045=LINE('',#64150,#15920);
#11046=LINE('',#64151,#15921);
#11047=LINE('',#64153,#15922);
#11048=LINE('',#64155,#15923);
#11049=LINE('',#64157,#15924);
#11050=LINE('',#64159,#15925);
#11051=LINE('',#64162,#15926);
#11052=LINE('',#64163,#15927);
#11053=LINE('',#64165,#15928);
#11054=LINE('',#64167,#15929);
#11055=LINE('',#64169,#15930);
#11056=LINE('',#64171,#15931);
#11057=LINE('',#64174,#15932);
#11058=LINE('',#64175,#15933);
#11059=LINE('',#64177,#15934);
#11060=LINE('',#64179,#15935);
#11061=LINE('',#64181,#15936);
#11062=LINE('',#64183,#15937);
#11063=LINE('',#64186,#15938);
#11064=LINE('',#64187,#15939);
#11065=LINE('',#64189,#15940);
#11066=LINE('',#64191,#15941);
#11067=LINE('',#64193,#15942);
#11068=LINE('',#64195,#15943);
#11069=LINE('',#64198,#15944);
#11070=LINE('',#64199,#15945);
#11071=LINE('',#64201,#15946);
#11072=LINE('',#64203,#15947);
#11073=LINE('',#64205,#15948);
#11074=LINE('',#64207,#15949);
#11075=LINE('',#64210,#15950);
#11076=LINE('',#64211,#15951);
#11077=LINE('',#64213,#15952);
#11078=LINE('',#64215,#15953);
#11079=LINE('',#64217,#15954);
#11080=LINE('',#64219,#15955);
#11081=LINE('',#64222,#15956);
#11082=LINE('',#64223,#15957);
#11083=LINE('',#64225,#15958);
#11084=LINE('',#64227,#15959);
#11085=LINE('',#64229,#15960);
#11086=LINE('',#64231,#15961);
#11087=LINE('',#64234,#15962);
#11088=LINE('',#64235,#15963);
#11089=LINE('',#64237,#15964);
#11090=LINE('',#64239,#15965);
#11091=LINE('',#64241,#15966);
#11092=LINE('',#64243,#15967);
#11093=LINE('',#64246,#15968);
#11094=LINE('',#64247,#15969);
#11095=LINE('',#64249,#15970);
#11096=LINE('',#64251,#15971);
#11097=LINE('',#64253,#15972);
#11098=LINE('',#64255,#15973);
#11099=LINE('',#64258,#15974);
#11100=LINE('',#64259,#15975);
#11101=LINE('',#64261,#15976);
#11102=LINE('',#64263,#15977);
#11103=LINE('',#64265,#15978);
#11104=LINE('',#64267,#15979);
#11105=LINE('',#64270,#15980);
#11106=LINE('',#64271,#15981);
#11107=LINE('',#64273,#15982);
#11108=LINE('',#64275,#15983);
#11109=LINE('',#64277,#15984);
#11110=LINE('',#64279,#15985);
#11111=LINE('',#64282,#15986);
#11112=LINE('',#64283,#15987);
#11113=LINE('',#64285,#15988);
#11114=LINE('',#64287,#15989);
#11115=LINE('',#64289,#15990);
#11116=LINE('',#64291,#15991);
#11117=LINE('',#64294,#15992);
#11118=LINE('',#64295,#15993);
#11119=LINE('',#64297,#15994);
#11120=LINE('',#64299,#15995);
#11121=LINE('',#64301,#15996);
#11122=LINE('',#64303,#15997);
#11123=LINE('',#64306,#15998);
#11124=LINE('',#64307,#15999);
#11125=LINE('',#64309,#16000);
#11126=LINE('',#64311,#16001);
#11127=LINE('',#64313,#16002);
#11128=LINE('',#64315,#16003);
#11129=LINE('',#64318,#16004);
#11130=LINE('',#64319,#16005);
#11131=LINE('',#64321,#16006);
#11132=LINE('',#64323,#16007);
#11133=LINE('',#64325,#16008);
#11134=LINE('',#64327,#16009);
#11135=LINE('',#64330,#16010);
#11136=LINE('',#64331,#16011);
#11137=LINE('',#64333,#16012);
#11138=LINE('',#64335,#16013);
#11139=LINE('',#64337,#16014);
#11140=LINE('',#64339,#16015);
#11141=LINE('',#64342,#16016);
#11142=LINE('',#64343,#16017);
#11143=LINE('',#64345,#16018);
#11144=LINE('',#64347,#16019);
#11145=LINE('',#64349,#16020);
#11146=LINE('',#64351,#16021);
#11147=LINE('',#64354,#16022);
#11148=LINE('',#64355,#16023);
#11149=LINE('',#64357,#16024);
#11150=LINE('',#64359,#16025);
#11151=LINE('',#64361,#16026);
#11152=LINE('',#64363,#16027);
#11153=LINE('',#64366,#16028);
#11154=LINE('',#64367,#16029);
#11155=LINE('',#64369,#16030);
#11156=LINE('',#64371,#16031);
#11157=LINE('',#64373,#16032);
#11158=LINE('',#64375,#16033);
#11159=LINE('',#64378,#16034);
#11160=LINE('',#64379,#16035);
#11161=LINE('',#64381,#16036);
#11162=LINE('',#64383,#16037);
#11163=LINE('',#64385,#16038);
#11164=LINE('',#64387,#16039);
#11165=LINE('',#64390,#16040);
#11166=LINE('',#64391,#16041);
#11167=LINE('',#64393,#16042);
#11168=LINE('',#64395,#16043);
#11169=LINE('',#64397,#16044);
#11170=LINE('',#64399,#16045);
#11171=LINE('',#64402,#16046);
#11172=LINE('',#64403,#16047);
#11173=LINE('',#64405,#16048);
#11174=LINE('',#64407,#16049);
#11175=LINE('',#64409,#16050);
#11176=LINE('',#64411,#16051);
#11177=LINE('',#64414,#16052);
#11178=LINE('',#64415,#16053);
#11179=LINE('',#64417,#16054);
#11180=LINE('',#64419,#16055);
#11181=LINE('',#64421,#16056);
#11182=LINE('',#64423,#16057);
#11183=LINE('',#64426,#16058);
#11184=LINE('',#64427,#16059);
#11185=LINE('',#64429,#16060);
#11186=LINE('',#64431,#16061);
#11187=LINE('',#64433,#16062);
#11188=LINE('',#64435,#16063);
#11189=LINE('',#64438,#16064);
#11190=LINE('',#64439,#16065);
#11191=LINE('',#64441,#16066);
#11192=LINE('',#64443,#16067);
#11193=LINE('',#64445,#16068);
#11194=LINE('',#64447,#16069);
#11195=LINE('',#64450,#16070);
#11196=LINE('',#64451,#16071);
#11197=LINE('',#64453,#16072);
#11198=LINE('',#64455,#16073);
#11199=LINE('',#64457,#16074);
#11200=LINE('',#64459,#16075);
#11201=LINE('',#64462,#16076);
#11202=LINE('',#64463,#16077);
#11203=LINE('',#64465,#16078);
#11204=LINE('',#64467,#16079);
#11205=LINE('',#64469,#16080);
#11206=LINE('',#64471,#16081);
#11207=LINE('',#64474,#16082);
#11208=LINE('',#64475,#16083);
#11209=LINE('',#64477,#16084);
#11210=LINE('',#64479,#16085);
#11211=LINE('',#64481,#16086);
#11212=LINE('',#64483,#16087);
#11213=LINE('',#64486,#16088);
#11214=LINE('',#64487,#16089);
#11215=LINE('',#64489,#16090);
#11216=LINE('',#64491,#16091);
#11217=LINE('',#64493,#16092);
#11218=LINE('',#64495,#16093);
#11219=LINE('',#64498,#16094);
#11220=LINE('',#64499,#16095);
#11221=LINE('',#64501,#16096);
#11222=LINE('',#64503,#16097);
#11223=LINE('',#64505,#16098);
#11224=LINE('',#64507,#16099);
#11225=LINE('',#64510,#16100);
#11226=LINE('',#64511,#16101);
#11227=LINE('',#64513,#16102);
#11228=LINE('',#64515,#16103);
#11229=LINE('',#64517,#16104);
#11230=LINE('',#64519,#16105);
#11231=LINE('',#64522,#16106);
#11232=LINE('',#64523,#16107);
#11233=LINE('',#64525,#16108);
#11234=LINE('',#64527,#16109);
#11235=LINE('',#64529,#16110);
#11236=LINE('',#64531,#16111);
#11237=LINE('',#64534,#16112);
#11238=LINE('',#64535,#16113);
#11239=LINE('',#64537,#16114);
#11240=LINE('',#64539,#16115);
#11241=LINE('',#64541,#16116);
#11242=LINE('',#64543,#16117);
#11243=LINE('',#64546,#16118);
#11244=LINE('',#64547,#16119);
#11245=LINE('',#64549,#16120);
#11246=LINE('',#64551,#16121);
#11247=LINE('',#64553,#16122);
#11248=LINE('',#64555,#16123);
#11249=LINE('',#64558,#16124);
#11250=LINE('',#64559,#16125);
#11251=LINE('',#64561,#16126);
#11252=LINE('',#64563,#16127);
#11253=LINE('',#64565,#16128);
#11254=LINE('',#64567,#16129);
#11255=LINE('',#64570,#16130);
#11256=LINE('',#64571,#16131);
#11257=LINE('',#64573,#16132);
#11258=LINE('',#64575,#16133);
#11259=LINE('',#64577,#16134);
#11260=LINE('',#64579,#16135);
#11261=LINE('',#64582,#16136);
#11262=LINE('',#64583,#16137);
#11263=LINE('',#64585,#16138);
#11264=LINE('',#64587,#16139);
#11265=LINE('',#64589,#16140);
#11266=LINE('',#64591,#16141);
#11267=LINE('',#64594,#16142);
#11268=LINE('',#64595,#16143);
#11269=LINE('',#64597,#16144);
#11270=LINE('',#64599,#16145);
#11271=LINE('',#64601,#16146);
#11272=LINE('',#64603,#16147);
#11273=LINE('',#64606,#16148);
#11274=LINE('',#64607,#16149);
#11275=LINE('',#64609,#16150);
#11276=LINE('',#64611,#16151);
#11277=LINE('',#64613,#16152);
#11278=LINE('',#64615,#16153);
#11279=LINE('',#64618,#16154);
#11280=LINE('',#64619,#16155);
#11281=LINE('',#64621,#16156);
#11282=LINE('',#64623,#16157);
#11283=LINE('',#64625,#16158);
#11284=LINE('',#64627,#16159);
#11285=LINE('',#64630,#16160);
#11286=LINE('',#64631,#16161);
#11287=LINE('',#64633,#16162);
#11288=LINE('',#64635,#16163);
#11289=LINE('',#64637,#16164);
#11290=LINE('',#64639,#16165);
#11291=LINE('',#64642,#16166);
#11292=LINE('',#64643,#16167);
#11293=LINE('',#64645,#16168);
#11294=LINE('',#64647,#16169);
#11295=LINE('',#64649,#16170);
#11296=LINE('',#64651,#16171);
#11297=LINE('',#64654,#16172);
#11298=LINE('',#64655,#16173);
#11299=LINE('',#64657,#16174);
#11300=LINE('',#64659,#16175);
#11301=LINE('',#64661,#16176);
#11302=LINE('',#64663,#16177);
#11303=LINE('',#64666,#16178);
#11304=LINE('',#64667,#16179);
#11305=LINE('',#64669,#16180);
#11306=LINE('',#64671,#16181);
#11307=LINE('',#64673,#16182);
#11308=LINE('',#64675,#16183);
#11309=LINE('',#64678,#16184);
#11310=LINE('',#64679,#16185);
#11311=LINE('',#64681,#16186);
#11312=LINE('',#64683,#16187);
#11313=LINE('',#64685,#16188);
#11314=LINE('',#64687,#16189);
#11315=LINE('',#64690,#16190);
#11316=LINE('',#64691,#16191);
#11317=LINE('',#64693,#16192);
#11318=LINE('',#64695,#16193);
#11319=LINE('',#64697,#16194);
#11320=LINE('',#64699,#16195);
#11321=LINE('',#64702,#16196);
#11322=LINE('',#64703,#16197);
#11323=LINE('',#64705,#16198);
#11324=LINE('',#64707,#16199);
#11325=LINE('',#64709,#16200);
#11326=LINE('',#64711,#16201);
#11327=LINE('',#64714,#16202);
#11328=LINE('',#64715,#16203);
#11329=LINE('',#64717,#16204);
#11330=LINE('',#64719,#16205);
#11331=LINE('',#64721,#16206);
#11332=LINE('',#64723,#16207);
#11333=LINE('',#64726,#16208);
#11334=LINE('',#64727,#16209);
#11335=LINE('',#64729,#16210);
#11336=LINE('',#64731,#16211);
#11337=LINE('',#64733,#16212);
#11338=LINE('',#64735,#16213);
#11339=LINE('',#64738,#16214);
#11340=LINE('',#64739,#16215);
#11341=LINE('',#64741,#16216);
#11342=LINE('',#64743,#16217);
#11343=LINE('',#64745,#16218);
#11344=LINE('',#64747,#16219);
#11345=LINE('',#64750,#16220);
#11346=LINE('',#64751,#16221);
#11347=LINE('',#64753,#16222);
#11348=LINE('',#64755,#16223);
#11349=LINE('',#64757,#16224);
#11350=LINE('',#64759,#16225);
#11351=LINE('',#64762,#16226);
#11352=LINE('',#64763,#16227);
#11353=LINE('',#64765,#16228);
#11354=LINE('',#64767,#16229);
#11355=LINE('',#64769,#16230);
#11356=LINE('',#64771,#16231);
#11357=LINE('',#64774,#16232);
#11358=LINE('',#64775,#16233);
#11359=LINE('',#64777,#16234);
#11360=LINE('',#64779,#16235);
#11361=LINE('',#64781,#16236);
#11362=LINE('',#64783,#16237);
#11363=LINE('',#64786,#16238);
#11364=LINE('',#64787,#16239);
#11365=LINE('',#64789,#16240);
#11366=LINE('',#64791,#16241);
#11367=LINE('',#64793,#16242);
#11368=LINE('',#64795,#16243);
#11369=LINE('',#64798,#16244);
#11370=LINE('',#64799,#16245);
#11371=LINE('',#64801,#16246);
#11372=LINE('',#64803,#16247);
#11373=LINE('',#64805,#16248);
#11374=LINE('',#64807,#16249);
#11375=LINE('',#64810,#16250);
#11376=LINE('',#64811,#16251);
#11377=LINE('',#64813,#16252);
#11378=LINE('',#64815,#16253);
#11379=LINE('',#64817,#16254);
#11380=LINE('',#64819,#16255);
#11381=LINE('',#64822,#16256);
#11382=LINE('',#64823,#16257);
#11383=LINE('',#64825,#16258);
#11384=LINE('',#64827,#16259);
#11385=LINE('',#64829,#16260);
#11386=LINE('',#64831,#16261);
#11387=LINE('',#64834,#16262);
#11388=LINE('',#64835,#16263);
#11389=LINE('',#64837,#16264);
#11390=LINE('',#64839,#16265);
#11391=LINE('',#64841,#16266);
#11392=LINE('',#64843,#16267);
#11393=LINE('',#64846,#16268);
#11394=LINE('',#64847,#16269);
#11395=LINE('',#64849,#16270);
#11396=LINE('',#64851,#16271);
#11397=LINE('',#64853,#16272);
#11398=LINE('',#64855,#16273);
#11399=LINE('',#64858,#16274);
#11400=LINE('',#64859,#16275);
#11401=LINE('',#64861,#16276);
#11402=LINE('',#64863,#16277);
#11403=LINE('',#64865,#16278);
#11404=LINE('',#64867,#16279);
#11405=LINE('',#64870,#16280);
#11406=LINE('',#64871,#16281);
#11407=LINE('',#64873,#16282);
#11408=LINE('',#64875,#16283);
#11409=LINE('',#64877,#16284);
#11410=LINE('',#64879,#16285);
#11411=LINE('',#64882,#16286);
#11412=LINE('',#64883,#16287);
#11413=LINE('',#64885,#16288);
#11414=LINE('',#64887,#16289);
#11415=LINE('',#64889,#16290);
#11416=LINE('',#64891,#16291);
#11417=LINE('',#64894,#16292);
#11418=LINE('',#64895,#16293);
#11419=LINE('',#64897,#16294);
#11420=LINE('',#64899,#16295);
#11421=LINE('',#64901,#16296);
#11422=LINE('',#64903,#16297);
#11423=LINE('',#64906,#16298);
#11424=LINE('',#64907,#16299);
#11425=LINE('',#64909,#16300);
#11426=LINE('',#64911,#16301);
#11427=LINE('',#64913,#16302);
#11428=LINE('',#64915,#16303);
#11429=LINE('',#64918,#16304);
#11430=LINE('',#64919,#16305);
#11431=LINE('',#64921,#16306);
#11432=LINE('',#64923,#16307);
#11433=LINE('',#64925,#16308);
#11434=LINE('',#64927,#16309);
#11435=LINE('',#64930,#16310);
#11436=LINE('',#64931,#16311);
#11437=LINE('',#64933,#16312);
#11438=LINE('',#64935,#16313);
#11439=LINE('',#64937,#16314);
#11440=LINE('',#64939,#16315);
#11441=LINE('',#64942,#16316);
#11442=LINE('',#64943,#16317);
#11443=LINE('',#64945,#16318);
#11444=LINE('',#64947,#16319);
#11445=LINE('',#64949,#16320);
#11446=LINE('',#64951,#16321);
#11447=LINE('',#64954,#16322);
#11448=LINE('',#64955,#16323);
#11449=LINE('',#64957,#16324);
#11450=LINE('',#64959,#16325);
#11451=LINE('',#64961,#16326);
#11452=LINE('',#64963,#16327);
#11453=LINE('',#64966,#16328);
#11454=LINE('',#64967,#16329);
#11455=LINE('',#64969,#16330);
#11456=LINE('',#64971,#16331);
#11457=LINE('',#64973,#16332);
#11458=LINE('',#64975,#16333);
#11459=LINE('',#64978,#16334);
#11460=LINE('',#64979,#16335);
#11461=LINE('',#64981,#16336);
#11462=LINE('',#64983,#16337);
#11463=LINE('',#64985,#16338);
#11464=LINE('',#64987,#16339);
#11465=LINE('',#64990,#16340);
#11466=LINE('',#64991,#16341);
#11467=LINE('',#64993,#16342);
#11468=LINE('',#64995,#16343);
#11469=LINE('',#64997,#16344);
#11470=LINE('',#64999,#16345);
#11471=LINE('',#65002,#16346);
#11472=LINE('',#65003,#16347);
#11473=LINE('',#65005,#16348);
#11474=LINE('',#65007,#16349);
#11475=LINE('',#65009,#16350);
#11476=LINE('',#65011,#16351);
#11477=LINE('',#65014,#16352);
#11478=LINE('',#65015,#16353);
#11479=LINE('',#65017,#16354);
#11480=LINE('',#65019,#16355);
#11481=LINE('',#65021,#16356);
#11482=LINE('',#65023,#16357);
#11483=LINE('',#65026,#16358);
#11484=LINE('',#65027,#16359);
#11485=LINE('',#65029,#16360);
#11486=LINE('',#65031,#16361);
#11487=LINE('',#65033,#16362);
#11488=LINE('',#65035,#16363);
#11489=LINE('',#65038,#16364);
#11490=LINE('',#65039,#16365);
#11491=LINE('',#65041,#16366);
#11492=LINE('',#65043,#16367);
#11493=LINE('',#65045,#16368);
#11494=LINE('',#65047,#16369);
#11495=LINE('',#65050,#16370);
#11496=LINE('',#65051,#16371);
#11497=LINE('',#65053,#16372);
#11498=LINE('',#65055,#16373);
#11499=LINE('',#65057,#16374);
#11500=LINE('',#65059,#16375);
#11501=LINE('',#65062,#16376);
#11502=LINE('',#65063,#16377);
#11503=LINE('',#65065,#16378);
#11504=LINE('',#65067,#16379);
#11505=LINE('',#65069,#16380);
#11506=LINE('',#65071,#16381);
#11507=LINE('',#65074,#16382);
#11508=LINE('',#65075,#16383);
#11509=LINE('',#65077,#16384);
#11510=LINE('',#65079,#16385);
#11511=LINE('',#65081,#16386);
#11512=LINE('',#65083,#16387);
#11513=LINE('',#65086,#16388);
#11514=LINE('',#65087,#16389);
#11515=LINE('',#65089,#16390);
#11516=LINE('',#65091,#16391);
#11517=LINE('',#65093,#16392);
#11518=LINE('',#65095,#16393);
#11519=LINE('',#65098,#16394);
#11520=LINE('',#65099,#16395);
#11521=LINE('',#65101,#16396);
#11522=LINE('',#65103,#16397);
#11523=LINE('',#65105,#16398);
#11524=LINE('',#65107,#16399);
#11525=LINE('',#65110,#16400);
#11526=LINE('',#65111,#16401);
#11527=LINE('',#65113,#16402);
#11528=LINE('',#65115,#16403);
#11529=LINE('',#65117,#16404);
#11530=LINE('',#65119,#16405);
#11531=LINE('',#65122,#16406);
#11532=LINE('',#65123,#16407);
#11533=LINE('',#65125,#16408);
#11534=LINE('',#65127,#16409);
#11535=LINE('',#65129,#16410);
#11536=LINE('',#65131,#16411);
#11537=LINE('',#65134,#16412);
#11538=LINE('',#65135,#16413);
#11539=LINE('',#65137,#16414);
#11540=LINE('',#65139,#16415);
#11541=LINE('',#65141,#16416);
#11542=LINE('',#65143,#16417);
#11543=LINE('',#65146,#16418);
#11544=LINE('',#65147,#16419);
#11545=LINE('',#65149,#16420);
#11546=LINE('',#65151,#16421);
#11547=LINE('',#65153,#16422);
#11548=LINE('',#65155,#16423);
#11549=LINE('',#65158,#16424);
#11550=LINE('',#65159,#16425);
#11551=LINE('',#65161,#16426);
#11552=LINE('',#65163,#16427);
#11553=LINE('',#65165,#16428);
#11554=LINE('',#65167,#16429);
#11555=LINE('',#65170,#16430);
#11556=LINE('',#65171,#16431);
#11557=LINE('',#65173,#16432);
#11558=LINE('',#65175,#16433);
#11559=LINE('',#65177,#16434);
#11560=LINE('',#65179,#16435);
#11561=LINE('',#65182,#16436);
#11562=LINE('',#65183,#16437);
#11563=LINE('',#65185,#16438);
#11564=LINE('',#65187,#16439);
#11565=LINE('',#65189,#16440);
#11566=LINE('',#65191,#16441);
#11567=LINE('',#65194,#16442);
#11568=LINE('',#65195,#16443);
#11569=LINE('',#65197,#16444);
#11570=LINE('',#65199,#16445);
#11571=LINE('',#65201,#16446);
#11572=LINE('',#65203,#16447);
#11573=LINE('',#65206,#16448);
#11574=LINE('',#65207,#16449);
#11575=LINE('',#65209,#16450);
#11576=LINE('',#65211,#16451);
#11577=LINE('',#65213,#16452);
#11578=LINE('',#65215,#16453);
#11579=LINE('',#65218,#16454);
#11580=LINE('',#65219,#16455);
#11581=LINE('',#65221,#16456);
#11582=LINE('',#65223,#16457);
#11583=LINE('',#65225,#16458);
#11584=LINE('',#65227,#16459);
#11585=LINE('',#65230,#16460);
#11586=LINE('',#65231,#16461);
#11587=LINE('',#65233,#16462);
#11588=LINE('',#65235,#16463);
#11589=LINE('',#65237,#16464);
#11590=LINE('',#65239,#16465);
#11591=LINE('',#65242,#16466);
#11592=LINE('',#65243,#16467);
#11593=LINE('',#65245,#16468);
#11594=LINE('',#65247,#16469);
#11595=LINE('',#65249,#16470);
#11596=LINE('',#65251,#16471);
#11597=LINE('',#65254,#16472);
#11598=LINE('',#65255,#16473);
#11599=LINE('',#65257,#16474);
#11600=LINE('',#65259,#16475);
#11601=LINE('',#65261,#16476);
#11602=LINE('',#65263,#16477);
#11603=LINE('',#65266,#16478);
#11604=LINE('',#65267,#16479);
#11605=LINE('',#65269,#16480);
#11606=LINE('',#65271,#16481);
#11607=LINE('',#65273,#16482);
#11608=LINE('',#65275,#16483);
#11609=LINE('',#65278,#16484);
#11610=LINE('',#65279,#16485);
#11611=LINE('',#65281,#16486);
#11612=LINE('',#65283,#16487);
#11613=LINE('',#65285,#16488);
#11614=LINE('',#65287,#16489);
#13054=VECTOR('',#46633,1000.);
#13055=VECTOR('',#46634,1000.);
#13056=VECTOR('',#46635,1000.);
#13057=VECTOR('',#46636,1000.);
#13058=VECTOR('',#46637,1000.);
#13059=VECTOR('',#46638,1000.);
#13060=VECTOR('',#46639,1000.);
#13061=VECTOR('',#46640,1000.);
#13062=VECTOR('',#46641,1000.);
#13063=VECTOR('',#46642,1000.);
#13064=VECTOR('',#46643,1000.);
#13065=VECTOR('',#46644,1000.);
#13066=VECTOR('',#46647,1000.);
#13067=VECTOR('',#46648,1000.);
#13068=VECTOR('',#46649,1000.);
#13069=VECTOR('',#46650,1000.);
#13070=VECTOR('',#46651,1000.);
#13071=VECTOR('',#46652,1000.);
#13072=VECTOR('',#46653,1000.);
#13073=VECTOR('',#46654,1000.);
#13074=VECTOR('',#46655,1000.);
#13075=VECTOR('',#46656,1000.);
#13076=VECTOR('',#46657,1000.);
#13077=VECTOR('',#46658,1000.);
#13078=VECTOR('',#46661,1000.);
#13079=VECTOR('',#46662,1000.);
#13080=VECTOR('',#46665,1000.);
#13081=VECTOR('',#46666,1000.);
#13082=VECTOR('',#46669,1000.);
#13083=VECTOR('',#46670,1000.);
#13084=VECTOR('',#46673,1000.);
#13085=VECTOR('',#46674,1000.);
#13086=VECTOR('',#46679,1000.);
#13087=VECTOR('',#46680,1000.);
#13088=VECTOR('',#46683,1000.);
#13089=VECTOR('',#46686,1000.);
#13090=VECTOR('',#46689,1000.);
#13091=VECTOR('',#46698,1000.);
#13092=VECTOR('',#46703,1000.);
#13093=VECTOR('',#46706,1000.);
#13094=VECTOR('',#46711,1000.);
#13095=VECTOR('',#46716,1000.);
#13096=VECTOR('',#46723,1000.);
#13097=VECTOR('',#46726,1000.);
#13098=VECTOR('',#46731,1000.);
#13099=VECTOR('',#46734,1000.);
#13100=VECTOR('',#46737,1000.);
#13101=VECTOR('',#46738,1000.);
#13102=VECTOR('',#46739,1000.);
#13103=VECTOR('',#46740,1000.);
#13104=VECTOR('',#46745,1000.);
#13105=VECTOR('',#46748,1000.);
#13106=VECTOR('',#46751,1000.);
#13107=VECTOR('',#46752,1000.);
#13108=VECTOR('',#46755,1000.);
#13109=VECTOR('',#46756,1000.);
#13110=VECTOR('',#46757,1000.);
#13111=VECTOR('',#46758,1000.);
#13112=VECTOR('',#46761,1000.);
#13113=VECTOR('',#46764,1000.);
#13114=VECTOR('',#46765,1000.);
#13115=VECTOR('',#46766,1000.);
#13116=VECTOR('',#46775,1000.);
#13117=VECTOR('',#46784,1000.);
#13118=VECTOR('',#46789,1000.);
#13119=VECTOR('',#46792,1000.);
#13120=VECTOR('',#46797,1000.);
#13121=VECTOR('',#46802,1000.);
#13122=VECTOR('',#46809,1000.);
#13123=VECTOR('',#46812,1000.);
#13124=VECTOR('',#46817,1000.);
#13125=VECTOR('',#46820,1000.);
#13126=VECTOR('',#46823,1000.);
#13127=VECTOR('',#46824,1000.);
#13128=VECTOR('',#46825,1000.);
#13129=VECTOR('',#46826,1000.);
#13130=VECTOR('',#46831,1000.);
#13131=VECTOR('',#46834,1000.);
#13132=VECTOR('',#46837,1000.);
#13133=VECTOR('',#46838,1000.);
#13134=VECTOR('',#46841,1000.);
#13135=VECTOR('',#46842,1000.);
#13136=VECTOR('',#46843,1000.);
#13137=VECTOR('',#46844,1000.);
#13138=VECTOR('',#46847,1000.);
#13139=VECTOR('',#46850,1000.);
#13140=VECTOR('',#46851,1000.);
#13141=VECTOR('',#46852,1000.);
#13142=VECTOR('',#46861,1000.);
#13143=VECTOR('',#46862,1000.);
#13144=VECTOR('',#46863,1000.);
#13145=VECTOR('',#46864,1000.);
#13146=VECTOR('',#46865,1000.);
#13147=VECTOR('',#46866,1000.);
#13148=VECTOR('',#46867,1000.);
#13149=VECTOR('',#46868,1000.);
#13150=VECTOR('',#46869,1000.);
#13151=VECTOR('',#46870,1000.);
#13152=VECTOR('',#46871,1000.);
#13153=VECTOR('',#46872,1000.);
#13154=VECTOR('',#46873,1000.);
#13155=VECTOR('',#46874,1000.);
#13156=VECTOR('',#46875,1000.);
#13157=VECTOR('',#46876,1000.);
#13158=VECTOR('',#46877,1000.);
#13159=VECTOR('',#46878,1000.);
#13160=VECTOR('',#46879,1000.);
#13161=VECTOR('',#46880,1000.);
#13162=VECTOR('',#46881,1000.);
#13163=VECTOR('',#46882,1000.);
#13164=VECTOR('',#46883,1000.);
#13165=VECTOR('',#46884,1000.);
#13166=VECTOR('',#46885,1000.);
#13167=VECTOR('',#46886,1000.);
#13168=VECTOR('',#46887,1000.);
#13169=VECTOR('',#46888,1000.);
#13170=VECTOR('',#46889,1000.);
#13171=VECTOR('',#46890,1000.);
#13172=VECTOR('',#46891,1000.);
#13173=VECTOR('',#46892,1000.);
#13174=VECTOR('',#46893,1000.);
#13175=VECTOR('',#46894,1000.);
#13176=VECTOR('',#46895,1000.);
#13177=VECTOR('',#46896,1000.);
#13178=VECTOR('',#46897,1000.);
#13179=VECTOR('',#46898,1000.);
#13180=VECTOR('',#46899,1000.);
#13181=VECTOR('',#46900,1000.);
#13182=VECTOR('',#46901,1000.);
#13183=VECTOR('',#46902,1000.);
#13184=VECTOR('',#46903,1000.);
#13185=VECTOR('',#46904,1000.);
#13186=VECTOR('',#46905,1000.);
#13187=VECTOR('',#46906,1000.);
#13188=VECTOR('',#46907,1000.);
#13189=VECTOR('',#46908,1000.);
#13190=VECTOR('',#46909,1000.);
#13191=VECTOR('',#46910,1000.);
#13192=VECTOR('',#46911,1000.);
#13193=VECTOR('',#46912,1000.);
#13194=VECTOR('',#46913,1000.);
#13195=VECTOR('',#46914,1000.);
#13196=VECTOR('',#46915,1000.);
#13197=VECTOR('',#46916,1000.);
#13198=VECTOR('',#46917,1000.);
#13199=VECTOR('',#46918,1000.);
#13200=VECTOR('',#46919,1000.);
#13201=VECTOR('',#46920,1000.);
#13202=VECTOR('',#46921,1000.);
#13203=VECTOR('',#46922,1000.);
#13204=VECTOR('',#46923,1000.);
#13205=VECTOR('',#46924,1000.);
#13206=VECTOR('',#46925,1000.);
#13207=VECTOR('',#46926,1000.);
#13208=VECTOR('',#46927,1000.);
#13209=VECTOR('',#46928,1000.);
#13210=VECTOR('',#46929,1000.);
#13211=VECTOR('',#46930,1000.);
#13212=VECTOR('',#46931,1000.);
#13213=VECTOR('',#46932,1000.);
#13214=VECTOR('',#46933,1000.);
#13215=VECTOR('',#46934,1000.);
#13216=VECTOR('',#46935,1000.);
#13217=VECTOR('',#46936,1000.);
#13218=VECTOR('',#46937,1000.);
#13219=VECTOR('',#46938,1000.);
#13220=VECTOR('',#46939,1000.);
#13221=VECTOR('',#46940,1000.);
#13222=VECTOR('',#46941,1000.);
#13223=VECTOR('',#46942,1000.);
#13224=VECTOR('',#46943,1000.);
#13225=VECTOR('',#46944,1000.);
#13226=VECTOR('',#46945,1000.);
#13227=VECTOR('',#46946,1000.);
#13228=VECTOR('',#46947,1000.);
#13229=VECTOR('',#46948,1000.);
#13230=VECTOR('',#46949,1000.);
#13231=VECTOR('',#46950,1000.);
#13232=VECTOR('',#46951,1000.);
#13233=VECTOR('',#46952,1000.);
#13234=VECTOR('',#46953,1000.);
#13235=VECTOR('',#46954,1000.);
#13236=VECTOR('',#46955,1000.);
#13237=VECTOR('',#46956,1000.);
#13238=VECTOR('',#46957,1000.);
#13239=VECTOR('',#46958,1000.);
#13240=VECTOR('',#46959,1000.);
#13241=VECTOR('',#46960,1000.);
#13242=VECTOR('',#46961,1000.);
#13243=VECTOR('',#46962,1000.);
#13244=VECTOR('',#46963,1000.);
#13245=VECTOR('',#46964,1000.);
#13246=VECTOR('',#46965,1000.);
#13247=VECTOR('',#46966,1000.);
#13248=VECTOR('',#46967,1000.);
#13249=VECTOR('',#46968,1000.);
#13250=VECTOR('',#46969,1000.);
#13251=VECTOR('',#46970,1000.);
#13252=VECTOR('',#46971,1000.);
#13253=VECTOR('',#46972,1000.);
#13254=VECTOR('',#46973,1000.);
#13255=VECTOR('',#46974,1000.);
#13256=VECTOR('',#46975,1000.);
#13257=VECTOR('',#46976,1000.);
#13258=VECTOR('',#46977,1000.);
#13259=VECTOR('',#46978,1000.);
#13260=VECTOR('',#46979,1000.);
#13261=VECTOR('',#46980,1000.);
#13262=VECTOR('',#46981,1000.);
#13263=VECTOR('',#46982,1000.);
#13264=VECTOR('',#46983,1000.);
#13265=VECTOR('',#46984,1000.);
#13266=VECTOR('',#46985,1000.);
#13267=VECTOR('',#46986,1000.);
#13268=VECTOR('',#46987,1000.);
#13269=VECTOR('',#46988,1000.);
#13270=VECTOR('',#46989,1000.);
#13271=VECTOR('',#46990,1000.);
#13272=VECTOR('',#46991,1000.);
#13273=VECTOR('',#46992,1000.);
#13274=VECTOR('',#46993,1000.);
#13275=VECTOR('',#46994,1000.);
#13276=VECTOR('',#46995,1000.);
#13277=VECTOR('',#46996,1000.);
#13278=VECTOR('',#46997,1000.);
#13279=VECTOR('',#46998,1000.);
#13280=VECTOR('',#46999,1000.);
#13281=VECTOR('',#47000,1000.);
#13282=VECTOR('',#47001,1000.);
#13283=VECTOR('',#47002,1000.);
#13284=VECTOR('',#47003,1000.);
#13285=VECTOR('',#47004,1000.);
#13286=VECTOR('',#47005,1000.);
#13287=VECTOR('',#47006,1000.);
#13288=VECTOR('',#47007,1000.);
#13289=VECTOR('',#47008,1000.);
#13290=VECTOR('',#47009,1000.);
#13291=VECTOR('',#47010,1000.);
#13292=VECTOR('',#47011,1000.);
#13293=VECTOR('',#47012,1000.);
#13294=VECTOR('',#47013,1000.);
#13295=VECTOR('',#47014,1000.);
#13296=VECTOR('',#47015,1000.);
#13297=VECTOR('',#47016,1000.);
#13298=VECTOR('',#47017,1000.);
#13299=VECTOR('',#47018,1000.);
#13300=VECTOR('',#47019,1000.);
#13301=VECTOR('',#47020,1000.);
#13302=VECTOR('',#47021,1000.);
#13303=VECTOR('',#47022,1000.);
#13304=VECTOR('',#47023,1000.);
#13305=VECTOR('',#47024,1000.);
#13306=VECTOR('',#47025,1000.);
#13307=VECTOR('',#47026,1000.);
#13308=VECTOR('',#47027,1000.);
#13309=VECTOR('',#47028,1000.);
#13310=VECTOR('',#47029,1000.);
#13311=VECTOR('',#47030,1000.);
#13312=VECTOR('',#47031,1000.);
#13313=VECTOR('',#47032,1000.);
#13314=VECTOR('',#47033,1000.);
#13315=VECTOR('',#47034,1000.);
#13316=VECTOR('',#47035,1000.);
#13317=VECTOR('',#47036,1000.);
#13318=VECTOR('',#47037,1000.);
#13319=VECTOR('',#47038,1000.);
#13320=VECTOR('',#47039,1000.);
#13321=VECTOR('',#47040,1000.);
#13322=VECTOR('',#47041,1000.);
#13323=VECTOR('',#47042,1000.);
#13324=VECTOR('',#47043,1000.);
#13325=VECTOR('',#47044,1000.);
#13326=VECTOR('',#47045,1000.);
#13327=VECTOR('',#47046,1000.);
#13328=VECTOR('',#47047,1000.);
#13329=VECTOR('',#47048,1000.);
#13330=VECTOR('',#47049,1000.);
#13331=VECTOR('',#47050,1000.);
#13332=VECTOR('',#47051,1000.);
#13333=VECTOR('',#47052,1000.);
#13334=VECTOR('',#47053,1000.);
#13335=VECTOR('',#47054,1000.);
#13336=VECTOR('',#47055,1000.);
#13337=VECTOR('',#47056,1000.);
#13338=VECTOR('',#47057,1000.);
#13339=VECTOR('',#47058,1000.);
#13340=VECTOR('',#47059,1000.);
#13341=VECTOR('',#47060,1000.);
#13342=VECTOR('',#47061,1000.);
#13343=VECTOR('',#47062,1000.);
#13344=VECTOR('',#47063,1000.);
#13345=VECTOR('',#47064,1000.);
#13346=VECTOR('',#47065,1000.);
#13347=VECTOR('',#47066,1000.);
#13348=VECTOR('',#47067,1000.);
#13349=VECTOR('',#47068,1000.);
#13350=VECTOR('',#47069,1000.);
#13351=VECTOR('',#47070,1000.);
#13352=VECTOR('',#47071,1000.);
#13353=VECTOR('',#47072,1000.);
#13354=VECTOR('',#47073,1000.);
#13355=VECTOR('',#47074,1000.);
#13356=VECTOR('',#47075,1000.);
#13357=VECTOR('',#47076,1000.);
#13358=VECTOR('',#47077,1000.);
#13359=VECTOR('',#47078,1000.);
#13360=VECTOR('',#47079,1000.);
#13361=VECTOR('',#47080,1000.);
#13362=VECTOR('',#47081,1000.);
#13363=VECTOR('',#47082,1000.);
#13364=VECTOR('',#47083,1000.);
#13365=VECTOR('',#47084,1000.);
#13366=VECTOR('',#47085,1000.);
#13367=VECTOR('',#47086,1000.);
#13368=VECTOR('',#47087,1000.);
#13369=VECTOR('',#47088,1000.);
#13370=VECTOR('',#47089,1000.);
#13371=VECTOR('',#47090,1000.);
#13372=VECTOR('',#47091,1000.);
#13373=VECTOR('',#47092,1000.);
#13374=VECTOR('',#47093,1000.);
#13375=VECTOR('',#47094,1000.);
#13376=VECTOR('',#47095,1000.);
#13377=VECTOR('',#47096,1000.);
#13378=VECTOR('',#47097,1000.);
#13379=VECTOR('',#47098,1000.);
#13380=VECTOR('',#47099,1000.);
#13381=VECTOR('',#47100,1000.);
#13382=VECTOR('',#47101,1000.);
#13383=VECTOR('',#47102,1000.);
#13384=VECTOR('',#47103,1000.);
#13385=VECTOR('',#47104,1000.);
#13386=VECTOR('',#47105,1000.);
#13387=VECTOR('',#47106,1000.);
#13388=VECTOR('',#47107,1000.);
#13389=VECTOR('',#47108,1000.);
#13390=VECTOR('',#47109,1000.);
#13391=VECTOR('',#47110,1000.);
#13392=VECTOR('',#47111,1000.);
#13393=VECTOR('',#47112,1000.);
#13394=VECTOR('',#47113,1000.);
#13395=VECTOR('',#47114,1000.);
#13396=VECTOR('',#47115,1000.);
#13397=VECTOR('',#47116,1000.);
#13398=VECTOR('',#47117,1000.);
#13399=VECTOR('',#47118,1000.);
#13400=VECTOR('',#47119,1000.);
#13401=VECTOR('',#47120,1000.);
#13402=VECTOR('',#47121,1000.);
#13403=VECTOR('',#47122,1000.);
#13404=VECTOR('',#47123,1000.);
#13405=VECTOR('',#47124,1000.);
#13406=VECTOR('',#47125,1000.);
#13407=VECTOR('',#47126,1000.);
#13408=VECTOR('',#47127,1000.);
#13409=VECTOR('',#47128,1000.);
#13410=VECTOR('',#47129,1000.);
#13411=VECTOR('',#47130,1000.);
#13412=VECTOR('',#47131,1000.);
#13413=VECTOR('',#47132,1000.);
#13414=VECTOR('',#47133,1000.);
#13415=VECTOR('',#47134,1000.);
#13416=VECTOR('',#47135,1000.);
#13417=VECTOR('',#47136,1000.);
#13418=VECTOR('',#47137,1000.);
#13419=VECTOR('',#47138,1000.);
#13420=VECTOR('',#47139,1000.);
#13421=VECTOR('',#47140,1000.);
#13422=VECTOR('',#47141,1000.);
#13423=VECTOR('',#47142,1000.);
#13424=VECTOR('',#47143,1000.);
#13425=VECTOR('',#47144,1000.);
#13426=VECTOR('',#47145,1000.);
#13427=VECTOR('',#47146,1000.);
#13428=VECTOR('',#47147,1000.);
#13429=VECTOR('',#47148,1000.);
#13430=VECTOR('',#47149,1000.);
#13431=VECTOR('',#47150,1000.);
#13432=VECTOR('',#47151,1000.);
#13433=VECTOR('',#47152,1000.);
#13434=VECTOR('',#47153,1000.);
#13435=VECTOR('',#47154,1000.);
#13436=VECTOR('',#47155,1000.);
#13437=VECTOR('',#47156,1000.);
#13438=VECTOR('',#47157,1000.);
#13439=VECTOR('',#47158,1000.);
#13440=VECTOR('',#47159,1000.);
#13441=VECTOR('',#47160,1000.);
#13442=VECTOR('',#47161,1000.);
#13443=VECTOR('',#47162,1000.);
#13444=VECTOR('',#47163,1000.);
#13445=VECTOR('',#47164,1000.);
#13446=VECTOR('',#47165,1000.);
#13447=VECTOR('',#47166,1000.);
#13448=VECTOR('',#47167,1000.);
#13449=VECTOR('',#47168,1000.);
#13450=VECTOR('',#47169,1000.);
#13451=VECTOR('',#47170,1000.);
#13452=VECTOR('',#47171,1000.);
#13453=VECTOR('',#47172,1000.);
#13454=VECTOR('',#47173,1000.);
#13455=VECTOR('',#47174,1000.);
#13456=VECTOR('',#47175,1000.);
#13457=VECTOR('',#47176,1000.);
#13458=VECTOR('',#47177,1000.);
#13459=VECTOR('',#47178,1000.);
#13460=VECTOR('',#47179,1000.);
#13461=VECTOR('',#47180,1000.);
#13462=VECTOR('',#47181,1000.);
#13463=VECTOR('',#47182,1000.);
#13464=VECTOR('',#47183,1000.);
#13465=VECTOR('',#47184,1000.);
#13466=VECTOR('',#47185,1000.);
#13467=VECTOR('',#47186,1000.);
#13468=VECTOR('',#47187,1000.);
#13469=VECTOR('',#47188,1000.);
#13470=VECTOR('',#47189,1000.);
#13471=VECTOR('',#47190,1000.);
#13472=VECTOR('',#47191,1000.);
#13473=VECTOR('',#47192,1000.);
#13474=VECTOR('',#47193,1000.);
#13475=VECTOR('',#47194,1000.);
#13476=VECTOR('',#47195,1000.);
#13477=VECTOR('',#47196,1000.);
#13478=VECTOR('',#47197,1000.);
#13479=VECTOR('',#47198,1000.);
#13480=VECTOR('',#47199,1000.);
#13481=VECTOR('',#47200,1000.);
#13482=VECTOR('',#47201,1000.);
#13483=VECTOR('',#47202,1000.);
#13484=VECTOR('',#47203,1000.);
#13485=VECTOR('',#47204,1000.);
#13486=VECTOR('',#47205,1000.);
#13487=VECTOR('',#47206,1000.);
#13488=VECTOR('',#47207,1000.);
#13489=VECTOR('',#47208,1000.);
#13490=VECTOR('',#47209,1000.);
#13491=VECTOR('',#47210,1000.);
#13492=VECTOR('',#47211,1000.);
#13493=VECTOR('',#47212,1000.);
#13494=VECTOR('',#47213,1000.);
#13495=VECTOR('',#47214,1000.);
#13496=VECTOR('',#47215,1000.);
#13497=VECTOR('',#47216,1000.);
#13498=VECTOR('',#47217,1000.);
#13499=VECTOR('',#47218,1000.);
#13500=VECTOR('',#47219,1000.);
#13501=VECTOR('',#47220,1000.);
#13502=VECTOR('',#47221,1000.);
#13503=VECTOR('',#47222,1000.);
#13504=VECTOR('',#47223,1000.);
#13505=VECTOR('',#47224,1000.);
#13506=VECTOR('',#47225,1000.);
#13507=VECTOR('',#47226,1000.);
#13508=VECTOR('',#47227,1000.);
#13509=VECTOR('',#47228,1000.);
#13510=VECTOR('',#47229,1000.);
#13511=VECTOR('',#47230,1000.);
#13512=VECTOR('',#47231,1000.);
#13513=VECTOR('',#47232,1000.);
#13514=VECTOR('',#47233,1000.);
#13515=VECTOR('',#47234,1000.);
#13516=VECTOR('',#47235,1000.);
#13517=VECTOR('',#47236,1000.);
#13518=VECTOR('',#47237,1000.);
#13519=VECTOR('',#47238,1000.);
#13520=VECTOR('',#47239,1000.);
#13521=VECTOR('',#47240,1000.);
#13522=VECTOR('',#47241,1000.);
#13523=VECTOR('',#47242,1000.);
#13524=VECTOR('',#47243,1000.);
#13525=VECTOR('',#47244,1000.);
#13526=VECTOR('',#47245,1000.);
#13527=VECTOR('',#47246,1000.);
#13528=VECTOR('',#47247,1000.);
#13529=VECTOR('',#47248,1000.);
#13530=VECTOR('',#47249,1000.);
#13531=VECTOR('',#47250,1000.);
#13532=VECTOR('',#47251,1000.);
#13533=VECTOR('',#47252,1000.);
#13534=VECTOR('',#47253,1000.);
#13535=VECTOR('',#47254,1000.);
#13536=VECTOR('',#47255,1000.);
#13537=VECTOR('',#47256,1000.);
#13538=VECTOR('',#47257,1000.);
#13539=VECTOR('',#47258,1000.);
#13540=VECTOR('',#47259,1000.);
#13541=VECTOR('',#47260,1000.);
#13542=VECTOR('',#47261,1000.);
#13543=VECTOR('',#47262,1000.);
#13544=VECTOR('',#47263,1000.);
#13545=VECTOR('',#47264,1000.);
#13546=VECTOR('',#47265,1000.);
#13547=VECTOR('',#47266,1000.);
#13548=VECTOR('',#47267,1000.);
#13549=VECTOR('',#47268,1000.);
#13550=VECTOR('',#47269,1000.);
#13551=VECTOR('',#47270,1000.);
#13552=VECTOR('',#47271,1000.);
#13553=VECTOR('',#47272,1000.);
#13554=VECTOR('',#47273,1000.);
#13555=VECTOR('',#47274,1000.);
#13556=VECTOR('',#47275,1000.);
#13557=VECTOR('',#47276,1000.);
#13558=VECTOR('',#47277,1000.);
#13559=VECTOR('',#47278,1000.);
#13560=VECTOR('',#47279,1000.);
#13561=VECTOR('',#47280,1000.);
#13562=VECTOR('',#47281,1000.);
#13563=VECTOR('',#47282,1000.);
#13564=VECTOR('',#47283,1000.);
#13565=VECTOR('',#47284,1000.);
#13566=VECTOR('',#47285,1000.);
#13567=VECTOR('',#47286,1000.);
#13568=VECTOR('',#47287,1000.);
#13569=VECTOR('',#47288,1000.);
#13570=VECTOR('',#47289,1000.);
#13571=VECTOR('',#47290,1000.);
#13572=VECTOR('',#47291,1000.);
#13573=VECTOR('',#47292,1000.);
#13574=VECTOR('',#47293,1000.);
#13575=VECTOR('',#47294,1000.);
#13576=VECTOR('',#47295,1000.);
#13577=VECTOR('',#47296,1000.);
#13578=VECTOR('',#47297,1000.);
#13579=VECTOR('',#47298,1000.);
#13580=VECTOR('',#47299,1000.);
#13581=VECTOR('',#47300,1000.);
#13582=VECTOR('',#47301,1000.);
#13583=VECTOR('',#47302,1000.);
#13584=VECTOR('',#47303,1000.);
#13585=VECTOR('',#47304,1000.);
#13586=VECTOR('',#47305,1000.);
#13587=VECTOR('',#47306,1000.);
#13588=VECTOR('',#47307,1000.);
#13589=VECTOR('',#47308,1000.);
#13590=VECTOR('',#47309,1000.);
#13591=VECTOR('',#47310,1000.);
#13592=VECTOR('',#47311,1000.);
#13593=VECTOR('',#47312,1000.);
#13594=VECTOR('',#47313,1000.);
#13595=VECTOR('',#47314,1000.);
#13596=VECTOR('',#47315,1000.);
#13597=VECTOR('',#47316,1000.);
#13598=VECTOR('',#47317,1000.);
#13599=VECTOR('',#47318,1000.);
#13600=VECTOR('',#47319,1000.);
#13601=VECTOR('',#47320,1000.);
#13602=VECTOR('',#47321,1000.);
#13603=VECTOR('',#47322,1000.);
#13604=VECTOR('',#47323,1000.);
#13605=VECTOR('',#47324,1000.);
#13606=VECTOR('',#47325,1000.);
#13607=VECTOR('',#47326,1000.);
#13608=VECTOR('',#47327,1000.);
#13609=VECTOR('',#47328,1000.);
#13610=VECTOR('',#47329,1000.);
#13611=VECTOR('',#47330,1000.);
#13612=VECTOR('',#47331,1000.);
#13613=VECTOR('',#47332,1000.);
#13614=VECTOR('',#47333,1000.);
#13615=VECTOR('',#47334,1000.);
#13616=VECTOR('',#47335,1000.);
#13617=VECTOR('',#47336,1000.);
#13618=VECTOR('',#47337,1000.);
#13619=VECTOR('',#47338,1000.);
#13620=VECTOR('',#47339,1000.);
#13621=VECTOR('',#47340,1000.);
#13622=VECTOR('',#47341,1000.);
#13623=VECTOR('',#47342,1000.);
#13624=VECTOR('',#47343,1000.);
#13625=VECTOR('',#47344,1000.);
#13626=VECTOR('',#47345,1000.);
#13627=VECTOR('',#47346,1000.);
#13628=VECTOR('',#47347,1000.);
#13629=VECTOR('',#47348,1000.);
#13630=VECTOR('',#47349,1000.);
#13631=VECTOR('',#47350,1000.);
#13632=VECTOR('',#47351,1000.);
#13633=VECTOR('',#47352,1000.);
#13634=VECTOR('',#47353,1000.);
#13635=VECTOR('',#47354,1000.);
#13636=VECTOR('',#47355,1000.);
#13637=VECTOR('',#47356,1000.);
#13638=VECTOR('',#47357,1000.);
#13639=VECTOR('',#47358,1000.);
#13640=VECTOR('',#47359,1000.);
#13641=VECTOR('',#47360,1000.);
#13642=VECTOR('',#47361,1000.);
#13643=VECTOR('',#47362,1000.);
#13644=VECTOR('',#47363,1000.);
#13645=VECTOR('',#47364,1000.);
#13646=VECTOR('',#47365,1000.);
#13647=VECTOR('',#47366,1000.);
#13648=VECTOR('',#47367,1000.);
#13649=VECTOR('',#47368,1000.);
#13650=VECTOR('',#47369,1000.);
#13651=VECTOR('',#47370,1000.);
#13652=VECTOR('',#47371,1000.);
#13653=VECTOR('',#47372,1000.);
#13654=VECTOR('',#47373,1000.);
#13655=VECTOR('',#47374,1000.);
#13656=VECTOR('',#47375,1000.);
#13657=VECTOR('',#47376,1000.);
#13658=VECTOR('',#47377,1000.);
#13659=VECTOR('',#47378,1000.);
#13660=VECTOR('',#47379,1000.);
#13661=VECTOR('',#47380,1000.);
#13662=VECTOR('',#47381,1000.);
#13663=VECTOR('',#47382,1000.);
#13664=VECTOR('',#47383,1000.);
#13665=VECTOR('',#47384,1000.);
#13666=VECTOR('',#47385,1000.);
#13667=VECTOR('',#47386,1000.);
#13668=VECTOR('',#47387,1000.);
#13669=VECTOR('',#47388,1000.);
#13670=VECTOR('',#47389,1000.);
#13671=VECTOR('',#47390,1000.);
#13672=VECTOR('',#47391,1000.);
#13673=VECTOR('',#47392,1000.);
#13674=VECTOR('',#47393,1000.);
#13675=VECTOR('',#47394,1000.);
#13676=VECTOR('',#47395,1000.);
#13677=VECTOR('',#47396,1000.);
#13678=VECTOR('',#47397,1000.);
#13679=VECTOR('',#47398,1000.);
#13680=VECTOR('',#47399,1000.);
#13681=VECTOR('',#47400,1000.);
#13682=VECTOR('',#47401,1000.);
#13683=VECTOR('',#47402,1000.);
#13684=VECTOR('',#47403,1000.);
#13685=VECTOR('',#47404,1000.);
#13686=VECTOR('',#47405,1000.);
#13687=VECTOR('',#47406,1000.);
#13688=VECTOR('',#47407,1000.);
#13689=VECTOR('',#47408,1000.);
#13690=VECTOR('',#47409,1000.);
#13691=VECTOR('',#47410,1000.);
#13692=VECTOR('',#47411,1000.);
#13693=VECTOR('',#47412,1000.);
#13694=VECTOR('',#47413,1000.);
#13695=VECTOR('',#47414,1000.);
#13696=VECTOR('',#47415,1000.);
#13697=VECTOR('',#47416,1000.);
#13698=VECTOR('',#47417,1000.);
#13699=VECTOR('',#47418,1000.);
#13700=VECTOR('',#47419,1000.);
#13701=VECTOR('',#47420,1000.);
#13702=VECTOR('',#47421,1000.);
#13703=VECTOR('',#47422,1000.);
#13704=VECTOR('',#47423,1000.);
#13705=VECTOR('',#47424,1000.);
#13706=VECTOR('',#47425,1000.);
#13707=VECTOR('',#47426,1000.);
#13708=VECTOR('',#47427,1000.);
#13709=VECTOR('',#47428,1000.);
#13710=VECTOR('',#47429,1000.);
#13711=VECTOR('',#47430,1000.);
#13712=VECTOR('',#47431,1000.);
#13713=VECTOR('',#47432,1000.);
#13714=VECTOR('',#47433,1000.);
#13715=VECTOR('',#47434,1000.);
#13716=VECTOR('',#47435,1000.);
#13717=VECTOR('',#47436,1000.);
#13718=VECTOR('',#47437,1000.);
#13719=VECTOR('',#47438,1000.);
#13720=VECTOR('',#47439,1000.);
#13721=VECTOR('',#47440,1000.);
#13722=VECTOR('',#47441,1000.);
#13723=VECTOR('',#47442,1000.);
#13724=VECTOR('',#47443,1000.);
#13725=VECTOR('',#47444,1000.);
#13726=VECTOR('',#47445,1000.);
#13727=VECTOR('',#47446,1000.);
#13728=VECTOR('',#47447,1000.);
#13729=VECTOR('',#47448,1000.);
#13730=VECTOR('',#47449,1000.);
#13731=VECTOR('',#47450,1000.);
#13732=VECTOR('',#47451,1000.);
#13733=VECTOR('',#47452,1000.);
#13734=VECTOR('',#47453,1000.);
#13735=VECTOR('',#47454,1000.);
#13736=VECTOR('',#47455,1000.);
#13737=VECTOR('',#47456,1000.);
#13738=VECTOR('',#47457,1000.);
#13739=VECTOR('',#47458,1000.);
#13740=VECTOR('',#47459,1000.);
#13741=VECTOR('',#47460,1000.);
#13742=VECTOR('',#47461,1000.);
#13743=VECTOR('',#47462,1000.);
#13744=VECTOR('',#47463,1000.);
#13745=VECTOR('',#47464,1000.);
#13746=VECTOR('',#47465,1000.);
#13747=VECTOR('',#47466,1000.);
#13748=VECTOR('',#47467,1000.);
#13749=VECTOR('',#47468,1000.);
#13750=VECTOR('',#47469,1000.);
#13751=VECTOR('',#47470,1000.);
#13752=VECTOR('',#47471,1000.);
#13753=VECTOR('',#47472,1000.);
#13754=VECTOR('',#47473,1000.);
#13755=VECTOR('',#47474,1000.);
#13756=VECTOR('',#47475,1000.);
#13757=VECTOR('',#47476,1000.);
#13758=VECTOR('',#47477,1000.);
#13759=VECTOR('',#47478,1000.);
#13760=VECTOR('',#47479,1000.);
#13761=VECTOR('',#47480,1000.);
#13762=VECTOR('',#47481,1000.);
#13763=VECTOR('',#47482,1000.);
#13764=VECTOR('',#47483,1000.);
#13765=VECTOR('',#47484,1000.);
#13766=VECTOR('',#47485,1000.);
#13767=VECTOR('',#47486,1000.);
#13768=VECTOR('',#47487,1000.);
#13769=VECTOR('',#47488,1000.);
#13770=VECTOR('',#47489,1000.);
#13771=VECTOR('',#47490,1000.);
#13772=VECTOR('',#47491,1000.);
#13773=VECTOR('',#47492,1000.);
#13774=VECTOR('',#47493,1000.);
#13775=VECTOR('',#47494,1000.);
#13776=VECTOR('',#47495,1000.);
#13777=VECTOR('',#47496,1000.);
#13778=VECTOR('',#47497,1000.);
#13779=VECTOR('',#47498,1000.);
#13780=VECTOR('',#47499,1000.);
#13781=VECTOR('',#47500,1000.);
#13782=VECTOR('',#47501,1000.);
#13783=VECTOR('',#47502,1000.);
#13784=VECTOR('',#47503,1000.);
#13785=VECTOR('',#47504,1000.);
#13786=VECTOR('',#47505,1000.);
#13787=VECTOR('',#47506,1000.);
#13788=VECTOR('',#47507,1000.);
#13789=VECTOR('',#47508,1000.);
#13790=VECTOR('',#47509,1000.);
#13791=VECTOR('',#47510,1000.);
#13792=VECTOR('',#47511,1000.);
#13793=VECTOR('',#47512,1000.);
#13794=VECTOR('',#47513,1000.);
#13795=VECTOR('',#47514,1000.);
#13796=VECTOR('',#47515,1000.);
#13797=VECTOR('',#47516,1000.);
#13798=VECTOR('',#47517,1000.);
#13799=VECTOR('',#47518,1000.);
#13800=VECTOR('',#47519,1000.);
#13801=VECTOR('',#47520,1000.);
#13802=VECTOR('',#47521,1000.);
#13803=VECTOR('',#47522,1000.);
#13804=VECTOR('',#47523,1000.);
#13805=VECTOR('',#47524,1000.);
#13806=VECTOR('',#47525,1000.);
#13807=VECTOR('',#47526,1000.);
#13808=VECTOR('',#47527,1000.);
#13809=VECTOR('',#47528,1000.);
#13810=VECTOR('',#47529,1000.);
#13811=VECTOR('',#47530,1000.);
#13812=VECTOR('',#47531,1000.);
#13813=VECTOR('',#47532,1000.);
#13814=VECTOR('',#47533,1000.);
#13815=VECTOR('',#47534,1000.);
#13816=VECTOR('',#47535,1000.);
#13817=VECTOR('',#47536,1000.);
#13818=VECTOR('',#47537,1000.);
#13819=VECTOR('',#47538,1000.);
#13820=VECTOR('',#47539,1000.);
#13821=VECTOR('',#47540,1000.);
#13822=VECTOR('',#47541,1000.);
#13823=VECTOR('',#47542,1000.);
#13824=VECTOR('',#47543,1000.);
#13825=VECTOR('',#47544,1000.);
#13826=VECTOR('',#47545,1000.);
#13827=VECTOR('',#47546,1000.);
#13828=VECTOR('',#47547,1000.);
#13829=VECTOR('',#47548,1000.);
#13830=VECTOR('',#47549,1000.);
#13831=VECTOR('',#47550,1000.);
#13832=VECTOR('',#47551,1000.);
#13833=VECTOR('',#47552,1000.);
#13834=VECTOR('',#47553,1000.);
#13835=VECTOR('',#47554,1000.);
#13836=VECTOR('',#47555,1000.);
#13837=VECTOR('',#47556,1000.);
#13838=VECTOR('',#47557,1000.);
#13839=VECTOR('',#47558,1000.);
#13840=VECTOR('',#47559,1000.);
#13841=VECTOR('',#47560,1000.);
#13842=VECTOR('',#47561,1000.);
#13843=VECTOR('',#47562,1000.);
#13844=VECTOR('',#47563,1000.);
#13845=VECTOR('',#47564,1000.);
#13846=VECTOR('',#47565,1000.);
#13847=VECTOR('',#47566,1000.);
#13848=VECTOR('',#47567,1000.);
#13849=VECTOR('',#47568,1000.);
#13850=VECTOR('',#47569,1000.);
#13851=VECTOR('',#47570,1000.);
#13852=VECTOR('',#47571,1000.);
#13853=VECTOR('',#47572,1000.);
#13854=VECTOR('',#47573,1000.);
#13855=VECTOR('',#47574,1000.);
#13856=VECTOR('',#47575,1000.);
#13857=VECTOR('',#47576,1000.);
#13858=VECTOR('',#47577,1000.);
#13859=VECTOR('',#47578,1000.);
#13860=VECTOR('',#47579,1000.);
#13861=VECTOR('',#47580,1000.);
#13862=VECTOR('',#47581,1000.);
#13863=VECTOR('',#47582,1000.);
#13864=VECTOR('',#47583,1000.);
#13865=VECTOR('',#47584,1000.);
#13866=VECTOR('',#47585,1000.);
#13867=VECTOR('',#47586,1000.);
#13868=VECTOR('',#47587,1000.);
#13869=VECTOR('',#47588,1000.);
#13870=VECTOR('',#47589,1000.);
#13871=VECTOR('',#47590,1000.);
#13872=VECTOR('',#47591,1000.);
#13873=VECTOR('',#47592,1000.);
#13874=VECTOR('',#47593,1000.);
#13875=VECTOR('',#47594,1000.);
#13876=VECTOR('',#47595,1000.);
#13877=VECTOR('',#47596,1000.);
#13878=VECTOR('',#47597,1000.);
#13879=VECTOR('',#47598,1000.);
#13880=VECTOR('',#47599,1000.);
#13881=VECTOR('',#47600,1000.);
#13882=VECTOR('',#47601,1000.);
#13883=VECTOR('',#47602,1000.);
#13884=VECTOR('',#47603,1000.);
#13885=VECTOR('',#47604,1000.);
#13886=VECTOR('',#47605,1000.);
#13887=VECTOR('',#47606,1000.);
#13888=VECTOR('',#47607,1000.);
#13889=VECTOR('',#47608,1000.);
#13890=VECTOR('',#47609,1000.);
#13891=VECTOR('',#47610,1000.);
#13892=VECTOR('',#47611,1000.);
#13893=VECTOR('',#47612,1000.);
#13894=VECTOR('',#47613,1000.);
#13895=VECTOR('',#47614,1000.);
#13896=VECTOR('',#47615,1000.);
#13897=VECTOR('',#47616,1000.);
#13898=VECTOR('',#47617,1000.);
#13899=VECTOR('',#47618,1000.);
#13900=VECTOR('',#47619,1000.);
#13901=VECTOR('',#47620,1000.);
#13902=VECTOR('',#47621,1000.);
#13903=VECTOR('',#47622,1000.);
#13904=VECTOR('',#47623,1000.);
#13905=VECTOR('',#47624,1000.);
#13906=VECTOR('',#47625,1000.);
#13907=VECTOR('',#47626,1000.);
#13908=VECTOR('',#47627,1000.);
#13909=VECTOR('',#47628,1000.);
#13910=VECTOR('',#47629,1000.);
#13911=VECTOR('',#47630,1000.);
#13912=VECTOR('',#47631,1000.);
#13913=VECTOR('',#47632,1000.);
#13914=VECTOR('',#47633,1000.);
#13915=VECTOR('',#47634,1000.);
#13916=VECTOR('',#47635,1000.);
#13917=VECTOR('',#47636,1000.);
#13918=VECTOR('',#47637,1000.);
#13919=VECTOR('',#47638,1000.);
#13920=VECTOR('',#47639,1000.);
#13921=VECTOR('',#47640,1000.);
#13922=VECTOR('',#47641,1000.);
#13923=VECTOR('',#47642,1000.);
#13924=VECTOR('',#47643,1000.);
#13925=VECTOR('',#47644,1000.);
#13926=VECTOR('',#47645,1000.);
#13927=VECTOR('',#47646,1000.);
#13928=VECTOR('',#47647,1000.);
#13929=VECTOR('',#47648,1000.);
#13930=VECTOR('',#47649,1000.);
#13931=VECTOR('',#47650,1000.);
#13932=VECTOR('',#47651,1000.);
#13933=VECTOR('',#47652,1000.);
#13934=VECTOR('',#47653,1000.);
#13935=VECTOR('',#47654,1000.);
#13936=VECTOR('',#47655,1000.);
#13937=VECTOR('',#47656,1000.);
#13938=VECTOR('',#47657,1000.);
#13939=VECTOR('',#47658,1000.);
#13940=VECTOR('',#47659,1000.);
#13941=VECTOR('',#47660,1000.);
#13942=VECTOR('',#47661,1000.);
#13943=VECTOR('',#47662,1000.);
#13944=VECTOR('',#47663,1000.);
#13945=VECTOR('',#47664,1000.);
#13946=VECTOR('',#47665,1000.);
#13947=VECTOR('',#47666,1000.);
#13948=VECTOR('',#47667,1000.);
#13949=VECTOR('',#47668,1000.);
#13950=VECTOR('',#47669,1000.);
#13951=VECTOR('',#47670,1000.);
#13952=VECTOR('',#47671,1000.);
#13953=VECTOR('',#47672,1000.);
#13954=VECTOR('',#47673,1000.);
#13955=VECTOR('',#47674,1000.);
#13956=VECTOR('',#47675,1000.);
#13957=VECTOR('',#47676,1000.);
#13958=VECTOR('',#47677,1000.);
#13959=VECTOR('',#47678,1000.);
#13960=VECTOR('',#47679,1000.);
#13961=VECTOR('',#47680,1000.);
#13962=VECTOR('',#47681,1000.);
#13963=VECTOR('',#47682,1000.);
#13964=VECTOR('',#47683,1000.);
#13965=VECTOR('',#47684,1000.);
#13966=VECTOR('',#47685,1000.);
#13967=VECTOR('',#47686,1000.);
#13968=VECTOR('',#47687,1000.);
#13969=VECTOR('',#47688,1000.);
#13970=VECTOR('',#47689,1000.);
#13971=VECTOR('',#47690,1000.);
#13972=VECTOR('',#47691,1000.);
#13973=VECTOR('',#47692,1000.);
#13974=VECTOR('',#47693,1000.);
#13975=VECTOR('',#47694,1000.);
#13976=VECTOR('',#47695,1000.);
#13977=VECTOR('',#47696,1000.);
#13978=VECTOR('',#47697,1000.);
#13979=VECTOR('',#47698,1000.);
#13980=VECTOR('',#47699,1000.);
#13981=VECTOR('',#47700,1000.);
#13982=VECTOR('',#47701,1000.);
#13983=VECTOR('',#47702,1000.);
#13984=VECTOR('',#47703,1000.);
#13985=VECTOR('',#47704,1000.);
#13986=VECTOR('',#47705,1000.);
#13987=VECTOR('',#47706,1000.);
#13988=VECTOR('',#47707,1000.);
#13989=VECTOR('',#47708,1000.);
#13990=VECTOR('',#47709,1000.);
#13991=VECTOR('',#47710,1000.);
#13992=VECTOR('',#47711,1000.);
#13993=VECTOR('',#47712,1000.);
#13994=VECTOR('',#47713,1000.);
#13995=VECTOR('',#47714,1000.);
#13996=VECTOR('',#47715,1000.);
#13997=VECTOR('',#47716,1000.);
#13998=VECTOR('',#47717,1000.);
#13999=VECTOR('',#47718,1000.);
#14000=VECTOR('',#47719,1000.);
#14001=VECTOR('',#47720,1000.);
#14002=VECTOR('',#47721,1000.);
#14003=VECTOR('',#47722,1000.);
#14004=VECTOR('',#47723,1000.);
#14005=VECTOR('',#47724,1000.);
#14006=VECTOR('',#47725,1000.);
#14007=VECTOR('',#47726,1000.);
#14008=VECTOR('',#47727,1000.);
#14009=VECTOR('',#47728,1000.);
#14010=VECTOR('',#47729,1000.);
#14011=VECTOR('',#47730,1000.);
#14012=VECTOR('',#47731,1000.);
#14013=VECTOR('',#47732,1000.);
#14014=VECTOR('',#47733,1000.);
#14015=VECTOR('',#47734,1000.);
#14016=VECTOR('',#47735,1000.);
#14017=VECTOR('',#47736,1000.);
#14018=VECTOR('',#47737,1000.);
#14019=VECTOR('',#47738,1000.);
#14020=VECTOR('',#47739,1000.);
#14021=VECTOR('',#47740,1000.);
#14022=VECTOR('',#47741,1000.);
#14023=VECTOR('',#47742,1000.);
#14024=VECTOR('',#47743,1000.);
#14025=VECTOR('',#47744,1000.);
#14026=VECTOR('',#47745,1000.);
#14027=VECTOR('',#47746,1000.);
#14028=VECTOR('',#47747,1000.);
#14029=VECTOR('',#47748,1000.);
#14030=VECTOR('',#47749,1000.);
#14031=VECTOR('',#47750,1000.);
#14032=VECTOR('',#47751,1000.);
#14033=VECTOR('',#47752,1000.);
#14034=VECTOR('',#47753,1000.);
#14035=VECTOR('',#47754,1000.);
#14036=VECTOR('',#47755,1000.);
#14037=VECTOR('',#47756,1000.);
#14038=VECTOR('',#47757,1000.);
#14039=VECTOR('',#47758,1000.);
#14040=VECTOR('',#47759,1000.);
#14041=VECTOR('',#47760,1000.);
#14042=VECTOR('',#47761,1000.);
#14043=VECTOR('',#47762,1000.);
#14044=VECTOR('',#47763,1000.);
#14045=VECTOR('',#47764,1000.);
#14046=VECTOR('',#47765,1000.);
#14047=VECTOR('',#47766,1000.);
#14048=VECTOR('',#47767,1000.);
#14049=VECTOR('',#47768,1000.);
#14050=VECTOR('',#47769,1000.);
#14051=VECTOR('',#47770,1000.);
#14052=VECTOR('',#47771,1000.);
#14053=VECTOR('',#47772,1000.);
#14054=VECTOR('',#47773,1000.);
#14055=VECTOR('',#47774,1000.);
#14056=VECTOR('',#47775,1000.);
#14057=VECTOR('',#47776,1000.);
#14058=VECTOR('',#47777,1000.);
#14059=VECTOR('',#47778,1000.);
#14060=VECTOR('',#47779,1000.);
#14061=VECTOR('',#47780,1000.);
#14062=VECTOR('',#47781,1000.);
#14063=VECTOR('',#47782,1000.);
#14064=VECTOR('',#47783,1000.);
#14065=VECTOR('',#47784,1000.);
#14066=VECTOR('',#47785,1000.);
#14067=VECTOR('',#47786,1000.);
#14068=VECTOR('',#47787,1000.);
#14069=VECTOR('',#47788,1000.);
#14070=VECTOR('',#47789,1000.);
#14071=VECTOR('',#47790,1000.);
#14072=VECTOR('',#47791,1000.);
#14073=VECTOR('',#47792,1000.);
#14074=VECTOR('',#47793,1000.);
#14075=VECTOR('',#47794,1000.);
#14076=VECTOR('',#47795,1000.);
#14077=VECTOR('',#47796,1000.);
#14078=VECTOR('',#47797,1000.);
#14079=VECTOR('',#47798,1000.);
#14080=VECTOR('',#47799,1000.);
#14081=VECTOR('',#47800,1000.);
#14082=VECTOR('',#47801,1000.);
#14083=VECTOR('',#47802,1000.);
#14084=VECTOR('',#47803,1000.);
#14085=VECTOR('',#47804,1000.);
#14086=VECTOR('',#47805,1000.);
#14087=VECTOR('',#47806,1000.);
#14088=VECTOR('',#47807,1000.);
#14089=VECTOR('',#47808,1000.);
#14090=VECTOR('',#47809,1000.);
#14091=VECTOR('',#47810,1000.);
#14092=VECTOR('',#47811,1000.);
#14093=VECTOR('',#47812,1000.);
#14094=VECTOR('',#47813,1000.);
#14095=VECTOR('',#47814,1000.);
#14096=VECTOR('',#47815,1000.);
#14097=VECTOR('',#47816,1000.);
#14098=VECTOR('',#47817,1000.);
#14099=VECTOR('',#47818,1000.);
#14100=VECTOR('',#47819,1000.);
#14101=VECTOR('',#47820,1000.);
#14102=VECTOR('',#47821,1000.);
#14103=VECTOR('',#47822,1000.);
#14104=VECTOR('',#47823,1000.);
#14105=VECTOR('',#47824,1000.);
#14106=VECTOR('',#47825,1000.);
#14107=VECTOR('',#47826,1000.);
#14108=VECTOR('',#47827,1000.);
#14109=VECTOR('',#47828,1000.);
#14110=VECTOR('',#47829,1000.);
#14111=VECTOR('',#47830,1000.);
#14112=VECTOR('',#47831,1000.);
#14113=VECTOR('',#47832,1000.);
#14114=VECTOR('',#47833,1000.);
#14115=VECTOR('',#47834,1000.);
#14116=VECTOR('',#47835,1000.);
#14117=VECTOR('',#47836,1000.);
#14118=VECTOR('',#47837,1000.);
#14119=VECTOR('',#47838,1000.);
#14120=VECTOR('',#47839,1000.);
#14121=VECTOR('',#47840,1000.);
#14122=VECTOR('',#47841,1000.);
#14123=VECTOR('',#47842,1000.);
#14124=VECTOR('',#47843,1000.);
#14125=VECTOR('',#47844,1000.);
#14126=VECTOR('',#47845,1000.);
#14127=VECTOR('',#47846,1000.);
#14128=VECTOR('',#47847,1000.);
#14129=VECTOR('',#47848,1000.);
#14130=VECTOR('',#47849,1000.);
#14131=VECTOR('',#47850,1000.);
#14132=VECTOR('',#47851,1000.);
#14133=VECTOR('',#47852,1000.);
#14134=VECTOR('',#47853,1000.);
#14135=VECTOR('',#47854,1000.);
#14136=VECTOR('',#47855,1000.);
#14137=VECTOR('',#47856,1000.);
#14138=VECTOR('',#47857,1000.);
#14139=VECTOR('',#47858,1000.);
#14140=VECTOR('',#47859,1000.);
#14141=VECTOR('',#47860,1000.);
#14142=VECTOR('',#47861,1000.);
#14143=VECTOR('',#47862,1000.);
#14144=VECTOR('',#47863,1000.);
#14145=VECTOR('',#47864,1000.);
#14146=VECTOR('',#47865,1000.);
#14147=VECTOR('',#47866,1000.);
#14148=VECTOR('',#47867,1000.);
#14149=VECTOR('',#47868,1000.);
#14150=VECTOR('',#47869,1000.);
#14151=VECTOR('',#47870,1000.);
#14152=VECTOR('',#47871,1000.);
#14153=VECTOR('',#47872,1000.);
#14154=VECTOR('',#47873,1000.);
#14155=VECTOR('',#47874,1000.);
#14156=VECTOR('',#47875,1000.);
#14157=VECTOR('',#47876,1000.);
#14158=VECTOR('',#47877,1000.);
#14159=VECTOR('',#47878,1000.);
#14160=VECTOR('',#47879,1000.);
#14161=VECTOR('',#47880,1000.);
#14162=VECTOR('',#47881,1000.);
#14163=VECTOR('',#47882,1000.);
#14164=VECTOR('',#47883,1000.);
#14165=VECTOR('',#47884,1000.);
#14166=VECTOR('',#47885,1000.);
#14167=VECTOR('',#47886,1000.);
#14168=VECTOR('',#47887,1000.);
#14169=VECTOR('',#47888,1000.);
#14170=VECTOR('',#47889,1000.);
#14171=VECTOR('',#47890,1000.);
#14172=VECTOR('',#47891,1000.);
#14173=VECTOR('',#47892,1000.);
#14174=VECTOR('',#47893,1000.);
#14175=VECTOR('',#47894,1000.);
#14176=VECTOR('',#47895,1000.);
#14177=VECTOR('',#47896,1000.);
#14178=VECTOR('',#47897,1000.);
#14179=VECTOR('',#47898,1000.);
#14180=VECTOR('',#47899,1000.);
#14181=VECTOR('',#47900,1000.);
#14182=VECTOR('',#47901,1000.);
#14183=VECTOR('',#47902,1000.);
#14184=VECTOR('',#47903,1000.);
#14185=VECTOR('',#47904,1000.);
#14186=VECTOR('',#47905,1000.);
#14187=VECTOR('',#47906,1000.);
#14188=VECTOR('',#47907,1000.);
#14189=VECTOR('',#47908,1000.);
#14190=VECTOR('',#47909,1000.);
#14191=VECTOR('',#47910,1000.);
#14192=VECTOR('',#47911,1000.);
#14193=VECTOR('',#47912,1000.);
#14194=VECTOR('',#47913,1000.);
#14195=VECTOR('',#47914,1000.);
#14196=VECTOR('',#47915,1000.);
#14197=VECTOR('',#47916,1000.);
#14198=VECTOR('',#47917,1000.);
#14199=VECTOR('',#47918,1000.);
#14200=VECTOR('',#47919,1000.);
#14201=VECTOR('',#47920,1000.);
#14202=VECTOR('',#47921,1000.);
#14203=VECTOR('',#47922,1000.);
#14204=VECTOR('',#47923,1000.);
#14205=VECTOR('',#47924,1000.);
#14206=VECTOR('',#47925,1000.);
#14207=VECTOR('',#47926,1000.);
#14208=VECTOR('',#47927,1000.);
#14209=VECTOR('',#47928,1000.);
#14210=VECTOR('',#47929,1000.);
#14211=VECTOR('',#47930,1000.);
#14212=VECTOR('',#47931,1000.);
#14213=VECTOR('',#47932,1000.);
#14214=VECTOR('',#47933,1000.);
#14215=VECTOR('',#47934,1000.);
#14216=VECTOR('',#47935,1000.);
#14217=VECTOR('',#47936,1000.);
#14218=VECTOR('',#47937,1000.);
#14219=VECTOR('',#47938,1000.);
#14220=VECTOR('',#47939,1000.);
#14221=VECTOR('',#47940,1000.);
#14222=VECTOR('',#47941,1000.);
#14223=VECTOR('',#47942,1000.);
#14224=VECTOR('',#47943,1000.);
#14225=VECTOR('',#47944,1000.);
#14226=VECTOR('',#47945,1000.);
#14227=VECTOR('',#47946,1000.);
#14228=VECTOR('',#47947,1000.);
#14229=VECTOR('',#47948,1000.);
#14230=VECTOR('',#47949,1000.);
#14231=VECTOR('',#47950,1000.);
#14232=VECTOR('',#47951,1000.);
#14233=VECTOR('',#47952,1000.);
#14234=VECTOR('',#47953,1000.);
#14235=VECTOR('',#47954,1000.);
#14236=VECTOR('',#47955,1000.);
#14237=VECTOR('',#47956,1000.);
#14238=VECTOR('',#47957,1000.);
#14239=VECTOR('',#47958,1000.);
#14240=VECTOR('',#47959,1000.);
#14241=VECTOR('',#47960,1000.);
#14242=VECTOR('',#47961,1000.);
#14243=VECTOR('',#47962,1000.);
#14244=VECTOR('',#47963,1000.);
#14245=VECTOR('',#47964,1000.);
#14246=VECTOR('',#47965,1000.);
#14247=VECTOR('',#47966,1000.);
#14248=VECTOR('',#47967,1000.);
#14249=VECTOR('',#47968,1000.);
#14250=VECTOR('',#47969,1000.);
#14251=VECTOR('',#47970,1000.);
#14252=VECTOR('',#47971,1000.);
#14253=VECTOR('',#47972,1000.);
#14254=VECTOR('',#47973,1000.);
#14255=VECTOR('',#47974,1000.);
#14256=VECTOR('',#47975,1000.);
#14257=VECTOR('',#47976,1000.);
#14258=VECTOR('',#47979,1000.);
#14259=VECTOR('',#47980,1000.);
#14260=VECTOR('',#47981,1000.);
#14261=VECTOR('',#47982,1000.);
#14262=VECTOR('',#47983,1000.);
#14263=VECTOR('',#47984,1000.);
#14264=VECTOR('',#47985,1000.);
#14265=VECTOR('',#47986,1000.);
#14266=VECTOR('',#47987,1000.);
#14267=VECTOR('',#47988,1000.);
#14268=VECTOR('',#47989,1000.);
#14269=VECTOR('',#47990,1000.);
#14270=VECTOR('',#47991,1000.);
#14271=VECTOR('',#47992,1000.);
#14272=VECTOR('',#47993,1000.);
#14273=VECTOR('',#47994,1000.);
#14274=VECTOR('',#47995,1000.);
#14275=VECTOR('',#47996,1000.);
#14276=VECTOR('',#47997,1000.);
#14277=VECTOR('',#47998,1000.);
#14278=VECTOR('',#47999,1000.);
#14279=VECTOR('',#48000,1000.);
#14280=VECTOR('',#48001,1000.);
#14281=VECTOR('',#48002,1000.);
#14282=VECTOR('',#48003,1000.);
#14283=VECTOR('',#48004,1000.);
#14284=VECTOR('',#48005,1000.);
#14285=VECTOR('',#48006,1000.);
#14286=VECTOR('',#48007,1000.);
#14287=VECTOR('',#48008,1000.);
#14288=VECTOR('',#48009,1000.);
#14289=VECTOR('',#48010,1000.);
#14290=VECTOR('',#48011,1000.);
#14291=VECTOR('',#48012,1000.);
#14292=VECTOR('',#48013,1000.);
#14293=VECTOR('',#48014,1000.);
#14294=VECTOR('',#48015,1000.);
#14295=VECTOR('',#48016,1000.);
#14296=VECTOR('',#48017,1000.);
#14297=VECTOR('',#48018,1000.);
#14298=VECTOR('',#48019,1000.);
#14299=VECTOR('',#48020,1000.);
#14300=VECTOR('',#48021,1000.);
#14301=VECTOR('',#48022,1000.);
#14302=VECTOR('',#48023,1000.);
#14303=VECTOR('',#48024,1000.);
#14304=VECTOR('',#48025,1000.);
#14305=VECTOR('',#48026,1000.);
#14306=VECTOR('',#48027,1000.);
#14307=VECTOR('',#48028,1000.);
#14308=VECTOR('',#48029,1000.);
#14309=VECTOR('',#48030,1000.);
#14310=VECTOR('',#48031,1000.);
#14311=VECTOR('',#48032,1000.);
#14312=VECTOR('',#48033,1000.);
#14313=VECTOR('',#48034,1000.);
#14314=VECTOR('',#48035,1000.);
#14315=VECTOR('',#48036,1000.);
#14316=VECTOR('',#48037,1000.);
#14317=VECTOR('',#48038,1000.);
#14318=VECTOR('',#48039,1000.);
#14319=VECTOR('',#48040,1000.);
#14320=VECTOR('',#48041,1000.);
#14321=VECTOR('',#48042,1000.);
#14322=VECTOR('',#48043,1000.);
#14323=VECTOR('',#48044,1000.);
#14324=VECTOR('',#48045,1000.);
#14325=VECTOR('',#48046,1000.);
#14326=VECTOR('',#48047,1000.);
#14327=VECTOR('',#48048,1000.);
#14328=VECTOR('',#48049,1000.);
#14329=VECTOR('',#48050,1000.);
#14330=VECTOR('',#48051,1000.);
#14331=VECTOR('',#48052,1000.);
#14332=VECTOR('',#48053,1000.);
#14333=VECTOR('',#48054,1000.);
#14334=VECTOR('',#48055,1000.);
#14335=VECTOR('',#48056,1000.);
#14336=VECTOR('',#48057,1000.);
#14337=VECTOR('',#48058,1000.);
#14338=VECTOR('',#48059,1000.);
#14339=VECTOR('',#48060,1000.);
#14340=VECTOR('',#48061,1000.);
#14341=VECTOR('',#48062,1000.);
#14342=VECTOR('',#48063,1000.);
#14343=VECTOR('',#48064,1000.);
#14344=VECTOR('',#48065,1000.);
#14345=VECTOR('',#48066,1000.);
#14346=VECTOR('',#48067,1000.);
#14347=VECTOR('',#48068,1000.);
#14348=VECTOR('',#48069,1000.);
#14349=VECTOR('',#48070,1000.);
#14350=VECTOR('',#48071,1000.);
#14351=VECTOR('',#48072,1000.);
#14352=VECTOR('',#48073,1000.);
#14353=VECTOR('',#48074,1000.);
#14354=VECTOR('',#48075,1000.);
#14355=VECTOR('',#48076,1000.);
#14356=VECTOR('',#48077,1000.);
#14357=VECTOR('',#48078,1000.);
#14358=VECTOR('',#48079,1000.);
#14359=VECTOR('',#48080,1000.);
#14360=VECTOR('',#48081,1000.);
#14361=VECTOR('',#48082,1000.);
#14362=VECTOR('',#48083,1000.);
#14363=VECTOR('',#48084,1000.);
#14364=VECTOR('',#48085,1000.);
#14365=VECTOR('',#48086,1000.);
#14366=VECTOR('',#48087,1000.);
#14367=VECTOR('',#48088,1000.);
#14368=VECTOR('',#48089,1000.);
#14369=VECTOR('',#48090,1000.);
#14370=VECTOR('',#48091,1000.);
#14371=VECTOR('',#48092,1000.);
#14372=VECTOR('',#48093,1000.);
#14373=VECTOR('',#48094,1000.);
#14374=VECTOR('',#48095,1000.);
#14375=VECTOR('',#48096,1000.);
#14376=VECTOR('',#48097,1000.);
#14377=VECTOR('',#48098,1000.);
#14378=VECTOR('',#48099,1000.);
#14379=VECTOR('',#48100,1000.);
#14380=VECTOR('',#48101,1000.);
#14381=VECTOR('',#48102,1000.);
#14382=VECTOR('',#48103,1000.);
#14383=VECTOR('',#48104,1000.);
#14384=VECTOR('',#48105,1000.);
#14385=VECTOR('',#48106,1000.);
#14386=VECTOR('',#48107,1000.);
#14387=VECTOR('',#48108,1000.);
#14388=VECTOR('',#48109,1000.);
#14389=VECTOR('',#48110,1000.);
#14390=VECTOR('',#48111,1000.);
#14391=VECTOR('',#48112,1000.);
#14392=VECTOR('',#48113,1000.);
#14393=VECTOR('',#48114,1000.);
#14394=VECTOR('',#48115,1000.);
#14395=VECTOR('',#48116,1000.);
#14396=VECTOR('',#48117,1000.);
#14397=VECTOR('',#48118,1000.);
#14398=VECTOR('',#48119,1000.);
#14399=VECTOR('',#48120,1000.);
#14400=VECTOR('',#48121,1000.);
#14401=VECTOR('',#48122,1000.);
#14402=VECTOR('',#48123,1000.);
#14403=VECTOR('',#48124,1000.);
#14404=VECTOR('',#48125,1000.);
#14405=VECTOR('',#48126,1000.);
#14406=VECTOR('',#48127,1000.);
#14407=VECTOR('',#48128,1000.);
#14408=VECTOR('',#48129,1000.);
#14409=VECTOR('',#48130,1000.);
#14410=VECTOR('',#48131,1000.);
#14411=VECTOR('',#48132,1000.);
#14412=VECTOR('',#48133,1000.);
#14413=VECTOR('',#48134,1000.);
#14414=VECTOR('',#48135,1000.);
#14415=VECTOR('',#48136,1000.);
#14416=VECTOR('',#48137,1000.);
#14417=VECTOR('',#48138,1000.);
#14418=VECTOR('',#48139,1000.);
#14419=VECTOR('',#48140,1000.);
#14420=VECTOR('',#48141,1000.);
#14421=VECTOR('',#48142,1000.);
#14422=VECTOR('',#48143,1000.);
#14423=VECTOR('',#48144,1000.);
#14424=VECTOR('',#48145,1000.);
#14425=VECTOR('',#48146,1000.);
#14426=VECTOR('',#48147,1000.);
#14427=VECTOR('',#48148,1000.);
#14428=VECTOR('',#48149,1000.);
#14429=VECTOR('',#48150,1000.);
#14430=VECTOR('',#48151,1000.);
#14431=VECTOR('',#48152,1000.);
#14432=VECTOR('',#48153,1000.);
#14433=VECTOR('',#48154,1000.);
#14434=VECTOR('',#48155,1000.);
#14435=VECTOR('',#48156,1000.);
#14436=VECTOR('',#48157,1000.);
#14437=VECTOR('',#48158,1000.);
#14438=VECTOR('',#48159,1000.);
#14439=VECTOR('',#48160,1000.);
#14440=VECTOR('',#48161,1000.);
#14441=VECTOR('',#48162,1000.);
#14442=VECTOR('',#48163,1000.);
#14443=VECTOR('',#48164,1000.);
#14444=VECTOR('',#48165,1000.);
#14445=VECTOR('',#48166,1000.);
#14446=VECTOR('',#48167,1000.);
#14447=VECTOR('',#48168,1000.);
#14448=VECTOR('',#48169,1000.);
#14449=VECTOR('',#48170,1000.);
#14450=VECTOR('',#48171,1000.);
#14451=VECTOR('',#48172,1000.);
#14452=VECTOR('',#48173,1000.);
#14453=VECTOR('',#48174,1000.);
#14454=VECTOR('',#48175,1000.);
#14455=VECTOR('',#48176,1000.);
#14456=VECTOR('',#48177,1000.);
#14457=VECTOR('',#48178,1000.);
#14458=VECTOR('',#48179,1000.);
#14459=VECTOR('',#48180,1000.);
#14460=VECTOR('',#48181,1000.);
#14461=VECTOR('',#48182,1000.);
#14462=VECTOR('',#48183,1000.);
#14463=VECTOR('',#48184,1000.);
#14464=VECTOR('',#48185,1000.);
#14465=VECTOR('',#48186,1000.);
#14466=VECTOR('',#48187,1000.);
#14467=VECTOR('',#48188,1000.);
#14468=VECTOR('',#48189,1000.);
#14469=VECTOR('',#48190,1000.);
#14470=VECTOR('',#48191,1000.);
#14471=VECTOR('',#48192,1000.);
#14472=VECTOR('',#48193,1000.);
#14473=VECTOR('',#48194,1000.);
#14474=VECTOR('',#48195,1000.);
#14475=VECTOR('',#48196,1000.);
#14476=VECTOR('',#48197,1000.);
#14477=VECTOR('',#48198,1000.);
#14478=VECTOR('',#48199,1000.);
#14479=VECTOR('',#48200,1000.);
#14480=VECTOR('',#48201,1000.);
#14481=VECTOR('',#48202,1000.);
#14482=VECTOR('',#48203,1000.);
#14483=VECTOR('',#48204,1000.);
#14484=VECTOR('',#48205,1000.);
#14485=VECTOR('',#48206,1000.);
#14486=VECTOR('',#48207,1000.);
#14487=VECTOR('',#48208,1000.);
#14488=VECTOR('',#48209,1000.);
#14489=VECTOR('',#48210,1000.);
#14490=VECTOR('',#48211,1000.);
#14491=VECTOR('',#48212,1000.);
#14492=VECTOR('',#48213,1000.);
#14493=VECTOR('',#48214,1000.);
#14494=VECTOR('',#48215,1000.);
#14495=VECTOR('',#48216,1000.);
#14496=VECTOR('',#48217,1000.);
#14497=VECTOR('',#48218,1000.);
#14498=VECTOR('',#48219,1000.);
#14499=VECTOR('',#48220,1000.);
#14500=VECTOR('',#48221,1000.);
#14501=VECTOR('',#48222,1000.);
#14502=VECTOR('',#48223,1000.);
#14503=VECTOR('',#48224,1000.);
#14504=VECTOR('',#48225,1000.);
#14505=VECTOR('',#48226,1000.);
#14506=VECTOR('',#48227,1000.);
#14507=VECTOR('',#48228,1000.);
#14508=VECTOR('',#48229,1000.);
#14509=VECTOR('',#48230,1000.);
#14510=VECTOR('',#48231,1000.);
#14511=VECTOR('',#48232,1000.);
#14512=VECTOR('',#48233,1000.);
#14513=VECTOR('',#48234,1000.);
#14514=VECTOR('',#48235,1000.);
#14515=VECTOR('',#48236,1000.);
#14516=VECTOR('',#48237,1000.);
#14517=VECTOR('',#48238,1000.);
#14518=VECTOR('',#48239,1000.);
#14519=VECTOR('',#48240,1000.);
#14520=VECTOR('',#48241,1000.);
#14521=VECTOR('',#48242,1000.);
#14522=VECTOR('',#48243,1000.);
#14523=VECTOR('',#48244,1000.);
#14524=VECTOR('',#48245,1000.);
#14525=VECTOR('',#48246,1000.);
#14526=VECTOR('',#48247,1000.);
#14527=VECTOR('',#48248,1000.);
#14528=VECTOR('',#48249,1000.);
#14529=VECTOR('',#48250,1000.);
#14530=VECTOR('',#48251,1000.);
#14531=VECTOR('',#48252,1000.);
#14532=VECTOR('',#48253,1000.);
#14533=VECTOR('',#48254,1000.);
#14534=VECTOR('',#48255,1000.);
#14535=VECTOR('',#48256,1000.);
#14536=VECTOR('',#48257,1000.);
#14537=VECTOR('',#48258,1000.);
#14538=VECTOR('',#48259,1000.);
#14539=VECTOR('',#48260,1000.);
#14540=VECTOR('',#48261,1000.);
#14541=VECTOR('',#48262,1000.);
#14542=VECTOR('',#48263,1000.);
#14543=VECTOR('',#48264,1000.);
#14544=VECTOR('',#48265,1000.);
#14545=VECTOR('',#48266,1000.);
#14546=VECTOR('',#48267,1000.);
#14547=VECTOR('',#48268,1000.);
#14548=VECTOR('',#48269,1000.);
#14549=VECTOR('',#48270,1000.);
#14550=VECTOR('',#48271,1000.);
#14551=VECTOR('',#48272,1000.);
#14552=VECTOR('',#48273,1000.);
#14553=VECTOR('',#48274,1000.);
#14554=VECTOR('',#48275,1000.);
#14555=VECTOR('',#48276,1000.);
#14556=VECTOR('',#48277,1000.);
#14557=VECTOR('',#48278,1000.);
#14558=VECTOR('',#48279,1000.);
#14559=VECTOR('',#48280,1000.);
#14560=VECTOR('',#48281,1000.);
#14561=VECTOR('',#48282,1000.);
#14562=VECTOR('',#48283,1000.);
#14563=VECTOR('',#48284,1000.);
#14564=VECTOR('',#48285,1000.);
#14565=VECTOR('',#48286,1000.);
#14566=VECTOR('',#48287,1000.);
#14567=VECTOR('',#48288,1000.);
#14568=VECTOR('',#48289,1000.);
#14569=VECTOR('',#48290,1000.);
#14570=VECTOR('',#48291,1000.);
#14571=VECTOR('',#48292,1000.);
#14572=VECTOR('',#48293,1000.);
#14573=VECTOR('',#48294,1000.);
#14574=VECTOR('',#48295,1000.);
#14575=VECTOR('',#48296,1000.);
#14576=VECTOR('',#48297,1000.);
#14577=VECTOR('',#48298,1000.);
#14578=VECTOR('',#48299,1000.);
#14579=VECTOR('',#48300,1000.);
#14580=VECTOR('',#48301,1000.);
#14581=VECTOR('',#48302,1000.);
#14582=VECTOR('',#48303,1000.);
#14583=VECTOR('',#48304,1000.);
#14584=VECTOR('',#48305,1000.);
#14585=VECTOR('',#48306,1000.);
#14586=VECTOR('',#48307,1000.);
#14587=VECTOR('',#48308,1000.);
#14588=VECTOR('',#48309,1000.);
#14589=VECTOR('',#48310,1000.);
#14590=VECTOR('',#48311,1000.);
#14591=VECTOR('',#48312,1000.);
#14592=VECTOR('',#48313,1000.);
#14593=VECTOR('',#48314,1000.);
#14594=VECTOR('',#48315,1000.);
#14595=VECTOR('',#48316,1000.);
#14596=VECTOR('',#48317,1000.);
#14597=VECTOR('',#48318,1000.);
#14598=VECTOR('',#48319,1000.);
#14599=VECTOR('',#48320,1000.);
#14600=VECTOR('',#48321,1000.);
#14601=VECTOR('',#48322,1000.);
#14602=VECTOR('',#48323,1000.);
#14603=VECTOR('',#48324,1000.);
#14604=VECTOR('',#48325,1000.);
#14605=VECTOR('',#48326,1000.);
#14606=VECTOR('',#48327,1000.);
#14607=VECTOR('',#48328,1000.);
#14608=VECTOR('',#48329,1000.);
#14609=VECTOR('',#48330,1000.);
#14610=VECTOR('',#48331,1000.);
#14611=VECTOR('',#48332,1000.);
#14612=VECTOR('',#48333,1000.);
#14613=VECTOR('',#48334,1000.);
#14614=VECTOR('',#48335,1000.);
#14615=VECTOR('',#48336,1000.);
#14616=VECTOR('',#48337,1000.);
#14617=VECTOR('',#48338,1000.);
#14618=VECTOR('',#48339,1000.);
#14619=VECTOR('',#48340,1000.);
#14620=VECTOR('',#48341,1000.);
#14621=VECTOR('',#48342,1000.);
#14622=VECTOR('',#48343,1000.);
#14623=VECTOR('',#48344,1000.);
#14624=VECTOR('',#48345,1000.);
#14625=VECTOR('',#48346,1000.);
#14626=VECTOR('',#48347,1000.);
#14627=VECTOR('',#48348,1000.);
#14628=VECTOR('',#48349,1000.);
#14629=VECTOR('',#48350,1000.);
#14630=VECTOR('',#48351,1000.);
#14631=VECTOR('',#48352,1000.);
#14632=VECTOR('',#48353,1000.);
#14633=VECTOR('',#48354,1000.);
#14634=VECTOR('',#48355,1000.);
#14635=VECTOR('',#48356,1000.);
#14636=VECTOR('',#48357,1000.);
#14637=VECTOR('',#48358,1000.);
#14638=VECTOR('',#48359,1000.);
#14639=VECTOR('',#48360,1000.);
#14640=VECTOR('',#48361,1000.);
#14641=VECTOR('',#48362,1000.);
#14642=VECTOR('',#48363,1000.);
#14643=VECTOR('',#48364,1000.);
#14644=VECTOR('',#48365,1000.);
#14645=VECTOR('',#48366,1000.);
#14646=VECTOR('',#48367,1000.);
#14647=VECTOR('',#48368,1000.);
#14648=VECTOR('',#48369,1000.);
#14649=VECTOR('',#48370,1000.);
#14650=VECTOR('',#48371,1000.);
#14651=VECTOR('',#48372,1000.);
#14652=VECTOR('',#48373,1000.);
#14653=VECTOR('',#48374,1000.);
#14654=VECTOR('',#48375,1000.);
#14655=VECTOR('',#48376,1000.);
#14656=VECTOR('',#48377,1000.);
#14657=VECTOR('',#48378,1000.);
#14658=VECTOR('',#48379,1000.);
#14659=VECTOR('',#48380,1000.);
#14660=VECTOR('',#48381,1000.);
#14661=VECTOR('',#48382,1000.);
#14662=VECTOR('',#48383,1000.);
#14663=VECTOR('',#48384,1000.);
#14664=VECTOR('',#48385,1000.);
#14665=VECTOR('',#48386,1000.);
#14666=VECTOR('',#48387,1000.);
#14667=VECTOR('',#48388,1000.);
#14668=VECTOR('',#48389,1000.);
#14669=VECTOR('',#48390,1000.);
#14670=VECTOR('',#48391,1000.);
#14671=VECTOR('',#48392,1000.);
#14672=VECTOR('',#48393,1000.);
#14673=VECTOR('',#48394,1000.);
#14674=VECTOR('',#48395,1000.);
#14675=VECTOR('',#48396,1000.);
#14676=VECTOR('',#48397,1000.);
#14677=VECTOR('',#48398,1000.);
#14678=VECTOR('',#48399,1000.);
#14679=VECTOR('',#48400,1000.);
#14680=VECTOR('',#48401,1000.);
#14681=VECTOR('',#48402,1000.);
#14682=VECTOR('',#48403,1000.);
#14683=VECTOR('',#48404,1000.);
#14684=VECTOR('',#48405,1000.);
#14685=VECTOR('',#48406,1000.);
#14686=VECTOR('',#48407,1000.);
#14687=VECTOR('',#48408,1000.);
#14688=VECTOR('',#48409,1000.);
#14689=VECTOR('',#48410,1000.);
#14690=VECTOR('',#48411,1000.);
#14691=VECTOR('',#48412,1000.);
#14692=VECTOR('',#48413,1000.);
#14693=VECTOR('',#48414,1000.);
#14694=VECTOR('',#48415,1000.);
#14695=VECTOR('',#48416,1000.);
#14696=VECTOR('',#48417,1000.);
#14697=VECTOR('',#48418,1000.);
#14698=VECTOR('',#48419,1000.);
#14699=VECTOR('',#48420,1000.);
#14700=VECTOR('',#48421,1000.);
#14701=VECTOR('',#48422,1000.);
#14702=VECTOR('',#48423,1000.);
#14703=VECTOR('',#48424,1000.);
#14704=VECTOR('',#48425,1000.);
#14705=VECTOR('',#48426,1000.);
#14706=VECTOR('',#48427,1000.);
#14707=VECTOR('',#48428,1000.);
#14708=VECTOR('',#48429,1000.);
#14709=VECTOR('',#48430,1000.);
#14710=VECTOR('',#48431,1000.);
#14711=VECTOR('',#48432,1000.);
#14712=VECTOR('',#48433,1000.);
#14713=VECTOR('',#48434,1000.);
#14714=VECTOR('',#48435,1000.);
#14715=VECTOR('',#48436,1000.);
#14716=VECTOR('',#48437,1000.);
#14717=VECTOR('',#48438,1000.);
#14718=VECTOR('',#48439,1000.);
#14719=VECTOR('',#48440,1000.);
#14720=VECTOR('',#48441,1000.);
#14721=VECTOR('',#48442,1000.);
#14722=VECTOR('',#48443,1000.);
#14723=VECTOR('',#48444,1000.);
#14724=VECTOR('',#48445,1000.);
#14725=VECTOR('',#48446,1000.);
#14726=VECTOR('',#48447,1000.);
#14727=VECTOR('',#48448,1000.);
#14728=VECTOR('',#48449,1000.);
#14729=VECTOR('',#48450,1000.);
#14730=VECTOR('',#48451,1000.);
#14731=VECTOR('',#48452,1000.);
#14732=VECTOR('',#48453,1000.);
#14733=VECTOR('',#48454,1000.);
#14734=VECTOR('',#48455,1000.);
#14735=VECTOR('',#48456,1000.);
#14736=VECTOR('',#48457,1000.);
#14737=VECTOR('',#48458,1000.);
#14738=VECTOR('',#48459,1000.);
#14739=VECTOR('',#48460,1000.);
#14740=VECTOR('',#48461,1000.);
#14741=VECTOR('',#48462,1000.);
#14742=VECTOR('',#48463,1000.);
#14743=VECTOR('',#48464,1000.);
#14744=VECTOR('',#48465,1000.);
#14745=VECTOR('',#48466,1000.);
#14746=VECTOR('',#48467,1000.);
#14747=VECTOR('',#48468,1000.);
#14748=VECTOR('',#48469,1000.);
#14749=VECTOR('',#48470,1000.);
#14750=VECTOR('',#48471,1000.);
#14751=VECTOR('',#48472,1000.);
#14752=VECTOR('',#48473,1000.);
#14753=VECTOR('',#48474,1000.);
#14754=VECTOR('',#48475,1000.);
#14755=VECTOR('',#48476,1000.);
#14756=VECTOR('',#48477,1000.);
#14757=VECTOR('',#48478,1000.);
#14758=VECTOR('',#48479,1000.);
#14759=VECTOR('',#48480,1000.);
#14760=VECTOR('',#48481,1000.);
#14761=VECTOR('',#48482,1000.);
#14762=VECTOR('',#48483,1000.);
#14763=VECTOR('',#48484,1000.);
#14764=VECTOR('',#48485,1000.);
#14765=VECTOR('',#48486,1000.);
#14766=VECTOR('',#48487,1000.);
#14767=VECTOR('',#48488,1000.);
#14768=VECTOR('',#48489,1000.);
#14769=VECTOR('',#48490,1000.);
#14770=VECTOR('',#48491,1000.);
#14771=VECTOR('',#48492,1000.);
#14772=VECTOR('',#48493,1000.);
#14773=VECTOR('',#48494,1000.);
#14774=VECTOR('',#48495,1000.);
#14775=VECTOR('',#48496,1000.);
#14776=VECTOR('',#48497,1000.);
#14777=VECTOR('',#48498,1000.);
#14778=VECTOR('',#48499,1000.);
#14779=VECTOR('',#48500,1000.);
#14780=VECTOR('',#48501,1000.);
#14781=VECTOR('',#48502,1000.);
#14782=VECTOR('',#48503,1000.);
#14783=VECTOR('',#48504,1000.);
#14784=VECTOR('',#48505,1000.);
#14785=VECTOR('',#48506,1000.);
#14786=VECTOR('',#48507,1000.);
#14787=VECTOR('',#48508,1000.);
#14788=VECTOR('',#48509,1000.);
#14789=VECTOR('',#48510,1000.);
#14790=VECTOR('',#48511,1000.);
#14791=VECTOR('',#48512,1000.);
#14792=VECTOR('',#48513,1000.);
#14793=VECTOR('',#48514,1000.);
#14794=VECTOR('',#48515,1000.);
#14795=VECTOR('',#48516,1000.);
#14796=VECTOR('',#48517,1000.);
#14797=VECTOR('',#48518,1000.);
#14798=VECTOR('',#48519,1000.);
#14799=VECTOR('',#48520,1000.);
#14800=VECTOR('',#48521,1000.);
#14801=VECTOR('',#48522,1000.);
#14802=VECTOR('',#48523,1000.);
#14803=VECTOR('',#48524,1000.);
#14804=VECTOR('',#48525,1000.);
#14805=VECTOR('',#48526,1000.);
#14806=VECTOR('',#48527,1000.);
#14807=VECTOR('',#48528,1000.);
#14808=VECTOR('',#48529,1000.);
#14809=VECTOR('',#48530,1000.);
#14810=VECTOR('',#48531,1000.);
#14811=VECTOR('',#48532,1000.);
#14812=VECTOR('',#48533,1000.);
#14813=VECTOR('',#48534,1000.);
#14814=VECTOR('',#48535,1000.);
#14815=VECTOR('',#48536,1000.);
#14816=VECTOR('',#48537,1000.);
#14817=VECTOR('',#48538,1000.);
#14818=VECTOR('',#48539,1000.);
#14819=VECTOR('',#48540,1000.);
#14820=VECTOR('',#48541,1000.);
#14821=VECTOR('',#48542,1000.);
#14822=VECTOR('',#48543,1000.);
#14823=VECTOR('',#48544,1000.);
#14824=VECTOR('',#48545,1000.);
#14825=VECTOR('',#48546,1000.);
#14826=VECTOR('',#48547,1000.);
#14827=VECTOR('',#48548,1000.);
#14828=VECTOR('',#48549,1000.);
#14829=VECTOR('',#48550,1000.);
#14830=VECTOR('',#48551,1000.);
#14831=VECTOR('',#48552,1000.);
#14832=VECTOR('',#48553,1000.);
#14833=VECTOR('',#48554,1000.);
#14834=VECTOR('',#48555,1000.);
#14835=VECTOR('',#48556,1000.);
#14836=VECTOR('',#48557,1000.);
#14837=VECTOR('',#48558,1000.);
#14838=VECTOR('',#48559,1000.);
#14839=VECTOR('',#48560,1000.);
#14840=VECTOR('',#48561,1000.);
#14841=VECTOR('',#48562,1000.);
#14842=VECTOR('',#48563,1000.);
#14843=VECTOR('',#48564,1000.);
#14844=VECTOR('',#48565,1000.);
#14845=VECTOR('',#48566,1000.);
#14846=VECTOR('',#48567,1000.);
#14847=VECTOR('',#48568,1000.);
#14848=VECTOR('',#48569,1000.);
#14849=VECTOR('',#48570,1000.);
#14850=VECTOR('',#48571,1000.);
#14851=VECTOR('',#48572,1000.);
#14852=VECTOR('',#48573,1000.);
#14853=VECTOR('',#48574,1000.);
#14854=VECTOR('',#48575,1000.);
#14855=VECTOR('',#48576,1000.);
#14856=VECTOR('',#48577,1000.);
#14857=VECTOR('',#48578,1000.);
#14858=VECTOR('',#48579,1000.);
#14859=VECTOR('',#48580,1000.);
#14860=VECTOR('',#48581,1000.);
#14861=VECTOR('',#48582,1000.);
#14862=VECTOR('',#48583,1000.);
#14863=VECTOR('',#48584,1000.);
#14864=VECTOR('',#48585,1000.);
#14865=VECTOR('',#48586,1000.);
#14866=VECTOR('',#48587,1000.);
#14867=VECTOR('',#48588,1000.);
#14868=VECTOR('',#48589,1000.);
#14869=VECTOR('',#48590,1000.);
#14870=VECTOR('',#48591,1000.);
#14871=VECTOR('',#48592,1000.);
#14872=VECTOR('',#48593,1000.);
#14873=VECTOR('',#48594,1000.);
#14874=VECTOR('',#48595,1000.);
#14875=VECTOR('',#48596,1000.);
#14876=VECTOR('',#48597,1000.);
#14877=VECTOR('',#48598,1000.);
#14878=VECTOR('',#48599,1000.);
#14879=VECTOR('',#48600,1000.);
#14880=VECTOR('',#48601,1000.);
#14881=VECTOR('',#48602,1000.);
#14882=VECTOR('',#48603,1000.);
#14883=VECTOR('',#48604,1000.);
#14884=VECTOR('',#48605,1000.);
#14885=VECTOR('',#48606,1000.);
#14886=VECTOR('',#48607,1000.);
#14887=VECTOR('',#48608,1000.);
#14888=VECTOR('',#48609,1000.);
#14889=VECTOR('',#48610,1000.);
#14890=VECTOR('',#48611,1000.);
#14891=VECTOR('',#48612,1000.);
#14892=VECTOR('',#48613,1000.);
#14893=VECTOR('',#48614,1000.);
#14894=VECTOR('',#48615,1000.);
#14895=VECTOR('',#48616,1000.);
#14896=VECTOR('',#48617,1000.);
#14897=VECTOR('',#48618,1000.);
#14898=VECTOR('',#48619,1000.);
#14899=VECTOR('',#48620,1000.);
#14900=VECTOR('',#48621,1000.);
#14901=VECTOR('',#48622,1000.);
#14902=VECTOR('',#48623,1000.);
#14903=VECTOR('',#48624,1000.);
#14904=VECTOR('',#48625,1000.);
#14905=VECTOR('',#48626,1000.);
#14906=VECTOR('',#48627,1000.);
#14907=VECTOR('',#48628,1000.);
#14908=VECTOR('',#48629,1000.);
#14909=VECTOR('',#48630,1000.);
#14910=VECTOR('',#48631,1000.);
#14911=VECTOR('',#48632,1000.);
#14912=VECTOR('',#48633,1000.);
#14913=VECTOR('',#48634,1000.);
#14914=VECTOR('',#48635,1000.);
#14915=VECTOR('',#48636,1000.);
#14916=VECTOR('',#48637,1000.);
#14917=VECTOR('',#48638,1000.);
#14918=VECTOR('',#48639,1000.);
#14919=VECTOR('',#48640,1000.);
#14920=VECTOR('',#48641,1000.);
#14921=VECTOR('',#48642,1000.);
#14922=VECTOR('',#48643,1000.);
#14923=VECTOR('',#48644,1000.);
#14924=VECTOR('',#48645,1000.);
#14925=VECTOR('',#48646,1000.);
#14926=VECTOR('',#48647,1000.);
#14927=VECTOR('',#48648,1000.);
#14928=VECTOR('',#48649,1000.);
#14929=VECTOR('',#48650,1000.);
#14930=VECTOR('',#48651,1000.);
#14931=VECTOR('',#48652,1000.);
#14932=VECTOR('',#48653,1000.);
#14933=VECTOR('',#48654,1000.);
#14934=VECTOR('',#48655,1000.);
#14935=VECTOR('',#48656,1000.);
#14936=VECTOR('',#48657,1000.);
#14937=VECTOR('',#48658,1000.);
#14938=VECTOR('',#48659,1000.);
#14939=VECTOR('',#48660,1000.);
#14940=VECTOR('',#48661,1000.);
#14941=VECTOR('',#48662,1000.);
#14942=VECTOR('',#48663,1000.);
#14943=VECTOR('',#48664,1000.);
#14944=VECTOR('',#48665,1000.);
#14945=VECTOR('',#48666,1000.);
#14946=VECTOR('',#48667,1000.);
#14947=VECTOR('',#48668,1000.);
#14948=VECTOR('',#48669,1000.);
#14949=VECTOR('',#48670,1000.);
#14950=VECTOR('',#48671,1000.);
#14951=VECTOR('',#48672,1000.);
#14952=VECTOR('',#48673,1000.);
#14953=VECTOR('',#48674,1000.);
#14954=VECTOR('',#48675,1000.);
#14955=VECTOR('',#48676,1000.);
#14956=VECTOR('',#48677,1000.);
#14957=VECTOR('',#48678,1000.);
#14958=VECTOR('',#48679,1000.);
#14959=VECTOR('',#48680,1000.);
#14960=VECTOR('',#48681,1000.);
#14961=VECTOR('',#48682,1000.);
#14962=VECTOR('',#48683,1000.);
#14963=VECTOR('',#48684,1000.);
#14964=VECTOR('',#48685,1000.);
#14965=VECTOR('',#48686,1000.);
#14966=VECTOR('',#48687,1000.);
#14967=VECTOR('',#48688,1000.);
#14968=VECTOR('',#48689,1000.);
#14969=VECTOR('',#48690,1000.);
#14970=VECTOR('',#48691,1000.);
#14971=VECTOR('',#48692,1000.);
#14972=VECTOR('',#48693,1000.);
#14973=VECTOR('',#48694,1000.);
#14974=VECTOR('',#48695,1000.);
#14975=VECTOR('',#48696,1000.);
#14976=VECTOR('',#48697,1000.);
#14977=VECTOR('',#48698,1000.);
#14978=VECTOR('',#48699,1000.);
#14979=VECTOR('',#48700,1000.);
#14980=VECTOR('',#48701,1000.);
#14981=VECTOR('',#48702,1000.);
#14982=VECTOR('',#48703,1000.);
#14983=VECTOR('',#48704,1000.);
#14984=VECTOR('',#48705,1000.);
#14985=VECTOR('',#48706,1000.);
#14986=VECTOR('',#48707,1000.);
#14987=VECTOR('',#48708,1000.);
#14988=VECTOR('',#48709,1000.);
#14989=VECTOR('',#48710,1000.);
#14990=VECTOR('',#48711,1000.);
#14991=VECTOR('',#48712,1000.);
#14992=VECTOR('',#48713,1000.);
#14993=VECTOR('',#48714,1000.);
#14994=VECTOR('',#48715,1000.);
#14995=VECTOR('',#48716,1000.);
#14996=VECTOR('',#48717,1000.);
#14997=VECTOR('',#48718,1000.);
#14998=VECTOR('',#48719,1000.);
#14999=VECTOR('',#48720,1000.);
#15000=VECTOR('',#48721,1000.);
#15001=VECTOR('',#48722,1000.);
#15002=VECTOR('',#48723,1000.);
#15003=VECTOR('',#48724,1000.);
#15004=VECTOR('',#48725,1000.);
#15005=VECTOR('',#48726,1000.);
#15006=VECTOR('',#48727,1000.);
#15007=VECTOR('',#48728,1000.);
#15008=VECTOR('',#48729,1000.);
#15009=VECTOR('',#48730,1000.);
#15010=VECTOR('',#48731,1000.);
#15011=VECTOR('',#48732,1000.);
#15012=VECTOR('',#48733,1000.);
#15013=VECTOR('',#48734,1000.);
#15014=VECTOR('',#48735,1000.);
#15015=VECTOR('',#48736,1000.);
#15016=VECTOR('',#48737,1000.);
#15017=VECTOR('',#48738,1000.);
#15018=VECTOR('',#48739,1000.);
#15019=VECTOR('',#48740,1000.);
#15020=VECTOR('',#48741,1000.);
#15021=VECTOR('',#48742,1000.);
#15022=VECTOR('',#48743,1000.);
#15023=VECTOR('',#48744,1000.);
#15024=VECTOR('',#48745,1000.);
#15025=VECTOR('',#48746,1000.);
#15026=VECTOR('',#48747,1000.);
#15027=VECTOR('',#48748,1000.);
#15028=VECTOR('',#48749,1000.);
#15029=VECTOR('',#48750,1000.);
#15030=VECTOR('',#48751,1000.);
#15031=VECTOR('',#48752,1000.);
#15032=VECTOR('',#48753,1000.);
#15033=VECTOR('',#48754,1000.);
#15034=VECTOR('',#48755,1000.);
#15035=VECTOR('',#48756,1000.);
#15036=VECTOR('',#48757,1000.);
#15037=VECTOR('',#48758,1000.);
#15038=VECTOR('',#48759,1000.);
#15039=VECTOR('',#48760,1000.);
#15040=VECTOR('',#48761,1000.);
#15041=VECTOR('',#48762,1000.);
#15042=VECTOR('',#48763,1000.);
#15043=VECTOR('',#48764,1000.);
#15044=VECTOR('',#48765,1000.);
#15045=VECTOR('',#48766,1000.);
#15046=VECTOR('',#48767,1000.);
#15047=VECTOR('',#48768,1000.);
#15048=VECTOR('',#48769,1000.);
#15049=VECTOR('',#48770,1000.);
#15050=VECTOR('',#48771,1000.);
#15051=VECTOR('',#48772,1000.);
#15052=VECTOR('',#48773,1000.);
#15053=VECTOR('',#48774,1000.);
#15054=VECTOR('',#48775,1000.);
#15055=VECTOR('',#48776,1000.);
#15056=VECTOR('',#48777,1000.);
#15057=VECTOR('',#48778,1000.);
#15058=VECTOR('',#48779,1000.);
#15059=VECTOR('',#48780,1000.);
#15060=VECTOR('',#48781,1000.);
#15061=VECTOR('',#48782,1000.);
#15062=VECTOR('',#48783,1000.);
#15063=VECTOR('',#48784,1000.);
#15064=VECTOR('',#48785,1000.);
#15065=VECTOR('',#48786,1000.);
#15066=VECTOR('',#48787,1000.);
#15067=VECTOR('',#48788,1000.);
#15068=VECTOR('',#48789,1000.);
#15069=VECTOR('',#48790,1000.);
#15070=VECTOR('',#48791,1000.);
#15071=VECTOR('',#48792,1000.);
#15072=VECTOR('',#48793,1000.);
#15073=VECTOR('',#48794,1000.);
#15074=VECTOR('',#48795,1000.);
#15075=VECTOR('',#48796,1000.);
#15076=VECTOR('',#48797,1000.);
#15077=VECTOR('',#48798,1000.);
#15078=VECTOR('',#48799,1000.);
#15079=VECTOR('',#48800,1000.);
#15080=VECTOR('',#48801,1000.);
#15081=VECTOR('',#48802,1000.);
#15082=VECTOR('',#48803,1000.);
#15083=VECTOR('',#48804,1000.);
#15084=VECTOR('',#48805,1000.);
#15085=VECTOR('',#48806,1000.);
#15086=VECTOR('',#48807,1000.);
#15087=VECTOR('',#48808,1000.);
#15088=VECTOR('',#48809,1000.);
#15089=VECTOR('',#48810,1000.);
#15090=VECTOR('',#48811,1000.);
#15091=VECTOR('',#48812,1000.);
#15092=VECTOR('',#48813,1000.);
#15093=VECTOR('',#48814,1000.);
#15094=VECTOR('',#48815,1000.);
#15095=VECTOR('',#48816,1000.);
#15096=VECTOR('',#48817,1000.);
#15097=VECTOR('',#48818,1000.);
#15098=VECTOR('',#48819,1000.);
#15099=VECTOR('',#48820,1000.);
#15100=VECTOR('',#48821,1000.);
#15101=VECTOR('',#48822,1000.);
#15102=VECTOR('',#48823,1000.);
#15103=VECTOR('',#48824,1000.);
#15104=VECTOR('',#48825,1000.);
#15105=VECTOR('',#48826,1000.);
#15106=VECTOR('',#48827,1000.);
#15107=VECTOR('',#48828,1000.);
#15108=VECTOR('',#48829,1000.);
#15109=VECTOR('',#48830,1000.);
#15110=VECTOR('',#48831,1000.);
#15111=VECTOR('',#48832,1000.);
#15112=VECTOR('',#48833,1000.);
#15113=VECTOR('',#48834,1000.);
#15114=VECTOR('',#48835,1000.);
#15115=VECTOR('',#48836,1000.);
#15116=VECTOR('',#48837,1000.);
#15117=VECTOR('',#48838,1000.);
#15118=VECTOR('',#48839,1000.);
#15119=VECTOR('',#48840,1000.);
#15120=VECTOR('',#48841,1000.);
#15121=VECTOR('',#48842,1000.);
#15122=VECTOR('',#48843,1000.);
#15123=VECTOR('',#48844,1000.);
#15124=VECTOR('',#48845,1000.);
#15125=VECTOR('',#48846,1000.);
#15126=VECTOR('',#48847,1000.);
#15127=VECTOR('',#48848,1000.);
#15128=VECTOR('',#48849,1000.);
#15129=VECTOR('',#48850,1000.);
#15130=VECTOR('',#48851,1000.);
#15131=VECTOR('',#48852,1000.);
#15132=VECTOR('',#48853,1000.);
#15133=VECTOR('',#48854,1000.);
#15134=VECTOR('',#48855,1000.);
#15135=VECTOR('',#48856,1000.);
#15136=VECTOR('',#48857,1000.);
#15137=VECTOR('',#48858,1000.);
#15138=VECTOR('',#48859,1000.);
#15139=VECTOR('',#48860,1000.);
#15140=VECTOR('',#48861,1000.);
#15141=VECTOR('',#48862,1000.);
#15142=VECTOR('',#48863,1000.);
#15143=VECTOR('',#48864,1000.);
#15144=VECTOR('',#48865,1000.);
#15145=VECTOR('',#48866,1000.);
#15146=VECTOR('',#48867,1000.);
#15147=VECTOR('',#48868,1000.);
#15148=VECTOR('',#48869,1000.);
#15149=VECTOR('',#48870,1000.);
#15150=VECTOR('',#48871,1000.);
#15151=VECTOR('',#48872,1000.);
#15152=VECTOR('',#48873,1000.);
#15153=VECTOR('',#48874,1000.);
#15154=VECTOR('',#48875,1000.);
#15155=VECTOR('',#48876,1000.);
#15156=VECTOR('',#48877,1000.);
#15157=VECTOR('',#48878,1000.);
#15158=VECTOR('',#48879,1000.);
#15159=VECTOR('',#48880,1000.);
#15160=VECTOR('',#48881,1000.);
#15161=VECTOR('',#48882,1000.);
#15162=VECTOR('',#48883,1000.);
#15163=VECTOR('',#48884,1000.);
#15164=VECTOR('',#48885,1000.);
#15165=VECTOR('',#48886,1000.);
#15166=VECTOR('',#48887,1000.);
#15167=VECTOR('',#48888,1000.);
#15168=VECTOR('',#48889,1000.);
#15169=VECTOR('',#48890,1000.);
#15170=VECTOR('',#48891,1000.);
#15171=VECTOR('',#48892,1000.);
#15172=VECTOR('',#48893,1000.);
#15173=VECTOR('',#48894,1000.);
#15174=VECTOR('',#48895,1000.);
#15175=VECTOR('',#48896,1000.);
#15176=VECTOR('',#48897,1000.);
#15177=VECTOR('',#48898,1000.);
#15178=VECTOR('',#48899,1000.);
#15179=VECTOR('',#48900,1000.);
#15180=VECTOR('',#48901,1000.);
#15181=VECTOR('',#48902,1000.);
#15182=VECTOR('',#48903,1000.);
#15183=VECTOR('',#48904,1000.);
#15184=VECTOR('',#48905,1000.);
#15185=VECTOR('',#48906,1000.);
#15186=VECTOR('',#48907,1000.);
#15187=VECTOR('',#48908,1000.);
#15188=VECTOR('',#48909,1000.);
#15189=VECTOR('',#48910,1000.);
#15190=VECTOR('',#48911,1000.);
#15191=VECTOR('',#48912,1000.);
#15192=VECTOR('',#48913,1000.);
#15193=VECTOR('',#48914,1000.);
#15194=VECTOR('',#48915,1000.);
#15195=VECTOR('',#48916,1000.);
#15196=VECTOR('',#48917,1000.);
#15197=VECTOR('',#48918,1000.);
#15198=VECTOR('',#48919,1000.);
#15199=VECTOR('',#48920,1000.);
#15200=VECTOR('',#48921,1000.);
#15201=VECTOR('',#48922,1000.);
#15202=VECTOR('',#48923,1000.);
#15203=VECTOR('',#48924,1000.);
#15204=VECTOR('',#48925,1000.);
#15205=VECTOR('',#48926,1000.);
#15206=VECTOR('',#48927,1000.);
#15207=VECTOR('',#48928,1000.);
#15208=VECTOR('',#48929,1000.);
#15209=VECTOR('',#48930,1000.);
#15210=VECTOR('',#48931,1000.);
#15211=VECTOR('',#48932,1000.);
#15212=VECTOR('',#48933,1000.);
#15213=VECTOR('',#48934,1000.);
#15214=VECTOR('',#48935,1000.);
#15215=VECTOR('',#48936,1000.);
#15216=VECTOR('',#48937,1000.);
#15217=VECTOR('',#48938,1000.);
#15218=VECTOR('',#48939,1000.);
#15219=VECTOR('',#48940,1000.);
#15220=VECTOR('',#48941,1000.);
#15221=VECTOR('',#48942,1000.);
#15222=VECTOR('',#48943,1000.);
#15223=VECTOR('',#48944,1000.);
#15224=VECTOR('',#48945,1000.);
#15225=VECTOR('',#48946,1000.);
#15226=VECTOR('',#48947,1000.);
#15227=VECTOR('',#48948,1000.);
#15228=VECTOR('',#48949,1000.);
#15229=VECTOR('',#48950,1000.);
#15230=VECTOR('',#48951,1000.);
#15231=VECTOR('',#48952,1000.);
#15232=VECTOR('',#48953,1000.);
#15233=VECTOR('',#48954,1000.);
#15234=VECTOR('',#48955,1000.);
#15235=VECTOR('',#48956,1000.);
#15236=VECTOR('',#48957,1000.);
#15237=VECTOR('',#48958,1000.);
#15238=VECTOR('',#48959,1000.);
#15239=VECTOR('',#48960,1000.);
#15240=VECTOR('',#48961,1000.);
#15241=VECTOR('',#48962,1000.);
#15242=VECTOR('',#48963,1000.);
#15243=VECTOR('',#48964,1000.);
#15244=VECTOR('',#48965,1000.);
#15245=VECTOR('',#48966,1000.);
#15246=VECTOR('',#48967,1000.);
#15247=VECTOR('',#48968,1000.);
#15248=VECTOR('',#48969,1000.);
#15249=VECTOR('',#48970,1000.);
#15250=VECTOR('',#48971,1000.);
#15251=VECTOR('',#48972,1000.);
#15252=VECTOR('',#48973,1000.);
#15253=VECTOR('',#48974,1000.);
#15254=VECTOR('',#48975,1000.);
#15255=VECTOR('',#48976,1000.);
#15256=VECTOR('',#48977,1000.);
#15257=VECTOR('',#48978,1000.);
#15258=VECTOR('',#48979,1000.);
#15259=VECTOR('',#48980,1000.);
#15260=VECTOR('',#48981,1000.);
#15261=VECTOR('',#48982,1000.);
#15262=VECTOR('',#48983,1000.);
#15263=VECTOR('',#48984,1000.);
#15264=VECTOR('',#48985,1000.);
#15265=VECTOR('',#48986,1000.);
#15266=VECTOR('',#48987,1000.);
#15267=VECTOR('',#48988,1000.);
#15268=VECTOR('',#48989,1000.);
#15269=VECTOR('',#48990,1000.);
#15270=VECTOR('',#48991,1000.);
#15271=VECTOR('',#48992,1000.);
#15272=VECTOR('',#48993,1000.);
#15273=VECTOR('',#48994,1000.);
#15274=VECTOR('',#48995,1000.);
#15275=VECTOR('',#48996,1000.);
#15276=VECTOR('',#48997,1000.);
#15277=VECTOR('',#48998,1000.);
#15278=VECTOR('',#48999,1000.);
#15279=VECTOR('',#49000,1000.);
#15280=VECTOR('',#49001,1000.);
#15281=VECTOR('',#49002,1000.);
#15282=VECTOR('',#49003,1000.);
#15283=VECTOR('',#49004,1000.);
#15284=VECTOR('',#49005,1000.);
#15285=VECTOR('',#49006,1000.);
#15286=VECTOR('',#49007,1000.);
#15287=VECTOR('',#49008,1000.);
#15288=VECTOR('',#49009,1000.);
#15289=VECTOR('',#49010,1000.);
#15290=VECTOR('',#49011,1000.);
#15291=VECTOR('',#49012,1000.);
#15292=VECTOR('',#49013,1000.);
#15293=VECTOR('',#49014,1000.);
#15294=VECTOR('',#49015,1000.);
#15295=VECTOR('',#49016,1000.);
#15296=VECTOR('',#49017,1000.);
#15297=VECTOR('',#49018,1000.);
#15298=VECTOR('',#49019,1000.);
#15299=VECTOR('',#49020,1000.);
#15300=VECTOR('',#49021,1000.);
#15301=VECTOR('',#49022,1000.);
#15302=VECTOR('',#49023,1000.);
#15303=VECTOR('',#49024,1000.);
#15304=VECTOR('',#49025,1000.);
#15305=VECTOR('',#49026,1000.);
#15306=VECTOR('',#49027,1000.);
#15307=VECTOR('',#49028,1000.);
#15308=VECTOR('',#49029,1000.);
#15309=VECTOR('',#49030,1000.);
#15310=VECTOR('',#49031,1000.);
#15311=VECTOR('',#49032,1000.);
#15312=VECTOR('',#49033,1000.);
#15313=VECTOR('',#49034,1000.);
#15314=VECTOR('',#49035,1000.);
#15315=VECTOR('',#49036,1000.);
#15316=VECTOR('',#49037,1000.);
#15317=VECTOR('',#49038,1000.);
#15318=VECTOR('',#49039,1000.);
#15319=VECTOR('',#49040,1000.);
#15320=VECTOR('',#49041,1000.);
#15321=VECTOR('',#49042,1000.);
#15322=VECTOR('',#49043,1000.);
#15323=VECTOR('',#49044,1000.);
#15324=VECTOR('',#49045,1000.);
#15325=VECTOR('',#49046,1000.);
#15326=VECTOR('',#49047,1000.);
#15327=VECTOR('',#49048,1000.);
#15328=VECTOR('',#49049,1000.);
#15329=VECTOR('',#49050,1000.);
#15330=VECTOR('',#49051,1000.);
#15331=VECTOR('',#49052,1000.);
#15332=VECTOR('',#49053,1000.);
#15333=VECTOR('',#49054,1000.);
#15334=VECTOR('',#49055,1000.);
#15335=VECTOR('',#49056,1000.);
#15336=VECTOR('',#49057,1000.);
#15337=VECTOR('',#49058,1000.);
#15338=VECTOR('',#49059,1000.);
#15339=VECTOR('',#49060,1000.);
#15340=VECTOR('',#49061,1000.);
#15341=VECTOR('',#49062,1000.);
#15342=VECTOR('',#49063,1000.);
#15343=VECTOR('',#49064,1000.);
#15344=VECTOR('',#49065,1000.);
#15345=VECTOR('',#49066,1000.);
#15346=VECTOR('',#49067,1000.);
#15347=VECTOR('',#49068,1000.);
#15348=VECTOR('',#49069,1000.);
#15349=VECTOR('',#49070,1000.);
#15350=VECTOR('',#49071,1000.);
#15351=VECTOR('',#49072,1000.);
#15352=VECTOR('',#49073,1000.);
#15353=VECTOR('',#49074,1000.);
#15354=VECTOR('',#49075,1000.);
#15355=VECTOR('',#49076,1000.);
#15356=VECTOR('',#49077,1000.);
#15357=VECTOR('',#49078,1000.);
#15358=VECTOR('',#49079,1000.);
#15359=VECTOR('',#49080,1000.);
#15360=VECTOR('',#49081,1000.);
#15361=VECTOR('',#49082,1000.);
#15362=VECTOR('',#49083,1000.);
#15363=VECTOR('',#49084,1000.);
#15364=VECTOR('',#49085,1000.);
#15365=VECTOR('',#49086,1000.);
#15366=VECTOR('',#49087,1000.);
#15367=VECTOR('',#49088,1000.);
#15368=VECTOR('',#49089,1000.);
#15369=VECTOR('',#49090,1000.);
#15370=VECTOR('',#49091,1000.);
#15371=VECTOR('',#49092,1000.);
#15372=VECTOR('',#49093,1000.);
#15373=VECTOR('',#49094,1000.);
#15374=VECTOR('',#49097,1000.);
#15375=VECTOR('',#49098,1000.);
#15376=VECTOR('',#49101,1000.);
#15377=VECTOR('',#49104,1000.);
#15378=VECTOR('',#49107,1000.);
#15379=VECTOR('',#49110,1000.);
#15380=VECTOR('',#49115,1000.);
#15381=VECTOR('',#49116,1000.);
#15382=VECTOR('',#49119,1000.);
#15383=VECTOR('',#49122,1000.);
#15384=VECTOR('',#49125,1000.);
#15385=VECTOR('',#49128,1000.);
#15386=VECTOR('',#49133,1000.);
#15387=VECTOR('',#49134,1000.);
#15388=VECTOR('',#49137,1000.);
#15389=VECTOR('',#49140,1000.);
#15390=VECTOR('',#49143,1000.);
#15391=VECTOR('',#49146,1000.);
#15392=VECTOR('',#49151,1000.);
#15393=VECTOR('',#49152,1000.);
#15394=VECTOR('',#49155,1000.);
#15395=VECTOR('',#49158,1000.);
#15396=VECTOR('',#49161,1000.);
#15397=VECTOR('',#49164,1000.);
#15398=VECTOR('',#49169,1000.);
#15399=VECTOR('',#49170,1000.);
#15400=VECTOR('',#49173,1000.);
#15401=VECTOR('',#49176,1000.);
#15402=VECTOR('',#49179,1000.);
#15403=VECTOR('',#49182,1000.);
#15404=VECTOR('',#49187,1000.);
#15405=VECTOR('',#49188,1000.);
#15406=VECTOR('',#49191,1000.);
#15407=VECTOR('',#49194,1000.);
#15408=VECTOR('',#49197,1000.);
#15409=VECTOR('',#49200,1000.);
#15410=VECTOR('',#49205,1000.);
#15411=VECTOR('',#49206,1000.);
#15412=VECTOR('',#49209,1000.);
#15413=VECTOR('',#49212,1000.);
#15414=VECTOR('',#49215,1000.);
#15415=VECTOR('',#49218,1000.);
#15416=VECTOR('',#49223,1000.);
#15417=VECTOR('',#49224,1000.);
#15418=VECTOR('',#49227,1000.);
#15419=VECTOR('',#49230,1000.);
#15420=VECTOR('',#49233,1000.);
#15421=VECTOR('',#49236,1000.);
#15422=VECTOR('',#49241,1000.);
#15423=VECTOR('',#49242,1000.);
#15424=VECTOR('',#49245,1000.);
#15425=VECTOR('',#49248,1000.);
#15426=VECTOR('',#49251,1000.);
#15427=VECTOR('',#49254,1000.);
#15428=VECTOR('',#49259,1000.);
#15429=VECTOR('',#49260,1000.);
#15430=VECTOR('',#49263,1000.);
#15431=VECTOR('',#49266,1000.);
#15432=VECTOR('',#49269,1000.);
#15433=VECTOR('',#49272,1000.);
#15434=VECTOR('',#49277,1000.);
#15435=VECTOR('',#49278,1000.);
#15436=VECTOR('',#49281,1000.);
#15437=VECTOR('',#49284,1000.);
#15438=VECTOR('',#49287,1000.);
#15439=VECTOR('',#49290,1000.);
#15440=VECTOR('',#49295,1000.);
#15441=VECTOR('',#49296,1000.);
#15442=VECTOR('',#49299,1000.);
#15443=VECTOR('',#49302,1000.);
#15444=VECTOR('',#49305,1000.);
#15445=VECTOR('',#49308,1000.);
#15446=VECTOR('',#49313,1000.);
#15447=VECTOR('',#49314,1000.);
#15448=VECTOR('',#49317,1000.);
#15449=VECTOR('',#49320,1000.);
#15450=VECTOR('',#49323,1000.);
#15451=VECTOR('',#49326,1000.);
#15452=VECTOR('',#49331,1000.);
#15453=VECTOR('',#49332,1000.);
#15454=VECTOR('',#49335,1000.);
#15455=VECTOR('',#49338,1000.);
#15456=VECTOR('',#49341,1000.);
#15457=VECTOR('',#49344,1000.);
#15458=VECTOR('',#49349,1000.);
#15459=VECTOR('',#49350,1000.);
#15460=VECTOR('',#49353,1000.);
#15461=VECTOR('',#49356,1000.);
#15462=VECTOR('',#49359,1000.);
#15463=VECTOR('',#49362,1000.);
#15464=VECTOR('',#49367,1000.);
#15465=VECTOR('',#49368,1000.);
#15466=VECTOR('',#49371,1000.);
#15467=VECTOR('',#49374,1000.);
#15468=VECTOR('',#49377,1000.);
#15469=VECTOR('',#49380,1000.);
#15470=VECTOR('',#49385,1000.);
#15471=VECTOR('',#49386,1000.);
#15472=VECTOR('',#49389,1000.);
#15473=VECTOR('',#49392,1000.);
#15474=VECTOR('',#49395,1000.);
#15475=VECTOR('',#49398,1000.);
#15476=VECTOR('',#49403,1000.);
#15477=VECTOR('',#49404,1000.);
#15478=VECTOR('',#49407,1000.);
#15479=VECTOR('',#49410,1000.);
#15480=VECTOR('',#49413,1000.);
#15481=VECTOR('',#49416,1000.);
#15482=VECTOR('',#49421,1000.);
#15483=VECTOR('',#49422,1000.);
#15484=VECTOR('',#49425,1000.);
#15485=VECTOR('',#49428,1000.);
#15486=VECTOR('',#49431,1000.);
#15487=VECTOR('',#49434,1000.);
#15488=VECTOR('',#49439,1000.);
#15489=VECTOR('',#49440,1000.);
#15490=VECTOR('',#49443,1000.);
#15491=VECTOR('',#49446,1000.);
#15492=VECTOR('',#49449,1000.);
#15493=VECTOR('',#49452,1000.);
#15494=VECTOR('',#49457,1000.);
#15495=VECTOR('',#49458,1000.);
#15496=VECTOR('',#49461,1000.);
#15497=VECTOR('',#49464,1000.);
#15498=VECTOR('',#49467,1000.);
#15499=VECTOR('',#49470,1000.);
#15500=VECTOR('',#49475,1000.);
#15501=VECTOR('',#49476,1000.);
#15502=VECTOR('',#49479,1000.);
#15503=VECTOR('',#49482,1000.);
#15504=VECTOR('',#49485,1000.);
#15505=VECTOR('',#49488,1000.);
#15506=VECTOR('',#49493,1000.);
#15507=VECTOR('',#49494,1000.);
#15508=VECTOR('',#49497,1000.);
#15509=VECTOR('',#49500,1000.);
#15510=VECTOR('',#49503,1000.);
#15511=VECTOR('',#49506,1000.);
#15512=VECTOR('',#49511,1000.);
#15513=VECTOR('',#49512,1000.);
#15514=VECTOR('',#49515,1000.);
#15515=VECTOR('',#49518,1000.);
#15516=VECTOR('',#49521,1000.);
#15517=VECTOR('',#49524,1000.);
#15518=VECTOR('',#49529,1000.);
#15519=VECTOR('',#49530,1000.);
#15520=VECTOR('',#49533,1000.);
#15521=VECTOR('',#49536,1000.);
#15522=VECTOR('',#49539,1000.);
#15523=VECTOR('',#49542,1000.);
#15524=VECTOR('',#49547,1000.);
#15525=VECTOR('',#49548,1000.);
#15526=VECTOR('',#49551,1000.);
#15527=VECTOR('',#49554,1000.);
#15528=VECTOR('',#49557,1000.);
#15529=VECTOR('',#49560,1000.);
#15530=VECTOR('',#49565,1000.);
#15531=VECTOR('',#49566,1000.);
#15532=VECTOR('',#49569,1000.);
#15533=VECTOR('',#49572,1000.);
#15534=VECTOR('',#49575,1000.);
#15535=VECTOR('',#49578,1000.);
#15536=VECTOR('',#49583,1000.);
#15537=VECTOR('',#49584,1000.);
#15538=VECTOR('',#49587,1000.);
#15539=VECTOR('',#49590,1000.);
#15540=VECTOR('',#49593,1000.);
#15541=VECTOR('',#49596,1000.);
#15542=VECTOR('',#49601,1000.);
#15543=VECTOR('',#49602,1000.);
#15544=VECTOR('',#49605,1000.);
#15545=VECTOR('',#49608,1000.);
#15546=VECTOR('',#49611,1000.);
#15547=VECTOR('',#49614,1000.);
#15548=VECTOR('',#49619,1000.);
#15549=VECTOR('',#49620,1000.);
#15550=VECTOR('',#49623,1000.);
#15551=VECTOR('',#49626,1000.);
#15552=VECTOR('',#49629,1000.);
#15553=VECTOR('',#49632,1000.);
#15554=VECTOR('',#49637,1000.);
#15555=VECTOR('',#49638,1000.);
#15556=VECTOR('',#49641,1000.);
#15557=VECTOR('',#49644,1000.);
#15558=VECTOR('',#49647,1000.);
#15559=VECTOR('',#49650,1000.);
#15560=VECTOR('',#49655,1000.);
#15561=VECTOR('',#49656,1000.);
#15562=VECTOR('',#49659,1000.);
#15563=VECTOR('',#49662,1000.);
#15564=VECTOR('',#49665,1000.);
#15565=VECTOR('',#49668,1000.);
#15566=VECTOR('',#49673,1000.);
#15567=VECTOR('',#49674,1000.);
#15568=VECTOR('',#49677,1000.);
#15569=VECTOR('',#49680,1000.);
#15570=VECTOR('',#49683,1000.);
#15571=VECTOR('',#49686,1000.);
#15572=VECTOR('',#49691,1000.);
#15573=VECTOR('',#49692,1000.);
#15574=VECTOR('',#49695,1000.);
#15575=VECTOR('',#49698,1000.);
#15576=VECTOR('',#49701,1000.);
#15577=VECTOR('',#49704,1000.);
#15578=VECTOR('',#49709,1000.);
#15579=VECTOR('',#49710,1000.);
#15580=VECTOR('',#49713,1000.);
#15581=VECTOR('',#49716,1000.);
#15582=VECTOR('',#49719,1000.);
#15583=VECTOR('',#49722,1000.);
#15584=VECTOR('',#49727,1000.);
#15585=VECTOR('',#49728,1000.);
#15586=VECTOR('',#49731,1000.);
#15587=VECTOR('',#49734,1000.);
#15588=VECTOR('',#49737,1000.);
#15589=VECTOR('',#49740,1000.);
#15590=VECTOR('',#49745,1000.);
#15591=VECTOR('',#49746,1000.);
#15592=VECTOR('',#49749,1000.);
#15593=VECTOR('',#49752,1000.);
#15594=VECTOR('',#49755,1000.);
#15595=VECTOR('',#49758,1000.);
#15596=VECTOR('',#49763,1000.);
#15597=VECTOR('',#49764,1000.);
#15598=VECTOR('',#49767,1000.);
#15599=VECTOR('',#49770,1000.);
#15600=VECTOR('',#49773,1000.);
#15601=VECTOR('',#49776,1000.);
#15602=VECTOR('',#49781,1000.);
#15603=VECTOR('',#49782,1000.);
#15604=VECTOR('',#49785,1000.);
#15605=VECTOR('',#49788,1000.);
#15606=VECTOR('',#49791,1000.);
#15607=VECTOR('',#49794,1000.);
#15608=VECTOR('',#49799,1000.);
#15609=VECTOR('',#49800,1000.);
#15610=VECTOR('',#49803,1000.);
#15611=VECTOR('',#49806,1000.);
#15612=VECTOR('',#49809,1000.);
#15613=VECTOR('',#49812,1000.);
#15614=VECTOR('',#49817,1000.);
#15615=VECTOR('',#49818,1000.);
#15616=VECTOR('',#49821,1000.);
#15617=VECTOR('',#49824,1000.);
#15618=VECTOR('',#49827,1000.);
#15619=VECTOR('',#49830,1000.);
#15620=VECTOR('',#49835,1000.);
#15621=VECTOR('',#49836,1000.);
#15622=VECTOR('',#49839,1000.);
#15623=VECTOR('',#49842,1000.);
#15624=VECTOR('',#49845,1000.);
#15625=VECTOR('',#49848,1000.);
#15626=VECTOR('',#49853,1000.);
#15627=VECTOR('',#49854,1000.);
#15628=VECTOR('',#49857,1000.);
#15629=VECTOR('',#49860,1000.);
#15630=VECTOR('',#49863,1000.);
#15631=VECTOR('',#49866,1000.);
#15632=VECTOR('',#49871,1000.);
#15633=VECTOR('',#49872,1000.);
#15634=VECTOR('',#49875,1000.);
#15635=VECTOR('',#49878,1000.);
#15636=VECTOR('',#49881,1000.);
#15637=VECTOR('',#49884,1000.);
#15638=VECTOR('',#49889,1000.);
#15639=VECTOR('',#49890,1000.);
#15640=VECTOR('',#49893,1000.);
#15641=VECTOR('',#49896,1000.);
#15642=VECTOR('',#49899,1000.);
#15643=VECTOR('',#49902,1000.);
#15644=VECTOR('',#49907,1000.);
#15645=VECTOR('',#49908,1000.);
#15646=VECTOR('',#49911,1000.);
#15647=VECTOR('',#49914,1000.);
#15648=VECTOR('',#49917,1000.);
#15649=VECTOR('',#49920,1000.);
#15650=VECTOR('',#49925,1000.);
#15651=VECTOR('',#49926,1000.);
#15652=VECTOR('',#49929,1000.);
#15653=VECTOR('',#49932,1000.);
#15654=VECTOR('',#49935,1000.);
#15655=VECTOR('',#49938,1000.);
#15656=VECTOR('',#49943,1000.);
#15657=VECTOR('',#49944,1000.);
#15658=VECTOR('',#49947,1000.);
#15659=VECTOR('',#49950,1000.);
#15660=VECTOR('',#49953,1000.);
#15661=VECTOR('',#49956,1000.);
#15662=VECTOR('',#49961,1000.);
#15663=VECTOR('',#49962,1000.);
#15664=VECTOR('',#49965,1000.);
#15665=VECTOR('',#49968,1000.);
#15666=VECTOR('',#49971,1000.);
#15667=VECTOR('',#49974,1000.);
#15668=VECTOR('',#49979,1000.);
#15669=VECTOR('',#49980,1000.);
#15670=VECTOR('',#49983,1000.);
#15671=VECTOR('',#49986,1000.);
#15672=VECTOR('',#49989,1000.);
#15673=VECTOR('',#49992,1000.);
#15674=VECTOR('',#49997,1000.);
#15675=VECTOR('',#49998,1000.);
#15676=VECTOR('',#50001,1000.);
#15677=VECTOR('',#50004,1000.);
#15678=VECTOR('',#50007,1000.);
#15679=VECTOR('',#50010,1000.);
#15680=VECTOR('',#50015,1000.);
#15681=VECTOR('',#50016,1000.);
#15682=VECTOR('',#50019,1000.);
#15683=VECTOR('',#50022,1000.);
#15684=VECTOR('',#50025,1000.);
#15685=VECTOR('',#50028,1000.);
#15686=VECTOR('',#50033,1000.);
#15687=VECTOR('',#50034,1000.);
#15688=VECTOR('',#50037,1000.);
#15689=VECTOR('',#50040,1000.);
#15690=VECTOR('',#50043,1000.);
#15691=VECTOR('',#50046,1000.);
#15692=VECTOR('',#50051,1000.);
#15693=VECTOR('',#50052,1000.);
#15694=VECTOR('',#50055,1000.);
#15695=VECTOR('',#50058,1000.);
#15696=VECTOR('',#50061,1000.);
#15697=VECTOR('',#50064,1000.);
#15698=VECTOR('',#50069,1000.);
#15699=VECTOR('',#50070,1000.);
#15700=VECTOR('',#50073,1000.);
#15701=VECTOR('',#50076,1000.);
#15702=VECTOR('',#50079,1000.);
#15703=VECTOR('',#50082,1000.);
#15704=VECTOR('',#50087,1000.);
#15705=VECTOR('',#50088,1000.);
#15706=VECTOR('',#50091,1000.);
#15707=VECTOR('',#50094,1000.);
#15708=VECTOR('',#50097,1000.);
#15709=VECTOR('',#50100,1000.);
#15710=VECTOR('',#50105,1000.);
#15711=VECTOR('',#50106,1000.);
#15712=VECTOR('',#50109,1000.);
#15713=VECTOR('',#50112,1000.);
#15714=VECTOR('',#50115,1000.);
#15715=VECTOR('',#50118,1000.);
#15716=VECTOR('',#50123,1000.);
#15717=VECTOR('',#50124,1000.);
#15718=VECTOR('',#50127,1000.);
#15719=VECTOR('',#50130,1000.);
#15720=VECTOR('',#50133,1000.);
#15721=VECTOR('',#50136,1000.);
#15722=VECTOR('',#50141,1000.);
#15723=VECTOR('',#50142,1000.);
#15724=VECTOR('',#50145,1000.);
#15725=VECTOR('',#50148,1000.);
#15726=VECTOR('',#50151,1000.);
#15727=VECTOR('',#50154,1000.);
#15728=VECTOR('',#50159,1000.);
#15729=VECTOR('',#50160,1000.);
#15730=VECTOR('',#50163,1000.);
#15731=VECTOR('',#50166,1000.);
#15732=VECTOR('',#50169,1000.);
#15733=VECTOR('',#50172,1000.);
#15734=VECTOR('',#50177,1000.);
#15735=VECTOR('',#50178,1000.);
#15736=VECTOR('',#50181,1000.);
#15737=VECTOR('',#50184,1000.);
#15738=VECTOR('',#50187,1000.);
#15739=VECTOR('',#50190,1000.);
#15740=VECTOR('',#50195,1000.);
#15741=VECTOR('',#50196,1000.);
#15742=VECTOR('',#50199,1000.);
#15743=VECTOR('',#50202,1000.);
#15744=VECTOR('',#50205,1000.);
#15745=VECTOR('',#50208,1000.);
#15746=VECTOR('',#50213,1000.);
#15747=VECTOR('',#50214,1000.);
#15748=VECTOR('',#50217,1000.);
#15749=VECTOR('',#50220,1000.);
#15750=VECTOR('',#50223,1000.);
#15751=VECTOR('',#50226,1000.);
#15752=VECTOR('',#50231,1000.);
#15753=VECTOR('',#50232,1000.);
#15754=VECTOR('',#50235,1000.);
#15755=VECTOR('',#50238,1000.);
#15756=VECTOR('',#50241,1000.);
#15757=VECTOR('',#50244,1000.);
#15758=VECTOR('',#50249,1000.);
#15759=VECTOR('',#50250,1000.);
#15760=VECTOR('',#50253,1000.);
#15761=VECTOR('',#50256,1000.);
#15762=VECTOR('',#50259,1000.);
#15763=VECTOR('',#50262,1000.);
#15764=VECTOR('',#50267,1000.);
#15765=VECTOR('',#50268,1000.);
#15766=VECTOR('',#50271,1000.);
#15767=VECTOR('',#50274,1000.);
#15768=VECTOR('',#50277,1000.);
#15769=VECTOR('',#50280,1000.);
#15770=VECTOR('',#50285,1000.);
#15771=VECTOR('',#50286,1000.);
#15772=VECTOR('',#50289,1000.);
#15773=VECTOR('',#50292,1000.);
#15774=VECTOR('',#50295,1000.);
#15775=VECTOR('',#50298,1000.);
#15776=VECTOR('',#50303,1000.);
#15777=VECTOR('',#50304,1000.);
#15778=VECTOR('',#50307,1000.);
#15779=VECTOR('',#50310,1000.);
#15780=VECTOR('',#50313,1000.);
#15781=VECTOR('',#50316,1000.);
#15782=VECTOR('',#50321,1000.);
#15783=VECTOR('',#50322,1000.);
#15784=VECTOR('',#50325,1000.);
#15785=VECTOR('',#50328,1000.);
#15786=VECTOR('',#50331,1000.);
#15787=VECTOR('',#50334,1000.);
#15788=VECTOR('',#50339,1000.);
#15789=VECTOR('',#50340,1000.);
#15790=VECTOR('',#50343,1000.);
#15791=VECTOR('',#50346,1000.);
#15792=VECTOR('',#50349,1000.);
#15793=VECTOR('',#50352,1000.);
#15794=VECTOR('',#50357,1000.);
#15795=VECTOR('',#50358,1000.);
#15796=VECTOR('',#50361,1000.);
#15797=VECTOR('',#50364,1000.);
#15798=VECTOR('',#50367,1000.);
#15799=VECTOR('',#50370,1000.);
#15800=VECTOR('',#50375,1000.);
#15801=VECTOR('',#50376,1000.);
#15802=VECTOR('',#50379,1000.);
#15803=VECTOR('',#50382,1000.);
#15804=VECTOR('',#50385,1000.);
#15805=VECTOR('',#50388,1000.);
#15806=VECTOR('',#50393,1000.);
#15807=VECTOR('',#50394,1000.);
#15808=VECTOR('',#50397,1000.);
#15809=VECTOR('',#50400,1000.);
#15810=VECTOR('',#50403,1000.);
#15811=VECTOR('',#50406,1000.);
#15812=VECTOR('',#50411,1000.);
#15813=VECTOR('',#50412,1000.);
#15814=VECTOR('',#50415,1000.);
#15815=VECTOR('',#50418,1000.);
#15816=VECTOR('',#50421,1000.);
#15817=VECTOR('',#50424,1000.);
#15818=VECTOR('',#50429,1000.);
#15819=VECTOR('',#50430,1000.);
#15820=VECTOR('',#50433,1000.);
#15821=VECTOR('',#50436,1000.);
#15822=VECTOR('',#50439,1000.);
#15823=VECTOR('',#50442,1000.);
#15824=VECTOR('',#50447,1000.);
#15825=VECTOR('',#50448,1000.);
#15826=VECTOR('',#50451,1000.);
#15827=VECTOR('',#50454,1000.);
#15828=VECTOR('',#50457,1000.);
#15829=VECTOR('',#50460,1000.);
#15830=VECTOR('',#50465,1000.);
#15831=VECTOR('',#50466,1000.);
#15832=VECTOR('',#50469,1000.);
#15833=VECTOR('',#50472,1000.);
#15834=VECTOR('',#50475,1000.);
#15835=VECTOR('',#50478,1000.);
#15836=VECTOR('',#50483,1000.);
#15837=VECTOR('',#50484,1000.);
#15838=VECTOR('',#50487,1000.);
#15839=VECTOR('',#50490,1000.);
#15840=VECTOR('',#50493,1000.);
#15841=VECTOR('',#50496,1000.);
#15842=VECTOR('',#50501,1000.);
#15843=VECTOR('',#50502,1000.);
#15844=VECTOR('',#50505,1000.);
#15845=VECTOR('',#50508,1000.);
#15846=VECTOR('',#50511,1000.);
#15847=VECTOR('',#50514,1000.);
#15848=VECTOR('',#50519,1000.);
#15849=VECTOR('',#50520,1000.);
#15850=VECTOR('',#50523,1000.);
#15851=VECTOR('',#50526,1000.);
#15852=VECTOR('',#50529,1000.);
#15853=VECTOR('',#50532,1000.);
#15854=VECTOR('',#50537,1000.);
#15855=VECTOR('',#50538,1000.);
#15856=VECTOR('',#50541,1000.);
#15857=VECTOR('',#50544,1000.);
#15858=VECTOR('',#50547,1000.);
#15859=VECTOR('',#50550,1000.);
#15860=VECTOR('',#50555,1000.);
#15861=VECTOR('',#50556,1000.);
#15862=VECTOR('',#50559,1000.);
#15863=VECTOR('',#50562,1000.);
#15864=VECTOR('',#50565,1000.);
#15865=VECTOR('',#50568,1000.);
#15866=VECTOR('',#50573,1000.);
#15867=VECTOR('',#50574,1000.);
#15868=VECTOR('',#50577,1000.);
#15869=VECTOR('',#50580,1000.);
#15870=VECTOR('',#50583,1000.);
#15871=VECTOR('',#50586,1000.);
#15872=VECTOR('',#50591,1000.);
#15873=VECTOR('',#50592,1000.);
#15874=VECTOR('',#50595,1000.);
#15875=VECTOR('',#50598,1000.);
#15876=VECTOR('',#50601,1000.);
#15877=VECTOR('',#50604,1000.);
#15878=VECTOR('',#50609,1000.);
#15879=VECTOR('',#50610,1000.);
#15880=VECTOR('',#50613,1000.);
#15881=VECTOR('',#50616,1000.);
#15882=VECTOR('',#50619,1000.);
#15883=VECTOR('',#50622,1000.);
#15884=VECTOR('',#50627,1000.);
#15885=VECTOR('',#50628,1000.);
#15886=VECTOR('',#50631,1000.);
#15887=VECTOR('',#50634,1000.);
#15888=VECTOR('',#50637,1000.);
#15889=VECTOR('',#50640,1000.);
#15890=VECTOR('',#50645,1000.);
#15891=VECTOR('',#50646,1000.);
#15892=VECTOR('',#50649,1000.);
#15893=VECTOR('',#50652,1000.);
#15894=VECTOR('',#50655,1000.);
#15895=VECTOR('',#50658,1000.);
#15896=VECTOR('',#50663,1000.);
#15897=VECTOR('',#50664,1000.);
#15898=VECTOR('',#50667,1000.);
#15899=VECTOR('',#50670,1000.);
#15900=VECTOR('',#50673,1000.);
#15901=VECTOR('',#50676,1000.);
#15902=VECTOR('',#50681,1000.);
#15903=VECTOR('',#50682,1000.);
#15904=VECTOR('',#50685,1000.);
#15905=VECTOR('',#50688,1000.);
#15906=VECTOR('',#50691,1000.);
#15907=VECTOR('',#50694,1000.);
#15908=VECTOR('',#50699,1000.);
#15909=VECTOR('',#50700,1000.);
#15910=VECTOR('',#50703,1000.);
#15911=VECTOR('',#50706,1000.);
#15912=VECTOR('',#50709,1000.);
#15913=VECTOR('',#50712,1000.);
#15914=VECTOR('',#50717,1000.);
#15915=VECTOR('',#50718,1000.);
#15916=VECTOR('',#50721,1000.);
#15917=VECTOR('',#50724,1000.);
#15918=VECTOR('',#50727,1000.);
#15919=VECTOR('',#50730,1000.);
#15920=VECTOR('',#50735,1000.);
#15921=VECTOR('',#50736,1000.);
#15922=VECTOR('',#50739,1000.);
#15923=VECTOR('',#50742,1000.);
#15924=VECTOR('',#50745,1000.);
#15925=VECTOR('',#50748,1000.);
#15926=VECTOR('',#50753,1000.);
#15927=VECTOR('',#50754,1000.);
#15928=VECTOR('',#50757,1000.);
#15929=VECTOR('',#50760,1000.);
#15930=VECTOR('',#50763,1000.);
#15931=VECTOR('',#50766,1000.);
#15932=VECTOR('',#50771,1000.);
#15933=VECTOR('',#50772,1000.);
#15934=VECTOR('',#50775,1000.);
#15935=VECTOR('',#50778,1000.);
#15936=VECTOR('',#50781,1000.);
#15937=VECTOR('',#50784,1000.);
#15938=VECTOR('',#50789,1000.);
#15939=VECTOR('',#50790,1000.);
#15940=VECTOR('',#50793,1000.);
#15941=VECTOR('',#50796,1000.);
#15942=VECTOR('',#50799,1000.);
#15943=VECTOR('',#50802,1000.);
#15944=VECTOR('',#50807,1000.);
#15945=VECTOR('',#50808,1000.);
#15946=VECTOR('',#50811,1000.);
#15947=VECTOR('',#50814,1000.);
#15948=VECTOR('',#50817,1000.);
#15949=VECTOR('',#50820,1000.);
#15950=VECTOR('',#50825,1000.);
#15951=VECTOR('',#50826,1000.);
#15952=VECTOR('',#50829,1000.);
#15953=VECTOR('',#50832,1000.);
#15954=VECTOR('',#50835,1000.);
#15955=VECTOR('',#50838,1000.);
#15956=VECTOR('',#50843,1000.);
#15957=VECTOR('',#50844,1000.);
#15958=VECTOR('',#50847,1000.);
#15959=VECTOR('',#50850,1000.);
#15960=VECTOR('',#50853,1000.);
#15961=VECTOR('',#50856,1000.);
#15962=VECTOR('',#50861,1000.);
#15963=VECTOR('',#50862,1000.);
#15964=VECTOR('',#50865,1000.);
#15965=VECTOR('',#50868,1000.);
#15966=VECTOR('',#50871,1000.);
#15967=VECTOR('',#50874,1000.);
#15968=VECTOR('',#50879,1000.);
#15969=VECTOR('',#50880,1000.);
#15970=VECTOR('',#50883,1000.);
#15971=VECTOR('',#50886,1000.);
#15972=VECTOR('',#50889,1000.);
#15973=VECTOR('',#50892,1000.);
#15974=VECTOR('',#50897,1000.);
#15975=VECTOR('',#50898,1000.);
#15976=VECTOR('',#50901,1000.);
#15977=VECTOR('',#50904,1000.);
#15978=VECTOR('',#50907,1000.);
#15979=VECTOR('',#50910,1000.);
#15980=VECTOR('',#50915,1000.);
#15981=VECTOR('',#50916,1000.);
#15982=VECTOR('',#50919,1000.);
#15983=VECTOR('',#50922,1000.);
#15984=VECTOR('',#50925,1000.);
#15985=VECTOR('',#50928,1000.);
#15986=VECTOR('',#50933,1000.);
#15987=VECTOR('',#50934,1000.);
#15988=VECTOR('',#50937,1000.);
#15989=VECTOR('',#50940,1000.);
#15990=VECTOR('',#50943,1000.);
#15991=VECTOR('',#50946,1000.);
#15992=VECTOR('',#50951,1000.);
#15993=VECTOR('',#50952,1000.);
#15994=VECTOR('',#50955,1000.);
#15995=VECTOR('',#50958,1000.);
#15996=VECTOR('',#50961,1000.);
#15997=VECTOR('',#50964,1000.);
#15998=VECTOR('',#50969,1000.);
#15999=VECTOR('',#50970,1000.);
#16000=VECTOR('',#50973,1000.);
#16001=VECTOR('',#50976,1000.);
#16002=VECTOR('',#50979,1000.);
#16003=VECTOR('',#50982,1000.);
#16004=VECTOR('',#50987,1000.);
#16005=VECTOR('',#50988,1000.);
#16006=VECTOR('',#50991,1000.);
#16007=VECTOR('',#50994,1000.);
#16008=VECTOR('',#50997,1000.);
#16009=VECTOR('',#51000,1000.);
#16010=VECTOR('',#51005,1000.);
#16011=VECTOR('',#51006,1000.);
#16012=VECTOR('',#51009,1000.);
#16013=VECTOR('',#51012,1000.);
#16014=VECTOR('',#51015,1000.);
#16015=VECTOR('',#51018,1000.);
#16016=VECTOR('',#51023,1000.);
#16017=VECTOR('',#51024,1000.);
#16018=VECTOR('',#51027,1000.);
#16019=VECTOR('',#51030,1000.);
#16020=VECTOR('',#51033,1000.);
#16021=VECTOR('',#51036,1000.);
#16022=VECTOR('',#51041,1000.);
#16023=VECTOR('',#51042,1000.);
#16024=VECTOR('',#51045,1000.);
#16025=VECTOR('',#51048,1000.);
#16026=VECTOR('',#51051,1000.);
#16027=VECTOR('',#51054,1000.);
#16028=VECTOR('',#51059,1000.);
#16029=VECTOR('',#51060,1000.);
#16030=VECTOR('',#51063,1000.);
#16031=VECTOR('',#51066,1000.);
#16032=VECTOR('',#51069,1000.);
#16033=VECTOR('',#51072,1000.);
#16034=VECTOR('',#51077,1000.);
#16035=VECTOR('',#51078,1000.);
#16036=VECTOR('',#51081,1000.);
#16037=VECTOR('',#51084,1000.);
#16038=VECTOR('',#51087,1000.);
#16039=VECTOR('',#51090,1000.);
#16040=VECTOR('',#51095,1000.);
#16041=VECTOR('',#51096,1000.);
#16042=VECTOR('',#51099,1000.);
#16043=VECTOR('',#51102,1000.);
#16044=VECTOR('',#51105,1000.);
#16045=VECTOR('',#51108,1000.);
#16046=VECTOR('',#51113,1000.);
#16047=VECTOR('',#51114,1000.);
#16048=VECTOR('',#51117,1000.);
#16049=VECTOR('',#51120,1000.);
#16050=VECTOR('',#51123,1000.);
#16051=VECTOR('',#51126,1000.);
#16052=VECTOR('',#51131,1000.);
#16053=VECTOR('',#51132,1000.);
#16054=VECTOR('',#51135,1000.);
#16055=VECTOR('',#51138,1000.);
#16056=VECTOR('',#51141,1000.);
#16057=VECTOR('',#51144,1000.);
#16058=VECTOR('',#51149,1000.);
#16059=VECTOR('',#51150,1000.);
#16060=VECTOR('',#51153,1000.);
#16061=VECTOR('',#51156,1000.);
#16062=VECTOR('',#51159,1000.);
#16063=VECTOR('',#51162,1000.);
#16064=VECTOR('',#51167,1000.);
#16065=VECTOR('',#51168,1000.);
#16066=VECTOR('',#51171,1000.);
#16067=VECTOR('',#51174,1000.);
#16068=VECTOR('',#51177,1000.);
#16069=VECTOR('',#51180,1000.);
#16070=VECTOR('',#51185,1000.);
#16071=VECTOR('',#51186,1000.);
#16072=VECTOR('',#51189,1000.);
#16073=VECTOR('',#51192,1000.);
#16074=VECTOR('',#51195,1000.);
#16075=VECTOR('',#51198,1000.);
#16076=VECTOR('',#51203,1000.);
#16077=VECTOR('',#51204,1000.);
#16078=VECTOR('',#51207,1000.);
#16079=VECTOR('',#51210,1000.);
#16080=VECTOR('',#51213,1000.);
#16081=VECTOR('',#51216,1000.);
#16082=VECTOR('',#51221,1000.);
#16083=VECTOR('',#51222,1000.);
#16084=VECTOR('',#51225,1000.);
#16085=VECTOR('',#51228,1000.);
#16086=VECTOR('',#51231,1000.);
#16087=VECTOR('',#51234,1000.);
#16088=VECTOR('',#51239,1000.);
#16089=VECTOR('',#51240,1000.);
#16090=VECTOR('',#51243,1000.);
#16091=VECTOR('',#51246,1000.);
#16092=VECTOR('',#51249,1000.);
#16093=VECTOR('',#51252,1000.);
#16094=VECTOR('',#51257,1000.);
#16095=VECTOR('',#51258,1000.);
#16096=VECTOR('',#51261,1000.);
#16097=VECTOR('',#51264,1000.);
#16098=VECTOR('',#51267,1000.);
#16099=VECTOR('',#51270,1000.);
#16100=VECTOR('',#51275,1000.);
#16101=VECTOR('',#51276,1000.);
#16102=VECTOR('',#51279,1000.);
#16103=VECTOR('',#51282,1000.);
#16104=VECTOR('',#51285,1000.);
#16105=VECTOR('',#51288,1000.);
#16106=VECTOR('',#51293,1000.);
#16107=VECTOR('',#51294,1000.);
#16108=VECTOR('',#51297,1000.);
#16109=VECTOR('',#51300,1000.);
#16110=VECTOR('',#51303,1000.);
#16111=VECTOR('',#51306,1000.);
#16112=VECTOR('',#51311,1000.);
#16113=VECTOR('',#51312,1000.);
#16114=VECTOR('',#51315,1000.);
#16115=VECTOR('',#51318,1000.);
#16116=VECTOR('',#51321,1000.);
#16117=VECTOR('',#51324,1000.);
#16118=VECTOR('',#51329,1000.);
#16119=VECTOR('',#51330,1000.);
#16120=VECTOR('',#51333,1000.);
#16121=VECTOR('',#51336,1000.);
#16122=VECTOR('',#51339,1000.);
#16123=VECTOR('',#51342,1000.);
#16124=VECTOR('',#51347,1000.);
#16125=VECTOR('',#51348,1000.);
#16126=VECTOR('',#51351,1000.);
#16127=VECTOR('',#51354,1000.);
#16128=VECTOR('',#51357,1000.);
#16129=VECTOR('',#51360,1000.);
#16130=VECTOR('',#51365,1000.);
#16131=VECTOR('',#51366,1000.);
#16132=VECTOR('',#51369,1000.);
#16133=VECTOR('',#51372,1000.);
#16134=VECTOR('',#51375,1000.);
#16135=VECTOR('',#51378,1000.);
#16136=VECTOR('',#51383,1000.);
#16137=VECTOR('',#51384,1000.);
#16138=VECTOR('',#51387,1000.);
#16139=VECTOR('',#51390,1000.);
#16140=VECTOR('',#51393,1000.);
#16141=VECTOR('',#51396,1000.);
#16142=VECTOR('',#51401,1000.);
#16143=VECTOR('',#51402,1000.);
#16144=VECTOR('',#51405,1000.);
#16145=VECTOR('',#51408,1000.);
#16146=VECTOR('',#51411,1000.);
#16147=VECTOR('',#51414,1000.);
#16148=VECTOR('',#51419,1000.);
#16149=VECTOR('',#51420,1000.);
#16150=VECTOR('',#51423,1000.);
#16151=VECTOR('',#51426,1000.);
#16152=VECTOR('',#51429,1000.);
#16153=VECTOR('',#51432,1000.);
#16154=VECTOR('',#51437,1000.);
#16155=VECTOR('',#51438,1000.);
#16156=VECTOR('',#51441,1000.);
#16157=VECTOR('',#51444,1000.);
#16158=VECTOR('',#51447,1000.);
#16159=VECTOR('',#51450,1000.);
#16160=VECTOR('',#51455,1000.);
#16161=VECTOR('',#51456,1000.);
#16162=VECTOR('',#51459,1000.);
#16163=VECTOR('',#51462,1000.);
#16164=VECTOR('',#51465,1000.);
#16165=VECTOR('',#51468,1000.);
#16166=VECTOR('',#51473,1000.);
#16167=VECTOR('',#51474,1000.);
#16168=VECTOR('',#51477,1000.);
#16169=VECTOR('',#51480,1000.);
#16170=VECTOR('',#51483,1000.);
#16171=VECTOR('',#51486,1000.);
#16172=VECTOR('',#51491,1000.);
#16173=VECTOR('',#51492,1000.);
#16174=VECTOR('',#51495,1000.);
#16175=VECTOR('',#51498,1000.);
#16176=VECTOR('',#51501,1000.);
#16177=VECTOR('',#51504,1000.);
#16178=VECTOR('',#51509,1000.);
#16179=VECTOR('',#51510,1000.);
#16180=VECTOR('',#51513,1000.);
#16181=VECTOR('',#51516,1000.);
#16182=VECTOR('',#51519,1000.);
#16183=VECTOR('',#51522,1000.);
#16184=VECTOR('',#51527,1000.);
#16185=VECTOR('',#51528,1000.);
#16186=VECTOR('',#51531,1000.);
#16187=VECTOR('',#51534,1000.);
#16188=VECTOR('',#51537,1000.);
#16189=VECTOR('',#51540,1000.);
#16190=VECTOR('',#51545,1000.);
#16191=VECTOR('',#51546,1000.);
#16192=VECTOR('',#51549,1000.);
#16193=VECTOR('',#51552,1000.);
#16194=VECTOR('',#51555,1000.);
#16195=VECTOR('',#51558,1000.);
#16196=VECTOR('',#51563,1000.);
#16197=VECTOR('',#51564,1000.);
#16198=VECTOR('',#51567,1000.);
#16199=VECTOR('',#51570,1000.);
#16200=VECTOR('',#51573,1000.);
#16201=VECTOR('',#51576,1000.);
#16202=VECTOR('',#51581,1000.);
#16203=VECTOR('',#51582,1000.);
#16204=VECTOR('',#51585,1000.);
#16205=VECTOR('',#51588,1000.);
#16206=VECTOR('',#51591,1000.);
#16207=VECTOR('',#51594,1000.);
#16208=VECTOR('',#51599,1000.);
#16209=VECTOR('',#51600,1000.);
#16210=VECTOR('',#51603,1000.);
#16211=VECTOR('',#51606,1000.);
#16212=VECTOR('',#51609,1000.);
#16213=VECTOR('',#51612,1000.);
#16214=VECTOR('',#51617,1000.);
#16215=VECTOR('',#51618,1000.);
#16216=VECTOR('',#51621,1000.);
#16217=VECTOR('',#51624,1000.);
#16218=VECTOR('',#51627,1000.);
#16219=VECTOR('',#51630,1000.);
#16220=VECTOR('',#51635,1000.);
#16221=VECTOR('',#51636,1000.);
#16222=VECTOR('',#51639,1000.);
#16223=VECTOR('',#51642,1000.);
#16224=VECTOR('',#51645,1000.);
#16225=VECTOR('',#51648,1000.);
#16226=VECTOR('',#51653,1000.);
#16227=VECTOR('',#51654,1000.);
#16228=VECTOR('',#51657,1000.);
#16229=VECTOR('',#51660,1000.);
#16230=VECTOR('',#51663,1000.);
#16231=VECTOR('',#51666,1000.);
#16232=VECTOR('',#51671,1000.);
#16233=VECTOR('',#51672,1000.);
#16234=VECTOR('',#51675,1000.);
#16235=VECTOR('',#51678,1000.);
#16236=VECTOR('',#51681,1000.);
#16237=VECTOR('',#51684,1000.);
#16238=VECTOR('',#51689,1000.);
#16239=VECTOR('',#51690,1000.);
#16240=VECTOR('',#51693,1000.);
#16241=VECTOR('',#51696,1000.);
#16242=VECTOR('',#51699,1000.);
#16243=VECTOR('',#51702,1000.);
#16244=VECTOR('',#51707,1000.);
#16245=VECTOR('',#51708,1000.);
#16246=VECTOR('',#51711,1000.);
#16247=VECTOR('',#51714,1000.);
#16248=VECTOR('',#51717,1000.);
#16249=VECTOR('',#51720,1000.);
#16250=VECTOR('',#51725,1000.);
#16251=VECTOR('',#51726,1000.);
#16252=VECTOR('',#51729,1000.);
#16253=VECTOR('',#51732,1000.);
#16254=VECTOR('',#51735,1000.);
#16255=VECTOR('',#51738,1000.);
#16256=VECTOR('',#51743,1000.);
#16257=VECTOR('',#51744,1000.);
#16258=VECTOR('',#51747,1000.);
#16259=VECTOR('',#51750,1000.);
#16260=VECTOR('',#51753,1000.);
#16261=VECTOR('',#51756,1000.);
#16262=VECTOR('',#51761,1000.);
#16263=VECTOR('',#51762,1000.);
#16264=VECTOR('',#51765,1000.);
#16265=VECTOR('',#51768,1000.);
#16266=VECTOR('',#51771,1000.);
#16267=VECTOR('',#51774,1000.);
#16268=VECTOR('',#51779,1000.);
#16269=VECTOR('',#51780,1000.);
#16270=VECTOR('',#51783,1000.);
#16271=VECTOR('',#51786,1000.);
#16272=VECTOR('',#51789,1000.);
#16273=VECTOR('',#51792,1000.);
#16274=VECTOR('',#51797,1000.);
#16275=VECTOR('',#51798,1000.);
#16276=VECTOR('',#51801,1000.);
#16277=VECTOR('',#51804,1000.);
#16278=VECTOR('',#51807,1000.);
#16279=VECTOR('',#51810,1000.);
#16280=VECTOR('',#51815,1000.);
#16281=VECTOR('',#51816,1000.);
#16282=VECTOR('',#51819,1000.);
#16283=VECTOR('',#51822,1000.);
#16284=VECTOR('',#51825,1000.);
#16285=VECTOR('',#51828,1000.);
#16286=VECTOR('',#51833,1000.);
#16287=VECTOR('',#51834,1000.);
#16288=VECTOR('',#51837,1000.);
#16289=VECTOR('',#51840,1000.);
#16290=VECTOR('',#51843,1000.);
#16291=VECTOR('',#51846,1000.);
#16292=VECTOR('',#51851,1000.);
#16293=VECTOR('',#51852,1000.);
#16294=VECTOR('',#51855,1000.);
#16295=VECTOR('',#51858,1000.);
#16296=VECTOR('',#51861,1000.);
#16297=VECTOR('',#51864,1000.);
#16298=VECTOR('',#51869,1000.);
#16299=VECTOR('',#51870,1000.);
#16300=VECTOR('',#51873,1000.);
#16301=VECTOR('',#51876,1000.);
#16302=VECTOR('',#51879,1000.);
#16303=VECTOR('',#51882,1000.);
#16304=VECTOR('',#51887,1000.);
#16305=VECTOR('',#51888,1000.);
#16306=VECTOR('',#51891,1000.);
#16307=VECTOR('',#51894,1000.);
#16308=VECTOR('',#51897,1000.);
#16309=VECTOR('',#51900,1000.);
#16310=VECTOR('',#51905,1000.);
#16311=VECTOR('',#51906,1000.);
#16312=VECTOR('',#51909,1000.);
#16313=VECTOR('',#51912,1000.);
#16314=VECTOR('',#51915,1000.);
#16315=VECTOR('',#51918,1000.);
#16316=VECTOR('',#51923,1000.);
#16317=VECTOR('',#51924,1000.);
#16318=VECTOR('',#51927,1000.);
#16319=VECTOR('',#51930,1000.);
#16320=VECTOR('',#51933,1000.);
#16321=VECTOR('',#51936,1000.);
#16322=VECTOR('',#51941,1000.);
#16323=VECTOR('',#51942,1000.);
#16324=VECTOR('',#51945,1000.);
#16325=VECTOR('',#51948,1000.);
#16326=VECTOR('',#51951,1000.);
#16327=VECTOR('',#51954,1000.);
#16328=VECTOR('',#51959,1000.);
#16329=VECTOR('',#51960,1000.);
#16330=VECTOR('',#51963,1000.);
#16331=VECTOR('',#51966,1000.);
#16332=VECTOR('',#51969,1000.);
#16333=VECTOR('',#51972,1000.);
#16334=VECTOR('',#51977,1000.);
#16335=VECTOR('',#51978,1000.);
#16336=VECTOR('',#51981,1000.);
#16337=VECTOR('',#51984,1000.);
#16338=VECTOR('',#51987,1000.);
#16339=VECTOR('',#51990,1000.);
#16340=VECTOR('',#51995,1000.);
#16341=VECTOR('',#51996,1000.);
#16342=VECTOR('',#51999,1000.);
#16343=VECTOR('',#52002,1000.);
#16344=VECTOR('',#52005,1000.);
#16345=VECTOR('',#52008,1000.);
#16346=VECTOR('',#52013,1000.);
#16347=VECTOR('',#52014,1000.);
#16348=VECTOR('',#52017,1000.);
#16349=VECTOR('',#52020,1000.);
#16350=VECTOR('',#52023,1000.);
#16351=VECTOR('',#52026,1000.);
#16352=VECTOR('',#52031,1000.);
#16353=VECTOR('',#52032,1000.);
#16354=VECTOR('',#52035,1000.);
#16355=VECTOR('',#52038,1000.);
#16356=VECTOR('',#52041,1000.);
#16357=VECTOR('',#52044,1000.);
#16358=VECTOR('',#52049,1000.);
#16359=VECTOR('',#52050,1000.);
#16360=VECTOR('',#52053,1000.);
#16361=VECTOR('',#52056,1000.);
#16362=VECTOR('',#52059,1000.);
#16363=VECTOR('',#52062,1000.);
#16364=VECTOR('',#52067,1000.);
#16365=VECTOR('',#52068,1000.);
#16366=VECTOR('',#52071,1000.);
#16367=VECTOR('',#52074,1000.);
#16368=VECTOR('',#52077,1000.);
#16369=VECTOR('',#52080,1000.);
#16370=VECTOR('',#52085,1000.);
#16371=VECTOR('',#52086,1000.);
#16372=VECTOR('',#52089,1000.);
#16373=VECTOR('',#52092,1000.);
#16374=VECTOR('',#52095,1000.);
#16375=VECTOR('',#52098,1000.);
#16376=VECTOR('',#52103,1000.);
#16377=VECTOR('',#52104,1000.);
#16378=VECTOR('',#52107,1000.);
#16379=VECTOR('',#52110,1000.);
#16380=VECTOR('',#52113,1000.);
#16381=VECTOR('',#52116,1000.);
#16382=VECTOR('',#52121,1000.);
#16383=VECTOR('',#52122,1000.);
#16384=VECTOR('',#52125,1000.);
#16385=VECTOR('',#52128,1000.);
#16386=VECTOR('',#52131,1000.);
#16387=VECTOR('',#52134,1000.);
#16388=VECTOR('',#52139,1000.);
#16389=VECTOR('',#52140,1000.);
#16390=VECTOR('',#52143,1000.);
#16391=VECTOR('',#52146,1000.);
#16392=VECTOR('',#52149,1000.);
#16393=VECTOR('',#52152,1000.);
#16394=VECTOR('',#52157,1000.);
#16395=VECTOR('',#52158,1000.);
#16396=VECTOR('',#52161,1000.);
#16397=VECTOR('',#52164,1000.);
#16398=VECTOR('',#52167,1000.);
#16399=VECTOR('',#52170,1000.);
#16400=VECTOR('',#52175,1000.);
#16401=VECTOR('',#52176,1000.);
#16402=VECTOR('',#52179,1000.);
#16403=VECTOR('',#52182,1000.);
#16404=VECTOR('',#52185,1000.);
#16405=VECTOR('',#52188,1000.);
#16406=VECTOR('',#52193,1000.);
#16407=VECTOR('',#52194,1000.);
#16408=VECTOR('',#52197,1000.);
#16409=VECTOR('',#52200,1000.);
#16410=VECTOR('',#52203,1000.);
#16411=VECTOR('',#52206,1000.);
#16412=VECTOR('',#52211,1000.);
#16413=VECTOR('',#52212,1000.);
#16414=VECTOR('',#52215,1000.);
#16415=VECTOR('',#52218,1000.);
#16416=VECTOR('',#52221,1000.);
#16417=VECTOR('',#52224,1000.);
#16418=VECTOR('',#52229,1000.);
#16419=VECTOR('',#52230,1000.);
#16420=VECTOR('',#52233,1000.);
#16421=VECTOR('',#52236,1000.);
#16422=VECTOR('',#52239,1000.);
#16423=VECTOR('',#52242,1000.);
#16424=VECTOR('',#52247,1000.);
#16425=VECTOR('',#52248,1000.);
#16426=VECTOR('',#52251,1000.);
#16427=VECTOR('',#52254,1000.);
#16428=VECTOR('',#52257,1000.);
#16429=VECTOR('',#52260,1000.);
#16430=VECTOR('',#52265,1000.);
#16431=VECTOR('',#52266,1000.);
#16432=VECTOR('',#52269,1000.);
#16433=VECTOR('',#52272,1000.);
#16434=VECTOR('',#52275,1000.);
#16435=VECTOR('',#52278,1000.);
#16436=VECTOR('',#52283,1000.);
#16437=VECTOR('',#52284,1000.);
#16438=VECTOR('',#52287,1000.);
#16439=VECTOR('',#52290,1000.);
#16440=VECTOR('',#52293,1000.);
#16441=VECTOR('',#52296,1000.);
#16442=VECTOR('',#52301,1000.);
#16443=VECTOR('',#52302,1000.);
#16444=VECTOR('',#52305,1000.);
#16445=VECTOR('',#52308,1000.);
#16446=VECTOR('',#52311,1000.);
#16447=VECTOR('',#52314,1000.);
#16448=VECTOR('',#52319,1000.);
#16449=VECTOR('',#52320,1000.);
#16450=VECTOR('',#52323,1000.);
#16451=VECTOR('',#52326,1000.);
#16452=VECTOR('',#52329,1000.);
#16453=VECTOR('',#52332,1000.);
#16454=VECTOR('',#52337,1000.);
#16455=VECTOR('',#52338,1000.);
#16456=VECTOR('',#52341,1000.);
#16457=VECTOR('',#52344,1000.);
#16458=VECTOR('',#52347,1000.);
#16459=VECTOR('',#52350,1000.);
#16460=VECTOR('',#52355,1000.);
#16461=VECTOR('',#52356,1000.);
#16462=VECTOR('',#52359,1000.);
#16463=VECTOR('',#52362,1000.);
#16464=VECTOR('',#52365,1000.);
#16465=VECTOR('',#52368,1000.);
#16466=VECTOR('',#52373,1000.);
#16467=VECTOR('',#52374,1000.);
#16468=VECTOR('',#52377,1000.);
#16469=VECTOR('',#52380,1000.);
#16470=VECTOR('',#52383,1000.);
#16471=VECTOR('',#52386,1000.);
#16472=VECTOR('',#52391,1000.);
#16473=VECTOR('',#52392,1000.);
#16474=VECTOR('',#52395,1000.);
#16475=VECTOR('',#52398,1000.);
#16476=VECTOR('',#52401,1000.);
#16477=VECTOR('',#52404,1000.);
#16478=VECTOR('',#52409,1000.);
#16479=VECTOR('',#52410,1000.);
#16480=VECTOR('',#52413,1000.);
#16481=VECTOR('',#52416,1000.);
#16482=VECTOR('',#52419,1000.);
#16483=VECTOR('',#52422,1000.);
#16484=VECTOR('',#52427,1000.);
#16485=VECTOR('',#52428,1000.);
#16486=VECTOR('',#52431,1000.);
#16487=VECTOR('',#52434,1000.);
#16488=VECTOR('',#52437,1000.);
#16489=VECTOR('',#52440,1000.);
#17110=CIRCLE('',#41309,59.9898979485574);
#17111=CIRCLE('',#41310,0.5);
#17112=CIRCLE('',#41311,59.5);
#17113=CIRCLE('',#41313,60.7737346662472);
#17114=CIRCLE('',#41314,1.2);
#17115=CIRCLE('',#41315,61.9494897427832);
#17116=CIRCLE('',#41317,59.5);
#17117=CIRCLE('',#41318,1.3);
#17118=CIRCLE('',#41320,61.9494897427832);
#17119=CIRCLE('',#41321,2.);
#17120=CIRCLE('',#41333,0.799999999999995);
#17121=CIRCLE('',#41334,1.6);
#17122=CIRCLE('',#41336,0.799999999999995);
#17123=CIRCLE('',#41337,1.6);
#17124=CIRCLE('',#41341,0.799999999999995);
#17125=CIRCLE('',#41342,1.6);
#17126=CIRCLE('',#41344,0.799999999999995);
#17127=CIRCLE('',#41345,1.6);
#17128=CIRCLE('',#41349,5.);
#17129=CIRCLE('',#41350,5.);
#17130=CIRCLE('',#41353,5.);
#17131=CIRCLE('',#41354,5.);
#17132=CIRCLE('',#41363,0.799999999999995);
#17133=CIRCLE('',#41364,1.6);
#17134=CIRCLE('',#41366,0.799999999999995);
#17135=CIRCLE('',#41367,1.6);
#17136=CIRCLE('',#41371,0.799999999999995);
#17137=CIRCLE('',#41372,1.6);
#17138=CIRCLE('',#41374,0.799999999999995);
#17139=CIRCLE('',#41375,1.6);
#17140=CIRCLE('',#41379,5.);
#17141=CIRCLE('',#41380,5.);
#17142=CIRCLE('',#41383,5.);
#17143=CIRCLE('',#41384,5.);
#18554=VERTEX_POINT('',#58350);
#18555=VERTEX_POINT('',#58352);
#18556=VERTEX_POINT('',#58356);
#18557=VERTEX_POINT('',#58358);
#18558=VERTEX_POINT('',#58362);
#18559=VERTEX_POINT('',#58366);
#18560=VERTEX_POINT('',#58370);
#18561=VERTEX_POINT('',#58371);
#18562=VERTEX_POINT('',#58373);
#18563=VERTEX_POINT('',#58375);
#18564=VERTEX_POINT('',#58377);
#18565=VERTEX_POINT('',#58379);
#18566=VERTEX_POINT('',#58381);
#18567=VERTEX_POINT('',#58383);
#18568=VERTEX_POINT('',#58385);
#18569=VERTEX_POINT('',#58387);
#18570=VERTEX_POINT('',#58389);
#18571=VERTEX_POINT('',#58391);
#18572=VERTEX_POINT('',#58395);
#18573=VERTEX_POINT('',#58396);
#18574=VERTEX_POINT('',#58398);
#18575=VERTEX_POINT('',#58400);
#18576=VERTEX_POINT('',#58402);
#18577=VERTEX_POINT('',#58404);
#18578=VERTEX_POINT('',#58406);
#18579=VERTEX_POINT('',#58408);
#18580=VERTEX_POINT('',#58410);
#18581=VERTEX_POINT('',#58412);
#18582=VERTEX_POINT('',#58414);
#18583=VERTEX_POINT('',#58416);
#18584=VERTEX_POINT('',#58440);
#18585=VERTEX_POINT('',#58441);
#18586=VERTEX_POINT('',#58446);
#18587=VERTEX_POINT('',#58448);
#18588=VERTEX_POINT('',#58456);
#18589=VERTEX_POINT('',#58458);
#18590=VERTEX_POINT('',#58462);
#18591=VERTEX_POINT('',#58463);
#18592=VERTEX_POINT('',#58472);
#18593=VERTEX_POINT('',#58473);
#18594=VERTEX_POINT('',#58475);
#18595=VERTEX_POINT('',#58477);
#18596=VERTEX_POINT('',#58481);
#18597=VERTEX_POINT('',#58482);
#18598=VERTEX_POINT('',#58484);
#18599=VERTEX_POINT('',#58486);
#18600=VERTEX_POINT('',#58490);
#18601=VERTEX_POINT('',#58491);
#18602=VERTEX_POINT('',#58493);
#18603=VERTEX_POINT('',#58495);
#18604=VERTEX_POINT('',#58516);
#18605=VERTEX_POINT('',#58517);
#18606=VERTEX_POINT('',#58522);
#18607=VERTEX_POINT('',#58524);
#18608=VERTEX_POINT('',#58532);
#18609=VERTEX_POINT('',#58534);
#18610=VERTEX_POINT('',#58538);
#18611=VERTEX_POINT('',#58539);
#18612=VERTEX_POINT('',#58548);
#18613=VERTEX_POINT('',#58549);
#18614=VERTEX_POINT('',#58551);
#18615=VERTEX_POINT('',#58553);
#18616=VERTEX_POINT('',#58557);
#18617=VERTEX_POINT('',#58558);
#18618=VERTEX_POINT('',#58560);
#18619=VERTEX_POINT('',#58562);
#18620=VERTEX_POINT('',#58566);
#18621=VERTEX_POINT('',#58567);
#18622=VERTEX_POINT('',#58569);
#18623=VERTEX_POINT('',#58571);
#18624=VERTEX_POINT('',#58592);
#18625=VERTEX_POINT('',#58593);
#18626=VERTEX_POINT('',#58595);
#18627=VERTEX_POINT('',#58597);
#18628=VERTEX_POINT('',#58599);
#18629=VERTEX_POINT('',#58601);
#18630=VERTEX_POINT('',#58604);
#18631=VERTEX_POINT('',#58605);
#18632=VERTEX_POINT('',#58607);
#18633=VERTEX_POINT('',#58609);
#18634=VERTEX_POINT('',#58611);
#18635=VERTEX_POINT('',#58613);
#18636=VERTEX_POINT('',#58616);
#18637=VERTEX_POINT('',#58617);
#18638=VERTEX_POINT('',#58619);
#18639=VERTEX_POINT('',#58621);
#18640=VERTEX_POINT('',#58623);
#18641=VERTEX_POINT('',#58625);
#18642=VERTEX_POINT('',#58628);
#18643=VERTEX_POINT('',#58629);
#18644=VERTEX_POINT('',#58631);
#18645=VERTEX_POINT('',#58633);
#18646=VERTEX_POINT('',#58635);
#18647=VERTEX_POINT('',#58637);
#18648=VERTEX_POINT('',#58640);
#18649=VERTEX_POINT('',#58641);
#18650=VERTEX_POINT('',#58643);
#18651=VERTEX_POINT('',#58645);
#18652=VERTEX_POINT('',#58647);
#18653=VERTEX_POINT('',#58649);
#18654=VERTEX_POINT('',#58652);
#18655=VERTEX_POINT('',#58653);
#18656=VERTEX_POINT('',#58655);
#18657=VERTEX_POINT('',#58657);
#18658=VERTEX_POINT('',#58659);
#18659=VERTEX_POINT('',#58661);
#18660=VERTEX_POINT('',#58664);
#18661=VERTEX_POINT('',#58665);
#18662=VERTEX_POINT('',#58667);
#18663=VERTEX_POINT('',#58669);
#18664=VERTEX_POINT('',#58671);
#18665=VERTEX_POINT('',#58673);
#18666=VERTEX_POINT('',#58676);
#18667=VERTEX_POINT('',#58677);
#18668=VERTEX_POINT('',#58679);
#18669=VERTEX_POINT('',#58681);
#18670=VERTEX_POINT('',#58683);
#18671=VERTEX_POINT('',#58685);
#18672=VERTEX_POINT('',#58688);
#18673=VERTEX_POINT('',#58689);
#18674=VERTEX_POINT('',#58691);
#18675=VERTEX_POINT('',#58693);
#18676=VERTEX_POINT('',#58695);
#18677=VERTEX_POINT('',#58697);
#18678=VERTEX_POINT('',#58700);
#18679=VERTEX_POINT('',#58701);
#18680=VERTEX_POINT('',#58703);
#18681=VERTEX_POINT('',#58705);
#18682=VERTEX_POINT('',#58707);
#18683=VERTEX_POINT('',#58709);
#18684=VERTEX_POINT('',#58712);
#18685=VERTEX_POINT('',#58713);
#18686=VERTEX_POINT('',#58715);
#18687=VERTEX_POINT('',#58717);
#18688=VERTEX_POINT('',#58719);
#18689=VERTEX_POINT('',#58721);
#18690=VERTEX_POINT('',#58724);
#18691=VERTEX_POINT('',#58725);
#18692=VERTEX_POINT('',#58727);
#18693=VERTEX_POINT('',#58729);
#18694=VERTEX_POINT('',#58731);
#18695=VERTEX_POINT('',#58733);
#18696=VERTEX_POINT('',#58736);
#18697=VERTEX_POINT('',#58737);
#18698=VERTEX_POINT('',#58739);
#18699=VERTEX_POINT('',#58741);
#18700=VERTEX_POINT('',#58743);
#18701=VERTEX_POINT('',#58745);
#18702=VERTEX_POINT('',#58748);
#18703=VERTEX_POINT('',#58749);
#18704=VERTEX_POINT('',#58751);
#18705=VERTEX_POINT('',#58753);
#18706=VERTEX_POINT('',#58755);
#18707=VERTEX_POINT('',#58757);
#18708=VERTEX_POINT('',#58760);
#18709=VERTEX_POINT('',#58761);
#18710=VERTEX_POINT('',#58763);
#18711=VERTEX_POINT('',#58765);
#18712=VERTEX_POINT('',#58767);
#18713=VERTEX_POINT('',#58769);
#18714=VERTEX_POINT('',#58772);
#18715=VERTEX_POINT('',#58773);
#18716=VERTEX_POINT('',#58775);
#18717=VERTEX_POINT('',#58777);
#18718=VERTEX_POINT('',#58779);
#18719=VERTEX_POINT('',#58781);
#18720=VERTEX_POINT('',#58784);
#18721=VERTEX_POINT('',#58785);
#18722=VERTEX_POINT('',#58787);
#18723=VERTEX_POINT('',#58789);
#18724=VERTEX_POINT('',#58791);
#18725=VERTEX_POINT('',#58793);
#18726=VERTEX_POINT('',#58796);
#18727=VERTEX_POINT('',#58797);
#18728=VERTEX_POINT('',#58799);
#18729=VERTEX_POINT('',#58801);
#18730=VERTEX_POINT('',#58803);
#18731=VERTEX_POINT('',#58805);
#18732=VERTEX_POINT('',#58808);
#18733=VERTEX_POINT('',#58809);
#18734=VERTEX_POINT('',#58811);
#18735=VERTEX_POINT('',#58813);
#18736=VERTEX_POINT('',#58815);
#18737=VERTEX_POINT('',#58817);
#18738=VERTEX_POINT('',#58820);
#18739=VERTEX_POINT('',#58821);
#18740=VERTEX_POINT('',#58823);
#18741=VERTEX_POINT('',#58825);
#18742=VERTEX_POINT('',#58827);
#18743=VERTEX_POINT('',#58829);
#18744=VERTEX_POINT('',#58832);
#18745=VERTEX_POINT('',#58833);
#18746=VERTEX_POINT('',#58835);
#18747=VERTEX_POINT('',#58837);
#18748=VERTEX_POINT('',#58839);
#18749=VERTEX_POINT('',#58841);
#18750=VERTEX_POINT('',#58844);
#18751=VERTEX_POINT('',#58845);
#18752=VERTEX_POINT('',#58847);
#18753=VERTEX_POINT('',#58849);
#18754=VERTEX_POINT('',#58851);
#18755=VERTEX_POINT('',#58853);
#18756=VERTEX_POINT('',#58856);
#18757=VERTEX_POINT('',#58857);
#18758=VERTEX_POINT('',#58859);
#18759=VERTEX_POINT('',#58861);
#18760=VERTEX_POINT('',#58863);
#18761=VERTEX_POINT('',#58865);
#18762=VERTEX_POINT('',#58868);
#18763=VERTEX_POINT('',#58869);
#18764=VERTEX_POINT('',#58871);
#18765=VERTEX_POINT('',#58873);
#18766=VERTEX_POINT('',#58875);
#18767=VERTEX_POINT('',#58877);
#18768=VERTEX_POINT('',#58880);
#18769=VERTEX_POINT('',#58881);
#18770=VERTEX_POINT('',#58883);
#18771=VERTEX_POINT('',#58885);
#18772=VERTEX_POINT('',#58887);
#18773=VERTEX_POINT('',#58889);
#18774=VERTEX_POINT('',#58892);
#18775=VERTEX_POINT('',#58893);
#18776=VERTEX_POINT('',#58895);
#18777=VERTEX_POINT('',#58897);
#18778=VERTEX_POINT('',#58899);
#18779=VERTEX_POINT('',#58901);
#18780=VERTEX_POINT('',#58904);
#18781=VERTEX_POINT('',#58905);
#18782=VERTEX_POINT('',#58907);
#18783=VERTEX_POINT('',#58909);
#18784=VERTEX_POINT('',#58911);
#18785=VERTEX_POINT('',#58913);
#18786=VERTEX_POINT('',#58916);
#18787=VERTEX_POINT('',#58917);
#18788=VERTEX_POINT('',#58919);
#18789=VERTEX_POINT('',#58921);
#18790=VERTEX_POINT('',#58923);
#18791=VERTEX_POINT('',#58925);
#18792=VERTEX_POINT('',#58928);
#18793=VERTEX_POINT('',#58929);
#18794=VERTEX_POINT('',#58931);
#18795=VERTEX_POINT('',#58933);
#18796=VERTEX_POINT('',#58935);
#18797=VERTEX_POINT('',#58937);
#18798=VERTEX_POINT('',#58940);
#18799=VERTEX_POINT('',#58941);
#18800=VERTEX_POINT('',#58943);
#18801=VERTEX_POINT('',#58945);
#18802=VERTEX_POINT('',#58947);
#18803=VERTEX_POINT('',#58949);
#18804=VERTEX_POINT('',#58952);
#18805=VERTEX_POINT('',#58953);
#18806=VERTEX_POINT('',#58955);
#18807=VERTEX_POINT('',#58957);
#18808=VERTEX_POINT('',#58959);
#18809=VERTEX_POINT('',#58961);
#18810=VERTEX_POINT('',#58964);
#18811=VERTEX_POINT('',#58965);
#18812=VERTEX_POINT('',#58967);
#18813=VERTEX_POINT('',#58969);
#18814=VERTEX_POINT('',#58971);
#18815=VERTEX_POINT('',#58973);
#18816=VERTEX_POINT('',#58976);
#18817=VERTEX_POINT('',#58977);
#18818=VERTEX_POINT('',#58979);
#18819=VERTEX_POINT('',#58981);
#18820=VERTEX_POINT('',#58983);
#18821=VERTEX_POINT('',#58985);
#18822=VERTEX_POINT('',#58988);
#18823=VERTEX_POINT('',#58989);
#18824=VERTEX_POINT('',#58991);
#18825=VERTEX_POINT('',#58993);
#18826=VERTEX_POINT('',#58995);
#18827=VERTEX_POINT('',#58997);
#18828=VERTEX_POINT('',#59000);
#18829=VERTEX_POINT('',#59001);
#18830=VERTEX_POINT('',#59003);
#18831=VERTEX_POINT('',#59005);
#18832=VERTEX_POINT('',#59007);
#18833=VERTEX_POINT('',#59009);
#18834=VERTEX_POINT('',#59012);
#18835=VERTEX_POINT('',#59013);
#18836=VERTEX_POINT('',#59015);
#18837=VERTEX_POINT('',#59017);
#18838=VERTEX_POINT('',#59019);
#18839=VERTEX_POINT('',#59021);
#18840=VERTEX_POINT('',#59024);
#18841=VERTEX_POINT('',#59025);
#18842=VERTEX_POINT('',#59027);
#18843=VERTEX_POINT('',#59029);
#18844=VERTEX_POINT('',#59031);
#18845=VERTEX_POINT('',#59033);
#18846=VERTEX_POINT('',#59036);
#18847=VERTEX_POINT('',#59037);
#18848=VERTEX_POINT('',#59039);
#18849=VERTEX_POINT('',#59041);
#18850=VERTEX_POINT('',#59043);
#18851=VERTEX_POINT('',#59045);
#18852=VERTEX_POINT('',#59048);
#18853=VERTEX_POINT('',#59049);
#18854=VERTEX_POINT('',#59051);
#18855=VERTEX_POINT('',#59053);
#18856=VERTEX_POINT('',#59055);
#18857=VERTEX_POINT('',#59057);
#18858=VERTEX_POINT('',#59060);
#18859=VERTEX_POINT('',#59061);
#18860=VERTEX_POINT('',#59063);
#18861=VERTEX_POINT('',#59065);
#18862=VERTEX_POINT('',#59067);
#18863=VERTEX_POINT('',#59069);
#18864=VERTEX_POINT('',#59072);
#18865=VERTEX_POINT('',#59073);
#18866=VERTEX_POINT('',#59075);
#18867=VERTEX_POINT('',#59077);
#18868=VERTEX_POINT('',#59079);
#18869=VERTEX_POINT('',#59081);
#18870=VERTEX_POINT('',#59084);
#18871=VERTEX_POINT('',#59085);
#18872=VERTEX_POINT('',#59087);
#18873=VERTEX_POINT('',#59089);
#18874=VERTEX_POINT('',#59091);
#18875=VERTEX_POINT('',#59093);
#18876=VERTEX_POINT('',#59096);
#18877=VERTEX_POINT('',#59097);
#18878=VERTEX_POINT('',#59099);
#18879=VERTEX_POINT('',#59101);
#18880=VERTEX_POINT('',#59103);
#18881=VERTEX_POINT('',#59105);
#18882=VERTEX_POINT('',#59108);
#18883=VERTEX_POINT('',#59109);
#18884=VERTEX_POINT('',#59111);
#18885=VERTEX_POINT('',#59113);
#18886=VERTEX_POINT('',#59115);
#18887=VERTEX_POINT('',#59117);
#18888=VERTEX_POINT('',#59120);
#18889=VERTEX_POINT('',#59121);
#18890=VERTEX_POINT('',#59123);
#18891=VERTEX_POINT('',#59125);
#18892=VERTEX_POINT('',#59127);
#18893=VERTEX_POINT('',#59129);
#18894=VERTEX_POINT('',#59132);
#18895=VERTEX_POINT('',#59133);
#18896=VERTEX_POINT('',#59135);
#18897=VERTEX_POINT('',#59137);
#18898=VERTEX_POINT('',#59139);
#18899=VERTEX_POINT('',#59141);
#18900=VERTEX_POINT('',#59144);
#18901=VERTEX_POINT('',#59145);
#18902=VERTEX_POINT('',#59147);
#18903=VERTEX_POINT('',#59149);
#18904=VERTEX_POINT('',#59151);
#18905=VERTEX_POINT('',#59153);
#18906=VERTEX_POINT('',#59156);
#18907=VERTEX_POINT('',#59157);
#18908=VERTEX_POINT('',#59159);
#18909=VERTEX_POINT('',#59161);
#18910=VERTEX_POINT('',#59163);
#18911=VERTEX_POINT('',#59165);
#18912=VERTEX_POINT('',#59168);
#18913=VERTEX_POINT('',#59169);
#18914=VERTEX_POINT('',#59171);
#18915=VERTEX_POINT('',#59173);
#18916=VERTEX_POINT('',#59175);
#18917=VERTEX_POINT('',#59177);
#18918=VERTEX_POINT('',#59180);
#18919=VERTEX_POINT('',#59181);
#18920=VERTEX_POINT('',#59183);
#18921=VERTEX_POINT('',#59185);
#18922=VERTEX_POINT('',#59187);
#18923=VERTEX_POINT('',#59189);
#18924=VERTEX_POINT('',#59192);
#18925=VERTEX_POINT('',#59193);
#18926=VERTEX_POINT('',#59195);
#18927=VERTEX_POINT('',#59197);
#18928=VERTEX_POINT('',#59199);
#18929=VERTEX_POINT('',#59201);
#18930=VERTEX_POINT('',#59204);
#18931=VERTEX_POINT('',#59205);
#18932=VERTEX_POINT('',#59207);
#18933=VERTEX_POINT('',#59209);
#18934=VERTEX_POINT('',#59211);
#18935=VERTEX_POINT('',#59213);
#18936=VERTEX_POINT('',#59216);
#18937=VERTEX_POINT('',#59217);
#18938=VERTEX_POINT('',#59219);
#18939=VERTEX_POINT('',#59221);
#18940=VERTEX_POINT('',#59223);
#18941=VERTEX_POINT('',#59225);
#18942=VERTEX_POINT('',#59228);
#18943=VERTEX_POINT('',#59229);
#18944=VERTEX_POINT('',#59231);
#18945=VERTEX_POINT('',#59233);
#18946=VERTEX_POINT('',#59235);
#18947=VERTEX_POINT('',#59237);
#18948=VERTEX_POINT('',#59240);
#18949=VERTEX_POINT('',#59241);
#18950=VERTEX_POINT('',#59243);
#18951=VERTEX_POINT('',#59245);
#18952=VERTEX_POINT('',#59247);
#18953=VERTEX_POINT('',#59249);
#18954=VERTEX_POINT('',#59252);
#18955=VERTEX_POINT('',#59253);
#18956=VERTEX_POINT('',#59255);
#18957=VERTEX_POINT('',#59257);
#18958=VERTEX_POINT('',#59259);
#18959=VERTEX_POINT('',#59261);
#18960=VERTEX_POINT('',#59264);
#18961=VERTEX_POINT('',#59265);
#18962=VERTEX_POINT('',#59267);
#18963=VERTEX_POINT('',#59269);
#18964=VERTEX_POINT('',#59271);
#18965=VERTEX_POINT('',#59273);
#18966=VERTEX_POINT('',#59276);
#18967=VERTEX_POINT('',#59277);
#18968=VERTEX_POINT('',#59279);
#18969=VERTEX_POINT('',#59281);
#18970=VERTEX_POINT('',#59283);
#18971=VERTEX_POINT('',#59285);
#18972=VERTEX_POINT('',#59288);
#18973=VERTEX_POINT('',#59289);
#18974=VERTEX_POINT('',#59291);
#18975=VERTEX_POINT('',#59293);
#18976=VERTEX_POINT('',#59295);
#18977=VERTEX_POINT('',#59297);
#18978=VERTEX_POINT('',#59300);
#18979=VERTEX_POINT('',#59301);
#18980=VERTEX_POINT('',#59303);
#18981=VERTEX_POINT('',#59305);
#18982=VERTEX_POINT('',#59307);
#18983=VERTEX_POINT('',#59309);
#18984=VERTEX_POINT('',#59312);
#18985=VERTEX_POINT('',#59313);
#18986=VERTEX_POINT('',#59315);
#18987=VERTEX_POINT('',#59317);
#18988=VERTEX_POINT('',#59319);
#18989=VERTEX_POINT('',#59321);
#18990=VERTEX_POINT('',#59324);
#18991=VERTEX_POINT('',#59325);
#18992=VERTEX_POINT('',#59327);
#18993=VERTEX_POINT('',#59329);
#18994=VERTEX_POINT('',#59331);
#18995=VERTEX_POINT('',#59333);
#18996=VERTEX_POINT('',#59336);
#18997=VERTEX_POINT('',#59337);
#18998=VERTEX_POINT('',#59339);
#18999=VERTEX_POINT('',#59341);
#19000=VERTEX_POINT('',#59343);
#19001=VERTEX_POINT('',#59345);
#19002=VERTEX_POINT('',#59348);
#19003=VERTEX_POINT('',#59349);
#19004=VERTEX_POINT('',#59351);
#19005=VERTEX_POINT('',#59353);
#19006=VERTEX_POINT('',#59355);
#19007=VERTEX_POINT('',#59357);
#19008=VERTEX_POINT('',#59360);
#19009=VERTEX_POINT('',#59361);
#19010=VERTEX_POINT('',#59363);
#19011=VERTEX_POINT('',#59365);
#19012=VERTEX_POINT('',#59367);
#19013=VERTEX_POINT('',#59369);
#19014=VERTEX_POINT('',#59372);
#19015=VERTEX_POINT('',#59373);
#19016=VERTEX_POINT('',#59375);
#19017=VERTEX_POINT('',#59377);
#19018=VERTEX_POINT('',#59379);
#19019=VERTEX_POINT('',#59381);
#19020=VERTEX_POINT('',#59384);
#19021=VERTEX_POINT('',#59385);
#19022=VERTEX_POINT('',#59387);
#19023=VERTEX_POINT('',#59389);
#19024=VERTEX_POINT('',#59391);
#19025=VERTEX_POINT('',#59393);
#19026=VERTEX_POINT('',#59396);
#19027=VERTEX_POINT('',#59397);
#19028=VERTEX_POINT('',#59399);
#19029=VERTEX_POINT('',#59401);
#19030=VERTEX_POINT('',#59403);
#19031=VERTEX_POINT('',#59405);
#19032=VERTEX_POINT('',#59408);
#19033=VERTEX_POINT('',#59409);
#19034=VERTEX_POINT('',#59411);
#19035=VERTEX_POINT('',#59413);
#19036=VERTEX_POINT('',#59415);
#19037=VERTEX_POINT('',#59417);
#19038=VERTEX_POINT('',#59420);
#19039=VERTEX_POINT('',#59421);
#19040=VERTEX_POINT('',#59423);
#19041=VERTEX_POINT('',#59425);
#19042=VERTEX_POINT('',#59427);
#19043=VERTEX_POINT('',#59429);
#19044=VERTEX_POINT('',#59432);
#19045=VERTEX_POINT('',#59433);
#19046=VERTEX_POINT('',#59435);
#19047=VERTEX_POINT('',#59437);
#19048=VERTEX_POINT('',#59439);
#19049=VERTEX_POINT('',#59441);
#19050=VERTEX_POINT('',#59444);
#19051=VERTEX_POINT('',#59445);
#19052=VERTEX_POINT('',#59447);
#19053=VERTEX_POINT('',#59449);
#19054=VERTEX_POINT('',#59451);
#19055=VERTEX_POINT('',#59453);
#19056=VERTEX_POINT('',#59456);
#19057=VERTEX_POINT('',#59457);
#19058=VERTEX_POINT('',#59459);
#19059=VERTEX_POINT('',#59461);
#19060=VERTEX_POINT('',#59463);
#19061=VERTEX_POINT('',#59465);
#19062=VERTEX_POINT('',#59468);
#19063=VERTEX_POINT('',#59469);
#19064=VERTEX_POINT('',#59471);
#19065=VERTEX_POINT('',#59473);
#19066=VERTEX_POINT('',#59475);
#19067=VERTEX_POINT('',#59477);
#19068=VERTEX_POINT('',#59480);
#19069=VERTEX_POINT('',#59481);
#19070=VERTEX_POINT('',#59483);
#19071=VERTEX_POINT('',#59485);
#19072=VERTEX_POINT('',#59487);
#19073=VERTEX_POINT('',#59489);
#19074=VERTEX_POINT('',#59492);
#19075=VERTEX_POINT('',#59493);
#19076=VERTEX_POINT('',#59495);
#19077=VERTEX_POINT('',#59497);
#19078=VERTEX_POINT('',#59499);
#19079=VERTEX_POINT('',#59501);
#19080=VERTEX_POINT('',#59504);
#19081=VERTEX_POINT('',#59505);
#19082=VERTEX_POINT('',#59507);
#19083=VERTEX_POINT('',#59509);
#19084=VERTEX_POINT('',#59511);
#19085=VERTEX_POINT('',#59513);
#19086=VERTEX_POINT('',#59516);
#19087=VERTEX_POINT('',#59517);
#19088=VERTEX_POINT('',#59519);
#19089=VERTEX_POINT('',#59521);
#19090=VERTEX_POINT('',#59523);
#19091=VERTEX_POINT('',#59525);
#19092=VERTEX_POINT('',#59528);
#19093=VERTEX_POINT('',#59529);
#19094=VERTEX_POINT('',#59531);
#19095=VERTEX_POINT('',#59533);
#19096=VERTEX_POINT('',#59535);
#19097=VERTEX_POINT('',#59537);
#19098=VERTEX_POINT('',#59540);
#19099=VERTEX_POINT('',#59541);
#19100=VERTEX_POINT('',#59543);
#19101=VERTEX_POINT('',#59545);
#19102=VERTEX_POINT('',#59547);
#19103=VERTEX_POINT('',#59549);
#19104=VERTEX_POINT('',#59552);
#19105=VERTEX_POINT('',#59553);
#19106=VERTEX_POINT('',#59555);
#19107=VERTEX_POINT('',#59557);
#19108=VERTEX_POINT('',#59559);
#19109=VERTEX_POINT('',#59561);
#19110=VERTEX_POINT('',#59564);
#19111=VERTEX_POINT('',#59565);
#19112=VERTEX_POINT('',#59567);
#19113=VERTEX_POINT('',#59569);
#19114=VERTEX_POINT('',#59571);
#19115=VERTEX_POINT('',#59573);
#19116=VERTEX_POINT('',#59576);
#19117=VERTEX_POINT('',#59577);
#19118=VERTEX_POINT('',#59579);
#19119=VERTEX_POINT('',#59581);
#19120=VERTEX_POINT('',#59583);
#19121=VERTEX_POINT('',#59585);
#19122=VERTEX_POINT('',#59588);
#19123=VERTEX_POINT('',#59589);
#19124=VERTEX_POINT('',#59591);
#19125=VERTEX_POINT('',#59593);
#19126=VERTEX_POINT('',#59595);
#19127=VERTEX_POINT('',#59597);
#19128=VERTEX_POINT('',#59600);
#19129=VERTEX_POINT('',#59601);
#19130=VERTEX_POINT('',#59603);
#19131=VERTEX_POINT('',#59605);
#19132=VERTEX_POINT('',#59607);
#19133=VERTEX_POINT('',#59609);
#19134=VERTEX_POINT('',#59612);
#19135=VERTEX_POINT('',#59613);
#19136=VERTEX_POINT('',#59615);
#19137=VERTEX_POINT('',#59617);
#19138=VERTEX_POINT('',#59619);
#19139=VERTEX_POINT('',#59621);
#19140=VERTEX_POINT('',#59624);
#19141=VERTEX_POINT('',#59625);
#19142=VERTEX_POINT('',#59627);
#19143=VERTEX_POINT('',#59629);
#19144=VERTEX_POINT('',#59631);
#19145=VERTEX_POINT('',#59633);
#19146=VERTEX_POINT('',#59636);
#19147=VERTEX_POINT('',#59637);
#19148=VERTEX_POINT('',#59639);
#19149=VERTEX_POINT('',#59641);
#19150=VERTEX_POINT('',#59643);
#19151=VERTEX_POINT('',#59645);
#19152=VERTEX_POINT('',#59648);
#19153=VERTEX_POINT('',#59649);
#19154=VERTEX_POINT('',#59651);
#19155=VERTEX_POINT('',#59653);
#19156=VERTEX_POINT('',#59655);
#19157=VERTEX_POINT('',#59657);
#19158=VERTEX_POINT('',#59660);
#19159=VERTEX_POINT('',#59661);
#19160=VERTEX_POINT('',#59663);
#19161=VERTEX_POINT('',#59665);
#19162=VERTEX_POINT('',#59667);
#19163=VERTEX_POINT('',#59669);
#19164=VERTEX_POINT('',#59672);
#19165=VERTEX_POINT('',#59673);
#19166=VERTEX_POINT('',#59675);
#19167=VERTEX_POINT('',#59677);
#19168=VERTEX_POINT('',#59679);
#19169=VERTEX_POINT('',#59681);
#19170=VERTEX_POINT('',#59684);
#19171=VERTEX_POINT('',#59685);
#19172=VERTEX_POINT('',#59687);
#19173=VERTEX_POINT('',#59689);
#19174=VERTEX_POINT('',#59691);
#19175=VERTEX_POINT('',#59693);
#19176=VERTEX_POINT('',#59696);
#19177=VERTEX_POINT('',#59697);
#19178=VERTEX_POINT('',#59699);
#19179=VERTEX_POINT('',#59701);
#19180=VERTEX_POINT('',#59703);
#19181=VERTEX_POINT('',#59705);
#19182=VERTEX_POINT('',#59708);
#19183=VERTEX_POINT('',#59709);
#19184=VERTEX_POINT('',#59711);
#19185=VERTEX_POINT('',#59713);
#19186=VERTEX_POINT('',#59715);
#19187=VERTEX_POINT('',#59717);
#19188=VERTEX_POINT('',#59720);
#19189=VERTEX_POINT('',#59721);
#19190=VERTEX_POINT('',#59723);
#19191=VERTEX_POINT('',#59725);
#19192=VERTEX_POINT('',#59727);
#19193=VERTEX_POINT('',#59729);
#19194=VERTEX_POINT('',#59732);
#19195=VERTEX_POINT('',#59733);
#19196=VERTEX_POINT('',#59735);
#19197=VERTEX_POINT('',#59737);
#19198=VERTEX_POINT('',#59739);
#19199=VERTEX_POINT('',#59741);
#19200=VERTEX_POINT('',#59744);
#19201=VERTEX_POINT('',#59745);
#19202=VERTEX_POINT('',#59747);
#19203=VERTEX_POINT('',#59749);
#19204=VERTEX_POINT('',#59751);
#19205=VERTEX_POINT('',#59753);
#19206=VERTEX_POINT('',#59756);
#19207=VERTEX_POINT('',#59757);
#19208=VERTEX_POINT('',#59759);
#19209=VERTEX_POINT('',#59761);
#19210=VERTEX_POINT('',#59763);
#19211=VERTEX_POINT('',#59765);
#19212=VERTEX_POINT('',#59768);
#19213=VERTEX_POINT('',#59769);
#19214=VERTEX_POINT('',#59771);
#19215=VERTEX_POINT('',#59773);
#19216=VERTEX_POINT('',#59775);
#19217=VERTEX_POINT('',#59777);
#19218=VERTEX_POINT('',#59780);
#19219=VERTEX_POINT('',#59781);
#19220=VERTEX_POINT('',#59783);
#19221=VERTEX_POINT('',#59785);
#19222=VERTEX_POINT('',#59787);
#19223=VERTEX_POINT('',#59789);
#19224=VERTEX_POINT('',#59792);
#19225=VERTEX_POINT('',#59793);
#19226=VERTEX_POINT('',#59795);
#19227=VERTEX_POINT('',#59797);
#19228=VERTEX_POINT('',#59799);
#19229=VERTEX_POINT('',#59801);
#19230=VERTEX_POINT('',#59804);
#19231=VERTEX_POINT('',#59805);
#19232=VERTEX_POINT('',#59807);
#19233=VERTEX_POINT('',#59809);
#19234=VERTEX_POINT('',#59811);
#19235=VERTEX_POINT('',#59813);
#19236=VERTEX_POINT('',#59816);
#19237=VERTEX_POINT('',#59817);
#19238=VERTEX_POINT('',#59819);
#19239=VERTEX_POINT('',#59821);
#19240=VERTEX_POINT('',#59823);
#19241=VERTEX_POINT('',#59825);
#19242=VERTEX_POINT('',#59828);
#19243=VERTEX_POINT('',#59829);
#19244=VERTEX_POINT('',#59831);
#19245=VERTEX_POINT('',#59833);
#19246=VERTEX_POINT('',#59835);
#19247=VERTEX_POINT('',#59837);
#19248=VERTEX_POINT('',#59840);
#19249=VERTEX_POINT('',#59841);
#19250=VERTEX_POINT('',#59843);
#19251=VERTEX_POINT('',#59845);
#19252=VERTEX_POINT('',#59847);
#19253=VERTEX_POINT('',#59849);
#19254=VERTEX_POINT('',#59852);
#19255=VERTEX_POINT('',#59853);
#19256=VERTEX_POINT('',#59855);
#19257=VERTEX_POINT('',#59857);
#19258=VERTEX_POINT('',#59859);
#19259=VERTEX_POINT('',#59861);
#19260=VERTEX_POINT('',#59864);
#19261=VERTEX_POINT('',#59865);
#19262=VERTEX_POINT('',#59867);
#19263=VERTEX_POINT('',#59869);
#19264=VERTEX_POINT('',#59871);
#19265=VERTEX_POINT('',#59873);
#19266=VERTEX_POINT('',#59876);
#19267=VERTEX_POINT('',#59877);
#19268=VERTEX_POINT('',#59879);
#19269=VERTEX_POINT('',#59881);
#19270=VERTEX_POINT('',#59883);
#19271=VERTEX_POINT('',#59885);
#19272=VERTEX_POINT('',#59888);
#19273=VERTEX_POINT('',#59889);
#19274=VERTEX_POINT('',#59891);
#19275=VERTEX_POINT('',#59893);
#19276=VERTEX_POINT('',#59895);
#19277=VERTEX_POINT('',#59897);
#19278=VERTEX_POINT('',#59900);
#19279=VERTEX_POINT('',#59901);
#19280=VERTEX_POINT('',#59903);
#19281=VERTEX_POINT('',#59905);
#19282=VERTEX_POINT('',#59907);
#19283=VERTEX_POINT('',#59909);
#19284=VERTEX_POINT('',#59912);
#19285=VERTEX_POINT('',#59913);
#19286=VERTEX_POINT('',#59915);
#19287=VERTEX_POINT('',#59917);
#19288=VERTEX_POINT('',#59919);
#19289=VERTEX_POINT('',#59921);
#19290=VERTEX_POINT('',#59924);
#19291=VERTEX_POINT('',#59925);
#19292=VERTEX_POINT('',#59927);
#19293=VERTEX_POINT('',#59929);
#19294=VERTEX_POINT('',#59931);
#19295=VERTEX_POINT('',#59933);
#19296=VERTEX_POINT('',#59936);
#19297=VERTEX_POINT('',#59937);
#19298=VERTEX_POINT('',#59939);
#19299=VERTEX_POINT('',#59941);
#19300=VERTEX_POINT('',#59943);
#19301=VERTEX_POINT('',#59945);
#19302=VERTEX_POINT('',#59948);
#19303=VERTEX_POINT('',#59949);
#19304=VERTEX_POINT('',#59951);
#19305=VERTEX_POINT('',#59953);
#19306=VERTEX_POINT('',#59955);
#19307=VERTEX_POINT('',#59957);
#19308=VERTEX_POINT('',#59960);
#19309=VERTEX_POINT('',#59961);
#19310=VERTEX_POINT('',#59963);
#19311=VERTEX_POINT('',#59965);
#19312=VERTEX_POINT('',#59967);
#19313=VERTEX_POINT('',#59969);
#19314=VERTEX_POINT('',#59972);
#19315=VERTEX_POINT('',#59973);
#19316=VERTEX_POINT('',#59975);
#19317=VERTEX_POINT('',#59977);
#19318=VERTEX_POINT('',#59979);
#19319=VERTEX_POINT('',#59981);
#19320=VERTEX_POINT('',#59984);
#19321=VERTEX_POINT('',#59985);
#19322=VERTEX_POINT('',#59987);
#19323=VERTEX_POINT('',#59989);
#19324=VERTEX_POINT('',#59991);
#19325=VERTEX_POINT('',#59993);
#19326=VERTEX_POINT('',#59996);
#19327=VERTEX_POINT('',#59997);
#19328=VERTEX_POINT('',#59999);
#19329=VERTEX_POINT('',#60001);
#19330=VERTEX_POINT('',#60003);
#19331=VERTEX_POINT('',#60005);
#19332=VERTEX_POINT('',#60008);
#19333=VERTEX_POINT('',#60009);
#19334=VERTEX_POINT('',#60011);
#19335=VERTEX_POINT('',#60013);
#19336=VERTEX_POINT('',#60015);
#19337=VERTEX_POINT('',#60017);
#19338=VERTEX_POINT('',#60020);
#19339=VERTEX_POINT('',#60021);
#19340=VERTEX_POINT('',#60023);
#19341=VERTEX_POINT('',#60025);
#19342=VERTEX_POINT('',#60027);
#19343=VERTEX_POINT('',#60029);
#19344=VERTEX_POINT('',#60032);
#19345=VERTEX_POINT('',#60033);
#19346=VERTEX_POINT('',#60035);
#19347=VERTEX_POINT('',#60037);
#19348=VERTEX_POINT('',#60039);
#19349=VERTEX_POINT('',#60041);
#19350=VERTEX_POINT('',#60044);
#19351=VERTEX_POINT('',#60045);
#19352=VERTEX_POINT('',#60047);
#19353=VERTEX_POINT('',#60049);
#19354=VERTEX_POINT('',#60051);
#19355=VERTEX_POINT('',#60053);
#19356=VERTEX_POINT('',#60056);
#19357=VERTEX_POINT('',#60057);
#19358=VERTEX_POINT('',#60059);
#19359=VERTEX_POINT('',#60061);
#19360=VERTEX_POINT('',#60063);
#19361=VERTEX_POINT('',#60065);
#19362=VERTEX_POINT('',#60068);
#19363=VERTEX_POINT('',#60069);
#19364=VERTEX_POINT('',#60071);
#19365=VERTEX_POINT('',#60073);
#19366=VERTEX_POINT('',#60075);
#19367=VERTEX_POINT('',#60077);
#19368=VERTEX_POINT('',#60080);
#19369=VERTEX_POINT('',#60081);
#19370=VERTEX_POINT('',#60083);
#19371=VERTEX_POINT('',#60085);
#19372=VERTEX_POINT('',#60087);
#19373=VERTEX_POINT('',#60089);
#19374=VERTEX_POINT('',#60092);
#19375=VERTEX_POINT('',#60093);
#19376=VERTEX_POINT('',#60095);
#19377=VERTEX_POINT('',#60097);
#19378=VERTEX_POINT('',#60099);
#19379=VERTEX_POINT('',#60101);
#19380=VERTEX_POINT('',#60104);
#19381=VERTEX_POINT('',#60105);
#19382=VERTEX_POINT('',#60107);
#19383=VERTEX_POINT('',#60109);
#19384=VERTEX_POINT('',#60111);
#19385=VERTEX_POINT('',#60113);
#19386=VERTEX_POINT('',#60116);
#19387=VERTEX_POINT('',#60117);
#19388=VERTEX_POINT('',#60119);
#19389=VERTEX_POINT('',#60121);
#19390=VERTEX_POINT('',#60123);
#19391=VERTEX_POINT('',#60125);
#19392=VERTEX_POINT('',#60128);
#19393=VERTEX_POINT('',#60129);
#19394=VERTEX_POINT('',#60131);
#19395=VERTEX_POINT('',#60133);
#19396=VERTEX_POINT('',#60135);
#19397=VERTEX_POINT('',#60137);
#19398=VERTEX_POINT('',#60140);
#19399=VERTEX_POINT('',#60141);
#19400=VERTEX_POINT('',#60143);
#19401=VERTEX_POINT('',#60145);
#19402=VERTEX_POINT('',#60147);
#19403=VERTEX_POINT('',#60149);
#19404=VERTEX_POINT('',#60152);
#19405=VERTEX_POINT('',#60153);
#19406=VERTEX_POINT('',#60155);
#19407=VERTEX_POINT('',#60157);
#19408=VERTEX_POINT('',#60159);
#19409=VERTEX_POINT('',#60161);
#19410=VERTEX_POINT('',#60164);
#19411=VERTEX_POINT('',#60165);
#19412=VERTEX_POINT('',#60167);
#19413=VERTEX_POINT('',#60169);
#19414=VERTEX_POINT('',#60171);
#19415=VERTEX_POINT('',#60173);
#19416=VERTEX_POINT('',#60176);
#19417=VERTEX_POINT('',#60177);
#19418=VERTEX_POINT('',#60179);
#19419=VERTEX_POINT('',#60181);
#19420=VERTEX_POINT('',#60183);
#19421=VERTEX_POINT('',#60185);
#19422=VERTEX_POINT('',#60188);
#19423=VERTEX_POINT('',#60189);
#19424=VERTEX_POINT('',#60191);
#19425=VERTEX_POINT('',#60193);
#19426=VERTEX_POINT('',#60195);
#19427=VERTEX_POINT('',#60197);
#19428=VERTEX_POINT('',#60200);
#19429=VERTEX_POINT('',#60201);
#19430=VERTEX_POINT('',#60203);
#19431=VERTEX_POINT('',#60205);
#19432=VERTEX_POINT('',#60207);
#19433=VERTEX_POINT('',#60209);
#19434=VERTEX_POINT('',#60212);
#19435=VERTEX_POINT('',#60213);
#19436=VERTEX_POINT('',#60215);
#19437=VERTEX_POINT('',#60217);
#19438=VERTEX_POINT('',#60219);
#19439=VERTEX_POINT('',#60221);
#19440=VERTEX_POINT('',#60224);
#19441=VERTEX_POINT('',#60225);
#19442=VERTEX_POINT('',#60227);
#19443=VERTEX_POINT('',#60229);
#19444=VERTEX_POINT('',#60231);
#19445=VERTEX_POINT('',#60233);
#19446=VERTEX_POINT('',#60236);
#19447=VERTEX_POINT('',#60237);
#19448=VERTEX_POINT('',#60239);
#19449=VERTEX_POINT('',#60241);
#19450=VERTEX_POINT('',#60243);
#19451=VERTEX_POINT('',#60245);
#19452=VERTEX_POINT('',#60248);
#19453=VERTEX_POINT('',#60249);
#19454=VERTEX_POINT('',#60251);
#19455=VERTEX_POINT('',#60253);
#19456=VERTEX_POINT('',#60255);
#19457=VERTEX_POINT('',#60257);
#19458=VERTEX_POINT('',#60260);
#19459=VERTEX_POINT('',#60261);
#19460=VERTEX_POINT('',#60263);
#19461=VERTEX_POINT('',#60265);
#19462=VERTEX_POINT('',#60267);
#19463=VERTEX_POINT('',#60269);
#19464=VERTEX_POINT('',#60272);
#19465=VERTEX_POINT('',#60273);
#19466=VERTEX_POINT('',#60275);
#19467=VERTEX_POINT('',#60277);
#19468=VERTEX_POINT('',#60279);
#19469=VERTEX_POINT('',#60281);
#19470=VERTEX_POINT('',#60284);
#19471=VERTEX_POINT('',#60285);
#19472=VERTEX_POINT('',#60287);
#19473=VERTEX_POINT('',#60289);
#19474=VERTEX_POINT('',#60291);
#19475=VERTEX_POINT('',#60293);
#19476=VERTEX_POINT('',#60296);
#19477=VERTEX_POINT('',#60297);
#19478=VERTEX_POINT('',#60299);
#19479=VERTEX_POINT('',#60301);
#19480=VERTEX_POINT('',#60303);
#19481=VERTEX_POINT('',#60305);
#19482=VERTEX_POINT('',#60308);
#19483=VERTEX_POINT('',#60309);
#19484=VERTEX_POINT('',#60311);
#19485=VERTEX_POINT('',#60313);
#19486=VERTEX_POINT('',#60315);
#19487=VERTEX_POINT('',#60317);
#19488=VERTEX_POINT('',#60320);
#19489=VERTEX_POINT('',#60321);
#19490=VERTEX_POINT('',#60323);
#19491=VERTEX_POINT('',#60325);
#19492=VERTEX_POINT('',#60327);
#19493=VERTEX_POINT('',#60329);
#19494=VERTEX_POINT('',#60332);
#19495=VERTEX_POINT('',#60333);
#19496=VERTEX_POINT('',#60335);
#19497=VERTEX_POINT('',#60337);
#19498=VERTEX_POINT('',#60339);
#19499=VERTEX_POINT('',#60341);
#19500=VERTEX_POINT('',#60344);
#19501=VERTEX_POINT('',#60345);
#19502=VERTEX_POINT('',#60347);
#19503=VERTEX_POINT('',#60349);
#19504=VERTEX_POINT('',#60351);
#19505=VERTEX_POINT('',#60353);
#19506=VERTEX_POINT('',#60356);
#19507=VERTEX_POINT('',#60357);
#19508=VERTEX_POINT('',#60359);
#19509=VERTEX_POINT('',#60361);
#19510=VERTEX_POINT('',#60363);
#19511=VERTEX_POINT('',#60365);
#19512=VERTEX_POINT('',#60368);
#19513=VERTEX_POINT('',#60369);
#19514=VERTEX_POINT('',#60371);
#19515=VERTEX_POINT('',#60373);
#19516=VERTEX_POINT('',#60375);
#19517=VERTEX_POINT('',#60377);
#19518=VERTEX_POINT('',#60380);
#19519=VERTEX_POINT('',#60381);
#19520=VERTEX_POINT('',#60383);
#19521=VERTEX_POINT('',#60385);
#19522=VERTEX_POINT('',#60387);
#19523=VERTEX_POINT('',#60389);
#19524=VERTEX_POINT('',#60392);
#19525=VERTEX_POINT('',#60393);
#19526=VERTEX_POINT('',#60395);
#19527=VERTEX_POINT('',#60397);
#19528=VERTEX_POINT('',#60399);
#19529=VERTEX_POINT('',#60401);
#19530=VERTEX_POINT('',#60404);
#19531=VERTEX_POINT('',#60405);
#19532=VERTEX_POINT('',#60407);
#19533=VERTEX_POINT('',#60409);
#19534=VERTEX_POINT('',#60411);
#19535=VERTEX_POINT('',#60413);
#19536=VERTEX_POINT('',#60416);
#19537=VERTEX_POINT('',#60417);
#19538=VERTEX_POINT('',#60419);
#19539=VERTEX_POINT('',#60421);
#19540=VERTEX_POINT('',#60423);
#19541=VERTEX_POINT('',#60425);
#19542=VERTEX_POINT('',#60428);
#19543=VERTEX_POINT('',#60429);
#19544=VERTEX_POINT('',#60431);
#19545=VERTEX_POINT('',#60433);
#19546=VERTEX_POINT('',#60435);
#19547=VERTEX_POINT('',#60437);
#19548=VERTEX_POINT('',#60440);
#19549=VERTEX_POINT('',#60441);
#19550=VERTEX_POINT('',#60443);
#19551=VERTEX_POINT('',#60445);
#19552=VERTEX_POINT('',#60447);
#19553=VERTEX_POINT('',#60449);
#19554=VERTEX_POINT('',#60452);
#19555=VERTEX_POINT('',#60453);
#19556=VERTEX_POINT('',#60455);
#19557=VERTEX_POINT('',#60457);
#19558=VERTEX_POINT('',#60459);
#19559=VERTEX_POINT('',#60461);
#19560=VERTEX_POINT('',#60464);
#19561=VERTEX_POINT('',#60465);
#19562=VERTEX_POINT('',#60467);
#19563=VERTEX_POINT('',#60469);
#19564=VERTEX_POINT('',#60471);
#19565=VERTEX_POINT('',#60473);
#19566=VERTEX_POINT('',#60476);
#19567=VERTEX_POINT('',#60477);
#19568=VERTEX_POINT('',#60479);
#19569=VERTEX_POINT('',#60481);
#19570=VERTEX_POINT('',#60483);
#19571=VERTEX_POINT('',#60485);
#19572=VERTEX_POINT('',#60488);
#19573=VERTEX_POINT('',#60489);
#19574=VERTEX_POINT('',#60491);
#19575=VERTEX_POINT('',#60493);
#19576=VERTEX_POINT('',#60495);
#19577=VERTEX_POINT('',#60497);
#19578=VERTEX_POINT('',#60500);
#19579=VERTEX_POINT('',#60501);
#19580=VERTEX_POINT('',#60503);
#19581=VERTEX_POINT('',#60505);
#19582=VERTEX_POINT('',#60507);
#19583=VERTEX_POINT('',#60509);
#19584=VERTEX_POINT('',#60512);
#19585=VERTEX_POINT('',#60513);
#19586=VERTEX_POINT('',#60515);
#19587=VERTEX_POINT('',#60517);
#19588=VERTEX_POINT('',#60519);
#19589=VERTEX_POINT('',#60521);
#19590=VERTEX_POINT('',#60524);
#19591=VERTEX_POINT('',#60525);
#19592=VERTEX_POINT('',#60527);
#19593=VERTEX_POINT('',#60529);
#19594=VERTEX_POINT('',#60531);
#19595=VERTEX_POINT('',#60533);
#19596=VERTEX_POINT('',#60536);
#19597=VERTEX_POINT('',#60537);
#19598=VERTEX_POINT('',#60539);
#19599=VERTEX_POINT('',#60541);
#19600=VERTEX_POINT('',#60543);
#19601=VERTEX_POINT('',#60545);
#19602=VERTEX_POINT('',#60548);
#19603=VERTEX_POINT('',#60549);
#19604=VERTEX_POINT('',#60551);
#19605=VERTEX_POINT('',#60553);
#19606=VERTEX_POINT('',#60555);
#19607=VERTEX_POINT('',#60557);
#19608=VERTEX_POINT('',#60560);
#19609=VERTEX_POINT('',#60561);
#19610=VERTEX_POINT('',#60563);
#19611=VERTEX_POINT('',#60565);
#19612=VERTEX_POINT('',#60567);
#19613=VERTEX_POINT('',#60569);
#19614=VERTEX_POINT('',#60572);
#19615=VERTEX_POINT('',#60573);
#19616=VERTEX_POINT('',#60575);
#19617=VERTEX_POINT('',#60577);
#19618=VERTEX_POINT('',#60579);
#19619=VERTEX_POINT('',#60581);
#19620=VERTEX_POINT('',#60584);
#19621=VERTEX_POINT('',#60585);
#19622=VERTEX_POINT('',#60587);
#19623=VERTEX_POINT('',#60589);
#19624=VERTEX_POINT('',#60591);
#19625=VERTEX_POINT('',#60593);
#19626=VERTEX_POINT('',#60596);
#19627=VERTEX_POINT('',#60597);
#19628=VERTEX_POINT('',#60599);
#19629=VERTEX_POINT('',#60601);
#19630=VERTEX_POINT('',#60603);
#19631=VERTEX_POINT('',#60605);
#19632=VERTEX_POINT('',#60608);
#19633=VERTEX_POINT('',#60609);
#19634=VERTEX_POINT('',#60611);
#19635=VERTEX_POINT('',#60613);
#19636=VERTEX_POINT('',#60615);
#19637=VERTEX_POINT('',#60617);
#19638=VERTEX_POINT('',#60620);
#19639=VERTEX_POINT('',#60621);
#19640=VERTEX_POINT('',#60623);
#19641=VERTEX_POINT('',#60625);
#19642=VERTEX_POINT('',#60627);
#19643=VERTEX_POINT('',#60629);
#19644=VERTEX_POINT('',#60632);
#19645=VERTEX_POINT('',#60633);
#19646=VERTEX_POINT('',#60635);
#19647=VERTEX_POINT('',#60637);
#19648=VERTEX_POINT('',#60639);
#19649=VERTEX_POINT('',#60641);
#19650=VERTEX_POINT('',#60644);
#19651=VERTEX_POINT('',#60645);
#19652=VERTEX_POINT('',#60647);
#19653=VERTEX_POINT('',#60649);
#19654=VERTEX_POINT('',#60651);
#19655=VERTEX_POINT('',#60653);
#19656=VERTEX_POINT('',#60656);
#19657=VERTEX_POINT('',#60657);
#19658=VERTEX_POINT('',#60659);
#19659=VERTEX_POINT('',#60661);
#19660=VERTEX_POINT('',#60663);
#19661=VERTEX_POINT('',#60665);
#19662=VERTEX_POINT('',#60668);
#19663=VERTEX_POINT('',#60669);
#19664=VERTEX_POINT('',#60671);
#19665=VERTEX_POINT('',#60673);
#19666=VERTEX_POINT('',#60675);
#19667=VERTEX_POINT('',#60677);
#19668=VERTEX_POINT('',#60680);
#19669=VERTEX_POINT('',#60681);
#19670=VERTEX_POINT('',#60683);
#19671=VERTEX_POINT('',#60685);
#19672=VERTEX_POINT('',#60687);
#19673=VERTEX_POINT('',#60689);
#19674=VERTEX_POINT('',#60692);
#19675=VERTEX_POINT('',#60693);
#19676=VERTEX_POINT('',#60695);
#19677=VERTEX_POINT('',#60697);
#19678=VERTEX_POINT('',#60699);
#19679=VERTEX_POINT('',#60701);
#19680=VERTEX_POINT('',#60704);
#19681=VERTEX_POINT('',#60705);
#19682=VERTEX_POINT('',#60707);
#19683=VERTEX_POINT('',#60709);
#19684=VERTEX_POINT('',#60711);
#19685=VERTEX_POINT('',#60713);
#19686=VERTEX_POINT('',#60716);
#19687=VERTEX_POINT('',#60717);
#19688=VERTEX_POINT('',#60719);
#19689=VERTEX_POINT('',#60721);
#19690=VERTEX_POINT('',#60723);
#19691=VERTEX_POINT('',#60725);
#19692=VERTEX_POINT('',#60728);
#19693=VERTEX_POINT('',#60729);
#19694=VERTEX_POINT('',#60731);
#19695=VERTEX_POINT('',#60733);
#19696=VERTEX_POINT('',#60735);
#19697=VERTEX_POINT('',#60737);
#19698=VERTEX_POINT('',#60740);
#19699=VERTEX_POINT('',#60741);
#19700=VERTEX_POINT('',#60743);
#19701=VERTEX_POINT('',#60745);
#19702=VERTEX_POINT('',#60747);
#19703=VERTEX_POINT('',#60749);
#19704=VERTEX_POINT('',#60752);
#19705=VERTEX_POINT('',#60753);
#19706=VERTEX_POINT('',#60755);
#19707=VERTEX_POINT('',#60757);
#19708=VERTEX_POINT('',#60759);
#19709=VERTEX_POINT('',#60761);
#19710=VERTEX_POINT('',#60764);
#19711=VERTEX_POINT('',#60765);
#19712=VERTEX_POINT('',#60767);
#19713=VERTEX_POINT('',#60769);
#19714=VERTEX_POINT('',#60771);
#19715=VERTEX_POINT('',#60773);
#19716=VERTEX_POINT('',#60776);
#19717=VERTEX_POINT('',#60777);
#19718=VERTEX_POINT('',#60779);
#19719=VERTEX_POINT('',#60781);
#19720=VERTEX_POINT('',#60783);
#19721=VERTEX_POINT('',#60785);
#19722=VERTEX_POINT('',#60788);
#19723=VERTEX_POINT('',#60789);
#19724=VERTEX_POINT('',#60791);
#19725=VERTEX_POINT('',#60793);
#19726=VERTEX_POINT('',#60795);
#19727=VERTEX_POINT('',#60797);
#19728=VERTEX_POINT('',#60800);
#19729=VERTEX_POINT('',#60801);
#19730=VERTEX_POINT('',#60803);
#19731=VERTEX_POINT('',#60805);
#19732=VERTEX_POINT('',#60807);
#19733=VERTEX_POINT('',#60809);
#19734=VERTEX_POINT('',#60812);
#19735=VERTEX_POINT('',#60813);
#19736=VERTEX_POINT('',#60815);
#19737=VERTEX_POINT('',#60817);
#19738=VERTEX_POINT('',#60819);
#19739=VERTEX_POINT('',#60821);
#19740=VERTEX_POINT('',#60825);
#19741=VERTEX_POINT('',#60826);
#19742=VERTEX_POINT('',#60828);
#19743=VERTEX_POINT('',#60830);
#19744=VERTEX_POINT('',#60832);
#19745=VERTEX_POINT('',#60834);
#19746=VERTEX_POINT('',#60837);
#19747=VERTEX_POINT('',#60838);
#19748=VERTEX_POINT('',#60840);
#19749=VERTEX_POINT('',#60842);
#19750=VERTEX_POINT('',#60844);
#19751=VERTEX_POINT('',#60846);
#19752=VERTEX_POINT('',#60849);
#19753=VERTEX_POINT('',#60850);
#19754=VERTEX_POINT('',#60852);
#19755=VERTEX_POINT('',#60854);
#19756=VERTEX_POINT('',#60856);
#19757=VERTEX_POINT('',#60858);
#19758=VERTEX_POINT('',#60861);
#19759=VERTEX_POINT('',#60862);
#19760=VERTEX_POINT('',#60864);
#19761=VERTEX_POINT('',#60866);
#19762=VERTEX_POINT('',#60868);
#19763=VERTEX_POINT('',#60870);
#19764=VERTEX_POINT('',#60873);
#19765=VERTEX_POINT('',#60874);
#19766=VERTEX_POINT('',#60876);
#19767=VERTEX_POINT('',#60878);
#19768=VERTEX_POINT('',#60880);
#19769=VERTEX_POINT('',#60882);
#19770=VERTEX_POINT('',#60885);
#19771=VERTEX_POINT('',#60886);
#19772=VERTEX_POINT('',#60888);
#19773=VERTEX_POINT('',#60890);
#19774=VERTEX_POINT('',#60892);
#19775=VERTEX_POINT('',#60894);
#19776=VERTEX_POINT('',#60897);
#19777=VERTEX_POINT('',#60898);
#19778=VERTEX_POINT('',#60900);
#19779=VERTEX_POINT('',#60902);
#19780=VERTEX_POINT('',#60904);
#19781=VERTEX_POINT('',#60906);
#19782=VERTEX_POINT('',#60909);
#19783=VERTEX_POINT('',#60910);
#19784=VERTEX_POINT('',#60912);
#19785=VERTEX_POINT('',#60914);
#19786=VERTEX_POINT('',#60916);
#19787=VERTEX_POINT('',#60918);
#19788=VERTEX_POINT('',#60921);
#19789=VERTEX_POINT('',#60922);
#19790=VERTEX_POINT('',#60924);
#19791=VERTEX_POINT('',#60926);
#19792=VERTEX_POINT('',#60928);
#19793=VERTEX_POINT('',#60930);
#19794=VERTEX_POINT('',#60933);
#19795=VERTEX_POINT('',#60934);
#19796=VERTEX_POINT('',#60936);
#19797=VERTEX_POINT('',#60938);
#19798=VERTEX_POINT('',#60940);
#19799=VERTEX_POINT('',#60942);
#19800=VERTEX_POINT('',#60945);
#19801=VERTEX_POINT('',#60946);
#19802=VERTEX_POINT('',#60948);
#19803=VERTEX_POINT('',#60950);
#19804=VERTEX_POINT('',#60952);
#19805=VERTEX_POINT('',#60954);
#19806=VERTEX_POINT('',#60957);
#19807=VERTEX_POINT('',#60958);
#19808=VERTEX_POINT('',#60960);
#19809=VERTEX_POINT('',#60962);
#19810=VERTEX_POINT('',#60964);
#19811=VERTEX_POINT('',#60966);
#19812=VERTEX_POINT('',#60969);
#19813=VERTEX_POINT('',#60970);
#19814=VERTEX_POINT('',#60972);
#19815=VERTEX_POINT('',#60974);
#19816=VERTEX_POINT('',#60976);
#19817=VERTEX_POINT('',#60978);
#19818=VERTEX_POINT('',#60981);
#19819=VERTEX_POINT('',#60982);
#19820=VERTEX_POINT('',#60984);
#19821=VERTEX_POINT('',#60986);
#19822=VERTEX_POINT('',#60988);
#19823=VERTEX_POINT('',#60990);
#19824=VERTEX_POINT('',#60993);
#19825=VERTEX_POINT('',#60994);
#19826=VERTEX_POINT('',#60996);
#19827=VERTEX_POINT('',#60998);
#19828=VERTEX_POINT('',#61000);
#19829=VERTEX_POINT('',#61002);
#19830=VERTEX_POINT('',#61005);
#19831=VERTEX_POINT('',#61006);
#19832=VERTEX_POINT('',#61008);
#19833=VERTEX_POINT('',#61010);
#19834=VERTEX_POINT('',#61012);
#19835=VERTEX_POINT('',#61014);
#19836=VERTEX_POINT('',#61017);
#19837=VERTEX_POINT('',#61018);
#19838=VERTEX_POINT('',#61020);
#19839=VERTEX_POINT('',#61022);
#19840=VERTEX_POINT('',#61024);
#19841=VERTEX_POINT('',#61026);
#19842=VERTEX_POINT('',#61029);
#19843=VERTEX_POINT('',#61030);
#19844=VERTEX_POINT('',#61032);
#19845=VERTEX_POINT('',#61034);
#19846=VERTEX_POINT('',#61036);
#19847=VERTEX_POINT('',#61038);
#19848=VERTEX_POINT('',#61041);
#19849=VERTEX_POINT('',#61042);
#19850=VERTEX_POINT('',#61044);
#19851=VERTEX_POINT('',#61046);
#19852=VERTEX_POINT('',#61048);
#19853=VERTEX_POINT('',#61050);
#19854=VERTEX_POINT('',#61053);
#19855=VERTEX_POINT('',#61054);
#19856=VERTEX_POINT('',#61056);
#19857=VERTEX_POINT('',#61058);
#19858=VERTEX_POINT('',#61060);
#19859=VERTEX_POINT('',#61062);
#19860=VERTEX_POINT('',#61065);
#19861=VERTEX_POINT('',#61066);
#19862=VERTEX_POINT('',#61068);
#19863=VERTEX_POINT('',#61070);
#19864=VERTEX_POINT('',#61072);
#19865=VERTEX_POINT('',#61074);
#19866=VERTEX_POINT('',#61077);
#19867=VERTEX_POINT('',#61078);
#19868=VERTEX_POINT('',#61080);
#19869=VERTEX_POINT('',#61082);
#19870=VERTEX_POINT('',#61084);
#19871=VERTEX_POINT('',#61086);
#19872=VERTEX_POINT('',#61089);
#19873=VERTEX_POINT('',#61090);
#19874=VERTEX_POINT('',#61092);
#19875=VERTEX_POINT('',#61094);
#19876=VERTEX_POINT('',#61096);
#19877=VERTEX_POINT('',#61098);
#19878=VERTEX_POINT('',#61101);
#19879=VERTEX_POINT('',#61102);
#19880=VERTEX_POINT('',#61104);
#19881=VERTEX_POINT('',#61106);
#19882=VERTEX_POINT('',#61108);
#19883=VERTEX_POINT('',#61110);
#19884=VERTEX_POINT('',#61113);
#19885=VERTEX_POINT('',#61114);
#19886=VERTEX_POINT('',#61116);
#19887=VERTEX_POINT('',#61118);
#19888=VERTEX_POINT('',#61120);
#19889=VERTEX_POINT('',#61122);
#19890=VERTEX_POINT('',#61125);
#19891=VERTEX_POINT('',#61126);
#19892=VERTEX_POINT('',#61128);
#19893=VERTEX_POINT('',#61130);
#19894=VERTEX_POINT('',#61132);
#19895=VERTEX_POINT('',#61134);
#19896=VERTEX_POINT('',#61137);
#19897=VERTEX_POINT('',#61138);
#19898=VERTEX_POINT('',#61140);
#19899=VERTEX_POINT('',#61142);
#19900=VERTEX_POINT('',#61144);
#19901=VERTEX_POINT('',#61146);
#19902=VERTEX_POINT('',#61149);
#19903=VERTEX_POINT('',#61150);
#19904=VERTEX_POINT('',#61152);
#19905=VERTEX_POINT('',#61154);
#19906=VERTEX_POINT('',#61156);
#19907=VERTEX_POINT('',#61158);
#19908=VERTEX_POINT('',#61161);
#19909=VERTEX_POINT('',#61162);
#19910=VERTEX_POINT('',#61164);
#19911=VERTEX_POINT('',#61166);
#19912=VERTEX_POINT('',#61168);
#19913=VERTEX_POINT('',#61170);
#19914=VERTEX_POINT('',#61173);
#19915=VERTEX_POINT('',#61174);
#19916=VERTEX_POINT('',#61176);
#19917=VERTEX_POINT('',#61178);
#19918=VERTEX_POINT('',#61180);
#19919=VERTEX_POINT('',#61182);
#19920=VERTEX_POINT('',#61185);
#19921=VERTEX_POINT('',#61186);
#19922=VERTEX_POINT('',#61188);
#19923=VERTEX_POINT('',#61190);
#19924=VERTEX_POINT('',#61192);
#19925=VERTEX_POINT('',#61194);
#19926=VERTEX_POINT('',#61197);
#19927=VERTEX_POINT('',#61198);
#19928=VERTEX_POINT('',#61200);
#19929=VERTEX_POINT('',#61202);
#19930=VERTEX_POINT('',#61204);
#19931=VERTEX_POINT('',#61206);
#19932=VERTEX_POINT('',#61209);
#19933=VERTEX_POINT('',#61210);
#19934=VERTEX_POINT('',#61212);
#19935=VERTEX_POINT('',#61214);
#19936=VERTEX_POINT('',#61216);
#19937=VERTEX_POINT('',#61218);
#19938=VERTEX_POINT('',#61221);
#19939=VERTEX_POINT('',#61222);
#19940=VERTEX_POINT('',#61224);
#19941=VERTEX_POINT('',#61226);
#19942=VERTEX_POINT('',#61228);
#19943=VERTEX_POINT('',#61230);
#19944=VERTEX_POINT('',#61233);
#19945=VERTEX_POINT('',#61234);
#19946=VERTEX_POINT('',#61236);
#19947=VERTEX_POINT('',#61238);
#19948=VERTEX_POINT('',#61240);
#19949=VERTEX_POINT('',#61242);
#19950=VERTEX_POINT('',#61245);
#19951=VERTEX_POINT('',#61246);
#19952=VERTEX_POINT('',#61248);
#19953=VERTEX_POINT('',#61250);
#19954=VERTEX_POINT('',#61252);
#19955=VERTEX_POINT('',#61254);
#19956=VERTEX_POINT('',#61257);
#19957=VERTEX_POINT('',#61258);
#19958=VERTEX_POINT('',#61260);
#19959=VERTEX_POINT('',#61262);
#19960=VERTEX_POINT('',#61264);
#19961=VERTEX_POINT('',#61266);
#19962=VERTEX_POINT('',#61269);
#19963=VERTEX_POINT('',#61270);
#19964=VERTEX_POINT('',#61272);
#19965=VERTEX_POINT('',#61274);
#19966=VERTEX_POINT('',#61276);
#19967=VERTEX_POINT('',#61278);
#19968=VERTEX_POINT('',#61281);
#19969=VERTEX_POINT('',#61282);
#19970=VERTEX_POINT('',#61284);
#19971=VERTEX_POINT('',#61286);
#19972=VERTEX_POINT('',#61288);
#19973=VERTEX_POINT('',#61290);
#19974=VERTEX_POINT('',#61293);
#19975=VERTEX_POINT('',#61294);
#19976=VERTEX_POINT('',#61296);
#19977=VERTEX_POINT('',#61298);
#19978=VERTEX_POINT('',#61300);
#19979=VERTEX_POINT('',#61302);
#19980=VERTEX_POINT('',#61305);
#19981=VERTEX_POINT('',#61306);
#19982=VERTEX_POINT('',#61308);
#19983=VERTEX_POINT('',#61310);
#19984=VERTEX_POINT('',#61312);
#19985=VERTEX_POINT('',#61314);
#19986=VERTEX_POINT('',#61317);
#19987=VERTEX_POINT('',#61318);
#19988=VERTEX_POINT('',#61320);
#19989=VERTEX_POINT('',#61322);
#19990=VERTEX_POINT('',#61324);
#19991=VERTEX_POINT('',#61326);
#19992=VERTEX_POINT('',#61329);
#19993=VERTEX_POINT('',#61330);
#19994=VERTEX_POINT('',#61332);
#19995=VERTEX_POINT('',#61334);
#19996=VERTEX_POINT('',#61336);
#19997=VERTEX_POINT('',#61338);
#19998=VERTEX_POINT('',#61341);
#19999=VERTEX_POINT('',#61342);
#20000=VERTEX_POINT('',#61344);
#20001=VERTEX_POINT('',#61346);
#20002=VERTEX_POINT('',#61348);
#20003=VERTEX_POINT('',#61350);
#20004=VERTEX_POINT('',#61353);
#20005=VERTEX_POINT('',#61354);
#20006=VERTEX_POINT('',#61356);
#20007=VERTEX_POINT('',#61358);
#20008=VERTEX_POINT('',#61360);
#20009=VERTEX_POINT('',#61362);
#20010=VERTEX_POINT('',#61365);
#20011=VERTEX_POINT('',#61366);
#20012=VERTEX_POINT('',#61368);
#20013=VERTEX_POINT('',#61370);
#20014=VERTEX_POINT('',#61372);
#20015=VERTEX_POINT('',#61374);
#20016=VERTEX_POINT('',#61377);
#20017=VERTEX_POINT('',#61378);
#20018=VERTEX_POINT('',#61380);
#20019=VERTEX_POINT('',#61382);
#20020=VERTEX_POINT('',#61384);
#20021=VERTEX_POINT('',#61386);
#20022=VERTEX_POINT('',#61389);
#20023=VERTEX_POINT('',#61390);
#20024=VERTEX_POINT('',#61392);
#20025=VERTEX_POINT('',#61394);
#20026=VERTEX_POINT('',#61396);
#20027=VERTEX_POINT('',#61398);
#20028=VERTEX_POINT('',#61401);
#20029=VERTEX_POINT('',#61402);
#20030=VERTEX_POINT('',#61404);
#20031=VERTEX_POINT('',#61406);
#20032=VERTEX_POINT('',#61408);
#20033=VERTEX_POINT('',#61410);
#20034=VERTEX_POINT('',#61413);
#20035=VERTEX_POINT('',#61414);
#20036=VERTEX_POINT('',#61416);
#20037=VERTEX_POINT('',#61418);
#20038=VERTEX_POINT('',#61420);
#20039=VERTEX_POINT('',#61422);
#20040=VERTEX_POINT('',#61425);
#20041=VERTEX_POINT('',#61426);
#20042=VERTEX_POINT('',#61428);
#20043=VERTEX_POINT('',#61430);
#20044=VERTEX_POINT('',#61432);
#20045=VERTEX_POINT('',#61434);
#20046=VERTEX_POINT('',#61437);
#20047=VERTEX_POINT('',#61438);
#20048=VERTEX_POINT('',#61440);
#20049=VERTEX_POINT('',#61442);
#20050=VERTEX_POINT('',#61444);
#20051=VERTEX_POINT('',#61446);
#20052=VERTEX_POINT('',#61449);
#20053=VERTEX_POINT('',#61450);
#20054=VERTEX_POINT('',#61452);
#20055=VERTEX_POINT('',#61454);
#20056=VERTEX_POINT('',#61456);
#20057=VERTEX_POINT('',#61458);
#20058=VERTEX_POINT('',#61461);
#20059=VERTEX_POINT('',#61462);
#20060=VERTEX_POINT('',#61464);
#20061=VERTEX_POINT('',#61466);
#20062=VERTEX_POINT('',#61468);
#20063=VERTEX_POINT('',#61470);
#20064=VERTEX_POINT('',#61473);
#20065=VERTEX_POINT('',#61474);
#20066=VERTEX_POINT('',#61476);
#20067=VERTEX_POINT('',#61478);
#20068=VERTEX_POINT('',#61480);
#20069=VERTEX_POINT('',#61482);
#20070=VERTEX_POINT('',#61485);
#20071=VERTEX_POINT('',#61486);
#20072=VERTEX_POINT('',#61488);
#20073=VERTEX_POINT('',#61490);
#20074=VERTEX_POINT('',#61492);
#20075=VERTEX_POINT('',#61494);
#20076=VERTEX_POINT('',#61497);
#20077=VERTEX_POINT('',#61498);
#20078=VERTEX_POINT('',#61500);
#20079=VERTEX_POINT('',#61502);
#20080=VERTEX_POINT('',#61504);
#20081=VERTEX_POINT('',#61506);
#20082=VERTEX_POINT('',#61509);
#20083=VERTEX_POINT('',#61510);
#20084=VERTEX_POINT('',#61512);
#20085=VERTEX_POINT('',#61514);
#20086=VERTEX_POINT('',#61516);
#20087=VERTEX_POINT('',#61518);
#20088=VERTEX_POINT('',#61521);
#20089=VERTEX_POINT('',#61522);
#20090=VERTEX_POINT('',#61524);
#20091=VERTEX_POINT('',#61526);
#20092=VERTEX_POINT('',#61528);
#20093=VERTEX_POINT('',#61530);
#20094=VERTEX_POINT('',#61533);
#20095=VERTEX_POINT('',#61534);
#20096=VERTEX_POINT('',#61536);
#20097=VERTEX_POINT('',#61538);
#20098=VERTEX_POINT('',#61540);
#20099=VERTEX_POINT('',#61542);
#20100=VERTEX_POINT('',#61545);
#20101=VERTEX_POINT('',#61546);
#20102=VERTEX_POINT('',#61548);
#20103=VERTEX_POINT('',#61550);
#20104=VERTEX_POINT('',#61552);
#20105=VERTEX_POINT('',#61554);
#20106=VERTEX_POINT('',#61557);
#20107=VERTEX_POINT('',#61558);
#20108=VERTEX_POINT('',#61560);
#20109=VERTEX_POINT('',#61562);
#20110=VERTEX_POINT('',#61564);
#20111=VERTEX_POINT('',#61566);
#20112=VERTEX_POINT('',#61569);
#20113=VERTEX_POINT('',#61570);
#20114=VERTEX_POINT('',#61572);
#20115=VERTEX_POINT('',#61574);
#20116=VERTEX_POINT('',#61576);
#20117=VERTEX_POINT('',#61578);
#20118=VERTEX_POINT('',#61581);
#20119=VERTEX_POINT('',#61582);
#20120=VERTEX_POINT('',#61584);
#20121=VERTEX_POINT('',#61586);
#20122=VERTEX_POINT('',#61588);
#20123=VERTEX_POINT('',#61590);
#20124=VERTEX_POINT('',#61593);
#20125=VERTEX_POINT('',#61594);
#20126=VERTEX_POINT('',#61596);
#20127=VERTEX_POINT('',#61598);
#20128=VERTEX_POINT('',#61600);
#20129=VERTEX_POINT('',#61602);
#20130=VERTEX_POINT('',#61605);
#20131=VERTEX_POINT('',#61606);
#20132=VERTEX_POINT('',#61608);
#20133=VERTEX_POINT('',#61610);
#20134=VERTEX_POINT('',#61612);
#20135=VERTEX_POINT('',#61614);
#20136=VERTEX_POINT('',#61617);
#20137=VERTEX_POINT('',#61618);
#20138=VERTEX_POINT('',#61620);
#20139=VERTEX_POINT('',#61622);
#20140=VERTEX_POINT('',#61624);
#20141=VERTEX_POINT('',#61626);
#20142=VERTEX_POINT('',#61629);
#20143=VERTEX_POINT('',#61630);
#20144=VERTEX_POINT('',#61632);
#20145=VERTEX_POINT('',#61634);
#20146=VERTEX_POINT('',#61636);
#20147=VERTEX_POINT('',#61638);
#20148=VERTEX_POINT('',#61641);
#20149=VERTEX_POINT('',#61642);
#20150=VERTEX_POINT('',#61644);
#20151=VERTEX_POINT('',#61646);
#20152=VERTEX_POINT('',#61648);
#20153=VERTEX_POINT('',#61650);
#20154=VERTEX_POINT('',#61653);
#20155=VERTEX_POINT('',#61654);
#20156=VERTEX_POINT('',#61656);
#20157=VERTEX_POINT('',#61658);
#20158=VERTEX_POINT('',#61660);
#20159=VERTEX_POINT('',#61662);
#20160=VERTEX_POINT('',#61665);
#20161=VERTEX_POINT('',#61666);
#20162=VERTEX_POINT('',#61668);
#20163=VERTEX_POINT('',#61670);
#20164=VERTEX_POINT('',#61672);
#20165=VERTEX_POINT('',#61674);
#20166=VERTEX_POINT('',#61677);
#20167=VERTEX_POINT('',#61678);
#20168=VERTEX_POINT('',#61680);
#20169=VERTEX_POINT('',#61682);
#20170=VERTEX_POINT('',#61684);
#20171=VERTEX_POINT('',#61686);
#20172=VERTEX_POINT('',#61689);
#20173=VERTEX_POINT('',#61690);
#20174=VERTEX_POINT('',#61692);
#20175=VERTEX_POINT('',#61694);
#20176=VERTEX_POINT('',#61696);
#20177=VERTEX_POINT('',#61698);
#20178=VERTEX_POINT('',#61701);
#20179=VERTEX_POINT('',#61702);
#20180=VERTEX_POINT('',#61704);
#20181=VERTEX_POINT('',#61706);
#20182=VERTEX_POINT('',#61708);
#20183=VERTEX_POINT('',#61710);
#20184=VERTEX_POINT('',#61713);
#20185=VERTEX_POINT('',#61714);
#20186=VERTEX_POINT('',#61716);
#20187=VERTEX_POINT('',#61718);
#20188=VERTEX_POINT('',#61720);
#20189=VERTEX_POINT('',#61722);
#20190=VERTEX_POINT('',#61725);
#20191=VERTEX_POINT('',#61726);
#20192=VERTEX_POINT('',#61728);
#20193=VERTEX_POINT('',#61730);
#20194=VERTEX_POINT('',#61732);
#20195=VERTEX_POINT('',#61734);
#20196=VERTEX_POINT('',#61737);
#20197=VERTEX_POINT('',#61738);
#20198=VERTEX_POINT('',#61740);
#20199=VERTEX_POINT('',#61742);
#20200=VERTEX_POINT('',#61744);
#20201=VERTEX_POINT('',#61746);
#20202=VERTEX_POINT('',#61749);
#20203=VERTEX_POINT('',#61750);
#20204=VERTEX_POINT('',#61752);
#20205=VERTEX_POINT('',#61754);
#20206=VERTEX_POINT('',#61756);
#20207=VERTEX_POINT('',#61758);
#20208=VERTEX_POINT('',#61761);
#20209=VERTEX_POINT('',#61762);
#20210=VERTEX_POINT('',#61764);
#20211=VERTEX_POINT('',#61766);
#20212=VERTEX_POINT('',#61768);
#20213=VERTEX_POINT('',#61770);
#20214=VERTEX_POINT('',#61773);
#20215=VERTEX_POINT('',#61774);
#20216=VERTEX_POINT('',#61776);
#20217=VERTEX_POINT('',#61778);
#20218=VERTEX_POINT('',#61780);
#20219=VERTEX_POINT('',#61782);
#20220=VERTEX_POINT('',#61785);
#20221=VERTEX_POINT('',#61786);
#20222=VERTEX_POINT('',#61788);
#20223=VERTEX_POINT('',#61790);
#20224=VERTEX_POINT('',#61792);
#20225=VERTEX_POINT('',#61794);
#20226=VERTEX_POINT('',#61797);
#20227=VERTEX_POINT('',#61798);
#20228=VERTEX_POINT('',#61800);
#20229=VERTEX_POINT('',#61802);
#20230=VERTEX_POINT('',#61804);
#20231=VERTEX_POINT('',#61806);
#20232=VERTEX_POINT('',#61809);
#20233=VERTEX_POINT('',#61810);
#20234=VERTEX_POINT('',#61812);
#20235=VERTEX_POINT('',#61814);
#20236=VERTEX_POINT('',#61816);
#20237=VERTEX_POINT('',#61818);
#20238=VERTEX_POINT('',#61821);
#20239=VERTEX_POINT('',#61822);
#20240=VERTEX_POINT('',#61824);
#20241=VERTEX_POINT('',#61826);
#20242=VERTEX_POINT('',#61828);
#20243=VERTEX_POINT('',#61830);
#20244=VERTEX_POINT('',#61833);
#20245=VERTEX_POINT('',#61834);
#20246=VERTEX_POINT('',#61836);
#20247=VERTEX_POINT('',#61838);
#20248=VERTEX_POINT('',#61840);
#20249=VERTEX_POINT('',#61842);
#20250=VERTEX_POINT('',#61845);
#20251=VERTEX_POINT('',#61846);
#20252=VERTEX_POINT('',#61848);
#20253=VERTEX_POINT('',#61850);
#20254=VERTEX_POINT('',#61852);
#20255=VERTEX_POINT('',#61854);
#20256=VERTEX_POINT('',#61857);
#20257=VERTEX_POINT('',#61858);
#20258=VERTEX_POINT('',#61860);
#20259=VERTEX_POINT('',#61862);
#20260=VERTEX_POINT('',#61864);
#20261=VERTEX_POINT('',#61866);
#20262=VERTEX_POINT('',#61869);
#20263=VERTEX_POINT('',#61870);
#20264=VERTEX_POINT('',#61872);
#20265=VERTEX_POINT('',#61874);
#20266=VERTEX_POINT('',#61876);
#20267=VERTEX_POINT('',#61878);
#20268=VERTEX_POINT('',#61881);
#20269=VERTEX_POINT('',#61882);
#20270=VERTEX_POINT('',#61884);
#20271=VERTEX_POINT('',#61886);
#20272=VERTEX_POINT('',#61888);
#20273=VERTEX_POINT('',#61890);
#20274=VERTEX_POINT('',#61893);
#20275=VERTEX_POINT('',#61894);
#20276=VERTEX_POINT('',#61896);
#20277=VERTEX_POINT('',#61898);
#20278=VERTEX_POINT('',#61900);
#20279=VERTEX_POINT('',#61902);
#20280=VERTEX_POINT('',#61905);
#20281=VERTEX_POINT('',#61906);
#20282=VERTEX_POINT('',#61908);
#20283=VERTEX_POINT('',#61910);
#20284=VERTEX_POINT('',#61912);
#20285=VERTEX_POINT('',#61914);
#20286=VERTEX_POINT('',#61917);
#20287=VERTEX_POINT('',#61918);
#20288=VERTEX_POINT('',#61920);
#20289=VERTEX_POINT('',#61922);
#20290=VERTEX_POINT('',#61924);
#20291=VERTEX_POINT('',#61926);
#20292=VERTEX_POINT('',#61929);
#20293=VERTEX_POINT('',#61930);
#20294=VERTEX_POINT('',#61932);
#20295=VERTEX_POINT('',#61934);
#20296=VERTEX_POINT('',#61936);
#20297=VERTEX_POINT('',#61938);
#20298=VERTEX_POINT('',#61941);
#20299=VERTEX_POINT('',#61942);
#20300=VERTEX_POINT('',#61944);
#20301=VERTEX_POINT('',#61946);
#20302=VERTEX_POINT('',#61948);
#20303=VERTEX_POINT('',#61950);
#20304=VERTEX_POINT('',#61953);
#20305=VERTEX_POINT('',#61954);
#20306=VERTEX_POINT('',#61956);
#20307=VERTEX_POINT('',#61958);
#20308=VERTEX_POINT('',#61960);
#20309=VERTEX_POINT('',#61962);
#20310=VERTEX_POINT('',#61965);
#20311=VERTEX_POINT('',#61966);
#20312=VERTEX_POINT('',#61968);
#20313=VERTEX_POINT('',#61970);
#20314=VERTEX_POINT('',#61972);
#20315=VERTEX_POINT('',#61974);
#20316=VERTEX_POINT('',#61977);
#20317=VERTEX_POINT('',#61978);
#20318=VERTEX_POINT('',#61980);
#20319=VERTEX_POINT('',#61982);
#20320=VERTEX_POINT('',#61984);
#20321=VERTEX_POINT('',#61986);
#20322=VERTEX_POINT('',#61989);
#20323=VERTEX_POINT('',#61990);
#20324=VERTEX_POINT('',#61992);
#20325=VERTEX_POINT('',#61994);
#20326=VERTEX_POINT('',#61996);
#20327=VERTEX_POINT('',#61998);
#20328=VERTEX_POINT('',#62001);
#20329=VERTEX_POINT('',#62002);
#20330=VERTEX_POINT('',#62004);
#20331=VERTEX_POINT('',#62006);
#20332=VERTEX_POINT('',#62008);
#20333=VERTEX_POINT('',#62010);
#20334=VERTEX_POINT('',#62013);
#20335=VERTEX_POINT('',#62014);
#20336=VERTEX_POINT('',#62016);
#20337=VERTEX_POINT('',#62018);
#20338=VERTEX_POINT('',#62020);
#20339=VERTEX_POINT('',#62022);
#20340=VERTEX_POINT('',#62025);
#20341=VERTEX_POINT('',#62026);
#20342=VERTEX_POINT('',#62028);
#20343=VERTEX_POINT('',#62030);
#20344=VERTEX_POINT('',#62032);
#20345=VERTEX_POINT('',#62034);
#20346=VERTEX_POINT('',#62037);
#20347=VERTEX_POINT('',#62038);
#20348=VERTEX_POINT('',#62040);
#20349=VERTEX_POINT('',#62042);
#20350=VERTEX_POINT('',#62044);
#20351=VERTEX_POINT('',#62046);
#20352=VERTEX_POINT('',#62049);
#20353=VERTEX_POINT('',#62050);
#20354=VERTEX_POINT('',#62052);
#20355=VERTEX_POINT('',#62054);
#20356=VERTEX_POINT('',#62056);
#20357=VERTEX_POINT('',#62058);
#20358=VERTEX_POINT('',#62061);
#20359=VERTEX_POINT('',#62062);
#20360=VERTEX_POINT('',#62064);
#20361=VERTEX_POINT('',#62066);
#20362=VERTEX_POINT('',#62068);
#20363=VERTEX_POINT('',#62070);
#20364=VERTEX_POINT('',#62073);
#20365=VERTEX_POINT('',#62074);
#20366=VERTEX_POINT('',#62076);
#20367=VERTEX_POINT('',#62078);
#20368=VERTEX_POINT('',#62080);
#20369=VERTEX_POINT('',#62082);
#20370=VERTEX_POINT('',#62085);
#20371=VERTEX_POINT('',#62086);
#20372=VERTEX_POINT('',#62088);
#20373=VERTEX_POINT('',#62090);
#20374=VERTEX_POINT('',#62092);
#20375=VERTEX_POINT('',#62094);
#20376=VERTEX_POINT('',#62097);
#20377=VERTEX_POINT('',#62098);
#20378=VERTEX_POINT('',#62100);
#20379=VERTEX_POINT('',#62102);
#20380=VERTEX_POINT('',#62104);
#20381=VERTEX_POINT('',#62106);
#20382=VERTEX_POINT('',#62109);
#20383=VERTEX_POINT('',#62110);
#20384=VERTEX_POINT('',#62112);
#20385=VERTEX_POINT('',#62114);
#20386=VERTEX_POINT('',#62116);
#20387=VERTEX_POINT('',#62118);
#20388=VERTEX_POINT('',#62121);
#20389=VERTEX_POINT('',#62122);
#20390=VERTEX_POINT('',#62124);
#20391=VERTEX_POINT('',#62126);
#20392=VERTEX_POINT('',#62128);
#20393=VERTEX_POINT('',#62130);
#20394=VERTEX_POINT('',#62133);
#20395=VERTEX_POINT('',#62134);
#20396=VERTEX_POINT('',#62136);
#20397=VERTEX_POINT('',#62138);
#20398=VERTEX_POINT('',#62140);
#20399=VERTEX_POINT('',#62142);
#20400=VERTEX_POINT('',#62145);
#20401=VERTEX_POINT('',#62146);
#20402=VERTEX_POINT('',#62148);
#20403=VERTEX_POINT('',#62150);
#20404=VERTEX_POINT('',#62152);
#20405=VERTEX_POINT('',#62154);
#20406=VERTEX_POINT('',#62157);
#20407=VERTEX_POINT('',#62158);
#20408=VERTEX_POINT('',#62160);
#20409=VERTEX_POINT('',#62162);
#20410=VERTEX_POINT('',#62164);
#20411=VERTEX_POINT('',#62166);
#20412=VERTEX_POINT('',#62169);
#20413=VERTEX_POINT('',#62170);
#20414=VERTEX_POINT('',#62172);
#20415=VERTEX_POINT('',#62174);
#20416=VERTEX_POINT('',#62176);
#20417=VERTEX_POINT('',#62178);
#20418=VERTEX_POINT('',#62181);
#20419=VERTEX_POINT('',#62182);
#20420=VERTEX_POINT('',#62184);
#20421=VERTEX_POINT('',#62186);
#20422=VERTEX_POINT('',#62188);
#20423=VERTEX_POINT('',#62190);
#20424=VERTEX_POINT('',#62193);
#20425=VERTEX_POINT('',#62194);
#20426=VERTEX_POINT('',#62196);
#20427=VERTEX_POINT('',#62198);
#20428=VERTEX_POINT('',#62200);
#20429=VERTEX_POINT('',#62202);
#20430=VERTEX_POINT('',#62205);
#20431=VERTEX_POINT('',#62206);
#20432=VERTEX_POINT('',#62208);
#20433=VERTEX_POINT('',#62210);
#20434=VERTEX_POINT('',#62212);
#20435=VERTEX_POINT('',#62214);
#20436=VERTEX_POINT('',#62217);
#20437=VERTEX_POINT('',#62218);
#20438=VERTEX_POINT('',#62220);
#20439=VERTEX_POINT('',#62222);
#20440=VERTEX_POINT('',#62224);
#20441=VERTEX_POINT('',#62226);
#20442=VERTEX_POINT('',#62229);
#20443=VERTEX_POINT('',#62230);
#20444=VERTEX_POINT('',#62232);
#20445=VERTEX_POINT('',#62234);
#20446=VERTEX_POINT('',#62236);
#20447=VERTEX_POINT('',#62238);
#20448=VERTEX_POINT('',#62241);
#20449=VERTEX_POINT('',#62242);
#20450=VERTEX_POINT('',#62244);
#20451=VERTEX_POINT('',#62246);
#20452=VERTEX_POINT('',#62248);
#20453=VERTEX_POINT('',#62250);
#20454=VERTEX_POINT('',#62253);
#20455=VERTEX_POINT('',#62254);
#20456=VERTEX_POINT('',#62256);
#20457=VERTEX_POINT('',#62258);
#20458=VERTEX_POINT('',#62260);
#20459=VERTEX_POINT('',#62262);
#20460=VERTEX_POINT('',#62265);
#20461=VERTEX_POINT('',#62266);
#20462=VERTEX_POINT('',#62268);
#20463=VERTEX_POINT('',#62270);
#20464=VERTEX_POINT('',#62272);
#20465=VERTEX_POINT('',#62274);
#20466=VERTEX_POINT('',#62277);
#20467=VERTEX_POINT('',#62278);
#20468=VERTEX_POINT('',#62280);
#20469=VERTEX_POINT('',#62282);
#20470=VERTEX_POINT('',#62284);
#20471=VERTEX_POINT('',#62286);
#20472=VERTEX_POINT('',#62289);
#20473=VERTEX_POINT('',#62290);
#20474=VERTEX_POINT('',#62292);
#20475=VERTEX_POINT('',#62294);
#20476=VERTEX_POINT('',#62296);
#20477=VERTEX_POINT('',#62298);
#20478=VERTEX_POINT('',#62301);
#20479=VERTEX_POINT('',#62302);
#20480=VERTEX_POINT('',#62304);
#20481=VERTEX_POINT('',#62306);
#20482=VERTEX_POINT('',#62308);
#20483=VERTEX_POINT('',#62310);
#20484=VERTEX_POINT('',#62313);
#20485=VERTEX_POINT('',#62314);
#20486=VERTEX_POINT('',#62316);
#20487=VERTEX_POINT('',#62318);
#20488=VERTEX_POINT('',#62320);
#20489=VERTEX_POINT('',#62322);
#20490=VERTEX_POINT('',#62325);
#20491=VERTEX_POINT('',#62326);
#20492=VERTEX_POINT('',#62328);
#20493=VERTEX_POINT('',#62330);
#20494=VERTEX_POINT('',#62332);
#20495=VERTEX_POINT('',#62334);
#20496=VERTEX_POINT('',#62337);
#20497=VERTEX_POINT('',#62338);
#20498=VERTEX_POINT('',#62340);
#20499=VERTEX_POINT('',#62342);
#20500=VERTEX_POINT('',#62344);
#20501=VERTEX_POINT('',#62346);
#20502=VERTEX_POINT('',#62349);
#20503=VERTEX_POINT('',#62350);
#20504=VERTEX_POINT('',#62352);
#20505=VERTEX_POINT('',#62354);
#20506=VERTEX_POINT('',#62356);
#20507=VERTEX_POINT('',#62358);
#20508=VERTEX_POINT('',#62361);
#20509=VERTEX_POINT('',#62362);
#20510=VERTEX_POINT('',#62364);
#20511=VERTEX_POINT('',#62366);
#20512=VERTEX_POINT('',#62368);
#20513=VERTEX_POINT('',#62370);
#20514=VERTEX_POINT('',#62373);
#20515=VERTEX_POINT('',#62374);
#20516=VERTEX_POINT('',#62376);
#20517=VERTEX_POINT('',#62378);
#20518=VERTEX_POINT('',#62380);
#20519=VERTEX_POINT('',#62382);
#20520=VERTEX_POINT('',#62385);
#20521=VERTEX_POINT('',#62386);
#20522=VERTEX_POINT('',#62388);
#20523=VERTEX_POINT('',#62390);
#20524=VERTEX_POINT('',#62392);
#20525=VERTEX_POINT('',#62394);
#20526=VERTEX_POINT('',#62397);
#20527=VERTEX_POINT('',#62398);
#20528=VERTEX_POINT('',#62400);
#20529=VERTEX_POINT('',#62402);
#20530=VERTEX_POINT('',#62404);
#20531=VERTEX_POINT('',#62406);
#20532=VERTEX_POINT('',#62409);
#20533=VERTEX_POINT('',#62410);
#20534=VERTEX_POINT('',#62412);
#20535=VERTEX_POINT('',#62414);
#20536=VERTEX_POINT('',#62416);
#20537=VERTEX_POINT('',#62418);
#20538=VERTEX_POINT('',#62421);
#20539=VERTEX_POINT('',#62422);
#20540=VERTEX_POINT('',#62424);
#20541=VERTEX_POINT('',#62426);
#20542=VERTEX_POINT('',#62428);
#20543=VERTEX_POINT('',#62430);
#20544=VERTEX_POINT('',#62433);
#20545=VERTEX_POINT('',#62434);
#20546=VERTEX_POINT('',#62436);
#20547=VERTEX_POINT('',#62438);
#20548=VERTEX_POINT('',#62440);
#20549=VERTEX_POINT('',#62442);
#20550=VERTEX_POINT('',#62445);
#20551=VERTEX_POINT('',#62446);
#20552=VERTEX_POINT('',#62448);
#20553=VERTEX_POINT('',#62450);
#20554=VERTEX_POINT('',#62452);
#20555=VERTEX_POINT('',#62454);
#20556=VERTEX_POINT('',#62457);
#20557=VERTEX_POINT('',#62458);
#20558=VERTEX_POINT('',#62460);
#20559=VERTEX_POINT('',#62462);
#20560=VERTEX_POINT('',#62464);
#20561=VERTEX_POINT('',#62466);
#20562=VERTEX_POINT('',#62469);
#20563=VERTEX_POINT('',#62470);
#20564=VERTEX_POINT('',#62472);
#20565=VERTEX_POINT('',#62474);
#20566=VERTEX_POINT('',#62476);
#20567=VERTEX_POINT('',#62478);
#20568=VERTEX_POINT('',#62481);
#20569=VERTEX_POINT('',#62482);
#20570=VERTEX_POINT('',#62484);
#20571=VERTEX_POINT('',#62486);
#20572=VERTEX_POINT('',#62488);
#20573=VERTEX_POINT('',#62490);
#20574=VERTEX_POINT('',#62493);
#20575=VERTEX_POINT('',#62494);
#20576=VERTEX_POINT('',#62496);
#20577=VERTEX_POINT('',#62498);
#20578=VERTEX_POINT('',#62500);
#20579=VERTEX_POINT('',#62502);
#20580=VERTEX_POINT('',#62505);
#20581=VERTEX_POINT('',#62506);
#20582=VERTEX_POINT('',#62508);
#20583=VERTEX_POINT('',#62510);
#20584=VERTEX_POINT('',#62512);
#20585=VERTEX_POINT('',#62514);
#20586=VERTEX_POINT('',#62517);
#20587=VERTEX_POINT('',#62518);
#20588=VERTEX_POINT('',#62520);
#20589=VERTEX_POINT('',#62522);
#20590=VERTEX_POINT('',#62524);
#20591=VERTEX_POINT('',#62526);
#20592=VERTEX_POINT('',#62529);
#20593=VERTEX_POINT('',#62530);
#20594=VERTEX_POINT('',#62532);
#20595=VERTEX_POINT('',#62534);
#20596=VERTEX_POINT('',#62536);
#20597=VERTEX_POINT('',#62538);
#20598=VERTEX_POINT('',#62541);
#20599=VERTEX_POINT('',#62542);
#20600=VERTEX_POINT('',#62544);
#20601=VERTEX_POINT('',#62546);
#20602=VERTEX_POINT('',#62548);
#20603=VERTEX_POINT('',#62550);
#20604=VERTEX_POINT('',#62553);
#20605=VERTEX_POINT('',#62554);
#20606=VERTEX_POINT('',#62556);
#20607=VERTEX_POINT('',#62558);
#20608=VERTEX_POINT('',#62560);
#20609=VERTEX_POINT('',#62562);
#20610=VERTEX_POINT('',#62565);
#20611=VERTEX_POINT('',#62566);
#20612=VERTEX_POINT('',#62568);
#20613=VERTEX_POINT('',#62570);
#20614=VERTEX_POINT('',#62572);
#20615=VERTEX_POINT('',#62574);
#20616=VERTEX_POINT('',#62577);
#20617=VERTEX_POINT('',#62578);
#20618=VERTEX_POINT('',#62580);
#20619=VERTEX_POINT('',#62582);
#20620=VERTEX_POINT('',#62584);
#20621=VERTEX_POINT('',#62586);
#20622=VERTEX_POINT('',#62589);
#20623=VERTEX_POINT('',#62590);
#20624=VERTEX_POINT('',#62592);
#20625=VERTEX_POINT('',#62594);
#20626=VERTEX_POINT('',#62596);
#20627=VERTEX_POINT('',#62598);
#20628=VERTEX_POINT('',#62601);
#20629=VERTEX_POINT('',#62602);
#20630=VERTEX_POINT('',#62604);
#20631=VERTEX_POINT('',#62606);
#20632=VERTEX_POINT('',#62608);
#20633=VERTEX_POINT('',#62610);
#20634=VERTEX_POINT('',#62613);
#20635=VERTEX_POINT('',#62614);
#20636=VERTEX_POINT('',#62616);
#20637=VERTEX_POINT('',#62618);
#20638=VERTEX_POINT('',#62620);
#20639=VERTEX_POINT('',#62622);
#20640=VERTEX_POINT('',#62625);
#20641=VERTEX_POINT('',#62626);
#20642=VERTEX_POINT('',#62628);
#20643=VERTEX_POINT('',#62630);
#20644=VERTEX_POINT('',#62632);
#20645=VERTEX_POINT('',#62634);
#20646=VERTEX_POINT('',#62637);
#20647=VERTEX_POINT('',#62638);
#20648=VERTEX_POINT('',#62640);
#20649=VERTEX_POINT('',#62642);
#20650=VERTEX_POINT('',#62644);
#20651=VERTEX_POINT('',#62646);
#20652=VERTEX_POINT('',#62649);
#20653=VERTEX_POINT('',#62650);
#20654=VERTEX_POINT('',#62652);
#20655=VERTEX_POINT('',#62654);
#20656=VERTEX_POINT('',#62656);
#20657=VERTEX_POINT('',#62658);
#20658=VERTEX_POINT('',#62661);
#20659=VERTEX_POINT('',#62662);
#20660=VERTEX_POINT('',#62664);
#20661=VERTEX_POINT('',#62666);
#20662=VERTEX_POINT('',#62668);
#20663=VERTEX_POINT('',#62670);
#20664=VERTEX_POINT('',#62673);
#20665=VERTEX_POINT('',#62674);
#20666=VERTEX_POINT('',#62676);
#20667=VERTEX_POINT('',#62678);
#20668=VERTEX_POINT('',#62680);
#20669=VERTEX_POINT('',#62682);
#20670=VERTEX_POINT('',#62685);
#20671=VERTEX_POINT('',#62686);
#20672=VERTEX_POINT('',#62688);
#20673=VERTEX_POINT('',#62690);
#20674=VERTEX_POINT('',#62692);
#20675=VERTEX_POINT('',#62694);
#20676=VERTEX_POINT('',#62697);
#20677=VERTEX_POINT('',#62698);
#20678=VERTEX_POINT('',#62700);
#20679=VERTEX_POINT('',#62702);
#20680=VERTEX_POINT('',#62704);
#20681=VERTEX_POINT('',#62706);
#20682=VERTEX_POINT('',#62709);
#20683=VERTEX_POINT('',#62710);
#20684=VERTEX_POINT('',#62712);
#20685=VERTEX_POINT('',#62714);
#20686=VERTEX_POINT('',#62716);
#20687=VERTEX_POINT('',#62718);
#20688=VERTEX_POINT('',#62721);
#20689=VERTEX_POINT('',#62722);
#20690=VERTEX_POINT('',#62724);
#20691=VERTEX_POINT('',#62726);
#20692=VERTEX_POINT('',#62728);
#20693=VERTEX_POINT('',#62730);
#20694=VERTEX_POINT('',#62733);
#20695=VERTEX_POINT('',#62734);
#20696=VERTEX_POINT('',#62736);
#20697=VERTEX_POINT('',#62738);
#20698=VERTEX_POINT('',#62740);
#20699=VERTEX_POINT('',#62742);
#20700=VERTEX_POINT('',#62745);
#20701=VERTEX_POINT('',#62746);
#20702=VERTEX_POINT('',#62748);
#20703=VERTEX_POINT('',#62750);
#20704=VERTEX_POINT('',#62752);
#20705=VERTEX_POINT('',#62754);
#20706=VERTEX_POINT('',#62757);
#20707=VERTEX_POINT('',#62758);
#20708=VERTEX_POINT('',#62760);
#20709=VERTEX_POINT('',#62762);
#20710=VERTEX_POINT('',#62764);
#20711=VERTEX_POINT('',#62766);
#20712=VERTEX_POINT('',#62769);
#20713=VERTEX_POINT('',#62770);
#20714=VERTEX_POINT('',#62772);
#20715=VERTEX_POINT('',#62774);
#20716=VERTEX_POINT('',#62776);
#20717=VERTEX_POINT('',#62778);
#20718=VERTEX_POINT('',#62781);
#20719=VERTEX_POINT('',#62782);
#20720=VERTEX_POINT('',#62784);
#20721=VERTEX_POINT('',#62786);
#20722=VERTEX_POINT('',#62788);
#20723=VERTEX_POINT('',#62790);
#20724=VERTEX_POINT('',#62793);
#20725=VERTEX_POINT('',#62794);
#20726=VERTEX_POINT('',#62796);
#20727=VERTEX_POINT('',#62798);
#20728=VERTEX_POINT('',#62800);
#20729=VERTEX_POINT('',#62802);
#20730=VERTEX_POINT('',#62805);
#20731=VERTEX_POINT('',#62806);
#20732=VERTEX_POINT('',#62808);
#20733=VERTEX_POINT('',#62810);
#20734=VERTEX_POINT('',#62812);
#20735=VERTEX_POINT('',#62814);
#20736=VERTEX_POINT('',#62817);
#20737=VERTEX_POINT('',#62818);
#20738=VERTEX_POINT('',#62820);
#20739=VERTEX_POINT('',#62822);
#20740=VERTEX_POINT('',#62824);
#20741=VERTEX_POINT('',#62826);
#20742=VERTEX_POINT('',#62829);
#20743=VERTEX_POINT('',#62830);
#20744=VERTEX_POINT('',#62832);
#20745=VERTEX_POINT('',#62834);
#20746=VERTEX_POINT('',#62836);
#20747=VERTEX_POINT('',#62838);
#20748=VERTEX_POINT('',#62841);
#20749=VERTEX_POINT('',#62842);
#20750=VERTEX_POINT('',#62844);
#20751=VERTEX_POINT('',#62846);
#20752=VERTEX_POINT('',#62848);
#20753=VERTEX_POINT('',#62850);
#20754=VERTEX_POINT('',#62853);
#20755=VERTEX_POINT('',#62854);
#20756=VERTEX_POINT('',#62856);
#20757=VERTEX_POINT('',#62858);
#20758=VERTEX_POINT('',#62860);
#20759=VERTEX_POINT('',#62862);
#20760=VERTEX_POINT('',#62865);
#20761=VERTEX_POINT('',#62866);
#20762=VERTEX_POINT('',#62868);
#20763=VERTEX_POINT('',#62870);
#20764=VERTEX_POINT('',#62872);
#20765=VERTEX_POINT('',#62874);
#20766=VERTEX_POINT('',#62877);
#20767=VERTEX_POINT('',#62878);
#20768=VERTEX_POINT('',#62880);
#20769=VERTEX_POINT('',#62882);
#20770=VERTEX_POINT('',#62884);
#20771=VERTEX_POINT('',#62886);
#20772=VERTEX_POINT('',#62889);
#20773=VERTEX_POINT('',#62890);
#20774=VERTEX_POINT('',#62892);
#20775=VERTEX_POINT('',#62894);
#20776=VERTEX_POINT('',#62896);
#20777=VERTEX_POINT('',#62898);
#20778=VERTEX_POINT('',#62901);
#20779=VERTEX_POINT('',#62902);
#20780=VERTEX_POINT('',#62904);
#20781=VERTEX_POINT('',#62906);
#20782=VERTEX_POINT('',#62908);
#20783=VERTEX_POINT('',#62910);
#20784=VERTEX_POINT('',#62913);
#20785=VERTEX_POINT('',#62914);
#20786=VERTEX_POINT('',#62916);
#20787=VERTEX_POINT('',#62918);
#20788=VERTEX_POINT('',#62920);
#20789=VERTEX_POINT('',#62922);
#20790=VERTEX_POINT('',#62925);
#20791=VERTEX_POINT('',#62926);
#20792=VERTEX_POINT('',#62928);
#20793=VERTEX_POINT('',#62930);
#20794=VERTEX_POINT('',#62932);
#20795=VERTEX_POINT('',#62934);
#20796=VERTEX_POINT('',#62937);
#20797=VERTEX_POINT('',#62938);
#20798=VERTEX_POINT('',#62940);
#20799=VERTEX_POINT('',#62942);
#20800=VERTEX_POINT('',#62944);
#20801=VERTEX_POINT('',#62946);
#20802=VERTEX_POINT('',#62949);
#20803=VERTEX_POINT('',#62950);
#20804=VERTEX_POINT('',#62952);
#20805=VERTEX_POINT('',#62954);
#20806=VERTEX_POINT('',#62956);
#20807=VERTEX_POINT('',#62958);
#20808=VERTEX_POINT('',#62961);
#20809=VERTEX_POINT('',#62962);
#20810=VERTEX_POINT('',#62964);
#20811=VERTEX_POINT('',#62966);
#20812=VERTEX_POINT('',#62968);
#20813=VERTEX_POINT('',#62970);
#20814=VERTEX_POINT('',#62973);
#20815=VERTEX_POINT('',#62974);
#20816=VERTEX_POINT('',#62976);
#20817=VERTEX_POINT('',#62978);
#20818=VERTEX_POINT('',#62980);
#20819=VERTEX_POINT('',#62982);
#20820=VERTEX_POINT('',#62985);
#20821=VERTEX_POINT('',#62986);
#20822=VERTEX_POINT('',#62988);
#20823=VERTEX_POINT('',#62990);
#20824=VERTEX_POINT('',#62992);
#20825=VERTEX_POINT('',#62994);
#20826=VERTEX_POINT('',#62997);
#20827=VERTEX_POINT('',#62998);
#20828=VERTEX_POINT('',#63000);
#20829=VERTEX_POINT('',#63002);
#20830=VERTEX_POINT('',#63004);
#20831=VERTEX_POINT('',#63006);
#20832=VERTEX_POINT('',#63009);
#20833=VERTEX_POINT('',#63010);
#20834=VERTEX_POINT('',#63012);
#20835=VERTEX_POINT('',#63014);
#20836=VERTEX_POINT('',#63016);
#20837=VERTEX_POINT('',#63018);
#20838=VERTEX_POINT('',#63021);
#20839=VERTEX_POINT('',#63022);
#20840=VERTEX_POINT('',#63024);
#20841=VERTEX_POINT('',#63026);
#20842=VERTEX_POINT('',#63028);
#20843=VERTEX_POINT('',#63030);
#20844=VERTEX_POINT('',#63033);
#20845=VERTEX_POINT('',#63034);
#20846=VERTEX_POINT('',#63036);
#20847=VERTEX_POINT('',#63038);
#20848=VERTEX_POINT('',#63040);
#20849=VERTEX_POINT('',#63042);
#20850=VERTEX_POINT('',#63045);
#20851=VERTEX_POINT('',#63046);
#20852=VERTEX_POINT('',#63048);
#20853=VERTEX_POINT('',#63050);
#20854=VERTEX_POINT('',#63052);
#20855=VERTEX_POINT('',#63054);
#23007=EDGE_CURVE('',#18554,#18554,#17110,.T.);
#23008=EDGE_CURVE('',#18554,#18555,#17111,.T.);
#23009=EDGE_CURVE('',#18555,#18555,#17112,.T.);
#23010=EDGE_CURVE('',#18556,#18556,#17113,.T.);
#23011=EDGE_CURVE('',#18556,#18557,#17114,.T.);
#23012=EDGE_CURVE('',#18557,#18557,#17115,.T.);
#23013=EDGE_CURVE('',#18558,#18558,#17116,.T.);
#23014=EDGE_CURVE('',#18558,#18556,#17117,.T.);
#23015=EDGE_CURVE('',#18559,#18559,#17118,.T.);
#23016=EDGE_CURVE('',#18559,#18554,#17119,.T.);
#23017=EDGE_CURVE('',#18560,#18561,#8179,.T.);
#23018=EDGE_CURVE('',#18562,#18560,#8180,.T.);
#23019=EDGE_CURVE('',#18562,#18563,#8181,.T.);
#23020=EDGE_CURVE('',#18564,#18563,#8182,.T.);
#23021=EDGE_CURVE('',#18564,#18565,#8183,.T.);
#23022=EDGE_CURVE('',#18565,#18566,#8184,.T.);
#23023=EDGE_CURVE('',#18567,#18566,#8185,.T.);
#23024=EDGE_CURVE('',#18567,#18568,#8186,.T.);
#23025=EDGE_CURVE('',#18568,#18569,#8187,.T.);
#23026=EDGE_CURVE('',#18569,#18570,#8188,.T.);
#23027=EDGE_CURVE('',#18571,#18570,#8189,.T.);
#23028=EDGE_CURVE('',#18561,#18571,#8190,.T.);
#23029=EDGE_CURVE('',#18572,#18573,#8191,.T.);
#23030=EDGE_CURVE('',#18574,#18572,#8192,.T.);
#23031=EDGE_CURVE('',#18574,#18575,#8193,.T.);
#23032=EDGE_CURVE('',#18575,#18576,#8194,.T.);
#23033=EDGE_CURVE('',#18577,#18576,#8195,.T.);
#23034=EDGE_CURVE('',#18577,#18578,#8196,.T.);
#23035=EDGE_CURVE('',#18578,#18579,#8197,.T.);
#23036=EDGE_CURVE('',#18580,#18579,#8198,.T.);
#23037=EDGE_CURVE('',#18581,#18580,#8199,.T.);
#23038=EDGE_CURVE('',#18582,#18581,#8200,.T.);
#23039=EDGE_CURVE('',#18582,#18583,#8201,.T.);
#23040=EDGE_CURVE('',#18583,#18573,#8202,.T.);
#23041=EDGE_CURVE('',#18570,#18576,#8203,.T.);
#23042=EDGE_CURVE('',#18575,#18571,#8204,.T.);
#23043=EDGE_CURVE('',#18564,#18582,#8205,.T.);
#23044=EDGE_CURVE('',#18581,#18565,#8206,.T.);
#23045=EDGE_CURVE('',#18574,#18561,#8207,.T.);
#23046=EDGE_CURVE('',#18560,#18572,#8208,.T.);
#23047=EDGE_CURVE('',#18563,#18583,#8209,.T.);
#23048=EDGE_CURVE('',#18562,#18573,#8210,.T.);
#23049=EDGE_CURVE('',#18569,#18577,#8211,.T.);
#23050=EDGE_CURVE('',#18568,#18578,#8212,.T.);
#23051=EDGE_CURVE('',#18567,#18579,#8213,.T.);
#23052=EDGE_CURVE('',#18580,#18566,#8214,.T.);
#23053=EDGE_CURVE('',#18584,#18585,#8215,.T.);
#23054=EDGE_CURVE('',#18585,#18569,#17120,.T.);
#23055=EDGE_CURVE('',#18584,#18577,#17121,.T.);
#23056=EDGE_CURVE('',#18570,#18586,#17122,.T.);
#23057=EDGE_CURVE('',#18587,#18586,#8216,.T.);
#23058=EDGE_CURVE('',#18576,#18587,#17123,.T.);
#23059=EDGE_CURVE('',#18584,#18587,#8217,.T.);
#23060=EDGE_CURVE('',#18585,#18586,#8218,.T.);
#23061=EDGE_CURVE('',#18566,#18588,#17124,.T.);
#23062=EDGE_CURVE('',#18588,#18589,#8219,.T.);
#23063=EDGE_CURVE('',#18580,#18589,#17125,.T.);
#23064=EDGE_CURVE('',#18590,#18591,#8220,.T.);
#23065=EDGE_CURVE('',#18590,#18565,#17126,.T.);
#23066=EDGE_CURVE('',#18591,#18581,#17127,.T.);
#23067=EDGE_CURVE('',#18591,#18589,#8221,.T.);
#23068=EDGE_CURVE('',#18590,#18588,#8222,.T.);
#23069=EDGE_CURVE('',#18592,#18593,#17128,.T.);
#23070=EDGE_CURVE('',#18594,#18592,#8223,.T.);
#23071=EDGE_CURVE('',#18595,#18594,#17129,.T.);
#23072=EDGE_CURVE('',#18593,#18595,#8224,.T.);
#23073=EDGE_CURVE('',#18596,#18597,#8225,.T.);
#23074=EDGE_CURVE('',#18597,#18598,#8226,.T.);
#23075=EDGE_CURVE('',#18598,#18599,#8227,.T.);
#23076=EDGE_CURVE('',#18596,#18599,#8228,.T.);
#23077=EDGE_CURVE('',#18600,#18601,#17130,.T.);
#23078=EDGE_CURVE('',#18602,#18600,#8229,.T.);
#23079=EDGE_CURVE('',#18603,#18602,#17131,.T.);
#23080=EDGE_CURVE('',#18601,#18603,#8230,.T.);
#23081=EDGE_CURVE('',#18602,#18595,#8231,.T.);
#23082=EDGE_CURVE('',#18600,#18593,#8232,.T.);
#23083=EDGE_CURVE('',#18591,#18601,#8233,.T.);
#23084=EDGE_CURVE('',#18599,#18589,#8234,.T.);
#23085=EDGE_CURVE('',#18598,#18584,#8235,.T.);
#23086=EDGE_CURVE('',#18587,#18592,#8236,.T.);
#23087=EDGE_CURVE('',#18588,#18596,#8237,.T.);
#23088=EDGE_CURVE('',#18590,#18603,#8238,.T.);
#23089=EDGE_CURVE('',#18586,#18594,#8239,.T.);
#23090=EDGE_CURVE('',#18585,#18597,#8240,.T.);
#23091=EDGE_CURVE('',#18604,#18605,#8241,.T.);
#23092=EDGE_CURVE('',#18605,#18563,#17132,.T.);
#23093=EDGE_CURVE('',#18604,#18583,#17133,.T.);
#23094=EDGE_CURVE('',#18564,#18606,#17134,.T.);
#23095=EDGE_CURVE('',#18607,#18606,#8242,.T.);
#23096=EDGE_CURVE('',#18582,#18607,#17135,.T.);
#23097=EDGE_CURVE('',#18607,#18604,#8243,.T.);
#23098=EDGE_CURVE('',#18606,#18605,#8244,.T.);
#23099=EDGE_CURVE('',#18561,#18608,#17136,.T.);
#23100=EDGE_CURVE('',#18608,#18609,#8245,.T.);
#23101=EDGE_CURVE('',#18574,#18609,#17137,.T.);
#23102=EDGE_CURVE('',#18610,#18611,#8246,.T.);
#23103=EDGE_CURVE('',#18610,#18571,#17138,.T.);
#23104=EDGE_CURVE('',#18611,#18575,#17139,.T.);
#23105=EDGE_CURVE('',#18609,#18611,#8247,.T.);
#23106=EDGE_CURVE('',#18608,#18610,#8248,.T.);
#23107=EDGE_CURVE('',#18612,#18613,#17140,.T.);
#23108=EDGE_CURVE('',#18614,#18612,#8249,.T.);
#23109=EDGE_CURVE('',#18615,#18614,#17141,.T.);
#23110=EDGE_CURVE('',#18613,#18615,#8250,.T.);
#23111=EDGE_CURVE('',#18616,#18617,#8251,.T.);
#23112=EDGE_CURVE('',#18618,#18617,#8252,.T.);
#23113=EDGE_CURVE('',#18619,#18618,#8253,.T.);
#23114=EDGE_CURVE('',#18616,#18619,#8254,.T.);
#23115=EDGE_CURVE('',#18620,#18621,#17142,.T.);
#23116=EDGE_CURVE('',#18622,#18620,#8255,.T.);
#23117=EDGE_CURVE('',#18623,#18622,#17143,.T.);
#23118=EDGE_CURVE('',#18621,#18623,#8256,.T.);
#23119=EDGE_CURVE('',#18612,#18621,#8257,.T.);
#23120=EDGE_CURVE('',#18614,#18623,#8258,.T.);
#23121=EDGE_CURVE('',#18622,#18611,#8259,.T.);
#23122=EDGE_CURVE('',#18618,#18609,#8260,.T.);
#23123=EDGE_CURVE('',#18617,#18604,#8261,.T.);
#23124=EDGE_CURVE('',#18615,#18607,#8262,.T.);
#23125=EDGE_CURVE('',#18608,#18619,#8263,.T.);
#23126=EDGE_CURVE('',#18620,#18610,#8264,.T.);
#23127=EDGE_CURVE('',#18613,#18606,#8265,.T.);
#23128=EDGE_CURVE('',#18605,#18616,#8266,.T.);
#23129=EDGE_CURVE('',#18624,#18625,#8267,.T.);
#23130=EDGE_CURVE('',#18626,#18624,#8268,.T.);
#23131=EDGE_CURVE('',#18627,#18626,#8269,.T.);
#23132=EDGE_CURVE('',#18628,#18627,#8270,.T.);
#23133=EDGE_CURVE('',#18629,#18628,#8271,.T.);
#23134=EDGE_CURVE('',#18625,#18629,#8272,.T.);
#23135=EDGE_CURVE('',#18630,#18631,#8273,.T.);
#23136=EDGE_CURVE('',#18632,#18630,#8274,.T.);
#23137=EDGE_CURVE('',#18633,#18632,#8275,.T.);
#23138=EDGE_CURVE('',#18634,#18633,#8276,.T.);
#23139=EDGE_CURVE('',#18635,#18634,#8277,.T.);
#23140=EDGE_CURVE('',#18631,#18635,#8278,.T.);
#23141=EDGE_CURVE('',#18636,#18637,#8279,.T.);
#23142=EDGE_CURVE('',#18638,#18636,#8280,.T.);
#23143=EDGE_CURVE('',#18639,#18638,#8281,.T.);
#23144=EDGE_CURVE('',#18640,#18639,#8282,.T.);
#23145=EDGE_CURVE('',#18641,#18640,#8283,.T.);
#23146=EDGE_CURVE('',#18637,#18641,#8284,.T.);
#23147=EDGE_CURVE('',#18642,#18643,#8285,.T.);
#23148=EDGE_CURVE('',#18644,#18642,#8286,.T.);
#23149=EDGE_CURVE('',#18645,#18644,#8287,.T.);
#23150=EDGE_CURVE('',#18646,#18645,#8288,.T.);
#23151=EDGE_CURVE('',#18647,#18646,#8289,.T.);
#23152=EDGE_CURVE('',#18643,#18647,#8290,.T.);
#23153=EDGE_CURVE('',#18648,#18649,#8291,.T.);
#23154=EDGE_CURVE('',#18650,#18648,#8292,.T.);
#23155=EDGE_CURVE('',#18651,#18650,#8293,.T.);
#23156=EDGE_CURVE('',#18652,#18651,#8294,.T.);
#23157=EDGE_CURVE('',#18653,#18652,#8295,.T.);
#23158=EDGE_CURVE('',#18649,#18653,#8296,.T.);
#23159=EDGE_CURVE('',#18654,#18655,#8297,.T.);
#23160=EDGE_CURVE('',#18656,#18654,#8298,.T.);
#23161=EDGE_CURVE('',#18657,#18656,#8299,.T.);
#23162=EDGE_CURVE('',#18658,#18657,#8300,.T.);
#23163=EDGE_CURVE('',#18659,#18658,#8301,.T.);
#23164=EDGE_CURVE('',#18655,#18659,#8302,.T.);
#23165=EDGE_CURVE('',#18660,#18661,#8303,.T.);
#23166=EDGE_CURVE('',#18662,#18660,#8304,.T.);
#23167=EDGE_CURVE('',#18663,#18662,#8305,.T.);
#23168=EDGE_CURVE('',#18664,#18663,#8306,.T.);
#23169=EDGE_CURVE('',#18665,#18664,#8307,.T.);
#23170=EDGE_CURVE('',#18661,#18665,#8308,.T.);
#23171=EDGE_CURVE('',#18666,#18667,#8309,.T.);
#23172=EDGE_CURVE('',#18668,#18666,#8310,.T.);
#23173=EDGE_CURVE('',#18669,#18668,#8311,.T.);
#23174=EDGE_CURVE('',#18670,#18669,#8312,.T.);
#23175=EDGE_CURVE('',#18671,#18670,#8313,.T.);
#23176=EDGE_CURVE('',#18667,#18671,#8314,.T.);
#23177=EDGE_CURVE('',#18672,#18673,#8315,.T.);
#23178=EDGE_CURVE('',#18674,#18672,#8316,.T.);
#23179=EDGE_CURVE('',#18675,#18674,#8317,.T.);
#23180=EDGE_CURVE('',#18676,#18675,#8318,.T.);
#23181=EDGE_CURVE('',#18677,#18676,#8319,.T.);
#23182=EDGE_CURVE('',#18673,#18677,#8320,.T.);
#23183=EDGE_CURVE('',#18678,#18679,#8321,.T.);
#23184=EDGE_CURVE('',#18680,#18678,#8322,.T.);
#23185=EDGE_CURVE('',#18681,#18680,#8323,.T.);
#23186=EDGE_CURVE('',#18682,#18681,#8324,.T.);
#23187=EDGE_CURVE('',#18683,#18682,#8325,.T.);
#23188=EDGE_CURVE('',#18679,#18683,#8326,.T.);
#23189=EDGE_CURVE('',#18684,#18685,#8327,.T.);
#23190=EDGE_CURVE('',#18686,#18684,#8328,.T.);
#23191=EDGE_CURVE('',#18687,#18686,#8329,.T.);
#23192=EDGE_CURVE('',#18688,#18687,#8330,.T.);
#23193=EDGE_CURVE('',#18689,#18688,#8331,.T.);
#23194=EDGE_CURVE('',#18685,#18689,#8332,.T.);
#23195=EDGE_CURVE('',#18690,#18691,#8333,.T.);
#23196=EDGE_CURVE('',#18692,#18690,#8334,.T.);
#23197=EDGE_CURVE('',#18693,#18692,#8335,.T.);
#23198=EDGE_CURVE('',#18694,#18693,#8336,.T.);
#23199=EDGE_CURVE('',#18695,#18694,#8337,.T.);
#23200=EDGE_CURVE('',#18691,#18695,#8338,.T.);
#23201=EDGE_CURVE('',#18696,#18697,#8339,.T.);
#23202=EDGE_CURVE('',#18698,#18696,#8340,.T.);
#23203=EDGE_CURVE('',#18699,#18698,#8341,.T.);
#23204=EDGE_CURVE('',#18700,#18699,#8342,.T.);
#23205=EDGE_CURVE('',#18701,#18700,#8343,.T.);
#23206=EDGE_CURVE('',#18697,#18701,#8344,.T.);
#23207=EDGE_CURVE('',#18702,#18703,#8345,.T.);
#23208=EDGE_CURVE('',#18704,#18702,#8346,.T.);
#23209=EDGE_CURVE('',#18705,#18704,#8347,.T.);
#23210=EDGE_CURVE('',#18706,#18705,#8348,.T.);
#23211=EDGE_CURVE('',#18707,#18706,#8349,.T.);
#23212=EDGE_CURVE('',#18703,#18707,#8350,.T.);
#23213=EDGE_CURVE('',#18708,#18709,#8351,.T.);
#23214=EDGE_CURVE('',#18710,#18708,#8352,.T.);
#23215=EDGE_CURVE('',#18711,#18710,#8353,.T.);
#23216=EDGE_CURVE('',#18712,#18711,#8354,.T.);
#23217=EDGE_CURVE('',#18713,#18712,#8355,.T.);
#23218=EDGE_CURVE('',#18709,#18713,#8356,.T.);
#23219=EDGE_CURVE('',#18714,#18715,#8357,.T.);
#23220=EDGE_CURVE('',#18716,#18714,#8358,.T.);
#23221=EDGE_CURVE('',#18717,#18716,#8359,.T.);
#23222=EDGE_CURVE('',#18718,#18717,#8360,.T.);
#23223=EDGE_CURVE('',#18719,#18718,#8361,.T.);
#23224=EDGE_CURVE('',#18715,#18719,#8362,.T.);
#23225=EDGE_CURVE('',#18720,#18721,#8363,.T.);
#23226=EDGE_CURVE('',#18722,#18720,#8364,.T.);
#23227=EDGE_CURVE('',#18723,#18722,#8365,.T.);
#23228=EDGE_CURVE('',#18724,#18723,#8366,.T.);
#23229=EDGE_CURVE('',#18725,#18724,#8367,.T.);
#23230=EDGE_CURVE('',#18721,#18725,#8368,.T.);
#23231=EDGE_CURVE('',#18726,#18727,#8369,.T.);
#23232=EDGE_CURVE('',#18728,#18726,#8370,.T.);
#23233=EDGE_CURVE('',#18729,#18728,#8371,.T.);
#23234=EDGE_CURVE('',#18730,#18729,#8372,.T.);
#23235=EDGE_CURVE('',#18731,#18730,#8373,.T.);
#23236=EDGE_CURVE('',#18727,#18731,#8374,.T.);
#23237=EDGE_CURVE('',#18732,#18733,#8375,.T.);
#23238=EDGE_CURVE('',#18734,#18732,#8376,.T.);
#23239=EDGE_CURVE('',#18735,#18734,#8377,.T.);
#23240=EDGE_CURVE('',#18736,#18735,#8378,.T.);
#23241=EDGE_CURVE('',#18737,#18736,#8379,.T.);
#23242=EDGE_CURVE('',#18733,#18737,#8380,.T.);
#23243=EDGE_CURVE('',#18738,#18739,#8381,.T.);
#23244=EDGE_CURVE('',#18740,#18738,#8382,.T.);
#23245=EDGE_CURVE('',#18741,#18740,#8383,.T.);
#23246=EDGE_CURVE('',#18742,#18741,#8384,.T.);
#23247=EDGE_CURVE('',#18743,#18742,#8385,.T.);
#23248=EDGE_CURVE('',#18739,#18743,#8386,.T.);
#23249=EDGE_CURVE('',#18744,#18745,#8387,.T.);
#23250=EDGE_CURVE('',#18746,#18744,#8388,.T.);
#23251=EDGE_CURVE('',#18747,#18746,#8389,.T.);
#23252=EDGE_CURVE('',#18748,#18747,#8390,.T.);
#23253=EDGE_CURVE('',#18749,#18748,#8391,.T.);
#23254=EDGE_CURVE('',#18745,#18749,#8392,.T.);
#23255=EDGE_CURVE('',#18750,#18751,#8393,.T.);
#23256=EDGE_CURVE('',#18752,#18750,#8394,.T.);
#23257=EDGE_CURVE('',#18753,#18752,#8395,.T.);
#23258=EDGE_CURVE('',#18754,#18753,#8396,.T.);
#23259=EDGE_CURVE('',#18755,#18754,#8397,.T.);
#23260=EDGE_CURVE('',#18751,#18755,#8398,.T.);
#23261=EDGE_CURVE('',#18756,#18757,#8399,.T.);
#23262=EDGE_CURVE('',#18758,#18756,#8400,.T.);
#23263=EDGE_CURVE('',#18759,#18758,#8401,.T.);
#23264=EDGE_CURVE('',#18760,#18759,#8402,.T.);
#23265=EDGE_CURVE('',#18761,#18760,#8403,.T.);
#23266=EDGE_CURVE('',#18757,#18761,#8404,.T.);
#23267=EDGE_CURVE('',#18762,#18763,#8405,.T.);
#23268=EDGE_CURVE('',#18764,#18762,#8406,.T.);
#23269=EDGE_CURVE('',#18765,#18764,#8407,.T.);
#23270=EDGE_CURVE('',#18766,#18765,#8408,.T.);
#23271=EDGE_CURVE('',#18767,#18766,#8409,.T.);
#23272=EDGE_CURVE('',#18763,#18767,#8410,.T.);
#23273=EDGE_CURVE('',#18768,#18769,#8411,.T.);
#23274=EDGE_CURVE('',#18770,#18768,#8412,.T.);
#23275=EDGE_CURVE('',#18771,#18770,#8413,.T.);
#23276=EDGE_CURVE('',#18772,#18771,#8414,.T.);
#23277=EDGE_CURVE('',#18773,#18772,#8415,.T.);
#23278=EDGE_CURVE('',#18769,#18773,#8416,.T.);
#23279=EDGE_CURVE('',#18774,#18775,#8417,.T.);
#23280=EDGE_CURVE('',#18776,#18774,#8418,.T.);
#23281=EDGE_CURVE('',#18777,#18776,#8419,.T.);
#23282=EDGE_CURVE('',#18778,#18777,#8420,.T.);
#23283=EDGE_CURVE('',#18779,#18778,#8421,.T.);
#23284=EDGE_CURVE('',#18775,#18779,#8422,.T.);
#23285=EDGE_CURVE('',#18780,#18781,#8423,.T.);
#23286=EDGE_CURVE('',#18782,#18780,#8424,.T.);
#23287=EDGE_CURVE('',#18783,#18782,#8425,.T.);
#23288=EDGE_CURVE('',#18784,#18783,#8426,.T.);
#23289=EDGE_CURVE('',#18785,#18784,#8427,.T.);
#23290=EDGE_CURVE('',#18781,#18785,#8428,.T.);
#23291=EDGE_CURVE('',#18786,#18787,#8429,.T.);
#23292=EDGE_CURVE('',#18788,#18786,#8430,.T.);
#23293=EDGE_CURVE('',#18789,#18788,#8431,.T.);
#23294=EDGE_CURVE('',#18790,#18789,#8432,.T.);
#23295=EDGE_CURVE('',#18791,#18790,#8433,.T.);
#23296=EDGE_CURVE('',#18787,#18791,#8434,.T.);
#23297=EDGE_CURVE('',#18792,#18793,#8435,.T.);
#23298=EDGE_CURVE('',#18794,#18792,#8436,.T.);
#23299=EDGE_CURVE('',#18795,#18794,#8437,.T.);
#23300=EDGE_CURVE('',#18796,#18795,#8438,.T.);
#23301=EDGE_CURVE('',#18797,#18796,#8439,.T.);
#23302=EDGE_CURVE('',#18793,#18797,#8440,.T.);
#23303=EDGE_CURVE('',#18798,#18799,#8441,.T.);
#23304=EDGE_CURVE('',#18800,#18798,#8442,.T.);
#23305=EDGE_CURVE('',#18801,#18800,#8443,.T.);
#23306=EDGE_CURVE('',#18802,#18801,#8444,.T.);
#23307=EDGE_CURVE('',#18803,#18802,#8445,.T.);
#23308=EDGE_CURVE('',#18799,#18803,#8446,.T.);
#23309=EDGE_CURVE('',#18804,#18805,#8447,.T.);
#23310=EDGE_CURVE('',#18806,#18804,#8448,.T.);
#23311=EDGE_CURVE('',#18807,#18806,#8449,.T.);
#23312=EDGE_CURVE('',#18808,#18807,#8450,.T.);
#23313=EDGE_CURVE('',#18809,#18808,#8451,.T.);
#23314=EDGE_CURVE('',#18805,#18809,#8452,.T.);
#23315=EDGE_CURVE('',#18810,#18811,#8453,.T.);
#23316=EDGE_CURVE('',#18812,#18810,#8454,.T.);
#23317=EDGE_CURVE('',#18813,#18812,#8455,.T.);
#23318=EDGE_CURVE('',#18814,#18813,#8456,.T.);
#23319=EDGE_CURVE('',#18815,#18814,#8457,.T.);
#23320=EDGE_CURVE('',#18811,#18815,#8458,.T.);
#23321=EDGE_CURVE('',#18816,#18817,#8459,.T.);
#23322=EDGE_CURVE('',#18818,#18816,#8460,.T.);
#23323=EDGE_CURVE('',#18819,#18818,#8461,.T.);
#23324=EDGE_CURVE('',#18820,#18819,#8462,.T.);
#23325=EDGE_CURVE('',#18821,#18820,#8463,.T.);
#23326=EDGE_CURVE('',#18817,#18821,#8464,.T.);
#23327=EDGE_CURVE('',#18822,#18823,#8465,.T.);
#23328=EDGE_CURVE('',#18824,#18822,#8466,.T.);
#23329=EDGE_CURVE('',#18825,#18824,#8467,.T.);
#23330=EDGE_CURVE('',#18826,#18825,#8468,.T.);
#23331=EDGE_CURVE('',#18827,#18826,#8469,.T.);
#23332=EDGE_CURVE('',#18823,#18827,#8470,.T.);
#23333=EDGE_CURVE('',#18828,#18829,#8471,.T.);
#23334=EDGE_CURVE('',#18830,#18828,#8472,.T.);
#23335=EDGE_CURVE('',#18831,#18830,#8473,.T.);
#23336=EDGE_CURVE('',#18832,#18831,#8474,.T.);
#23337=EDGE_CURVE('',#18833,#18832,#8475,.T.);
#23338=EDGE_CURVE('',#18829,#18833,#8476,.T.);
#23339=EDGE_CURVE('',#18834,#18835,#8477,.T.);
#23340=EDGE_CURVE('',#18836,#18834,#8478,.T.);
#23341=EDGE_CURVE('',#18837,#18836,#8479,.T.);
#23342=EDGE_CURVE('',#18838,#18837,#8480,.T.);
#23343=EDGE_CURVE('',#18839,#18838,#8481,.T.);
#23344=EDGE_CURVE('',#18835,#18839,#8482,.T.);
#23345=EDGE_CURVE('',#18840,#18841,#8483,.T.);
#23346=EDGE_CURVE('',#18842,#18840,#8484,.T.);
#23347=EDGE_CURVE('',#18843,#18842,#8485,.T.);
#23348=EDGE_CURVE('',#18844,#18843,#8486,.T.);
#23349=EDGE_CURVE('',#18845,#18844,#8487,.T.);
#23350=EDGE_CURVE('',#18841,#18845,#8488,.T.);
#23351=EDGE_CURVE('',#18846,#18847,#8489,.T.);
#23352=EDGE_CURVE('',#18848,#18846,#8490,.T.);
#23353=EDGE_CURVE('',#18849,#18848,#8491,.T.);
#23354=EDGE_CURVE('',#18850,#18849,#8492,.T.);
#23355=EDGE_CURVE('',#18851,#18850,#8493,.T.);
#23356=EDGE_CURVE('',#18847,#18851,#8494,.T.);
#23357=EDGE_CURVE('',#18852,#18853,#8495,.T.);
#23358=EDGE_CURVE('',#18854,#18852,#8496,.T.);
#23359=EDGE_CURVE('',#18855,#18854,#8497,.T.);
#23360=EDGE_CURVE('',#18856,#18855,#8498,.T.);
#23361=EDGE_CURVE('',#18857,#18856,#8499,.T.);
#23362=EDGE_CURVE('',#18853,#18857,#8500,.T.);
#23363=EDGE_CURVE('',#18858,#18859,#8501,.T.);
#23364=EDGE_CURVE('',#18860,#18858,#8502,.T.);
#23365=EDGE_CURVE('',#18861,#18860,#8503,.T.);
#23366=EDGE_CURVE('',#18862,#18861,#8504,.T.);
#23367=EDGE_CURVE('',#18863,#18862,#8505,.T.);
#23368=EDGE_CURVE('',#18859,#18863,#8506,.T.);
#23369=EDGE_CURVE('',#18864,#18865,#8507,.T.);
#23370=EDGE_CURVE('',#18866,#18864,#8508,.T.);
#23371=EDGE_CURVE('',#18867,#18866,#8509,.T.);
#23372=EDGE_CURVE('',#18868,#18867,#8510,.T.);
#23373=EDGE_CURVE('',#18869,#18868,#8511,.T.);
#23374=EDGE_CURVE('',#18865,#18869,#8512,.T.);
#23375=EDGE_CURVE('',#18870,#18871,#8513,.T.);
#23376=EDGE_CURVE('',#18872,#18870,#8514,.T.);
#23377=EDGE_CURVE('',#18873,#18872,#8515,.T.);
#23378=EDGE_CURVE('',#18874,#18873,#8516,.T.);
#23379=EDGE_CURVE('',#18875,#18874,#8517,.T.);
#23380=EDGE_CURVE('',#18871,#18875,#8518,.T.);
#23381=EDGE_CURVE('',#18876,#18877,#8519,.T.);
#23382=EDGE_CURVE('',#18878,#18876,#8520,.T.);
#23383=EDGE_CURVE('',#18879,#18878,#8521,.T.);
#23384=EDGE_CURVE('',#18880,#18879,#8522,.T.);
#23385=EDGE_CURVE('',#18881,#18880,#8523,.T.);
#23386=EDGE_CURVE('',#18877,#18881,#8524,.T.);
#23387=EDGE_CURVE('',#18882,#18883,#8525,.T.);
#23388=EDGE_CURVE('',#18884,#18882,#8526,.T.);
#23389=EDGE_CURVE('',#18885,#18884,#8527,.T.);
#23390=EDGE_CURVE('',#18886,#18885,#8528,.T.);
#23391=EDGE_CURVE('',#18887,#18886,#8529,.T.);
#23392=EDGE_CURVE('',#18883,#18887,#8530,.T.);
#23393=EDGE_CURVE('',#18888,#18889,#8531,.T.);
#23394=EDGE_CURVE('',#18890,#18888,#8532,.T.);
#23395=EDGE_CURVE('',#18891,#18890,#8533,.T.);
#23396=EDGE_CURVE('',#18892,#18891,#8534,.T.);
#23397=EDGE_CURVE('',#18893,#18892,#8535,.T.);
#23398=EDGE_CURVE('',#18889,#18893,#8536,.T.);
#23399=EDGE_CURVE('',#18894,#18895,#8537,.T.);
#23400=EDGE_CURVE('',#18896,#18894,#8538,.T.);
#23401=EDGE_CURVE('',#18897,#18896,#8539,.T.);
#23402=EDGE_CURVE('',#18898,#18897,#8540,.T.);
#23403=EDGE_CURVE('',#18899,#18898,#8541,.T.);
#23404=EDGE_CURVE('',#18895,#18899,#8542,.T.);
#23405=EDGE_CURVE('',#18900,#18901,#8543,.T.);
#23406=EDGE_CURVE('',#18902,#18900,#8544,.T.);
#23407=EDGE_CURVE('',#18903,#18902,#8545,.T.);
#23408=EDGE_CURVE('',#18904,#18903,#8546,.T.);
#23409=EDGE_CURVE('',#18905,#18904,#8547,.T.);
#23410=EDGE_CURVE('',#18901,#18905,#8548,.T.);
#23411=EDGE_CURVE('',#18906,#18907,#8549,.T.);
#23412=EDGE_CURVE('',#18908,#18906,#8550,.T.);
#23413=EDGE_CURVE('',#18909,#18908,#8551,.T.);
#23414=EDGE_CURVE('',#18910,#18909,#8552,.T.);
#23415=EDGE_CURVE('',#18911,#18910,#8553,.T.);
#23416=EDGE_CURVE('',#18907,#18911,#8554,.T.);
#23417=EDGE_CURVE('',#18912,#18913,#8555,.T.);
#23418=EDGE_CURVE('',#18914,#18912,#8556,.T.);
#23419=EDGE_CURVE('',#18915,#18914,#8557,.T.);
#23420=EDGE_CURVE('',#18916,#18915,#8558,.T.);
#23421=EDGE_CURVE('',#18917,#18916,#8559,.T.);
#23422=EDGE_CURVE('',#18913,#18917,#8560,.T.);
#23423=EDGE_CURVE('',#18918,#18919,#8561,.T.);
#23424=EDGE_CURVE('',#18920,#18918,#8562,.T.);
#23425=EDGE_CURVE('',#18921,#18920,#8563,.T.);
#23426=EDGE_CURVE('',#18922,#18921,#8564,.T.);
#23427=EDGE_CURVE('',#18923,#18922,#8565,.T.);
#23428=EDGE_CURVE('',#18919,#18923,#8566,.T.);
#23429=EDGE_CURVE('',#18924,#18925,#8567,.T.);
#23430=EDGE_CURVE('',#18926,#18924,#8568,.T.);
#23431=EDGE_CURVE('',#18927,#18926,#8569,.T.);
#23432=EDGE_CURVE('',#18928,#18927,#8570,.T.);
#23433=EDGE_CURVE('',#18929,#18928,#8571,.T.);
#23434=EDGE_CURVE('',#18925,#18929,#8572,.T.);
#23435=EDGE_CURVE('',#18930,#18931,#8573,.T.);
#23436=EDGE_CURVE('',#18932,#18930,#8574,.T.);
#23437=EDGE_CURVE('',#18933,#18932,#8575,.T.);
#23438=EDGE_CURVE('',#18934,#18933,#8576,.T.);
#23439=EDGE_CURVE('',#18935,#18934,#8577,.T.);
#23440=EDGE_CURVE('',#18931,#18935,#8578,.T.);
#23441=EDGE_CURVE('',#18936,#18937,#8579,.T.);
#23442=EDGE_CURVE('',#18938,#18936,#8580,.T.);
#23443=EDGE_CURVE('',#18939,#18938,#8581,.T.);
#23444=EDGE_CURVE('',#18940,#18939,#8582,.T.);
#23445=EDGE_CURVE('',#18941,#18940,#8583,.T.);
#23446=EDGE_CURVE('',#18937,#18941,#8584,.T.);
#23447=EDGE_CURVE('',#18942,#18943,#8585,.T.);
#23448=EDGE_CURVE('',#18944,#18942,#8586,.T.);
#23449=EDGE_CURVE('',#18945,#18944,#8587,.T.);
#23450=EDGE_CURVE('',#18946,#18945,#8588,.T.);
#23451=EDGE_CURVE('',#18947,#18946,#8589,.T.);
#23452=EDGE_CURVE('',#18943,#18947,#8590,.T.);
#23453=EDGE_CURVE('',#18948,#18949,#8591,.T.);
#23454=EDGE_CURVE('',#18950,#18948,#8592,.T.);
#23455=EDGE_CURVE('',#18951,#18950,#8593,.T.);
#23456=EDGE_CURVE('',#18952,#18951,#8594,.T.);
#23457=EDGE_CURVE('',#18953,#18952,#8595,.T.);
#23458=EDGE_CURVE('',#18949,#18953,#8596,.T.);
#23459=EDGE_CURVE('',#18954,#18955,#8597,.T.);
#23460=EDGE_CURVE('',#18956,#18954,#8598,.T.);
#23461=EDGE_CURVE('',#18957,#18956,#8599,.T.);
#23462=EDGE_CURVE('',#18958,#18957,#8600,.T.);
#23463=EDGE_CURVE('',#18959,#18958,#8601,.T.);
#23464=EDGE_CURVE('',#18955,#18959,#8602,.T.);
#23465=EDGE_CURVE('',#18960,#18961,#8603,.T.);
#23466=EDGE_CURVE('',#18962,#18960,#8604,.T.);
#23467=EDGE_CURVE('',#18963,#18962,#8605,.T.);
#23468=EDGE_CURVE('',#18964,#18963,#8606,.T.);
#23469=EDGE_CURVE('',#18965,#18964,#8607,.T.);
#23470=EDGE_CURVE('',#18961,#18965,#8608,.T.);
#23471=EDGE_CURVE('',#18966,#18967,#8609,.T.);
#23472=EDGE_CURVE('',#18968,#18966,#8610,.T.);
#23473=EDGE_CURVE('',#18969,#18968,#8611,.T.);
#23474=EDGE_CURVE('',#18970,#18969,#8612,.T.);
#23475=EDGE_CURVE('',#18971,#18970,#8613,.T.);
#23476=EDGE_CURVE('',#18967,#18971,#8614,.T.);
#23477=EDGE_CURVE('',#18972,#18973,#8615,.T.);
#23478=EDGE_CURVE('',#18974,#18972,#8616,.T.);
#23479=EDGE_CURVE('',#18975,#18974,#8617,.T.);
#23480=EDGE_CURVE('',#18976,#18975,#8618,.T.);
#23481=EDGE_CURVE('',#18977,#18976,#8619,.T.);
#23482=EDGE_CURVE('',#18973,#18977,#8620,.T.);
#23483=EDGE_CURVE('',#18978,#18979,#8621,.T.);
#23484=EDGE_CURVE('',#18980,#18978,#8622,.T.);
#23485=EDGE_CURVE('',#18981,#18980,#8623,.T.);
#23486=EDGE_CURVE('',#18982,#18981,#8624,.T.);
#23487=EDGE_CURVE('',#18983,#18982,#8625,.T.);
#23488=EDGE_CURVE('',#18979,#18983,#8626,.T.);
#23489=EDGE_CURVE('',#18984,#18985,#8627,.T.);
#23490=EDGE_CURVE('',#18986,#18984,#8628,.T.);
#23491=EDGE_CURVE('',#18987,#18986,#8629,.T.);
#23492=EDGE_CURVE('',#18988,#18987,#8630,.T.);
#23493=EDGE_CURVE('',#18989,#18988,#8631,.T.);
#23494=EDGE_CURVE('',#18985,#18989,#8632,.T.);
#23495=EDGE_CURVE('',#18990,#18991,#8633,.T.);
#23496=EDGE_CURVE('',#18992,#18990,#8634,.T.);
#23497=EDGE_CURVE('',#18993,#18992,#8635,.T.);
#23498=EDGE_CURVE('',#18994,#18993,#8636,.T.);
#23499=EDGE_CURVE('',#18995,#18994,#8637,.T.);
#23500=EDGE_CURVE('',#18991,#18995,#8638,.T.);
#23501=EDGE_CURVE('',#18996,#18997,#8639,.T.);
#23502=EDGE_CURVE('',#18998,#18996,#8640,.T.);
#23503=EDGE_CURVE('',#18999,#18998,#8641,.T.);
#23504=EDGE_CURVE('',#19000,#18999,#8642,.T.);
#23505=EDGE_CURVE('',#19001,#19000,#8643,.T.);
#23506=EDGE_CURVE('',#18997,#19001,#8644,.T.);
#23507=EDGE_CURVE('',#19002,#19003,#8645,.T.);
#23508=EDGE_CURVE('',#19004,#19002,#8646,.T.);
#23509=EDGE_CURVE('',#19005,#19004,#8647,.T.);
#23510=EDGE_CURVE('',#19006,#19005,#8648,.T.);
#23511=EDGE_CURVE('',#19007,#19006,#8649,.T.);
#23512=EDGE_CURVE('',#19003,#19007,#8650,.T.);
#23513=EDGE_CURVE('',#19008,#19009,#8651,.T.);
#23514=EDGE_CURVE('',#19010,#19008,#8652,.T.);
#23515=EDGE_CURVE('',#19011,#19010,#8653,.T.);
#23516=EDGE_CURVE('',#19012,#19011,#8654,.T.);
#23517=EDGE_CURVE('',#19013,#19012,#8655,.T.);
#23518=EDGE_CURVE('',#19009,#19013,#8656,.T.);
#23519=EDGE_CURVE('',#19014,#19015,#8657,.T.);
#23520=EDGE_CURVE('',#19016,#19014,#8658,.T.);
#23521=EDGE_CURVE('',#19017,#19016,#8659,.T.);
#23522=EDGE_CURVE('',#19018,#19017,#8660,.T.);
#23523=EDGE_CURVE('',#19019,#19018,#8661,.T.);
#23524=EDGE_CURVE('',#19015,#19019,#8662,.T.);
#23525=EDGE_CURVE('',#19020,#19021,#8663,.T.);
#23526=EDGE_CURVE('',#19022,#19020,#8664,.T.);
#23527=EDGE_CURVE('',#19023,#19022,#8665,.T.);
#23528=EDGE_CURVE('',#19024,#19023,#8666,.T.);
#23529=EDGE_CURVE('',#19025,#19024,#8667,.T.);
#23530=EDGE_CURVE('',#19021,#19025,#8668,.T.);
#23531=EDGE_CURVE('',#19026,#19027,#8669,.T.);
#23532=EDGE_CURVE('',#19028,#19026,#8670,.T.);
#23533=EDGE_CURVE('',#19029,#19028,#8671,.T.);
#23534=EDGE_CURVE('',#19030,#19029,#8672,.T.);
#23535=EDGE_CURVE('',#19031,#19030,#8673,.T.);
#23536=EDGE_CURVE('',#19027,#19031,#8674,.T.);
#23537=EDGE_CURVE('',#19032,#19033,#8675,.T.);
#23538=EDGE_CURVE('',#19034,#19032,#8676,.T.);
#23539=EDGE_CURVE('',#19035,#19034,#8677,.T.);
#23540=EDGE_CURVE('',#19036,#19035,#8678,.T.);
#23541=EDGE_CURVE('',#19037,#19036,#8679,.T.);
#23542=EDGE_CURVE('',#19033,#19037,#8680,.T.);
#23543=EDGE_CURVE('',#19038,#19039,#8681,.T.);
#23544=EDGE_CURVE('',#19040,#19038,#8682,.T.);
#23545=EDGE_CURVE('',#19041,#19040,#8683,.T.);
#23546=EDGE_CURVE('',#19042,#19041,#8684,.T.);
#23547=EDGE_CURVE('',#19043,#19042,#8685,.T.);
#23548=EDGE_CURVE('',#19039,#19043,#8686,.T.);
#23549=EDGE_CURVE('',#19044,#19045,#8687,.T.);
#23550=EDGE_CURVE('',#19046,#19044,#8688,.T.);
#23551=EDGE_CURVE('',#19047,#19046,#8689,.T.);
#23552=EDGE_CURVE('',#19048,#19047,#8690,.T.);
#23553=EDGE_CURVE('',#19049,#19048,#8691,.T.);
#23554=EDGE_CURVE('',#19045,#19049,#8692,.T.);
#23555=EDGE_CURVE('',#19050,#19051,#8693,.T.);
#23556=EDGE_CURVE('',#19052,#19050,#8694,.T.);
#23557=EDGE_CURVE('',#19053,#19052,#8695,.T.);
#23558=EDGE_CURVE('',#19054,#19053,#8696,.T.);
#23559=EDGE_CURVE('',#19055,#19054,#8697,.T.);
#23560=EDGE_CURVE('',#19051,#19055,#8698,.T.);
#23561=EDGE_CURVE('',#19056,#19057,#8699,.T.);
#23562=EDGE_CURVE('',#19058,#19056,#8700,.T.);
#23563=EDGE_CURVE('',#19059,#19058,#8701,.T.);
#23564=EDGE_CURVE('',#19060,#19059,#8702,.T.);
#23565=EDGE_CURVE('',#19061,#19060,#8703,.T.);
#23566=EDGE_CURVE('',#19057,#19061,#8704,.T.);
#23567=EDGE_CURVE('',#19062,#19063,#8705,.T.);
#23568=EDGE_CURVE('',#19064,#19062,#8706,.T.);
#23569=EDGE_CURVE('',#19065,#19064,#8707,.T.);
#23570=EDGE_CURVE('',#19066,#19065,#8708,.T.);
#23571=EDGE_CURVE('',#19067,#19066,#8709,.T.);
#23572=EDGE_CURVE('',#19063,#19067,#8710,.T.);
#23573=EDGE_CURVE('',#19068,#19069,#8711,.T.);
#23574=EDGE_CURVE('',#19070,#19068,#8712,.T.);
#23575=EDGE_CURVE('',#19071,#19070,#8713,.T.);
#23576=EDGE_CURVE('',#19072,#19071,#8714,.T.);
#23577=EDGE_CURVE('',#19073,#19072,#8715,.T.);
#23578=EDGE_CURVE('',#19069,#19073,#8716,.T.);
#23579=EDGE_CURVE('',#19074,#19075,#8717,.T.);
#23580=EDGE_CURVE('',#19076,#19074,#8718,.T.);
#23581=EDGE_CURVE('',#19077,#19076,#8719,.T.);
#23582=EDGE_CURVE('',#19078,#19077,#8720,.T.);
#23583=EDGE_CURVE('',#19079,#19078,#8721,.T.);
#23584=EDGE_CURVE('',#19075,#19079,#8722,.T.);
#23585=EDGE_CURVE('',#19080,#19081,#8723,.T.);
#23586=EDGE_CURVE('',#19082,#19080,#8724,.T.);
#23587=EDGE_CURVE('',#19083,#19082,#8725,.T.);
#23588=EDGE_CURVE('',#19084,#19083,#8726,.T.);
#23589=EDGE_CURVE('',#19085,#19084,#8727,.T.);
#23590=EDGE_CURVE('',#19081,#19085,#8728,.T.);
#23591=EDGE_CURVE('',#19086,#19087,#8729,.T.);
#23592=EDGE_CURVE('',#19088,#19086,#8730,.T.);
#23593=EDGE_CURVE('',#19089,#19088,#8731,.T.);
#23594=EDGE_CURVE('',#19090,#19089,#8732,.T.);
#23595=EDGE_CURVE('',#19091,#19090,#8733,.T.);
#23596=EDGE_CURVE('',#19087,#19091,#8734,.T.);
#23597=EDGE_CURVE('',#19092,#19093,#8735,.T.);
#23598=EDGE_CURVE('',#19094,#19092,#8736,.T.);
#23599=EDGE_CURVE('',#19095,#19094,#8737,.T.);
#23600=EDGE_CURVE('',#19096,#19095,#8738,.T.);
#23601=EDGE_CURVE('',#19097,#19096,#8739,.T.);
#23602=EDGE_CURVE('',#19093,#19097,#8740,.T.);
#23603=EDGE_CURVE('',#19098,#19099,#8741,.T.);
#23604=EDGE_CURVE('',#19100,#19098,#8742,.T.);
#23605=EDGE_CURVE('',#19101,#19100,#8743,.T.);
#23606=EDGE_CURVE('',#19102,#19101,#8744,.T.);
#23607=EDGE_CURVE('',#19103,#19102,#8745,.T.);
#23608=EDGE_CURVE('',#19099,#19103,#8746,.T.);
#23609=EDGE_CURVE('',#19104,#19105,#8747,.T.);
#23610=EDGE_CURVE('',#19106,#19104,#8748,.T.);
#23611=EDGE_CURVE('',#19107,#19106,#8749,.T.);
#23612=EDGE_CURVE('',#19108,#19107,#8750,.T.);
#23613=EDGE_CURVE('',#19109,#19108,#8751,.T.);
#23614=EDGE_CURVE('',#19105,#19109,#8752,.T.);
#23615=EDGE_CURVE('',#19110,#19111,#8753,.T.);
#23616=EDGE_CURVE('',#19112,#19110,#8754,.T.);
#23617=EDGE_CURVE('',#19113,#19112,#8755,.T.);
#23618=EDGE_CURVE('',#19114,#19113,#8756,.T.);
#23619=EDGE_CURVE('',#19115,#19114,#8757,.T.);
#23620=EDGE_CURVE('',#19111,#19115,#8758,.T.);
#23621=EDGE_CURVE('',#19116,#19117,#8759,.T.);
#23622=EDGE_CURVE('',#19118,#19116,#8760,.T.);
#23623=EDGE_CURVE('',#19119,#19118,#8761,.T.);
#23624=EDGE_CURVE('',#19120,#19119,#8762,.T.);
#23625=EDGE_CURVE('',#19121,#19120,#8763,.T.);
#23626=EDGE_CURVE('',#19117,#19121,#8764,.T.);
#23627=EDGE_CURVE('',#19122,#19123,#8765,.T.);
#23628=EDGE_CURVE('',#19124,#19122,#8766,.T.);
#23629=EDGE_CURVE('',#19125,#19124,#8767,.T.);
#23630=EDGE_CURVE('',#19126,#19125,#8768,.T.);
#23631=EDGE_CURVE('',#19127,#19126,#8769,.T.);
#23632=EDGE_CURVE('',#19123,#19127,#8770,.T.);
#23633=EDGE_CURVE('',#19128,#19129,#8771,.T.);
#23634=EDGE_CURVE('',#19130,#19128,#8772,.T.);
#23635=EDGE_CURVE('',#19131,#19130,#8773,.T.);
#23636=EDGE_CURVE('',#19132,#19131,#8774,.T.);
#23637=EDGE_CURVE('',#19133,#19132,#8775,.T.);
#23638=EDGE_CURVE('',#19129,#19133,#8776,.T.);
#23639=EDGE_CURVE('',#19134,#19135,#8777,.T.);
#23640=EDGE_CURVE('',#19136,#19134,#8778,.T.);
#23641=EDGE_CURVE('',#19137,#19136,#8779,.T.);
#23642=EDGE_CURVE('',#19138,#19137,#8780,.T.);
#23643=EDGE_CURVE('',#19139,#19138,#8781,.T.);
#23644=EDGE_CURVE('',#19135,#19139,#8782,.T.);
#23645=EDGE_CURVE('',#19140,#19141,#8783,.T.);
#23646=EDGE_CURVE('',#19142,#19140,#8784,.T.);
#23647=EDGE_CURVE('',#19143,#19142,#8785,.T.);
#23648=EDGE_CURVE('',#19144,#19143,#8786,.T.);
#23649=EDGE_CURVE('',#19145,#19144,#8787,.T.);
#23650=EDGE_CURVE('',#19141,#19145,#8788,.T.);
#23651=EDGE_CURVE('',#19146,#19147,#8789,.T.);
#23652=EDGE_CURVE('',#19148,#19146,#8790,.T.);
#23653=EDGE_CURVE('',#19149,#19148,#8791,.T.);
#23654=EDGE_CURVE('',#19150,#19149,#8792,.T.);
#23655=EDGE_CURVE('',#19151,#19150,#8793,.T.);
#23656=EDGE_CURVE('',#19147,#19151,#8794,.T.);
#23657=EDGE_CURVE('',#19152,#19153,#8795,.T.);
#23658=EDGE_CURVE('',#19154,#19152,#8796,.T.);
#23659=EDGE_CURVE('',#19155,#19154,#8797,.T.);
#23660=EDGE_CURVE('',#19156,#19155,#8798,.T.);
#23661=EDGE_CURVE('',#19157,#19156,#8799,.T.);
#23662=EDGE_CURVE('',#19153,#19157,#8800,.T.);
#23663=EDGE_CURVE('',#19158,#19159,#8801,.T.);
#23664=EDGE_CURVE('',#19160,#19158,#8802,.T.);
#23665=EDGE_CURVE('',#19161,#19160,#8803,.T.);
#23666=EDGE_CURVE('',#19162,#19161,#8804,.T.);
#23667=EDGE_CURVE('',#19163,#19162,#8805,.T.);
#23668=EDGE_CURVE('',#19159,#19163,#8806,.T.);
#23669=EDGE_CURVE('',#19164,#19165,#8807,.T.);
#23670=EDGE_CURVE('',#19166,#19164,#8808,.T.);
#23671=EDGE_CURVE('',#19167,#19166,#8809,.T.);
#23672=EDGE_CURVE('',#19168,#19167,#8810,.T.);
#23673=EDGE_CURVE('',#19169,#19168,#8811,.T.);
#23674=EDGE_CURVE('',#19165,#19169,#8812,.T.);
#23675=EDGE_CURVE('',#19170,#19171,#8813,.T.);
#23676=EDGE_CURVE('',#19172,#19170,#8814,.T.);
#23677=EDGE_CURVE('',#19173,#19172,#8815,.T.);
#23678=EDGE_CURVE('',#19174,#19173,#8816,.T.);
#23679=EDGE_CURVE('',#19175,#19174,#8817,.T.);
#23680=EDGE_CURVE('',#19171,#19175,#8818,.T.);
#23681=EDGE_CURVE('',#19176,#19177,#8819,.T.);
#23682=EDGE_CURVE('',#19178,#19176,#8820,.T.);
#23683=EDGE_CURVE('',#19179,#19178,#8821,.T.);
#23684=EDGE_CURVE('',#19180,#19179,#8822,.T.);
#23685=EDGE_CURVE('',#19181,#19180,#8823,.T.);
#23686=EDGE_CURVE('',#19177,#19181,#8824,.T.);
#23687=EDGE_CURVE('',#19182,#19183,#8825,.T.);
#23688=EDGE_CURVE('',#19184,#19182,#8826,.T.);
#23689=EDGE_CURVE('',#19185,#19184,#8827,.T.);
#23690=EDGE_CURVE('',#19186,#19185,#8828,.T.);
#23691=EDGE_CURVE('',#19187,#19186,#8829,.T.);
#23692=EDGE_CURVE('',#19183,#19187,#8830,.T.);
#23693=EDGE_CURVE('',#19188,#19189,#8831,.T.);
#23694=EDGE_CURVE('',#19190,#19188,#8832,.T.);
#23695=EDGE_CURVE('',#19191,#19190,#8833,.T.);
#23696=EDGE_CURVE('',#19192,#19191,#8834,.T.);
#23697=EDGE_CURVE('',#19193,#19192,#8835,.T.);
#23698=EDGE_CURVE('',#19189,#19193,#8836,.T.);
#23699=EDGE_CURVE('',#19194,#19195,#8837,.T.);
#23700=EDGE_CURVE('',#19196,#19194,#8838,.T.);
#23701=EDGE_CURVE('',#19197,#19196,#8839,.T.);
#23702=EDGE_CURVE('',#19198,#19197,#8840,.T.);
#23703=EDGE_CURVE('',#19199,#19198,#8841,.T.);
#23704=EDGE_CURVE('',#19195,#19199,#8842,.T.);
#23705=EDGE_CURVE('',#19200,#19201,#8843,.T.);
#23706=EDGE_CURVE('',#19202,#19200,#8844,.T.);
#23707=EDGE_CURVE('',#19203,#19202,#8845,.T.);
#23708=EDGE_CURVE('',#19204,#19203,#8846,.T.);
#23709=EDGE_CURVE('',#19205,#19204,#8847,.T.);
#23710=EDGE_CURVE('',#19201,#19205,#8848,.T.);
#23711=EDGE_CURVE('',#19206,#19207,#8849,.T.);
#23712=EDGE_CURVE('',#19208,#19206,#8850,.T.);
#23713=EDGE_CURVE('',#19209,#19208,#8851,.T.);
#23714=EDGE_CURVE('',#19210,#19209,#8852,.T.);
#23715=EDGE_CURVE('',#19211,#19210,#8853,.T.);
#23716=EDGE_CURVE('',#19207,#19211,#8854,.T.);
#23717=EDGE_CURVE('',#19212,#19213,#8855,.T.);
#23718=EDGE_CURVE('',#19214,#19212,#8856,.T.);
#23719=EDGE_CURVE('',#19215,#19214,#8857,.T.);
#23720=EDGE_CURVE('',#19216,#19215,#8858,.T.);
#23721=EDGE_CURVE('',#19217,#19216,#8859,.T.);
#23722=EDGE_CURVE('',#19213,#19217,#8860,.T.);
#23723=EDGE_CURVE('',#19218,#19219,#8861,.T.);
#23724=EDGE_CURVE('',#19220,#19218,#8862,.T.);
#23725=EDGE_CURVE('',#19221,#19220,#8863,.T.);
#23726=EDGE_CURVE('',#19222,#19221,#8864,.T.);
#23727=EDGE_CURVE('',#19223,#19222,#8865,.T.);
#23728=EDGE_CURVE('',#19219,#19223,#8866,.T.);
#23729=EDGE_CURVE('',#19224,#19225,#8867,.T.);
#23730=EDGE_CURVE('',#19226,#19224,#8868,.T.);
#23731=EDGE_CURVE('',#19227,#19226,#8869,.T.);
#23732=EDGE_CURVE('',#19228,#19227,#8870,.T.);
#23733=EDGE_CURVE('',#19229,#19228,#8871,.T.);
#23734=EDGE_CURVE('',#19225,#19229,#8872,.T.);
#23735=EDGE_CURVE('',#19230,#19231,#8873,.T.);
#23736=EDGE_CURVE('',#19232,#19230,#8874,.T.);
#23737=EDGE_CURVE('',#19233,#19232,#8875,.T.);
#23738=EDGE_CURVE('',#19234,#19233,#8876,.T.);
#23739=EDGE_CURVE('',#19235,#19234,#8877,.T.);
#23740=EDGE_CURVE('',#19231,#19235,#8878,.T.);
#23741=EDGE_CURVE('',#19236,#19237,#8879,.T.);
#23742=EDGE_CURVE('',#19238,#19236,#8880,.T.);
#23743=EDGE_CURVE('',#19239,#19238,#8881,.T.);
#23744=EDGE_CURVE('',#19240,#19239,#8882,.T.);
#23745=EDGE_CURVE('',#19241,#19240,#8883,.T.);
#23746=EDGE_CURVE('',#19237,#19241,#8884,.T.);
#23747=EDGE_CURVE('',#19242,#19243,#8885,.T.);
#23748=EDGE_CURVE('',#19244,#19242,#8886,.T.);
#23749=EDGE_CURVE('',#19245,#19244,#8887,.T.);
#23750=EDGE_CURVE('',#19246,#19245,#8888,.T.);
#23751=EDGE_CURVE('',#19247,#19246,#8889,.T.);
#23752=EDGE_CURVE('',#19243,#19247,#8890,.T.);
#23753=EDGE_CURVE('',#19248,#19249,#8891,.T.);
#23754=EDGE_CURVE('',#19250,#19248,#8892,.T.);
#23755=EDGE_CURVE('',#19251,#19250,#8893,.T.);
#23756=EDGE_CURVE('',#19252,#19251,#8894,.T.);
#23757=EDGE_CURVE('',#19253,#19252,#8895,.T.);
#23758=EDGE_CURVE('',#19249,#19253,#8896,.T.);
#23759=EDGE_CURVE('',#19254,#19255,#8897,.T.);
#23760=EDGE_CURVE('',#19256,#19254,#8898,.T.);
#23761=EDGE_CURVE('',#19257,#19256,#8899,.T.);
#23762=EDGE_CURVE('',#19258,#19257,#8900,.T.);
#23763=EDGE_CURVE('',#19259,#19258,#8901,.T.);
#23764=EDGE_CURVE('',#19255,#19259,#8902,.T.);
#23765=EDGE_CURVE('',#19260,#19261,#8903,.T.);
#23766=EDGE_CURVE('',#19262,#19260,#8904,.T.);
#23767=EDGE_CURVE('',#19263,#19262,#8905,.T.);
#23768=EDGE_CURVE('',#19264,#19263,#8906,.T.);
#23769=EDGE_CURVE('',#19265,#19264,#8907,.T.);
#23770=EDGE_CURVE('',#19261,#19265,#8908,.T.);
#23771=EDGE_CURVE('',#19266,#19267,#8909,.T.);
#23772=EDGE_CURVE('',#19268,#19266,#8910,.T.);
#23773=EDGE_CURVE('',#19269,#19268,#8911,.T.);
#23774=EDGE_CURVE('',#19270,#19269,#8912,.T.);
#23775=EDGE_CURVE('',#19271,#19270,#8913,.T.);
#23776=EDGE_CURVE('',#19267,#19271,#8914,.T.);
#23777=EDGE_CURVE('',#19272,#19273,#8915,.T.);
#23778=EDGE_CURVE('',#19274,#19272,#8916,.T.);
#23779=EDGE_CURVE('',#19275,#19274,#8917,.T.);
#23780=EDGE_CURVE('',#19276,#19275,#8918,.T.);
#23781=EDGE_CURVE('',#19277,#19276,#8919,.T.);
#23782=EDGE_CURVE('',#19273,#19277,#8920,.T.);
#23783=EDGE_CURVE('',#19278,#19279,#8921,.T.);
#23784=EDGE_CURVE('',#19280,#19278,#8922,.T.);
#23785=EDGE_CURVE('',#19281,#19280,#8923,.T.);
#23786=EDGE_CURVE('',#19282,#19281,#8924,.T.);
#23787=EDGE_CURVE('',#19283,#19282,#8925,.T.);
#23788=EDGE_CURVE('',#19279,#19283,#8926,.T.);
#23789=EDGE_CURVE('',#19284,#19285,#8927,.T.);
#23790=EDGE_CURVE('',#19286,#19284,#8928,.T.);
#23791=EDGE_CURVE('',#19287,#19286,#8929,.T.);
#23792=EDGE_CURVE('',#19288,#19287,#8930,.T.);
#23793=EDGE_CURVE('',#19289,#19288,#8931,.T.);
#23794=EDGE_CURVE('',#19285,#19289,#8932,.T.);
#23795=EDGE_CURVE('',#19290,#19291,#8933,.T.);
#23796=EDGE_CURVE('',#19292,#19290,#8934,.T.);
#23797=EDGE_CURVE('',#19293,#19292,#8935,.T.);
#23798=EDGE_CURVE('',#19294,#19293,#8936,.T.);
#23799=EDGE_CURVE('',#19295,#19294,#8937,.T.);
#23800=EDGE_CURVE('',#19291,#19295,#8938,.T.);
#23801=EDGE_CURVE('',#19296,#19297,#8939,.T.);
#23802=EDGE_CURVE('',#19298,#19296,#8940,.T.);
#23803=EDGE_CURVE('',#19299,#19298,#8941,.T.);
#23804=EDGE_CURVE('',#19300,#19299,#8942,.T.);
#23805=EDGE_CURVE('',#19301,#19300,#8943,.T.);
#23806=EDGE_CURVE('',#19297,#19301,#8944,.T.);
#23807=EDGE_CURVE('',#19302,#19303,#8945,.T.);
#23808=EDGE_CURVE('',#19304,#19302,#8946,.T.);
#23809=EDGE_CURVE('',#19305,#19304,#8947,.T.);
#23810=EDGE_CURVE('',#19306,#19305,#8948,.T.);
#23811=EDGE_CURVE('',#19307,#19306,#8949,.T.);
#23812=EDGE_CURVE('',#19303,#19307,#8950,.T.);
#23813=EDGE_CURVE('',#19308,#19309,#8951,.T.);
#23814=EDGE_CURVE('',#19310,#19308,#8952,.T.);
#23815=EDGE_CURVE('',#19311,#19310,#8953,.T.);
#23816=EDGE_CURVE('',#19312,#19311,#8954,.T.);
#23817=EDGE_CURVE('',#19313,#19312,#8955,.T.);
#23818=EDGE_CURVE('',#19309,#19313,#8956,.T.);
#23819=EDGE_CURVE('',#19314,#19315,#8957,.T.);
#23820=EDGE_CURVE('',#19316,#19314,#8958,.T.);
#23821=EDGE_CURVE('',#19317,#19316,#8959,.T.);
#23822=EDGE_CURVE('',#19318,#19317,#8960,.T.);
#23823=EDGE_CURVE('',#19319,#19318,#8961,.T.);
#23824=EDGE_CURVE('',#19315,#19319,#8962,.T.);
#23825=EDGE_CURVE('',#19320,#19321,#8963,.T.);
#23826=EDGE_CURVE('',#19322,#19320,#8964,.T.);
#23827=EDGE_CURVE('',#19323,#19322,#8965,.T.);
#23828=EDGE_CURVE('',#19324,#19323,#8966,.T.);
#23829=EDGE_CURVE('',#19325,#19324,#8967,.T.);
#23830=EDGE_CURVE('',#19321,#19325,#8968,.T.);
#23831=EDGE_CURVE('',#19326,#19327,#8969,.T.);
#23832=EDGE_CURVE('',#19328,#19326,#8970,.T.);
#23833=EDGE_CURVE('',#19329,#19328,#8971,.T.);
#23834=EDGE_CURVE('',#19330,#19329,#8972,.T.);
#23835=EDGE_CURVE('',#19331,#19330,#8973,.T.);
#23836=EDGE_CURVE('',#19327,#19331,#8974,.T.);
#23837=EDGE_CURVE('',#19332,#19333,#8975,.T.);
#23838=EDGE_CURVE('',#19334,#19332,#8976,.T.);
#23839=EDGE_CURVE('',#19335,#19334,#8977,.T.);
#23840=EDGE_CURVE('',#19336,#19335,#8978,.T.);
#23841=EDGE_CURVE('',#19337,#19336,#8979,.T.);
#23842=EDGE_CURVE('',#19333,#19337,#8980,.T.);
#23843=EDGE_CURVE('',#19338,#19339,#8981,.T.);
#23844=EDGE_CURVE('',#19340,#19338,#8982,.T.);
#23845=EDGE_CURVE('',#19341,#19340,#8983,.T.);
#23846=EDGE_CURVE('',#19342,#19341,#8984,.T.);
#23847=EDGE_CURVE('',#19343,#19342,#8985,.T.);
#23848=EDGE_CURVE('',#19339,#19343,#8986,.T.);
#23849=EDGE_CURVE('',#19344,#19345,#8987,.T.);
#23850=EDGE_CURVE('',#19346,#19344,#8988,.T.);
#23851=EDGE_CURVE('',#19347,#19346,#8989,.T.);
#23852=EDGE_CURVE('',#19348,#19347,#8990,.T.);
#23853=EDGE_CURVE('',#19349,#19348,#8991,.T.);
#23854=EDGE_CURVE('',#19345,#19349,#8992,.T.);
#23855=EDGE_CURVE('',#19350,#19351,#8993,.T.);
#23856=EDGE_CURVE('',#19352,#19350,#8994,.T.);
#23857=EDGE_CURVE('',#19353,#19352,#8995,.T.);
#23858=EDGE_CURVE('',#19354,#19353,#8996,.T.);
#23859=EDGE_CURVE('',#19355,#19354,#8997,.T.);
#23860=EDGE_CURVE('',#19351,#19355,#8998,.T.);
#23861=EDGE_CURVE('',#19356,#19357,#8999,.T.);
#23862=EDGE_CURVE('',#19358,#19356,#9000,.T.);
#23863=EDGE_CURVE('',#19359,#19358,#9001,.T.);
#23864=EDGE_CURVE('',#19360,#19359,#9002,.T.);
#23865=EDGE_CURVE('',#19361,#19360,#9003,.T.);
#23866=EDGE_CURVE('',#19357,#19361,#9004,.T.);
#23867=EDGE_CURVE('',#19362,#19363,#9005,.T.);
#23868=EDGE_CURVE('',#19364,#19362,#9006,.T.);
#23869=EDGE_CURVE('',#19365,#19364,#9007,.T.);
#23870=EDGE_CURVE('',#19366,#19365,#9008,.T.);
#23871=EDGE_CURVE('',#19367,#19366,#9009,.T.);
#23872=EDGE_CURVE('',#19363,#19367,#9010,.T.);
#23873=EDGE_CURVE('',#19368,#19369,#9011,.T.);
#23874=EDGE_CURVE('',#19370,#19368,#9012,.T.);
#23875=EDGE_CURVE('',#19371,#19370,#9013,.T.);
#23876=EDGE_CURVE('',#19372,#19371,#9014,.T.);
#23877=EDGE_CURVE('',#19373,#19372,#9015,.T.);
#23878=EDGE_CURVE('',#19369,#19373,#9016,.T.);
#23879=EDGE_CURVE('',#19374,#19375,#9017,.T.);
#23880=EDGE_CURVE('',#19376,#19374,#9018,.T.);
#23881=EDGE_CURVE('',#19377,#19376,#9019,.T.);
#23882=EDGE_CURVE('',#19378,#19377,#9020,.T.);
#23883=EDGE_CURVE('',#19379,#19378,#9021,.T.);
#23884=EDGE_CURVE('',#19375,#19379,#9022,.T.);
#23885=EDGE_CURVE('',#19380,#19381,#9023,.T.);
#23886=EDGE_CURVE('',#19382,#19380,#9024,.T.);
#23887=EDGE_CURVE('',#19383,#19382,#9025,.T.);
#23888=EDGE_CURVE('',#19384,#19383,#9026,.T.);
#23889=EDGE_CURVE('',#19385,#19384,#9027,.T.);
#23890=EDGE_CURVE('',#19381,#19385,#9028,.T.);
#23891=EDGE_CURVE('',#19386,#19387,#9029,.T.);
#23892=EDGE_CURVE('',#19388,#19386,#9030,.T.);
#23893=EDGE_CURVE('',#19389,#19388,#9031,.T.);
#23894=EDGE_CURVE('',#19390,#19389,#9032,.T.);
#23895=EDGE_CURVE('',#19391,#19390,#9033,.T.);
#23896=EDGE_CURVE('',#19387,#19391,#9034,.T.);
#23897=EDGE_CURVE('',#19392,#19393,#9035,.T.);
#23898=EDGE_CURVE('',#19394,#19392,#9036,.T.);
#23899=EDGE_CURVE('',#19395,#19394,#9037,.T.);
#23900=EDGE_CURVE('',#19396,#19395,#9038,.T.);
#23901=EDGE_CURVE('',#19397,#19396,#9039,.T.);
#23902=EDGE_CURVE('',#19393,#19397,#9040,.T.);
#23903=EDGE_CURVE('',#19398,#19399,#9041,.T.);
#23904=EDGE_CURVE('',#19400,#19398,#9042,.T.);
#23905=EDGE_CURVE('',#19401,#19400,#9043,.T.);
#23906=EDGE_CURVE('',#19402,#19401,#9044,.T.);
#23907=EDGE_CURVE('',#19403,#19402,#9045,.T.);
#23908=EDGE_CURVE('',#19399,#19403,#9046,.T.);
#23909=EDGE_CURVE('',#19404,#19405,#9047,.T.);
#23910=EDGE_CURVE('',#19406,#19404,#9048,.T.);
#23911=EDGE_CURVE('',#19407,#19406,#9049,.T.);
#23912=EDGE_CURVE('',#19408,#19407,#9050,.T.);
#23913=EDGE_CURVE('',#19409,#19408,#9051,.T.);
#23914=EDGE_CURVE('',#19405,#19409,#9052,.T.);
#23915=EDGE_CURVE('',#19410,#19411,#9053,.T.);
#23916=EDGE_CURVE('',#19412,#19410,#9054,.T.);
#23917=EDGE_CURVE('',#19413,#19412,#9055,.T.);
#23918=EDGE_CURVE('',#19414,#19413,#9056,.T.);
#23919=EDGE_CURVE('',#19415,#19414,#9057,.T.);
#23920=EDGE_CURVE('',#19411,#19415,#9058,.T.);
#23921=EDGE_CURVE('',#19416,#19417,#9059,.T.);
#23922=EDGE_CURVE('',#19418,#19416,#9060,.T.);
#23923=EDGE_CURVE('',#19419,#19418,#9061,.T.);
#23924=EDGE_CURVE('',#19420,#19419,#9062,.T.);
#23925=EDGE_CURVE('',#19421,#19420,#9063,.T.);
#23926=EDGE_CURVE('',#19417,#19421,#9064,.T.);
#23927=EDGE_CURVE('',#19422,#19423,#9065,.T.);
#23928=EDGE_CURVE('',#19424,#19422,#9066,.T.);
#23929=EDGE_CURVE('',#19425,#19424,#9067,.T.);
#23930=EDGE_CURVE('',#19426,#19425,#9068,.T.);
#23931=EDGE_CURVE('',#19427,#19426,#9069,.T.);
#23932=EDGE_CURVE('',#19423,#19427,#9070,.T.);
#23933=EDGE_CURVE('',#19428,#19429,#9071,.T.);
#23934=EDGE_CURVE('',#19430,#19428,#9072,.T.);
#23935=EDGE_CURVE('',#19431,#19430,#9073,.T.);
#23936=EDGE_CURVE('',#19432,#19431,#9074,.T.);
#23937=EDGE_CURVE('',#19433,#19432,#9075,.T.);
#23938=EDGE_CURVE('',#19429,#19433,#9076,.T.);
#23939=EDGE_CURVE('',#19434,#19435,#9077,.T.);
#23940=EDGE_CURVE('',#19436,#19434,#9078,.T.);
#23941=EDGE_CURVE('',#19437,#19436,#9079,.T.);
#23942=EDGE_CURVE('',#19438,#19437,#9080,.T.);
#23943=EDGE_CURVE('',#19439,#19438,#9081,.T.);
#23944=EDGE_CURVE('',#19435,#19439,#9082,.T.);
#23945=EDGE_CURVE('',#19440,#19441,#9083,.T.);
#23946=EDGE_CURVE('',#19442,#19440,#9084,.T.);
#23947=EDGE_CURVE('',#19443,#19442,#9085,.T.);
#23948=EDGE_CURVE('',#19444,#19443,#9086,.T.);
#23949=EDGE_CURVE('',#19445,#19444,#9087,.T.);
#23950=EDGE_CURVE('',#19441,#19445,#9088,.T.);
#23951=EDGE_CURVE('',#19446,#19447,#9089,.T.);
#23952=EDGE_CURVE('',#19448,#19446,#9090,.T.);
#23953=EDGE_CURVE('',#19449,#19448,#9091,.T.);
#23954=EDGE_CURVE('',#19450,#19449,#9092,.T.);
#23955=EDGE_CURVE('',#19451,#19450,#9093,.T.);
#23956=EDGE_CURVE('',#19447,#19451,#9094,.T.);
#23957=EDGE_CURVE('',#19452,#19453,#9095,.T.);
#23958=EDGE_CURVE('',#19454,#19452,#9096,.T.);
#23959=EDGE_CURVE('',#19455,#19454,#9097,.T.);
#23960=EDGE_CURVE('',#19456,#19455,#9098,.T.);
#23961=EDGE_CURVE('',#19457,#19456,#9099,.T.);
#23962=EDGE_CURVE('',#19453,#19457,#9100,.T.);
#23963=EDGE_CURVE('',#19458,#19459,#9101,.T.);
#23964=EDGE_CURVE('',#19460,#19458,#9102,.T.);
#23965=EDGE_CURVE('',#19461,#19460,#9103,.T.);
#23966=EDGE_CURVE('',#19462,#19461,#9104,.T.);
#23967=EDGE_CURVE('',#19463,#19462,#9105,.T.);
#23968=EDGE_CURVE('',#19459,#19463,#9106,.T.);
#23969=EDGE_CURVE('',#19464,#19465,#9107,.T.);
#23970=EDGE_CURVE('',#19466,#19464,#9108,.T.);
#23971=EDGE_CURVE('',#19467,#19466,#9109,.T.);
#23972=EDGE_CURVE('',#19468,#19467,#9110,.T.);
#23973=EDGE_CURVE('',#19469,#19468,#9111,.T.);
#23974=EDGE_CURVE('',#19465,#19469,#9112,.T.);
#23975=EDGE_CURVE('',#19470,#19471,#9113,.T.);
#23976=EDGE_CURVE('',#19472,#19470,#9114,.T.);
#23977=EDGE_CURVE('',#19473,#19472,#9115,.T.);
#23978=EDGE_CURVE('',#19474,#19473,#9116,.T.);
#23979=EDGE_CURVE('',#19475,#19474,#9117,.T.);
#23980=EDGE_CURVE('',#19471,#19475,#9118,.T.);
#23981=EDGE_CURVE('',#19476,#19477,#9119,.T.);
#23982=EDGE_CURVE('',#19478,#19476,#9120,.T.);
#23983=EDGE_CURVE('',#19479,#19478,#9121,.T.);
#23984=EDGE_CURVE('',#19480,#19479,#9122,.T.);
#23985=EDGE_CURVE('',#19481,#19480,#9123,.T.);
#23986=EDGE_CURVE('',#19477,#19481,#9124,.T.);
#23987=EDGE_CURVE('',#19482,#19483,#9125,.T.);
#23988=EDGE_CURVE('',#19484,#19482,#9126,.T.);
#23989=EDGE_CURVE('',#19485,#19484,#9127,.T.);
#23990=EDGE_CURVE('',#19486,#19485,#9128,.T.);
#23991=EDGE_CURVE('',#19487,#19486,#9129,.T.);
#23992=EDGE_CURVE('',#19483,#19487,#9130,.T.);
#23993=EDGE_CURVE('',#19488,#19489,#9131,.T.);
#23994=EDGE_CURVE('',#19490,#19488,#9132,.T.);
#23995=EDGE_CURVE('',#19491,#19490,#9133,.T.);
#23996=EDGE_CURVE('',#19492,#19491,#9134,.T.);
#23997=EDGE_CURVE('',#19493,#19492,#9135,.T.);
#23998=EDGE_CURVE('',#19489,#19493,#9136,.T.);
#23999=EDGE_CURVE('',#19494,#19495,#9137,.T.);
#24000=EDGE_CURVE('',#19496,#19494,#9138,.T.);
#24001=EDGE_CURVE('',#19497,#19496,#9139,.T.);
#24002=EDGE_CURVE('',#19498,#19497,#9140,.T.);
#24003=EDGE_CURVE('',#19499,#19498,#9141,.T.);
#24004=EDGE_CURVE('',#19495,#19499,#9142,.T.);
#24005=EDGE_CURVE('',#19500,#19501,#9143,.T.);
#24006=EDGE_CURVE('',#19502,#19500,#9144,.T.);
#24007=EDGE_CURVE('',#19503,#19502,#9145,.T.);
#24008=EDGE_CURVE('',#19504,#19503,#9146,.T.);
#24009=EDGE_CURVE('',#19505,#19504,#9147,.T.);
#24010=EDGE_CURVE('',#19501,#19505,#9148,.T.);
#24011=EDGE_CURVE('',#19506,#19507,#9149,.T.);
#24012=EDGE_CURVE('',#19508,#19506,#9150,.T.);
#24013=EDGE_CURVE('',#19509,#19508,#9151,.T.);
#24014=EDGE_CURVE('',#19510,#19509,#9152,.T.);
#24015=EDGE_CURVE('',#19511,#19510,#9153,.T.);
#24016=EDGE_CURVE('',#19507,#19511,#9154,.T.);
#24017=EDGE_CURVE('',#19512,#19513,#9155,.T.);
#24018=EDGE_CURVE('',#19514,#19512,#9156,.T.);
#24019=EDGE_CURVE('',#19515,#19514,#9157,.T.);
#24020=EDGE_CURVE('',#19516,#19515,#9158,.T.);
#24021=EDGE_CURVE('',#19517,#19516,#9159,.T.);
#24022=EDGE_CURVE('',#19513,#19517,#9160,.T.);
#24023=EDGE_CURVE('',#19518,#19519,#9161,.T.);
#24024=EDGE_CURVE('',#19520,#19518,#9162,.T.);
#24025=EDGE_CURVE('',#19521,#19520,#9163,.T.);
#24026=EDGE_CURVE('',#19522,#19521,#9164,.T.);
#24027=EDGE_CURVE('',#19523,#19522,#9165,.T.);
#24028=EDGE_CURVE('',#19519,#19523,#9166,.T.);
#24029=EDGE_CURVE('',#19524,#19525,#9167,.T.);
#24030=EDGE_CURVE('',#19526,#19524,#9168,.T.);
#24031=EDGE_CURVE('',#19527,#19526,#9169,.T.);
#24032=EDGE_CURVE('',#19528,#19527,#9170,.T.);
#24033=EDGE_CURVE('',#19529,#19528,#9171,.T.);
#24034=EDGE_CURVE('',#19525,#19529,#9172,.T.);
#24035=EDGE_CURVE('',#19530,#19531,#9173,.T.);
#24036=EDGE_CURVE('',#19532,#19530,#9174,.T.);
#24037=EDGE_CURVE('',#19533,#19532,#9175,.T.);
#24038=EDGE_CURVE('',#19534,#19533,#9176,.T.);
#24039=EDGE_CURVE('',#19535,#19534,#9177,.T.);
#24040=EDGE_CURVE('',#19531,#19535,#9178,.T.);
#24041=EDGE_CURVE('',#19536,#19537,#9179,.T.);
#24042=EDGE_CURVE('',#19538,#19536,#9180,.T.);
#24043=EDGE_CURVE('',#19539,#19538,#9181,.T.);
#24044=EDGE_CURVE('',#19540,#19539,#9182,.T.);
#24045=EDGE_CURVE('',#19541,#19540,#9183,.T.);
#24046=EDGE_CURVE('',#19537,#19541,#9184,.T.);
#24047=EDGE_CURVE('',#19542,#19543,#9185,.T.);
#24048=EDGE_CURVE('',#19544,#19542,#9186,.T.);
#24049=EDGE_CURVE('',#19545,#19544,#9187,.T.);
#24050=EDGE_CURVE('',#19546,#19545,#9188,.T.);
#24051=EDGE_CURVE('',#19547,#19546,#9189,.T.);
#24052=EDGE_CURVE('',#19543,#19547,#9190,.T.);
#24053=EDGE_CURVE('',#19548,#19549,#9191,.T.);
#24054=EDGE_CURVE('',#19550,#19548,#9192,.T.);
#24055=EDGE_CURVE('',#19551,#19550,#9193,.T.);
#24056=EDGE_CURVE('',#19552,#19551,#9194,.T.);
#24057=EDGE_CURVE('',#19553,#19552,#9195,.T.);
#24058=EDGE_CURVE('',#19549,#19553,#9196,.T.);
#24059=EDGE_CURVE('',#19554,#19555,#9197,.T.);
#24060=EDGE_CURVE('',#19556,#19554,#9198,.T.);
#24061=EDGE_CURVE('',#19557,#19556,#9199,.T.);
#24062=EDGE_CURVE('',#19558,#19557,#9200,.T.);
#24063=EDGE_CURVE('',#19559,#19558,#9201,.T.);
#24064=EDGE_CURVE('',#19555,#19559,#9202,.T.);
#24065=EDGE_CURVE('',#19560,#19561,#9203,.T.);
#24066=EDGE_CURVE('',#19562,#19560,#9204,.T.);
#24067=EDGE_CURVE('',#19563,#19562,#9205,.T.);
#24068=EDGE_CURVE('',#19564,#19563,#9206,.T.);
#24069=EDGE_CURVE('',#19565,#19564,#9207,.T.);
#24070=EDGE_CURVE('',#19561,#19565,#9208,.T.);
#24071=EDGE_CURVE('',#19566,#19567,#9209,.T.);
#24072=EDGE_CURVE('',#19568,#19566,#9210,.T.);
#24073=EDGE_CURVE('',#19569,#19568,#9211,.T.);
#24074=EDGE_CURVE('',#19570,#19569,#9212,.T.);
#24075=EDGE_CURVE('',#19571,#19570,#9213,.T.);
#24076=EDGE_CURVE('',#19567,#19571,#9214,.T.);
#24077=EDGE_CURVE('',#19572,#19573,#9215,.T.);
#24078=EDGE_CURVE('',#19574,#19572,#9216,.T.);
#24079=EDGE_CURVE('',#19575,#19574,#9217,.T.);
#24080=EDGE_CURVE('',#19576,#19575,#9218,.T.);
#24081=EDGE_CURVE('',#19577,#19576,#9219,.T.);
#24082=EDGE_CURVE('',#19573,#19577,#9220,.T.);
#24083=EDGE_CURVE('',#19578,#19579,#9221,.T.);
#24084=EDGE_CURVE('',#19580,#19578,#9222,.T.);
#24085=EDGE_CURVE('',#19581,#19580,#9223,.T.);
#24086=EDGE_CURVE('',#19582,#19581,#9224,.T.);
#24087=EDGE_CURVE('',#19583,#19582,#9225,.T.);
#24088=EDGE_CURVE('',#19579,#19583,#9226,.T.);
#24089=EDGE_CURVE('',#19584,#19585,#9227,.T.);
#24090=EDGE_CURVE('',#19586,#19584,#9228,.T.);
#24091=EDGE_CURVE('',#19587,#19586,#9229,.T.);
#24092=EDGE_CURVE('',#19588,#19587,#9230,.T.);
#24093=EDGE_CURVE('',#19589,#19588,#9231,.T.);
#24094=EDGE_CURVE('',#19585,#19589,#9232,.T.);
#24095=EDGE_CURVE('',#19590,#19591,#9233,.T.);
#24096=EDGE_CURVE('',#19592,#19590,#9234,.T.);
#24097=EDGE_CURVE('',#19593,#19592,#9235,.T.);
#24098=EDGE_CURVE('',#19594,#19593,#9236,.T.);
#24099=EDGE_CURVE('',#19595,#19594,#9237,.T.);
#24100=EDGE_CURVE('',#19591,#19595,#9238,.T.);
#24101=EDGE_CURVE('',#19596,#19597,#9239,.T.);
#24102=EDGE_CURVE('',#19598,#19596,#9240,.T.);
#24103=EDGE_CURVE('',#19599,#19598,#9241,.T.);
#24104=EDGE_CURVE('',#19600,#19599,#9242,.T.);
#24105=EDGE_CURVE('',#19601,#19600,#9243,.T.);
#24106=EDGE_CURVE('',#19597,#19601,#9244,.T.);
#24107=EDGE_CURVE('',#19602,#19603,#9245,.T.);
#24108=EDGE_CURVE('',#19604,#19602,#9246,.T.);
#24109=EDGE_CURVE('',#19605,#19604,#9247,.T.);
#24110=EDGE_CURVE('',#19606,#19605,#9248,.T.);
#24111=EDGE_CURVE('',#19607,#19606,#9249,.T.);
#24112=EDGE_CURVE('',#19603,#19607,#9250,.T.);
#24113=EDGE_CURVE('',#19608,#19609,#9251,.T.);
#24114=EDGE_CURVE('',#19610,#19608,#9252,.T.);
#24115=EDGE_CURVE('',#19611,#19610,#9253,.T.);
#24116=EDGE_CURVE('',#19612,#19611,#9254,.T.);
#24117=EDGE_CURVE('',#19613,#19612,#9255,.T.);
#24118=EDGE_CURVE('',#19609,#19613,#9256,.T.);
#24119=EDGE_CURVE('',#19614,#19615,#9257,.T.);
#24120=EDGE_CURVE('',#19616,#19614,#9258,.T.);
#24121=EDGE_CURVE('',#19617,#19616,#9259,.T.);
#24122=EDGE_CURVE('',#19618,#19617,#9260,.T.);
#24123=EDGE_CURVE('',#19619,#19618,#9261,.T.);
#24124=EDGE_CURVE('',#19615,#19619,#9262,.T.);
#24125=EDGE_CURVE('',#19620,#19621,#9263,.T.);
#24126=EDGE_CURVE('',#19622,#19620,#9264,.T.);
#24127=EDGE_CURVE('',#19623,#19622,#9265,.T.);
#24128=EDGE_CURVE('',#19624,#19623,#9266,.T.);
#24129=EDGE_CURVE('',#19625,#19624,#9267,.T.);
#24130=EDGE_CURVE('',#19621,#19625,#9268,.T.);
#24131=EDGE_CURVE('',#19626,#19627,#9269,.T.);
#24132=EDGE_CURVE('',#19628,#19626,#9270,.T.);
#24133=EDGE_CURVE('',#19629,#19628,#9271,.T.);
#24134=EDGE_CURVE('',#19630,#19629,#9272,.T.);
#24135=EDGE_CURVE('',#19631,#19630,#9273,.T.);
#24136=EDGE_CURVE('',#19627,#19631,#9274,.T.);
#24137=EDGE_CURVE('',#19632,#19633,#9275,.T.);
#24138=EDGE_CURVE('',#19634,#19632,#9276,.T.);
#24139=EDGE_CURVE('',#19635,#19634,#9277,.T.);
#24140=EDGE_CURVE('',#19636,#19635,#9278,.T.);
#24141=EDGE_CURVE('',#19637,#19636,#9279,.T.);
#24142=EDGE_CURVE('',#19633,#19637,#9280,.T.);
#24143=EDGE_CURVE('',#19638,#19639,#9281,.T.);
#24144=EDGE_CURVE('',#19640,#19638,#9282,.T.);
#24145=EDGE_CURVE('',#19641,#19640,#9283,.T.);
#24146=EDGE_CURVE('',#19642,#19641,#9284,.T.);
#24147=EDGE_CURVE('',#19643,#19642,#9285,.T.);
#24148=EDGE_CURVE('',#19639,#19643,#9286,.T.);
#24149=EDGE_CURVE('',#19644,#19645,#9287,.T.);
#24150=EDGE_CURVE('',#19646,#19644,#9288,.T.);
#24151=EDGE_CURVE('',#19647,#19646,#9289,.T.);
#24152=EDGE_CURVE('',#19648,#19647,#9290,.T.);
#24153=EDGE_CURVE('',#19649,#19648,#9291,.T.);
#24154=EDGE_CURVE('',#19645,#19649,#9292,.T.);
#24155=EDGE_CURVE('',#19650,#19651,#9293,.T.);
#24156=EDGE_CURVE('',#19652,#19650,#9294,.T.);
#24157=EDGE_CURVE('',#19653,#19652,#9295,.T.);
#24158=EDGE_CURVE('',#19654,#19653,#9296,.T.);
#24159=EDGE_CURVE('',#19655,#19654,#9297,.T.);
#24160=EDGE_CURVE('',#19651,#19655,#9298,.T.);
#24161=EDGE_CURVE('',#19656,#19657,#9299,.T.);
#24162=EDGE_CURVE('',#19658,#19656,#9300,.T.);
#24163=EDGE_CURVE('',#19659,#19658,#9301,.T.);
#24164=EDGE_CURVE('',#19660,#19659,#9302,.T.);
#24165=EDGE_CURVE('',#19661,#19660,#9303,.T.);
#24166=EDGE_CURVE('',#19657,#19661,#9304,.T.);
#24167=EDGE_CURVE('',#19662,#19663,#9305,.T.);
#24168=EDGE_CURVE('',#19664,#19662,#9306,.T.);
#24169=EDGE_CURVE('',#19665,#19664,#9307,.T.);
#24170=EDGE_CURVE('',#19666,#19665,#9308,.T.);
#24171=EDGE_CURVE('',#19667,#19666,#9309,.T.);
#24172=EDGE_CURVE('',#19663,#19667,#9310,.T.);
#24173=EDGE_CURVE('',#19668,#19669,#9311,.T.);
#24174=EDGE_CURVE('',#19670,#19668,#9312,.T.);
#24175=EDGE_CURVE('',#19671,#19670,#9313,.T.);
#24176=EDGE_CURVE('',#19672,#19671,#9314,.T.);
#24177=EDGE_CURVE('',#19673,#19672,#9315,.T.);
#24178=EDGE_CURVE('',#19669,#19673,#9316,.T.);
#24179=EDGE_CURVE('',#19674,#19675,#9317,.T.);
#24180=EDGE_CURVE('',#19676,#19674,#9318,.T.);
#24181=EDGE_CURVE('',#19677,#19676,#9319,.T.);
#24182=EDGE_CURVE('',#19678,#19677,#9320,.T.);
#24183=EDGE_CURVE('',#19679,#19678,#9321,.T.);
#24184=EDGE_CURVE('',#19675,#19679,#9322,.T.);
#24185=EDGE_CURVE('',#19680,#19681,#9323,.T.);
#24186=EDGE_CURVE('',#19682,#19680,#9324,.T.);
#24187=EDGE_CURVE('',#19683,#19682,#9325,.T.);
#24188=EDGE_CURVE('',#19684,#19683,#9326,.T.);
#24189=EDGE_CURVE('',#19685,#19684,#9327,.T.);
#24190=EDGE_CURVE('',#19681,#19685,#9328,.T.);
#24191=EDGE_CURVE('',#19686,#19687,#9329,.T.);
#24192=EDGE_CURVE('',#19688,#19686,#9330,.T.);
#24193=EDGE_CURVE('',#19689,#19688,#9331,.T.);
#24194=EDGE_CURVE('',#19690,#19689,#9332,.T.);
#24195=EDGE_CURVE('',#19691,#19690,#9333,.T.);
#24196=EDGE_CURVE('',#19687,#19691,#9334,.T.);
#24197=EDGE_CURVE('',#19692,#19693,#9335,.T.);
#24198=EDGE_CURVE('',#19694,#19692,#9336,.T.);
#24199=EDGE_CURVE('',#19695,#19694,#9337,.T.);
#24200=EDGE_CURVE('',#19696,#19695,#9338,.T.);
#24201=EDGE_CURVE('',#19697,#19696,#9339,.T.);
#24202=EDGE_CURVE('',#19693,#19697,#9340,.T.);
#24203=EDGE_CURVE('',#19698,#19699,#9341,.T.);
#24204=EDGE_CURVE('',#19700,#19698,#9342,.T.);
#24205=EDGE_CURVE('',#19701,#19700,#9343,.T.);
#24206=EDGE_CURVE('',#19702,#19701,#9344,.T.);
#24207=EDGE_CURVE('',#19703,#19702,#9345,.T.);
#24208=EDGE_CURVE('',#19699,#19703,#9346,.T.);
#24209=EDGE_CURVE('',#19704,#19705,#9347,.T.);
#24210=EDGE_CURVE('',#19706,#19704,#9348,.T.);
#24211=EDGE_CURVE('',#19707,#19706,#9349,.T.);
#24212=EDGE_CURVE('',#19708,#19707,#9350,.T.);
#24213=EDGE_CURVE('',#19709,#19708,#9351,.T.);
#24214=EDGE_CURVE('',#19705,#19709,#9352,.T.);
#24215=EDGE_CURVE('',#19710,#19711,#9353,.T.);
#24216=EDGE_CURVE('',#19712,#19710,#9354,.T.);
#24217=EDGE_CURVE('',#19713,#19712,#9355,.T.);
#24218=EDGE_CURVE('',#19714,#19713,#9356,.T.);
#24219=EDGE_CURVE('',#19715,#19714,#9357,.T.);
#24220=EDGE_CURVE('',#19711,#19715,#9358,.T.);
#24221=EDGE_CURVE('',#19716,#19717,#9359,.T.);
#24222=EDGE_CURVE('',#19718,#19716,#9360,.T.);
#24223=EDGE_CURVE('',#19719,#19718,#9361,.T.);
#24224=EDGE_CURVE('',#19720,#19719,#9362,.T.);
#24225=EDGE_CURVE('',#19721,#19720,#9363,.T.);
#24226=EDGE_CURVE('',#19717,#19721,#9364,.T.);
#24227=EDGE_CURVE('',#19722,#19723,#9365,.T.);
#24228=EDGE_CURVE('',#19724,#19722,#9366,.T.);
#24229=EDGE_CURVE('',#19725,#19724,#9367,.T.);
#24230=EDGE_CURVE('',#19726,#19725,#9368,.T.);
#24231=EDGE_CURVE('',#19727,#19726,#9369,.T.);
#24232=EDGE_CURVE('',#19723,#19727,#9370,.T.);
#24233=EDGE_CURVE('',#19728,#19729,#9371,.T.);
#24234=EDGE_CURVE('',#19730,#19728,#9372,.T.);
#24235=EDGE_CURVE('',#19731,#19730,#9373,.T.);
#24236=EDGE_CURVE('',#19732,#19731,#9374,.T.);
#24237=EDGE_CURVE('',#19733,#19732,#9375,.T.);
#24238=EDGE_CURVE('',#19729,#19733,#9376,.T.);
#24239=EDGE_CURVE('',#19734,#19735,#9377,.T.);
#24240=EDGE_CURVE('',#19736,#19734,#9378,.T.);
#24241=EDGE_CURVE('',#19737,#19736,#9379,.T.);
#24242=EDGE_CURVE('',#19738,#19737,#9380,.T.);
#24243=EDGE_CURVE('',#19739,#19738,#9381,.T.);
#24244=EDGE_CURVE('',#19735,#19739,#9382,.T.);
#24245=EDGE_CURVE('',#19740,#19741,#9383,.T.);
#24246=EDGE_CURVE('',#19741,#19742,#9384,.T.);
#24247=EDGE_CURVE('',#19742,#19743,#9385,.T.);
#24248=EDGE_CURVE('',#19743,#19744,#9386,.T.);
#24249=EDGE_CURVE('',#19744,#19745,#9387,.T.);
#24250=EDGE_CURVE('',#19745,#19740,#9388,.T.);
#24251=EDGE_CURVE('',#19746,#19747,#9389,.T.);
#24252=EDGE_CURVE('',#19747,#19748,#9390,.T.);
#24253=EDGE_CURVE('',#19748,#19749,#9391,.T.);
#24254=EDGE_CURVE('',#19749,#19750,#9392,.T.);
#24255=EDGE_CURVE('',#19750,#19751,#9393,.T.);
#24256=EDGE_CURVE('',#19751,#19746,#9394,.T.);
#24257=EDGE_CURVE('',#19752,#19753,#9395,.T.);
#24258=EDGE_CURVE('',#19753,#19754,#9396,.T.);
#24259=EDGE_CURVE('',#19754,#19755,#9397,.T.);
#24260=EDGE_CURVE('',#19755,#19756,#9398,.T.);
#24261=EDGE_CURVE('',#19756,#19757,#9399,.T.);
#24262=EDGE_CURVE('',#19757,#19752,#9400,.T.);
#24263=EDGE_CURVE('',#19758,#19759,#9401,.T.);
#24264=EDGE_CURVE('',#19759,#19760,#9402,.T.);
#24265=EDGE_CURVE('',#19760,#19761,#9403,.T.);
#24266=EDGE_CURVE('',#19761,#19762,#9404,.T.);
#24267=EDGE_CURVE('',#19762,#19763,#9405,.T.);
#24268=EDGE_CURVE('',#19763,#19758,#9406,.T.);
#24269=EDGE_CURVE('',#19764,#19765,#9407,.T.);
#24270=EDGE_CURVE('',#19765,#19766,#9408,.T.);
#24271=EDGE_CURVE('',#19766,#19767,#9409,.T.);
#24272=EDGE_CURVE('',#19767,#19768,#9410,.T.);
#24273=EDGE_CURVE('',#19768,#19769,#9411,.T.);
#24274=EDGE_CURVE('',#19769,#19764,#9412,.T.);
#24275=EDGE_CURVE('',#19770,#19771,#9413,.T.);
#24276=EDGE_CURVE('',#19771,#19772,#9414,.T.);
#24277=EDGE_CURVE('',#19772,#19773,#9415,.T.);
#24278=EDGE_CURVE('',#19773,#19774,#9416,.T.);
#24279=EDGE_CURVE('',#19774,#19775,#9417,.T.);
#24280=EDGE_CURVE('',#19775,#19770,#9418,.T.);
#24281=EDGE_CURVE('',#19776,#19777,#9419,.T.);
#24282=EDGE_CURVE('',#19777,#19778,#9420,.T.);
#24283=EDGE_CURVE('',#19778,#19779,#9421,.T.);
#24284=EDGE_CURVE('',#19779,#19780,#9422,.T.);
#24285=EDGE_CURVE('',#19780,#19781,#9423,.T.);
#24286=EDGE_CURVE('',#19781,#19776,#9424,.T.);
#24287=EDGE_CURVE('',#19782,#19783,#9425,.T.);
#24288=EDGE_CURVE('',#19783,#19784,#9426,.T.);
#24289=EDGE_CURVE('',#19784,#19785,#9427,.T.);
#24290=EDGE_CURVE('',#19785,#19786,#9428,.T.);
#24291=EDGE_CURVE('',#19786,#19787,#9429,.T.);
#24292=EDGE_CURVE('',#19787,#19782,#9430,.T.);
#24293=EDGE_CURVE('',#19788,#19789,#9431,.T.);
#24294=EDGE_CURVE('',#19789,#19790,#9432,.T.);
#24295=EDGE_CURVE('',#19790,#19791,#9433,.T.);
#24296=EDGE_CURVE('',#19791,#19792,#9434,.T.);
#24297=EDGE_CURVE('',#19792,#19793,#9435,.T.);
#24298=EDGE_CURVE('',#19793,#19788,#9436,.T.);
#24299=EDGE_CURVE('',#19794,#19795,#9437,.T.);
#24300=EDGE_CURVE('',#19795,#19796,#9438,.T.);
#24301=EDGE_CURVE('',#19796,#19797,#9439,.T.);
#24302=EDGE_CURVE('',#19797,#19798,#9440,.T.);
#24303=EDGE_CURVE('',#19798,#19799,#9441,.T.);
#24304=EDGE_CURVE('',#19799,#19794,#9442,.T.);
#24305=EDGE_CURVE('',#19800,#19801,#9443,.T.);
#24306=EDGE_CURVE('',#19801,#19802,#9444,.T.);
#24307=EDGE_CURVE('',#19802,#19803,#9445,.T.);
#24308=EDGE_CURVE('',#19803,#19804,#9446,.T.);
#24309=EDGE_CURVE('',#19804,#19805,#9447,.T.);
#24310=EDGE_CURVE('',#19805,#19800,#9448,.T.);
#24311=EDGE_CURVE('',#19806,#19807,#9449,.T.);
#24312=EDGE_CURVE('',#19807,#19808,#9450,.T.);
#24313=EDGE_CURVE('',#19808,#19809,#9451,.T.);
#24314=EDGE_CURVE('',#19809,#19810,#9452,.T.);
#24315=EDGE_CURVE('',#19810,#19811,#9453,.T.);
#24316=EDGE_CURVE('',#19811,#19806,#9454,.T.);
#24317=EDGE_CURVE('',#19812,#19813,#9455,.T.);
#24318=EDGE_CURVE('',#19813,#19814,#9456,.T.);
#24319=EDGE_CURVE('',#19814,#19815,#9457,.T.);
#24320=EDGE_CURVE('',#19815,#19816,#9458,.T.);
#24321=EDGE_CURVE('',#19816,#19817,#9459,.T.);
#24322=EDGE_CURVE('',#19817,#19812,#9460,.T.);
#24323=EDGE_CURVE('',#19818,#19819,#9461,.T.);
#24324=EDGE_CURVE('',#19819,#19820,#9462,.T.);
#24325=EDGE_CURVE('',#19820,#19821,#9463,.T.);
#24326=EDGE_CURVE('',#19821,#19822,#9464,.T.);
#24327=EDGE_CURVE('',#19822,#19823,#9465,.T.);
#24328=EDGE_CURVE('',#19823,#19818,#9466,.T.);
#24329=EDGE_CURVE('',#19824,#19825,#9467,.T.);
#24330=EDGE_CURVE('',#19825,#19826,#9468,.T.);
#24331=EDGE_CURVE('',#19826,#19827,#9469,.T.);
#24332=EDGE_CURVE('',#19827,#19828,#9470,.T.);
#24333=EDGE_CURVE('',#19828,#19829,#9471,.T.);
#24334=EDGE_CURVE('',#19829,#19824,#9472,.T.);
#24335=EDGE_CURVE('',#19830,#19831,#9473,.T.);
#24336=EDGE_CURVE('',#19831,#19832,#9474,.T.);
#24337=EDGE_CURVE('',#19832,#19833,#9475,.T.);
#24338=EDGE_CURVE('',#19833,#19834,#9476,.T.);
#24339=EDGE_CURVE('',#19834,#19835,#9477,.T.);
#24340=EDGE_CURVE('',#19835,#19830,#9478,.T.);
#24341=EDGE_CURVE('',#19836,#19837,#9479,.T.);
#24342=EDGE_CURVE('',#19837,#19838,#9480,.T.);
#24343=EDGE_CURVE('',#19838,#19839,#9481,.T.);
#24344=EDGE_CURVE('',#19839,#19840,#9482,.T.);
#24345=EDGE_CURVE('',#19840,#19841,#9483,.T.);
#24346=EDGE_CURVE('',#19841,#19836,#9484,.T.);
#24347=EDGE_CURVE('',#19842,#19843,#9485,.T.);
#24348=EDGE_CURVE('',#19843,#19844,#9486,.T.);
#24349=EDGE_CURVE('',#19844,#19845,#9487,.T.);
#24350=EDGE_CURVE('',#19845,#19846,#9488,.T.);
#24351=EDGE_CURVE('',#19846,#19847,#9489,.T.);
#24352=EDGE_CURVE('',#19847,#19842,#9490,.T.);
#24353=EDGE_CURVE('',#19848,#19849,#9491,.T.);
#24354=EDGE_CURVE('',#19849,#19850,#9492,.T.);
#24355=EDGE_CURVE('',#19850,#19851,#9493,.T.);
#24356=EDGE_CURVE('',#19851,#19852,#9494,.T.);
#24357=EDGE_CURVE('',#19852,#19853,#9495,.T.);
#24358=EDGE_CURVE('',#19853,#19848,#9496,.T.);
#24359=EDGE_CURVE('',#19854,#19855,#9497,.T.);
#24360=EDGE_CURVE('',#19855,#19856,#9498,.T.);
#24361=EDGE_CURVE('',#19856,#19857,#9499,.T.);
#24362=EDGE_CURVE('',#19857,#19858,#9500,.T.);
#24363=EDGE_CURVE('',#19858,#19859,#9501,.T.);
#24364=EDGE_CURVE('',#19859,#19854,#9502,.T.);
#24365=EDGE_CURVE('',#19860,#19861,#9503,.T.);
#24366=EDGE_CURVE('',#19861,#19862,#9504,.T.);
#24367=EDGE_CURVE('',#19862,#19863,#9505,.T.);
#24368=EDGE_CURVE('',#19863,#19864,#9506,.T.);
#24369=EDGE_CURVE('',#19864,#19865,#9507,.T.);
#24370=EDGE_CURVE('',#19865,#19860,#9508,.T.);
#24371=EDGE_CURVE('',#19866,#19867,#9509,.T.);
#24372=EDGE_CURVE('',#19867,#19868,#9510,.T.);
#24373=EDGE_CURVE('',#19868,#19869,#9511,.T.);
#24374=EDGE_CURVE('',#19869,#19870,#9512,.T.);
#24375=EDGE_CURVE('',#19870,#19871,#9513,.T.);
#24376=EDGE_CURVE('',#19871,#19866,#9514,.T.);
#24377=EDGE_CURVE('',#19872,#19873,#9515,.T.);
#24378=EDGE_CURVE('',#19873,#19874,#9516,.T.);
#24379=EDGE_CURVE('',#19874,#19875,#9517,.T.);
#24380=EDGE_CURVE('',#19875,#19876,#9518,.T.);
#24381=EDGE_CURVE('',#19876,#19877,#9519,.T.);
#24382=EDGE_CURVE('',#19877,#19872,#9520,.T.);
#24383=EDGE_CURVE('',#19878,#19879,#9521,.T.);
#24384=EDGE_CURVE('',#19879,#19880,#9522,.T.);
#24385=EDGE_CURVE('',#19880,#19881,#9523,.T.);
#24386=EDGE_CURVE('',#19881,#19882,#9524,.T.);
#24387=EDGE_CURVE('',#19882,#19883,#9525,.T.);
#24388=EDGE_CURVE('',#19883,#19878,#9526,.T.);
#24389=EDGE_CURVE('',#19884,#19885,#9527,.T.);
#24390=EDGE_CURVE('',#19885,#19886,#9528,.T.);
#24391=EDGE_CURVE('',#19886,#19887,#9529,.T.);
#24392=EDGE_CURVE('',#19887,#19888,#9530,.T.);
#24393=EDGE_CURVE('',#19888,#19889,#9531,.T.);
#24394=EDGE_CURVE('',#19889,#19884,#9532,.T.);
#24395=EDGE_CURVE('',#19890,#19891,#9533,.T.);
#24396=EDGE_CURVE('',#19891,#19892,#9534,.T.);
#24397=EDGE_CURVE('',#19892,#19893,#9535,.T.);
#24398=EDGE_CURVE('',#19893,#19894,#9536,.T.);
#24399=EDGE_CURVE('',#19894,#19895,#9537,.T.);
#24400=EDGE_CURVE('',#19895,#19890,#9538,.T.);
#24401=EDGE_CURVE('',#19896,#19897,#9539,.T.);
#24402=EDGE_CURVE('',#19897,#19898,#9540,.T.);
#24403=EDGE_CURVE('',#19898,#19899,#9541,.T.);
#24404=EDGE_CURVE('',#19899,#19900,#9542,.T.);
#24405=EDGE_CURVE('',#19900,#19901,#9543,.T.);
#24406=EDGE_CURVE('',#19901,#19896,#9544,.T.);
#24407=EDGE_CURVE('',#19902,#19903,#9545,.T.);
#24408=EDGE_CURVE('',#19903,#19904,#9546,.T.);
#24409=EDGE_CURVE('',#19904,#19905,#9547,.T.);
#24410=EDGE_CURVE('',#19905,#19906,#9548,.T.);
#24411=EDGE_CURVE('',#19906,#19907,#9549,.T.);
#24412=EDGE_CURVE('',#19907,#19902,#9550,.T.);
#24413=EDGE_CURVE('',#19908,#19909,#9551,.T.);
#24414=EDGE_CURVE('',#19909,#19910,#9552,.T.);
#24415=EDGE_CURVE('',#19910,#19911,#9553,.T.);
#24416=EDGE_CURVE('',#19911,#19912,#9554,.T.);
#24417=EDGE_CURVE('',#19912,#19913,#9555,.T.);
#24418=EDGE_CURVE('',#19913,#19908,#9556,.T.);
#24419=EDGE_CURVE('',#19914,#19915,#9557,.T.);
#24420=EDGE_CURVE('',#19915,#19916,#9558,.T.);
#24421=EDGE_CURVE('',#19916,#19917,#9559,.T.);
#24422=EDGE_CURVE('',#19917,#19918,#9560,.T.);
#24423=EDGE_CURVE('',#19918,#19919,#9561,.T.);
#24424=EDGE_CURVE('',#19919,#19914,#9562,.T.);
#24425=EDGE_CURVE('',#19920,#19921,#9563,.T.);
#24426=EDGE_CURVE('',#19921,#19922,#9564,.T.);
#24427=EDGE_CURVE('',#19922,#19923,#9565,.T.);
#24428=EDGE_CURVE('',#19923,#19924,#9566,.T.);
#24429=EDGE_CURVE('',#19924,#19925,#9567,.T.);
#24430=EDGE_CURVE('',#19925,#19920,#9568,.T.);
#24431=EDGE_CURVE('',#19926,#19927,#9569,.T.);
#24432=EDGE_CURVE('',#19927,#19928,#9570,.T.);
#24433=EDGE_CURVE('',#19928,#19929,#9571,.T.);
#24434=EDGE_CURVE('',#19929,#19930,#9572,.T.);
#24435=EDGE_CURVE('',#19930,#19931,#9573,.T.);
#24436=EDGE_CURVE('',#19931,#19926,#9574,.T.);
#24437=EDGE_CURVE('',#19932,#19933,#9575,.T.);
#24438=EDGE_CURVE('',#19933,#19934,#9576,.T.);
#24439=EDGE_CURVE('',#19934,#19935,#9577,.T.);
#24440=EDGE_CURVE('',#19935,#19936,#9578,.T.);
#24441=EDGE_CURVE('',#19936,#19937,#9579,.T.);
#24442=EDGE_CURVE('',#19937,#19932,#9580,.T.);
#24443=EDGE_CURVE('',#19938,#19939,#9581,.T.);
#24444=EDGE_CURVE('',#19939,#19940,#9582,.T.);
#24445=EDGE_CURVE('',#19940,#19941,#9583,.T.);
#24446=EDGE_CURVE('',#19941,#19942,#9584,.T.);
#24447=EDGE_CURVE('',#19942,#19943,#9585,.T.);
#24448=EDGE_CURVE('',#19943,#19938,#9586,.T.);
#24449=EDGE_CURVE('',#19944,#19945,#9587,.T.);
#24450=EDGE_CURVE('',#19945,#19946,#9588,.T.);
#24451=EDGE_CURVE('',#19946,#19947,#9589,.T.);
#24452=EDGE_CURVE('',#19947,#19948,#9590,.T.);
#24453=EDGE_CURVE('',#19948,#19949,#9591,.T.);
#24454=EDGE_CURVE('',#19949,#19944,#9592,.T.);
#24455=EDGE_CURVE('',#19950,#19951,#9593,.T.);
#24456=EDGE_CURVE('',#19951,#19952,#9594,.T.);
#24457=EDGE_CURVE('',#19952,#19953,#9595,.T.);
#24458=EDGE_CURVE('',#19953,#19954,#9596,.T.);
#24459=EDGE_CURVE('',#19954,#19955,#9597,.T.);
#24460=EDGE_CURVE('',#19955,#19950,#9598,.T.);
#24461=EDGE_CURVE('',#19956,#19957,#9599,.T.);
#24462=EDGE_CURVE('',#19957,#19958,#9600,.T.);
#24463=EDGE_CURVE('',#19958,#19959,#9601,.T.);
#24464=EDGE_CURVE('',#19959,#19960,#9602,.T.);
#24465=EDGE_CURVE('',#19960,#19961,#9603,.T.);
#24466=EDGE_CURVE('',#19961,#19956,#9604,.T.);
#24467=EDGE_CURVE('',#19962,#19963,#9605,.T.);
#24468=EDGE_CURVE('',#19963,#19964,#9606,.T.);
#24469=EDGE_CURVE('',#19964,#19965,#9607,.T.);
#24470=EDGE_CURVE('',#19965,#19966,#9608,.T.);
#24471=EDGE_CURVE('',#19966,#19967,#9609,.T.);
#24472=EDGE_CURVE('',#19967,#19962,#9610,.T.);
#24473=EDGE_CURVE('',#19968,#19969,#9611,.T.);
#24474=EDGE_CURVE('',#19969,#19970,#9612,.T.);
#24475=EDGE_CURVE('',#19970,#19971,#9613,.T.);
#24476=EDGE_CURVE('',#19971,#19972,#9614,.T.);
#24477=EDGE_CURVE('',#19972,#19973,#9615,.T.);
#24478=EDGE_CURVE('',#19973,#19968,#9616,.T.);
#24479=EDGE_CURVE('',#19974,#19975,#9617,.T.);
#24480=EDGE_CURVE('',#19975,#19976,#9618,.T.);
#24481=EDGE_CURVE('',#19976,#19977,#9619,.T.);
#24482=EDGE_CURVE('',#19977,#19978,#9620,.T.);
#24483=EDGE_CURVE('',#19978,#19979,#9621,.T.);
#24484=EDGE_CURVE('',#19979,#19974,#9622,.T.);
#24485=EDGE_CURVE('',#19980,#19981,#9623,.T.);
#24486=EDGE_CURVE('',#19981,#19982,#9624,.T.);
#24487=EDGE_CURVE('',#19982,#19983,#9625,.T.);
#24488=EDGE_CURVE('',#19983,#19984,#9626,.T.);
#24489=EDGE_CURVE('',#19984,#19985,#9627,.T.);
#24490=EDGE_CURVE('',#19985,#19980,#9628,.T.);
#24491=EDGE_CURVE('',#19986,#19987,#9629,.T.);
#24492=EDGE_CURVE('',#19987,#19988,#9630,.T.);
#24493=EDGE_CURVE('',#19988,#19989,#9631,.T.);
#24494=EDGE_CURVE('',#19989,#19990,#9632,.T.);
#24495=EDGE_CURVE('',#19990,#19991,#9633,.T.);
#24496=EDGE_CURVE('',#19991,#19986,#9634,.T.);
#24497=EDGE_CURVE('',#19992,#19993,#9635,.T.);
#24498=EDGE_CURVE('',#19993,#19994,#9636,.T.);
#24499=EDGE_CURVE('',#19994,#19995,#9637,.T.);
#24500=EDGE_CURVE('',#19995,#19996,#9638,.T.);
#24501=EDGE_CURVE('',#19996,#19997,#9639,.T.);
#24502=EDGE_CURVE('',#19997,#19992,#9640,.T.);
#24503=EDGE_CURVE('',#19998,#19999,#9641,.T.);
#24504=EDGE_CURVE('',#19999,#20000,#9642,.T.);
#24505=EDGE_CURVE('',#20000,#20001,#9643,.T.);
#24506=EDGE_CURVE('',#20001,#20002,#9644,.T.);
#24507=EDGE_CURVE('',#20002,#20003,#9645,.T.);
#24508=EDGE_CURVE('',#20003,#19998,#9646,.T.);
#24509=EDGE_CURVE('',#20004,#20005,#9647,.T.);
#24510=EDGE_CURVE('',#20005,#20006,#9648,.T.);
#24511=EDGE_CURVE('',#20006,#20007,#9649,.T.);
#24512=EDGE_CURVE('',#20007,#20008,#9650,.T.);
#24513=EDGE_CURVE('',#20008,#20009,#9651,.T.);
#24514=EDGE_CURVE('',#20009,#20004,#9652,.T.);
#24515=EDGE_CURVE('',#20010,#20011,#9653,.T.);
#24516=EDGE_CURVE('',#20011,#20012,#9654,.T.);
#24517=EDGE_CURVE('',#20012,#20013,#9655,.T.);
#24518=EDGE_CURVE('',#20013,#20014,#9656,.T.);
#24519=EDGE_CURVE('',#20014,#20015,#9657,.T.);
#24520=EDGE_CURVE('',#20015,#20010,#9658,.T.);
#24521=EDGE_CURVE('',#20016,#20017,#9659,.T.);
#24522=EDGE_CURVE('',#20017,#20018,#9660,.T.);
#24523=EDGE_CURVE('',#20018,#20019,#9661,.T.);
#24524=EDGE_CURVE('',#20019,#20020,#9662,.T.);
#24525=EDGE_CURVE('',#20020,#20021,#9663,.T.);
#24526=EDGE_CURVE('',#20021,#20016,#9664,.T.);
#24527=EDGE_CURVE('',#20022,#20023,#9665,.T.);
#24528=EDGE_CURVE('',#20023,#20024,#9666,.T.);
#24529=EDGE_CURVE('',#20024,#20025,#9667,.T.);
#24530=EDGE_CURVE('',#20025,#20026,#9668,.T.);
#24531=EDGE_CURVE('',#20026,#20027,#9669,.T.);
#24532=EDGE_CURVE('',#20027,#20022,#9670,.T.);
#24533=EDGE_CURVE('',#20028,#20029,#9671,.T.);
#24534=EDGE_CURVE('',#20029,#20030,#9672,.T.);
#24535=EDGE_CURVE('',#20030,#20031,#9673,.T.);
#24536=EDGE_CURVE('',#20031,#20032,#9674,.T.);
#24537=EDGE_CURVE('',#20032,#20033,#9675,.T.);
#24538=EDGE_CURVE('',#20033,#20028,#9676,.T.);
#24539=EDGE_CURVE('',#20034,#20035,#9677,.T.);
#24540=EDGE_CURVE('',#20035,#20036,#9678,.T.);
#24541=EDGE_CURVE('',#20036,#20037,#9679,.T.);
#24542=EDGE_CURVE('',#20037,#20038,#9680,.T.);
#24543=EDGE_CURVE('',#20038,#20039,#9681,.T.);
#24544=EDGE_CURVE('',#20039,#20034,#9682,.T.);
#24545=EDGE_CURVE('',#20040,#20041,#9683,.T.);
#24546=EDGE_CURVE('',#20041,#20042,#9684,.T.);
#24547=EDGE_CURVE('',#20042,#20043,#9685,.T.);
#24548=EDGE_CURVE('',#20043,#20044,#9686,.T.);
#24549=EDGE_CURVE('',#20044,#20045,#9687,.T.);
#24550=EDGE_CURVE('',#20045,#20040,#9688,.T.);
#24551=EDGE_CURVE('',#20046,#20047,#9689,.T.);
#24552=EDGE_CURVE('',#20047,#20048,#9690,.T.);
#24553=EDGE_CURVE('',#20048,#20049,#9691,.T.);
#24554=EDGE_CURVE('',#20049,#20050,#9692,.T.);
#24555=EDGE_CURVE('',#20050,#20051,#9693,.T.);
#24556=EDGE_CURVE('',#20051,#20046,#9694,.T.);
#24557=EDGE_CURVE('',#20052,#20053,#9695,.T.);
#24558=EDGE_CURVE('',#20053,#20054,#9696,.T.);
#24559=EDGE_CURVE('',#20054,#20055,#9697,.T.);
#24560=EDGE_CURVE('',#20055,#20056,#9698,.T.);
#24561=EDGE_CURVE('',#20056,#20057,#9699,.T.);
#24562=EDGE_CURVE('',#20057,#20052,#9700,.T.);
#24563=EDGE_CURVE('',#20058,#20059,#9701,.T.);
#24564=EDGE_CURVE('',#20059,#20060,#9702,.T.);
#24565=EDGE_CURVE('',#20060,#20061,#9703,.T.);
#24566=EDGE_CURVE('',#20061,#20062,#9704,.T.);
#24567=EDGE_CURVE('',#20062,#20063,#9705,.T.);
#24568=EDGE_CURVE('',#20063,#20058,#9706,.T.);
#24569=EDGE_CURVE('',#20064,#20065,#9707,.T.);
#24570=EDGE_CURVE('',#20065,#20066,#9708,.T.);
#24571=EDGE_CURVE('',#20066,#20067,#9709,.T.);
#24572=EDGE_CURVE('',#20067,#20068,#9710,.T.);
#24573=EDGE_CURVE('',#20068,#20069,#9711,.T.);
#24574=EDGE_CURVE('',#20069,#20064,#9712,.T.);
#24575=EDGE_CURVE('',#20070,#20071,#9713,.T.);
#24576=EDGE_CURVE('',#20071,#20072,#9714,.T.);
#24577=EDGE_CURVE('',#20072,#20073,#9715,.T.);
#24578=EDGE_CURVE('',#20073,#20074,#9716,.T.);
#24579=EDGE_CURVE('',#20074,#20075,#9717,.T.);
#24580=EDGE_CURVE('',#20075,#20070,#9718,.T.);
#24581=EDGE_CURVE('',#20076,#20077,#9719,.T.);
#24582=EDGE_CURVE('',#20077,#20078,#9720,.T.);
#24583=EDGE_CURVE('',#20078,#20079,#9721,.T.);
#24584=EDGE_CURVE('',#20079,#20080,#9722,.T.);
#24585=EDGE_CURVE('',#20080,#20081,#9723,.T.);
#24586=EDGE_CURVE('',#20081,#20076,#9724,.T.);
#24587=EDGE_CURVE('',#20082,#20083,#9725,.T.);
#24588=EDGE_CURVE('',#20083,#20084,#9726,.T.);
#24589=EDGE_CURVE('',#20084,#20085,#9727,.T.);
#24590=EDGE_CURVE('',#20085,#20086,#9728,.T.);
#24591=EDGE_CURVE('',#20086,#20087,#9729,.T.);
#24592=EDGE_CURVE('',#20087,#20082,#9730,.T.);
#24593=EDGE_CURVE('',#20088,#20089,#9731,.T.);
#24594=EDGE_CURVE('',#20089,#20090,#9732,.T.);
#24595=EDGE_CURVE('',#20090,#20091,#9733,.T.);
#24596=EDGE_CURVE('',#20091,#20092,#9734,.T.);
#24597=EDGE_CURVE('',#20092,#20093,#9735,.T.);
#24598=EDGE_CURVE('',#20093,#20088,#9736,.T.);
#24599=EDGE_CURVE('',#20094,#20095,#9737,.T.);
#24600=EDGE_CURVE('',#20095,#20096,#9738,.T.);
#24601=EDGE_CURVE('',#20096,#20097,#9739,.T.);
#24602=EDGE_CURVE('',#20097,#20098,#9740,.T.);
#24603=EDGE_CURVE('',#20098,#20099,#9741,.T.);
#24604=EDGE_CURVE('',#20099,#20094,#9742,.T.);
#24605=EDGE_CURVE('',#20100,#20101,#9743,.T.);
#24606=EDGE_CURVE('',#20101,#20102,#9744,.T.);
#24607=EDGE_CURVE('',#20102,#20103,#9745,.T.);
#24608=EDGE_CURVE('',#20103,#20104,#9746,.T.);
#24609=EDGE_CURVE('',#20104,#20105,#9747,.T.);
#24610=EDGE_CURVE('',#20105,#20100,#9748,.T.);
#24611=EDGE_CURVE('',#20106,#20107,#9749,.T.);
#24612=EDGE_CURVE('',#20107,#20108,#9750,.T.);
#24613=EDGE_CURVE('',#20108,#20109,#9751,.T.);
#24614=EDGE_CURVE('',#20109,#20110,#9752,.T.);
#24615=EDGE_CURVE('',#20110,#20111,#9753,.T.);
#24616=EDGE_CURVE('',#20111,#20106,#9754,.T.);
#24617=EDGE_CURVE('',#20112,#20113,#9755,.T.);
#24618=EDGE_CURVE('',#20113,#20114,#9756,.T.);
#24619=EDGE_CURVE('',#20114,#20115,#9757,.T.);
#24620=EDGE_CURVE('',#20115,#20116,#9758,.T.);
#24621=EDGE_CURVE('',#20116,#20117,#9759,.T.);
#24622=EDGE_CURVE('',#20117,#20112,#9760,.T.);
#24623=EDGE_CURVE('',#20118,#20119,#9761,.T.);
#24624=EDGE_CURVE('',#20119,#20120,#9762,.T.);
#24625=EDGE_CURVE('',#20120,#20121,#9763,.T.);
#24626=EDGE_CURVE('',#20121,#20122,#9764,.T.);
#24627=EDGE_CURVE('',#20122,#20123,#9765,.T.);
#24628=EDGE_CURVE('',#20123,#20118,#9766,.T.);
#24629=EDGE_CURVE('',#20124,#20125,#9767,.T.);
#24630=EDGE_CURVE('',#20125,#20126,#9768,.T.);
#24631=EDGE_CURVE('',#20126,#20127,#9769,.T.);
#24632=EDGE_CURVE('',#20127,#20128,#9770,.T.);
#24633=EDGE_CURVE('',#20128,#20129,#9771,.T.);
#24634=EDGE_CURVE('',#20129,#20124,#9772,.T.);
#24635=EDGE_CURVE('',#20130,#20131,#9773,.T.);
#24636=EDGE_CURVE('',#20131,#20132,#9774,.T.);
#24637=EDGE_CURVE('',#20132,#20133,#9775,.T.);
#24638=EDGE_CURVE('',#20133,#20134,#9776,.T.);
#24639=EDGE_CURVE('',#20134,#20135,#9777,.T.);
#24640=EDGE_CURVE('',#20135,#20130,#9778,.T.);
#24641=EDGE_CURVE('',#20136,#20137,#9779,.T.);
#24642=EDGE_CURVE('',#20137,#20138,#9780,.T.);
#24643=EDGE_CURVE('',#20138,#20139,#9781,.T.);
#24644=EDGE_CURVE('',#20139,#20140,#9782,.T.);
#24645=EDGE_CURVE('',#20140,#20141,#9783,.T.);
#24646=EDGE_CURVE('',#20141,#20136,#9784,.T.);
#24647=EDGE_CURVE('',#20142,#20143,#9785,.T.);
#24648=EDGE_CURVE('',#20143,#20144,#9786,.T.);
#24649=EDGE_CURVE('',#20144,#20145,#9787,.T.);
#24650=EDGE_CURVE('',#20145,#20146,#9788,.T.);
#24651=EDGE_CURVE('',#20146,#20147,#9789,.T.);
#24652=EDGE_CURVE('',#20147,#20142,#9790,.T.);
#24653=EDGE_CURVE('',#20148,#20149,#9791,.T.);
#24654=EDGE_CURVE('',#20149,#20150,#9792,.T.);
#24655=EDGE_CURVE('',#20150,#20151,#9793,.T.);
#24656=EDGE_CURVE('',#20151,#20152,#9794,.T.);
#24657=EDGE_CURVE('',#20152,#20153,#9795,.T.);
#24658=EDGE_CURVE('',#20153,#20148,#9796,.T.);
#24659=EDGE_CURVE('',#20154,#20155,#9797,.T.);
#24660=EDGE_CURVE('',#20155,#20156,#9798,.T.);
#24661=EDGE_CURVE('',#20156,#20157,#9799,.T.);
#24662=EDGE_CURVE('',#20157,#20158,#9800,.T.);
#24663=EDGE_CURVE('',#20158,#20159,#9801,.T.);
#24664=EDGE_CURVE('',#20159,#20154,#9802,.T.);
#24665=EDGE_CURVE('',#20160,#20161,#9803,.T.);
#24666=EDGE_CURVE('',#20161,#20162,#9804,.T.);
#24667=EDGE_CURVE('',#20162,#20163,#9805,.T.);
#24668=EDGE_CURVE('',#20163,#20164,#9806,.T.);
#24669=EDGE_CURVE('',#20164,#20165,#9807,.T.);
#24670=EDGE_CURVE('',#20165,#20160,#9808,.T.);
#24671=EDGE_CURVE('',#20166,#20167,#9809,.T.);
#24672=EDGE_CURVE('',#20167,#20168,#9810,.T.);
#24673=EDGE_CURVE('',#20168,#20169,#9811,.T.);
#24674=EDGE_CURVE('',#20169,#20170,#9812,.T.);
#24675=EDGE_CURVE('',#20170,#20171,#9813,.T.);
#24676=EDGE_CURVE('',#20171,#20166,#9814,.T.);
#24677=EDGE_CURVE('',#20172,#20173,#9815,.T.);
#24678=EDGE_CURVE('',#20173,#20174,#9816,.T.);
#24679=EDGE_CURVE('',#20174,#20175,#9817,.T.);
#24680=EDGE_CURVE('',#20175,#20176,#9818,.T.);
#24681=EDGE_CURVE('',#20176,#20177,#9819,.T.);
#24682=EDGE_CURVE('',#20177,#20172,#9820,.T.);
#24683=EDGE_CURVE('',#20178,#20179,#9821,.T.);
#24684=EDGE_CURVE('',#20179,#20180,#9822,.T.);
#24685=EDGE_CURVE('',#20180,#20181,#9823,.T.);
#24686=EDGE_CURVE('',#20181,#20182,#9824,.T.);
#24687=EDGE_CURVE('',#20182,#20183,#9825,.T.);
#24688=EDGE_CURVE('',#20183,#20178,#9826,.T.);
#24689=EDGE_CURVE('',#20184,#20185,#9827,.T.);
#24690=EDGE_CURVE('',#20185,#20186,#9828,.T.);
#24691=EDGE_CURVE('',#20186,#20187,#9829,.T.);
#24692=EDGE_CURVE('',#20187,#20188,#9830,.T.);
#24693=EDGE_CURVE('',#20188,#20189,#9831,.T.);
#24694=EDGE_CURVE('',#20189,#20184,#9832,.T.);
#24695=EDGE_CURVE('',#20190,#20191,#9833,.T.);
#24696=EDGE_CURVE('',#20191,#20192,#9834,.T.);
#24697=EDGE_CURVE('',#20192,#20193,#9835,.T.);
#24698=EDGE_CURVE('',#20193,#20194,#9836,.T.);
#24699=EDGE_CURVE('',#20194,#20195,#9837,.T.);
#24700=EDGE_CURVE('',#20195,#20190,#9838,.T.);
#24701=EDGE_CURVE('',#20196,#20197,#9839,.T.);
#24702=EDGE_CURVE('',#20197,#20198,#9840,.T.);
#24703=EDGE_CURVE('',#20198,#20199,#9841,.T.);
#24704=EDGE_CURVE('',#20199,#20200,#9842,.T.);
#24705=EDGE_CURVE('',#20200,#20201,#9843,.T.);
#24706=EDGE_CURVE('',#20201,#20196,#9844,.T.);
#24707=EDGE_CURVE('',#20202,#20203,#9845,.T.);
#24708=EDGE_CURVE('',#20203,#20204,#9846,.T.);
#24709=EDGE_CURVE('',#20204,#20205,#9847,.T.);
#24710=EDGE_CURVE('',#20205,#20206,#9848,.T.);
#24711=EDGE_CURVE('',#20206,#20207,#9849,.T.);
#24712=EDGE_CURVE('',#20207,#20202,#9850,.T.);
#24713=EDGE_CURVE('',#20208,#20209,#9851,.T.);
#24714=EDGE_CURVE('',#20209,#20210,#9852,.T.);
#24715=EDGE_CURVE('',#20210,#20211,#9853,.T.);
#24716=EDGE_CURVE('',#20211,#20212,#9854,.T.);
#24717=EDGE_CURVE('',#20212,#20213,#9855,.T.);
#24718=EDGE_CURVE('',#20213,#20208,#9856,.T.);
#24719=EDGE_CURVE('',#20214,#20215,#9857,.T.);
#24720=EDGE_CURVE('',#20215,#20216,#9858,.T.);
#24721=EDGE_CURVE('',#20216,#20217,#9859,.T.);
#24722=EDGE_CURVE('',#20217,#20218,#9860,.T.);
#24723=EDGE_CURVE('',#20218,#20219,#9861,.T.);
#24724=EDGE_CURVE('',#20219,#20214,#9862,.T.);
#24725=EDGE_CURVE('',#20220,#20221,#9863,.T.);
#24726=EDGE_CURVE('',#20221,#20222,#9864,.T.);
#24727=EDGE_CURVE('',#20222,#20223,#9865,.T.);
#24728=EDGE_CURVE('',#20223,#20224,#9866,.T.);
#24729=EDGE_CURVE('',#20224,#20225,#9867,.T.);
#24730=EDGE_CURVE('',#20225,#20220,#9868,.T.);
#24731=EDGE_CURVE('',#20226,#20227,#9869,.T.);
#24732=EDGE_CURVE('',#20227,#20228,#9870,.T.);
#24733=EDGE_CURVE('',#20228,#20229,#9871,.T.);
#24734=EDGE_CURVE('',#20229,#20230,#9872,.T.);
#24735=EDGE_CURVE('',#20230,#20231,#9873,.T.);
#24736=EDGE_CURVE('',#20231,#20226,#9874,.T.);
#24737=EDGE_CURVE('',#20232,#20233,#9875,.T.);
#24738=EDGE_CURVE('',#20233,#20234,#9876,.T.);
#24739=EDGE_CURVE('',#20234,#20235,#9877,.T.);
#24740=EDGE_CURVE('',#20235,#20236,#9878,.T.);
#24741=EDGE_CURVE('',#20236,#20237,#9879,.T.);
#24742=EDGE_CURVE('',#20237,#20232,#9880,.T.);
#24743=EDGE_CURVE('',#20238,#20239,#9881,.T.);
#24744=EDGE_CURVE('',#20239,#20240,#9882,.T.);
#24745=EDGE_CURVE('',#20240,#20241,#9883,.T.);
#24746=EDGE_CURVE('',#20241,#20242,#9884,.T.);
#24747=EDGE_CURVE('',#20242,#20243,#9885,.T.);
#24748=EDGE_CURVE('',#20243,#20238,#9886,.T.);
#24749=EDGE_CURVE('',#20244,#20245,#9887,.T.);
#24750=EDGE_CURVE('',#20245,#20246,#9888,.T.);
#24751=EDGE_CURVE('',#20246,#20247,#9889,.T.);
#24752=EDGE_CURVE('',#20247,#20248,#9890,.T.);
#24753=EDGE_CURVE('',#20248,#20249,#9891,.T.);
#24754=EDGE_CURVE('',#20249,#20244,#9892,.T.);
#24755=EDGE_CURVE('',#20250,#20251,#9893,.T.);
#24756=EDGE_CURVE('',#20251,#20252,#9894,.T.);
#24757=EDGE_CURVE('',#20252,#20253,#9895,.T.);
#24758=EDGE_CURVE('',#20253,#20254,#9896,.T.);
#24759=EDGE_CURVE('',#20254,#20255,#9897,.T.);
#24760=EDGE_CURVE('',#20255,#20250,#9898,.T.);
#24761=EDGE_CURVE('',#20256,#20257,#9899,.T.);
#24762=EDGE_CURVE('',#20257,#20258,#9900,.T.);
#24763=EDGE_CURVE('',#20258,#20259,#9901,.T.);
#24764=EDGE_CURVE('',#20259,#20260,#9902,.T.);
#24765=EDGE_CURVE('',#20260,#20261,#9903,.T.);
#24766=EDGE_CURVE('',#20261,#20256,#9904,.T.);
#24767=EDGE_CURVE('',#20262,#20263,#9905,.T.);
#24768=EDGE_CURVE('',#20263,#20264,#9906,.T.);
#24769=EDGE_CURVE('',#20264,#20265,#9907,.T.);
#24770=EDGE_CURVE('',#20265,#20266,#9908,.T.);
#24771=EDGE_CURVE('',#20266,#20267,#9909,.T.);
#24772=EDGE_CURVE('',#20267,#20262,#9910,.T.);
#24773=EDGE_CURVE('',#20268,#20269,#9911,.T.);
#24774=EDGE_CURVE('',#20269,#20270,#9912,.T.);
#24775=EDGE_CURVE('',#20270,#20271,#9913,.T.);
#24776=EDGE_CURVE('',#20271,#20272,#9914,.T.);
#24777=EDGE_CURVE('',#20272,#20273,#9915,.T.);
#24778=EDGE_CURVE('',#20273,#20268,#9916,.T.);
#24779=EDGE_CURVE('',#20274,#20275,#9917,.T.);
#24780=EDGE_CURVE('',#20275,#20276,#9918,.T.);
#24781=EDGE_CURVE('',#20276,#20277,#9919,.T.);
#24782=EDGE_CURVE('',#20277,#20278,#9920,.T.);
#24783=EDGE_CURVE('',#20278,#20279,#9921,.T.);
#24784=EDGE_CURVE('',#20279,#20274,#9922,.T.);
#24785=EDGE_CURVE('',#20280,#20281,#9923,.T.);
#24786=EDGE_CURVE('',#20281,#20282,#9924,.T.);
#24787=EDGE_CURVE('',#20282,#20283,#9925,.T.);
#24788=EDGE_CURVE('',#20283,#20284,#9926,.T.);
#24789=EDGE_CURVE('',#20284,#20285,#9927,.T.);
#24790=EDGE_CURVE('',#20285,#20280,#9928,.T.);
#24791=EDGE_CURVE('',#20286,#20287,#9929,.T.);
#24792=EDGE_CURVE('',#20287,#20288,#9930,.T.);
#24793=EDGE_CURVE('',#20288,#20289,#9931,.T.);
#24794=EDGE_CURVE('',#20289,#20290,#9932,.T.);
#24795=EDGE_CURVE('',#20290,#20291,#9933,.T.);
#24796=EDGE_CURVE('',#20291,#20286,#9934,.T.);
#24797=EDGE_CURVE('',#20292,#20293,#9935,.T.);
#24798=EDGE_CURVE('',#20293,#20294,#9936,.T.);
#24799=EDGE_CURVE('',#20294,#20295,#9937,.T.);
#24800=EDGE_CURVE('',#20295,#20296,#9938,.T.);
#24801=EDGE_CURVE('',#20296,#20297,#9939,.T.);
#24802=EDGE_CURVE('',#20297,#20292,#9940,.T.);
#24803=EDGE_CURVE('',#20298,#20299,#9941,.T.);
#24804=EDGE_CURVE('',#20299,#20300,#9942,.T.);
#24805=EDGE_CURVE('',#20300,#20301,#9943,.T.);
#24806=EDGE_CURVE('',#20301,#20302,#9944,.T.);
#24807=EDGE_CURVE('',#20302,#20303,#9945,.T.);
#24808=EDGE_CURVE('',#20303,#20298,#9946,.T.);
#24809=EDGE_CURVE('',#20304,#20305,#9947,.T.);
#24810=EDGE_CURVE('',#20305,#20306,#9948,.T.);
#24811=EDGE_CURVE('',#20306,#20307,#9949,.T.);
#24812=EDGE_CURVE('',#20307,#20308,#9950,.T.);
#24813=EDGE_CURVE('',#20308,#20309,#9951,.T.);
#24814=EDGE_CURVE('',#20309,#20304,#9952,.T.);
#24815=EDGE_CURVE('',#20310,#20311,#9953,.T.);
#24816=EDGE_CURVE('',#20311,#20312,#9954,.T.);
#24817=EDGE_CURVE('',#20312,#20313,#9955,.T.);
#24818=EDGE_CURVE('',#20313,#20314,#9956,.T.);
#24819=EDGE_CURVE('',#20314,#20315,#9957,.T.);
#24820=EDGE_CURVE('',#20315,#20310,#9958,.T.);
#24821=EDGE_CURVE('',#20316,#20317,#9959,.T.);
#24822=EDGE_CURVE('',#20317,#20318,#9960,.T.);
#24823=EDGE_CURVE('',#20318,#20319,#9961,.T.);
#24824=EDGE_CURVE('',#20319,#20320,#9962,.T.);
#24825=EDGE_CURVE('',#20320,#20321,#9963,.T.);
#24826=EDGE_CURVE('',#20321,#20316,#9964,.T.);
#24827=EDGE_CURVE('',#20322,#20323,#9965,.T.);
#24828=EDGE_CURVE('',#20323,#20324,#9966,.T.);
#24829=EDGE_CURVE('',#20324,#20325,#9967,.T.);
#24830=EDGE_CURVE('',#20325,#20326,#9968,.T.);
#24831=EDGE_CURVE('',#20326,#20327,#9969,.T.);
#24832=EDGE_CURVE('',#20327,#20322,#9970,.T.);
#24833=EDGE_CURVE('',#20328,#20329,#9971,.T.);
#24834=EDGE_CURVE('',#20329,#20330,#9972,.T.);
#24835=EDGE_CURVE('',#20330,#20331,#9973,.T.);
#24836=EDGE_CURVE('',#20331,#20332,#9974,.T.);
#24837=EDGE_CURVE('',#20332,#20333,#9975,.T.);
#24838=EDGE_CURVE('',#20333,#20328,#9976,.T.);
#24839=EDGE_CURVE('',#20334,#20335,#9977,.T.);
#24840=EDGE_CURVE('',#20335,#20336,#9978,.T.);
#24841=EDGE_CURVE('',#20336,#20337,#9979,.T.);
#24842=EDGE_CURVE('',#20337,#20338,#9980,.T.);
#24843=EDGE_CURVE('',#20338,#20339,#9981,.T.);
#24844=EDGE_CURVE('',#20339,#20334,#9982,.T.);
#24845=EDGE_CURVE('',#20340,#20341,#9983,.T.);
#24846=EDGE_CURVE('',#20341,#20342,#9984,.T.);
#24847=EDGE_CURVE('',#20342,#20343,#9985,.T.);
#24848=EDGE_CURVE('',#20343,#20344,#9986,.T.);
#24849=EDGE_CURVE('',#20344,#20345,#9987,.T.);
#24850=EDGE_CURVE('',#20345,#20340,#9988,.T.);
#24851=EDGE_CURVE('',#20346,#20347,#9989,.T.);
#24852=EDGE_CURVE('',#20347,#20348,#9990,.T.);
#24853=EDGE_CURVE('',#20348,#20349,#9991,.T.);
#24854=EDGE_CURVE('',#20349,#20350,#9992,.T.);
#24855=EDGE_CURVE('',#20350,#20351,#9993,.T.);
#24856=EDGE_CURVE('',#20351,#20346,#9994,.T.);
#24857=EDGE_CURVE('',#20352,#20353,#9995,.T.);
#24858=EDGE_CURVE('',#20353,#20354,#9996,.T.);
#24859=EDGE_CURVE('',#20354,#20355,#9997,.T.);
#24860=EDGE_CURVE('',#20355,#20356,#9998,.T.);
#24861=EDGE_CURVE('',#20356,#20357,#9999,.T.);
#24862=EDGE_CURVE('',#20357,#20352,#10000,.T.);
#24863=EDGE_CURVE('',#20358,#20359,#10001,.T.);
#24864=EDGE_CURVE('',#20359,#20360,#10002,.T.);
#24865=EDGE_CURVE('',#20360,#20361,#10003,.T.);
#24866=EDGE_CURVE('',#20361,#20362,#10004,.T.);
#24867=EDGE_CURVE('',#20362,#20363,#10005,.T.);
#24868=EDGE_CURVE('',#20363,#20358,#10006,.T.);
#24869=EDGE_CURVE('',#20364,#20365,#10007,.T.);
#24870=EDGE_CURVE('',#20365,#20366,#10008,.T.);
#24871=EDGE_CURVE('',#20366,#20367,#10009,.T.);
#24872=EDGE_CURVE('',#20367,#20368,#10010,.T.);
#24873=EDGE_CURVE('',#20368,#20369,#10011,.T.);
#24874=EDGE_CURVE('',#20369,#20364,#10012,.T.);
#24875=EDGE_CURVE('',#20370,#20371,#10013,.T.);
#24876=EDGE_CURVE('',#20371,#20372,#10014,.T.);
#24877=EDGE_CURVE('',#20372,#20373,#10015,.T.);
#24878=EDGE_CURVE('',#20373,#20374,#10016,.T.);
#24879=EDGE_CURVE('',#20374,#20375,#10017,.T.);
#24880=EDGE_CURVE('',#20375,#20370,#10018,.T.);
#24881=EDGE_CURVE('',#20376,#20377,#10019,.T.);
#24882=EDGE_CURVE('',#20377,#20378,#10020,.T.);
#24883=EDGE_CURVE('',#20378,#20379,#10021,.T.);
#24884=EDGE_CURVE('',#20379,#20380,#10022,.T.);
#24885=EDGE_CURVE('',#20380,#20381,#10023,.T.);
#24886=EDGE_CURVE('',#20381,#20376,#10024,.T.);
#24887=EDGE_CURVE('',#20382,#20383,#10025,.T.);
#24888=EDGE_CURVE('',#20383,#20384,#10026,.T.);
#24889=EDGE_CURVE('',#20384,#20385,#10027,.T.);
#24890=EDGE_CURVE('',#20385,#20386,#10028,.T.);
#24891=EDGE_CURVE('',#20386,#20387,#10029,.T.);
#24892=EDGE_CURVE('',#20387,#20382,#10030,.T.);
#24893=EDGE_CURVE('',#20388,#20389,#10031,.T.);
#24894=EDGE_CURVE('',#20389,#20390,#10032,.T.);
#24895=EDGE_CURVE('',#20390,#20391,#10033,.T.);
#24896=EDGE_CURVE('',#20391,#20392,#10034,.T.);
#24897=EDGE_CURVE('',#20392,#20393,#10035,.T.);
#24898=EDGE_CURVE('',#20393,#20388,#10036,.T.);
#24899=EDGE_CURVE('',#20394,#20395,#10037,.T.);
#24900=EDGE_CURVE('',#20395,#20396,#10038,.T.);
#24901=EDGE_CURVE('',#20396,#20397,#10039,.T.);
#24902=EDGE_CURVE('',#20397,#20398,#10040,.T.);
#24903=EDGE_CURVE('',#20398,#20399,#10041,.T.);
#24904=EDGE_CURVE('',#20399,#20394,#10042,.T.);
#24905=EDGE_CURVE('',#20400,#20401,#10043,.T.);
#24906=EDGE_CURVE('',#20401,#20402,#10044,.T.);
#24907=EDGE_CURVE('',#20402,#20403,#10045,.T.);
#24908=EDGE_CURVE('',#20403,#20404,#10046,.T.);
#24909=EDGE_CURVE('',#20404,#20405,#10047,.T.);
#24910=EDGE_CURVE('',#20405,#20400,#10048,.T.);
#24911=EDGE_CURVE('',#20406,#20407,#10049,.T.);
#24912=EDGE_CURVE('',#20407,#20408,#10050,.T.);
#24913=EDGE_CURVE('',#20408,#20409,#10051,.T.);
#24914=EDGE_CURVE('',#20409,#20410,#10052,.T.);
#24915=EDGE_CURVE('',#20410,#20411,#10053,.T.);
#24916=EDGE_CURVE('',#20411,#20406,#10054,.T.);
#24917=EDGE_CURVE('',#20412,#20413,#10055,.T.);
#24918=EDGE_CURVE('',#20413,#20414,#10056,.T.);
#24919=EDGE_CURVE('',#20414,#20415,#10057,.T.);
#24920=EDGE_CURVE('',#20415,#20416,#10058,.T.);
#24921=EDGE_CURVE('',#20416,#20417,#10059,.T.);
#24922=EDGE_CURVE('',#20417,#20412,#10060,.T.);
#24923=EDGE_CURVE('',#20418,#20419,#10061,.T.);
#24924=EDGE_CURVE('',#20419,#20420,#10062,.T.);
#24925=EDGE_CURVE('',#20420,#20421,#10063,.T.);
#24926=EDGE_CURVE('',#20421,#20422,#10064,.T.);
#24927=EDGE_CURVE('',#20422,#20423,#10065,.T.);
#24928=EDGE_CURVE('',#20423,#20418,#10066,.T.);
#24929=EDGE_CURVE('',#20424,#20425,#10067,.T.);
#24930=EDGE_CURVE('',#20425,#20426,#10068,.T.);
#24931=EDGE_CURVE('',#20426,#20427,#10069,.T.);
#24932=EDGE_CURVE('',#20427,#20428,#10070,.T.);
#24933=EDGE_CURVE('',#20428,#20429,#10071,.T.);
#24934=EDGE_CURVE('',#20429,#20424,#10072,.T.);
#24935=EDGE_CURVE('',#20430,#20431,#10073,.T.);
#24936=EDGE_CURVE('',#20431,#20432,#10074,.T.);
#24937=EDGE_CURVE('',#20432,#20433,#10075,.T.);
#24938=EDGE_CURVE('',#20433,#20434,#10076,.T.);
#24939=EDGE_CURVE('',#20434,#20435,#10077,.T.);
#24940=EDGE_CURVE('',#20435,#20430,#10078,.T.);
#24941=EDGE_CURVE('',#20436,#20437,#10079,.T.);
#24942=EDGE_CURVE('',#20437,#20438,#10080,.T.);
#24943=EDGE_CURVE('',#20438,#20439,#10081,.T.);
#24944=EDGE_CURVE('',#20439,#20440,#10082,.T.);
#24945=EDGE_CURVE('',#20440,#20441,#10083,.T.);
#24946=EDGE_CURVE('',#20441,#20436,#10084,.T.);
#24947=EDGE_CURVE('',#20442,#20443,#10085,.T.);
#24948=EDGE_CURVE('',#20443,#20444,#10086,.T.);
#24949=EDGE_CURVE('',#20444,#20445,#10087,.T.);
#24950=EDGE_CURVE('',#20445,#20446,#10088,.T.);
#24951=EDGE_CURVE('',#20446,#20447,#10089,.T.);
#24952=EDGE_CURVE('',#20447,#20442,#10090,.T.);
#24953=EDGE_CURVE('',#20448,#20449,#10091,.T.);
#24954=EDGE_CURVE('',#20449,#20450,#10092,.T.);
#24955=EDGE_CURVE('',#20450,#20451,#10093,.T.);
#24956=EDGE_CURVE('',#20451,#20452,#10094,.T.);
#24957=EDGE_CURVE('',#20452,#20453,#10095,.T.);
#24958=EDGE_CURVE('',#20453,#20448,#10096,.T.);
#24959=EDGE_CURVE('',#20454,#20455,#10097,.T.);
#24960=EDGE_CURVE('',#20455,#20456,#10098,.T.);
#24961=EDGE_CURVE('',#20456,#20457,#10099,.T.);
#24962=EDGE_CURVE('',#20457,#20458,#10100,.T.);
#24963=EDGE_CURVE('',#20458,#20459,#10101,.T.);
#24964=EDGE_CURVE('',#20459,#20454,#10102,.T.);
#24965=EDGE_CURVE('',#20460,#20461,#10103,.T.);
#24966=EDGE_CURVE('',#20461,#20462,#10104,.T.);
#24967=EDGE_CURVE('',#20462,#20463,#10105,.T.);
#24968=EDGE_CURVE('',#20463,#20464,#10106,.T.);
#24969=EDGE_CURVE('',#20464,#20465,#10107,.T.);
#24970=EDGE_CURVE('',#20465,#20460,#10108,.T.);
#24971=EDGE_CURVE('',#20466,#20467,#10109,.T.);
#24972=EDGE_CURVE('',#20467,#20468,#10110,.T.);
#24973=EDGE_CURVE('',#20468,#20469,#10111,.T.);
#24974=EDGE_CURVE('',#20469,#20470,#10112,.T.);
#24975=EDGE_CURVE('',#20470,#20471,#10113,.T.);
#24976=EDGE_CURVE('',#20471,#20466,#10114,.T.);
#24977=EDGE_CURVE('',#20472,#20473,#10115,.T.);
#24978=EDGE_CURVE('',#20473,#20474,#10116,.T.);
#24979=EDGE_CURVE('',#20474,#20475,#10117,.T.);
#24980=EDGE_CURVE('',#20475,#20476,#10118,.T.);
#24981=EDGE_CURVE('',#20476,#20477,#10119,.T.);
#24982=EDGE_CURVE('',#20477,#20472,#10120,.T.);
#24983=EDGE_CURVE('',#20478,#20479,#10121,.T.);
#24984=EDGE_CURVE('',#20479,#20480,#10122,.T.);
#24985=EDGE_CURVE('',#20480,#20481,#10123,.T.);
#24986=EDGE_CURVE('',#20481,#20482,#10124,.T.);
#24987=EDGE_CURVE('',#20482,#20483,#10125,.T.);
#24988=EDGE_CURVE('',#20483,#20478,#10126,.T.);
#24989=EDGE_CURVE('',#20484,#20485,#10127,.T.);
#24990=EDGE_CURVE('',#20485,#20486,#10128,.T.);
#24991=EDGE_CURVE('',#20486,#20487,#10129,.T.);
#24992=EDGE_CURVE('',#20487,#20488,#10130,.T.);
#24993=EDGE_CURVE('',#20488,#20489,#10131,.T.);
#24994=EDGE_CURVE('',#20489,#20484,#10132,.T.);
#24995=EDGE_CURVE('',#20490,#20491,#10133,.T.);
#24996=EDGE_CURVE('',#20491,#20492,#10134,.T.);
#24997=EDGE_CURVE('',#20492,#20493,#10135,.T.);
#24998=EDGE_CURVE('',#20493,#20494,#10136,.T.);
#24999=EDGE_CURVE('',#20494,#20495,#10137,.T.);
#25000=EDGE_CURVE('',#20495,#20490,#10138,.T.);
#25001=EDGE_CURVE('',#20496,#20497,#10139,.T.);
#25002=EDGE_CURVE('',#20497,#20498,#10140,.T.);
#25003=EDGE_CURVE('',#20498,#20499,#10141,.T.);
#25004=EDGE_CURVE('',#20499,#20500,#10142,.T.);
#25005=EDGE_CURVE('',#20500,#20501,#10143,.T.);
#25006=EDGE_CURVE('',#20501,#20496,#10144,.T.);
#25007=EDGE_CURVE('',#20502,#20503,#10145,.T.);
#25008=EDGE_CURVE('',#20503,#20504,#10146,.T.);
#25009=EDGE_CURVE('',#20504,#20505,#10147,.T.);
#25010=EDGE_CURVE('',#20505,#20506,#10148,.T.);
#25011=EDGE_CURVE('',#20506,#20507,#10149,.T.);
#25012=EDGE_CURVE('',#20507,#20502,#10150,.T.);
#25013=EDGE_CURVE('',#20508,#20509,#10151,.T.);
#25014=EDGE_CURVE('',#20509,#20510,#10152,.T.);
#25015=EDGE_CURVE('',#20510,#20511,#10153,.T.);
#25016=EDGE_CURVE('',#20511,#20512,#10154,.T.);
#25017=EDGE_CURVE('',#20512,#20513,#10155,.T.);
#25018=EDGE_CURVE('',#20513,#20508,#10156,.T.);
#25019=EDGE_CURVE('',#20514,#20515,#10157,.T.);
#25020=EDGE_CURVE('',#20515,#20516,#10158,.T.);
#25021=EDGE_CURVE('',#20516,#20517,#10159,.T.);
#25022=EDGE_CURVE('',#20517,#20518,#10160,.T.);
#25023=EDGE_CURVE('',#20518,#20519,#10161,.T.);
#25024=EDGE_CURVE('',#20519,#20514,#10162,.T.);
#25025=EDGE_CURVE('',#20520,#20521,#10163,.T.);
#25026=EDGE_CURVE('',#20521,#20522,#10164,.T.);
#25027=EDGE_CURVE('',#20522,#20523,#10165,.T.);
#25028=EDGE_CURVE('',#20523,#20524,#10166,.T.);
#25029=EDGE_CURVE('',#20524,#20525,#10167,.T.);
#25030=EDGE_CURVE('',#20525,#20520,#10168,.T.);
#25031=EDGE_CURVE('',#20526,#20527,#10169,.T.);
#25032=EDGE_CURVE('',#20527,#20528,#10170,.T.);
#25033=EDGE_CURVE('',#20528,#20529,#10171,.T.);
#25034=EDGE_CURVE('',#20529,#20530,#10172,.T.);
#25035=EDGE_CURVE('',#20530,#20531,#10173,.T.);
#25036=EDGE_CURVE('',#20531,#20526,#10174,.T.);
#25037=EDGE_CURVE('',#20532,#20533,#10175,.T.);
#25038=EDGE_CURVE('',#20533,#20534,#10176,.T.);
#25039=EDGE_CURVE('',#20534,#20535,#10177,.T.);
#25040=EDGE_CURVE('',#20535,#20536,#10178,.T.);
#25041=EDGE_CURVE('',#20536,#20537,#10179,.T.);
#25042=EDGE_CURVE('',#20537,#20532,#10180,.T.);
#25043=EDGE_CURVE('',#20538,#20539,#10181,.T.);
#25044=EDGE_CURVE('',#20539,#20540,#10182,.T.);
#25045=EDGE_CURVE('',#20540,#20541,#10183,.T.);
#25046=EDGE_CURVE('',#20541,#20542,#10184,.T.);
#25047=EDGE_CURVE('',#20542,#20543,#10185,.T.);
#25048=EDGE_CURVE('',#20543,#20538,#10186,.T.);
#25049=EDGE_CURVE('',#20544,#20545,#10187,.T.);
#25050=EDGE_CURVE('',#20545,#20546,#10188,.T.);
#25051=EDGE_CURVE('',#20546,#20547,#10189,.T.);
#25052=EDGE_CURVE('',#20547,#20548,#10190,.T.);
#25053=EDGE_CURVE('',#20548,#20549,#10191,.T.);
#25054=EDGE_CURVE('',#20549,#20544,#10192,.T.);
#25055=EDGE_CURVE('',#20550,#20551,#10193,.T.);
#25056=EDGE_CURVE('',#20551,#20552,#10194,.T.);
#25057=EDGE_CURVE('',#20552,#20553,#10195,.T.);
#25058=EDGE_CURVE('',#20553,#20554,#10196,.T.);
#25059=EDGE_CURVE('',#20554,#20555,#10197,.T.);
#25060=EDGE_CURVE('',#20555,#20550,#10198,.T.);
#25061=EDGE_CURVE('',#20556,#20557,#10199,.T.);
#25062=EDGE_CURVE('',#20557,#20558,#10200,.T.);
#25063=EDGE_CURVE('',#20558,#20559,#10201,.T.);
#25064=EDGE_CURVE('',#20559,#20560,#10202,.T.);
#25065=EDGE_CURVE('',#20560,#20561,#10203,.T.);
#25066=EDGE_CURVE('',#20561,#20556,#10204,.T.);
#25067=EDGE_CURVE('',#20562,#20563,#10205,.T.);
#25068=EDGE_CURVE('',#20563,#20564,#10206,.T.);
#25069=EDGE_CURVE('',#20564,#20565,#10207,.T.);
#25070=EDGE_CURVE('',#20565,#20566,#10208,.T.);
#25071=EDGE_CURVE('',#20566,#20567,#10209,.T.);
#25072=EDGE_CURVE('',#20567,#20562,#10210,.T.);
#25073=EDGE_CURVE('',#20568,#20569,#10211,.T.);
#25074=EDGE_CURVE('',#20569,#20570,#10212,.T.);
#25075=EDGE_CURVE('',#20570,#20571,#10213,.T.);
#25076=EDGE_CURVE('',#20571,#20572,#10214,.T.);
#25077=EDGE_CURVE('',#20572,#20573,#10215,.T.);
#25078=EDGE_CURVE('',#20573,#20568,#10216,.T.);
#25079=EDGE_CURVE('',#20574,#20575,#10217,.T.);
#25080=EDGE_CURVE('',#20575,#20576,#10218,.T.);
#25081=EDGE_CURVE('',#20576,#20577,#10219,.T.);
#25082=EDGE_CURVE('',#20577,#20578,#10220,.T.);
#25083=EDGE_CURVE('',#20578,#20579,#10221,.T.);
#25084=EDGE_CURVE('',#20579,#20574,#10222,.T.);
#25085=EDGE_CURVE('',#20580,#20581,#10223,.T.);
#25086=EDGE_CURVE('',#20581,#20582,#10224,.T.);
#25087=EDGE_CURVE('',#20582,#20583,#10225,.T.);
#25088=EDGE_CURVE('',#20583,#20584,#10226,.T.);
#25089=EDGE_CURVE('',#20584,#20585,#10227,.T.);
#25090=EDGE_CURVE('',#20585,#20580,#10228,.T.);
#25091=EDGE_CURVE('',#20586,#20587,#10229,.T.);
#25092=EDGE_CURVE('',#20587,#20588,#10230,.T.);
#25093=EDGE_CURVE('',#20588,#20589,#10231,.T.);
#25094=EDGE_CURVE('',#20589,#20590,#10232,.T.);
#25095=EDGE_CURVE('',#20590,#20591,#10233,.T.);
#25096=EDGE_CURVE('',#20591,#20586,#10234,.T.);
#25097=EDGE_CURVE('',#20592,#20593,#10235,.T.);
#25098=EDGE_CURVE('',#20593,#20594,#10236,.T.);
#25099=EDGE_CURVE('',#20594,#20595,#10237,.T.);
#25100=EDGE_CURVE('',#20595,#20596,#10238,.T.);
#25101=EDGE_CURVE('',#20596,#20597,#10239,.T.);
#25102=EDGE_CURVE('',#20597,#20592,#10240,.T.);
#25103=EDGE_CURVE('',#20598,#20599,#10241,.T.);
#25104=EDGE_CURVE('',#20599,#20600,#10242,.T.);
#25105=EDGE_CURVE('',#20600,#20601,#10243,.T.);
#25106=EDGE_CURVE('',#20601,#20602,#10244,.T.);
#25107=EDGE_CURVE('',#20602,#20603,#10245,.T.);
#25108=EDGE_CURVE('',#20603,#20598,#10246,.T.);
#25109=EDGE_CURVE('',#20604,#20605,#10247,.T.);
#25110=EDGE_CURVE('',#20605,#20606,#10248,.T.);
#25111=EDGE_CURVE('',#20606,#20607,#10249,.T.);
#25112=EDGE_CURVE('',#20607,#20608,#10250,.T.);
#25113=EDGE_CURVE('',#20608,#20609,#10251,.T.);
#25114=EDGE_CURVE('',#20609,#20604,#10252,.T.);
#25115=EDGE_CURVE('',#20610,#20611,#10253,.T.);
#25116=EDGE_CURVE('',#20611,#20612,#10254,.T.);
#25117=EDGE_CURVE('',#20612,#20613,#10255,.T.);
#25118=EDGE_CURVE('',#20613,#20614,#10256,.T.);
#25119=EDGE_CURVE('',#20614,#20615,#10257,.T.);
#25120=EDGE_CURVE('',#20615,#20610,#10258,.T.);
#25121=EDGE_CURVE('',#20616,#20617,#10259,.T.);
#25122=EDGE_CURVE('',#20617,#20618,#10260,.T.);
#25123=EDGE_CURVE('',#20618,#20619,#10261,.T.);
#25124=EDGE_CURVE('',#20619,#20620,#10262,.T.);
#25125=EDGE_CURVE('',#20620,#20621,#10263,.T.);
#25126=EDGE_CURVE('',#20621,#20616,#10264,.T.);
#25127=EDGE_CURVE('',#20622,#20623,#10265,.T.);
#25128=EDGE_CURVE('',#20623,#20624,#10266,.T.);
#25129=EDGE_CURVE('',#20624,#20625,#10267,.T.);
#25130=EDGE_CURVE('',#20625,#20626,#10268,.T.);
#25131=EDGE_CURVE('',#20626,#20627,#10269,.T.);
#25132=EDGE_CURVE('',#20627,#20622,#10270,.T.);
#25133=EDGE_CURVE('',#20628,#20629,#10271,.T.);
#25134=EDGE_CURVE('',#20629,#20630,#10272,.T.);
#25135=EDGE_CURVE('',#20630,#20631,#10273,.T.);
#25136=EDGE_CURVE('',#20631,#20632,#10274,.T.);
#25137=EDGE_CURVE('',#20632,#20633,#10275,.T.);
#25138=EDGE_CURVE('',#20633,#20628,#10276,.T.);
#25139=EDGE_CURVE('',#20634,#20635,#10277,.T.);
#25140=EDGE_CURVE('',#20635,#20636,#10278,.T.);
#25141=EDGE_CURVE('',#20636,#20637,#10279,.T.);
#25142=EDGE_CURVE('',#20637,#20638,#10280,.T.);
#25143=EDGE_CURVE('',#20638,#20639,#10281,.T.);
#25144=EDGE_CURVE('',#20639,#20634,#10282,.T.);
#25145=EDGE_CURVE('',#20640,#20641,#10283,.T.);
#25146=EDGE_CURVE('',#20641,#20642,#10284,.T.);
#25147=EDGE_CURVE('',#20642,#20643,#10285,.T.);
#25148=EDGE_CURVE('',#20643,#20644,#10286,.T.);
#25149=EDGE_CURVE('',#20644,#20645,#10287,.T.);
#25150=EDGE_CURVE('',#20645,#20640,#10288,.T.);
#25151=EDGE_CURVE('',#20646,#20647,#10289,.T.);
#25152=EDGE_CURVE('',#20647,#20648,#10290,.T.);
#25153=EDGE_CURVE('',#20648,#20649,#10291,.T.);
#25154=EDGE_CURVE('',#20649,#20650,#10292,.T.);
#25155=EDGE_CURVE('',#20650,#20651,#10293,.T.);
#25156=EDGE_CURVE('',#20651,#20646,#10294,.T.);
#25157=EDGE_CURVE('',#20652,#20653,#10295,.T.);
#25158=EDGE_CURVE('',#20653,#20654,#10296,.T.);
#25159=EDGE_CURVE('',#20654,#20655,#10297,.T.);
#25160=EDGE_CURVE('',#20655,#20656,#10298,.T.);
#25161=EDGE_CURVE('',#20656,#20657,#10299,.T.);
#25162=EDGE_CURVE('',#20657,#20652,#10300,.T.);
#25163=EDGE_CURVE('',#20658,#20659,#10301,.T.);
#25164=EDGE_CURVE('',#20659,#20660,#10302,.T.);
#25165=EDGE_CURVE('',#20660,#20661,#10303,.T.);
#25166=EDGE_CURVE('',#20661,#20662,#10304,.T.);
#25167=EDGE_CURVE('',#20662,#20663,#10305,.T.);
#25168=EDGE_CURVE('',#20663,#20658,#10306,.T.);
#25169=EDGE_CURVE('',#20664,#20665,#10307,.T.);
#25170=EDGE_CURVE('',#20665,#20666,#10308,.T.);
#25171=EDGE_CURVE('',#20666,#20667,#10309,.T.);
#25172=EDGE_CURVE('',#20667,#20668,#10310,.T.);
#25173=EDGE_CURVE('',#20668,#20669,#10311,.T.);
#25174=EDGE_CURVE('',#20669,#20664,#10312,.T.);
#25175=EDGE_CURVE('',#20670,#20671,#10313,.T.);
#25176=EDGE_CURVE('',#20671,#20672,#10314,.T.);
#25177=EDGE_CURVE('',#20672,#20673,#10315,.T.);
#25178=EDGE_CURVE('',#20673,#20674,#10316,.T.);
#25179=EDGE_CURVE('',#20674,#20675,#10317,.T.);
#25180=EDGE_CURVE('',#20675,#20670,#10318,.T.);
#25181=EDGE_CURVE('',#20676,#20677,#10319,.T.);
#25182=EDGE_CURVE('',#20677,#20678,#10320,.T.);
#25183=EDGE_CURVE('',#20678,#20679,#10321,.T.);
#25184=EDGE_CURVE('',#20679,#20680,#10322,.T.);
#25185=EDGE_CURVE('',#20680,#20681,#10323,.T.);
#25186=EDGE_CURVE('',#20681,#20676,#10324,.T.);
#25187=EDGE_CURVE('',#20682,#20683,#10325,.T.);
#25188=EDGE_CURVE('',#20683,#20684,#10326,.T.);
#25189=EDGE_CURVE('',#20684,#20685,#10327,.T.);
#25190=EDGE_CURVE('',#20685,#20686,#10328,.T.);
#25191=EDGE_CURVE('',#20686,#20687,#10329,.T.);
#25192=EDGE_CURVE('',#20687,#20682,#10330,.T.);
#25193=EDGE_CURVE('',#20688,#20689,#10331,.T.);
#25194=EDGE_CURVE('',#20689,#20690,#10332,.T.);
#25195=EDGE_CURVE('',#20690,#20691,#10333,.T.);
#25196=EDGE_CURVE('',#20691,#20692,#10334,.T.);
#25197=EDGE_CURVE('',#20692,#20693,#10335,.T.);
#25198=EDGE_CURVE('',#20693,#20688,#10336,.T.);
#25199=EDGE_CURVE('',#20694,#20695,#10337,.T.);
#25200=EDGE_CURVE('',#20695,#20696,#10338,.T.);
#25201=EDGE_CURVE('',#20696,#20697,#10339,.T.);
#25202=EDGE_CURVE('',#20697,#20698,#10340,.T.);
#25203=EDGE_CURVE('',#20698,#20699,#10341,.T.);
#25204=EDGE_CURVE('',#20699,#20694,#10342,.T.);
#25205=EDGE_CURVE('',#20700,#20701,#10343,.T.);
#25206=EDGE_CURVE('',#20701,#20702,#10344,.T.);
#25207=EDGE_CURVE('',#20702,#20703,#10345,.T.);
#25208=EDGE_CURVE('',#20703,#20704,#10346,.T.);
#25209=EDGE_CURVE('',#20704,#20705,#10347,.T.);
#25210=EDGE_CURVE('',#20705,#20700,#10348,.T.);
#25211=EDGE_CURVE('',#20706,#20707,#10349,.T.);
#25212=EDGE_CURVE('',#20707,#20708,#10350,.T.);
#25213=EDGE_CURVE('',#20708,#20709,#10351,.T.);
#25214=EDGE_CURVE('',#20709,#20710,#10352,.T.);
#25215=EDGE_CURVE('',#20710,#20711,#10353,.T.);
#25216=EDGE_CURVE('',#20711,#20706,#10354,.T.);
#25217=EDGE_CURVE('',#20712,#20713,#10355,.T.);
#25218=EDGE_CURVE('',#20713,#20714,#10356,.T.);
#25219=EDGE_CURVE('',#20714,#20715,#10357,.T.);
#25220=EDGE_CURVE('',#20715,#20716,#10358,.T.);
#25221=EDGE_CURVE('',#20716,#20717,#10359,.T.);
#25222=EDGE_CURVE('',#20717,#20712,#10360,.T.);
#25223=EDGE_CURVE('',#20718,#20719,#10361,.T.);
#25224=EDGE_CURVE('',#20719,#20720,#10362,.T.);
#25225=EDGE_CURVE('',#20720,#20721,#10363,.T.);
#25226=EDGE_CURVE('',#20721,#20722,#10364,.T.);
#25227=EDGE_CURVE('',#20722,#20723,#10365,.T.);
#25228=EDGE_CURVE('',#20723,#20718,#10366,.T.);
#25229=EDGE_CURVE('',#20724,#20725,#10367,.T.);
#25230=EDGE_CURVE('',#20725,#20726,#10368,.T.);
#25231=EDGE_CURVE('',#20726,#20727,#10369,.T.);
#25232=EDGE_CURVE('',#20727,#20728,#10370,.T.);
#25233=EDGE_CURVE('',#20728,#20729,#10371,.T.);
#25234=EDGE_CURVE('',#20729,#20724,#10372,.T.);
#25235=EDGE_CURVE('',#20730,#20731,#10373,.T.);
#25236=EDGE_CURVE('',#20731,#20732,#10374,.T.);
#25237=EDGE_CURVE('',#20732,#20733,#10375,.T.);
#25238=EDGE_CURVE('',#20733,#20734,#10376,.T.);
#25239=EDGE_CURVE('',#20734,#20735,#10377,.T.);
#25240=EDGE_CURVE('',#20735,#20730,#10378,.T.);
#25241=EDGE_CURVE('',#20736,#20737,#10379,.T.);
#25242=EDGE_CURVE('',#20737,#20738,#10380,.T.);
#25243=EDGE_CURVE('',#20738,#20739,#10381,.T.);
#25244=EDGE_CURVE('',#20739,#20740,#10382,.T.);
#25245=EDGE_CURVE('',#20740,#20741,#10383,.T.);
#25246=EDGE_CURVE('',#20741,#20736,#10384,.T.);
#25247=EDGE_CURVE('',#20742,#20743,#10385,.T.);
#25248=EDGE_CURVE('',#20743,#20744,#10386,.T.);
#25249=EDGE_CURVE('',#20744,#20745,#10387,.T.);
#25250=EDGE_CURVE('',#20745,#20746,#10388,.T.);
#25251=EDGE_CURVE('',#20746,#20747,#10389,.T.);
#25252=EDGE_CURVE('',#20747,#20742,#10390,.T.);
#25253=EDGE_CURVE('',#20748,#20749,#10391,.T.);
#25254=EDGE_CURVE('',#20749,#20750,#10392,.T.);
#25255=EDGE_CURVE('',#20750,#20751,#10393,.T.);
#25256=EDGE_CURVE('',#20751,#20752,#10394,.T.);
#25257=EDGE_CURVE('',#20752,#20753,#10395,.T.);
#25258=EDGE_CURVE('',#20753,#20748,#10396,.T.);
#25259=EDGE_CURVE('',#20754,#20755,#10397,.T.);
#25260=EDGE_CURVE('',#20755,#20756,#10398,.T.);
#25261=EDGE_CURVE('',#20756,#20757,#10399,.T.);
#25262=EDGE_CURVE('',#20757,#20758,#10400,.T.);
#25263=EDGE_CURVE('',#20758,#20759,#10401,.T.);
#25264=EDGE_CURVE('',#20759,#20754,#10402,.T.);
#25265=EDGE_CURVE('',#20760,#20761,#10403,.T.);
#25266=EDGE_CURVE('',#20761,#20762,#10404,.T.);
#25267=EDGE_CURVE('',#20762,#20763,#10405,.T.);
#25268=EDGE_CURVE('',#20763,#20764,#10406,.T.);
#25269=EDGE_CURVE('',#20764,#20765,#10407,.T.);
#25270=EDGE_CURVE('',#20765,#20760,#10408,.T.);
#25271=EDGE_CURVE('',#20766,#20767,#10409,.T.);
#25272=EDGE_CURVE('',#20767,#20768,#10410,.T.);
#25273=EDGE_CURVE('',#20768,#20769,#10411,.T.);
#25274=EDGE_CURVE('',#20769,#20770,#10412,.T.);
#25275=EDGE_CURVE('',#20770,#20771,#10413,.T.);
#25276=EDGE_CURVE('',#20771,#20766,#10414,.T.);
#25277=EDGE_CURVE('',#20772,#20773,#10415,.T.);
#25278=EDGE_CURVE('',#20773,#20774,#10416,.T.);
#25279=EDGE_CURVE('',#20774,#20775,#10417,.T.);
#25280=EDGE_CURVE('',#20775,#20776,#10418,.T.);
#25281=EDGE_CURVE('',#20776,#20777,#10419,.T.);
#25282=EDGE_CURVE('',#20777,#20772,#10420,.T.);
#25283=EDGE_CURVE('',#20778,#20779,#10421,.T.);
#25284=EDGE_CURVE('',#20779,#20780,#10422,.T.);
#25285=EDGE_CURVE('',#20780,#20781,#10423,.T.);
#25286=EDGE_CURVE('',#20781,#20782,#10424,.T.);
#25287=EDGE_CURVE('',#20782,#20783,#10425,.T.);
#25288=EDGE_CURVE('',#20783,#20778,#10426,.T.);
#25289=EDGE_CURVE('',#20784,#20785,#10427,.T.);
#25290=EDGE_CURVE('',#20785,#20786,#10428,.T.);
#25291=EDGE_CURVE('',#20786,#20787,#10429,.T.);
#25292=EDGE_CURVE('',#20787,#20788,#10430,.T.);
#25293=EDGE_CURVE('',#20788,#20789,#10431,.T.);
#25294=EDGE_CURVE('',#20789,#20784,#10432,.T.);
#25295=EDGE_CURVE('',#20790,#20791,#10433,.T.);
#25296=EDGE_CURVE('',#20791,#20792,#10434,.T.);
#25297=EDGE_CURVE('',#20792,#20793,#10435,.T.);
#25298=EDGE_CURVE('',#20793,#20794,#10436,.T.);
#25299=EDGE_CURVE('',#20794,#20795,#10437,.T.);
#25300=EDGE_CURVE('',#20795,#20790,#10438,.T.);
#25301=EDGE_CURVE('',#20796,#20797,#10439,.T.);
#25302=EDGE_CURVE('',#20797,#20798,#10440,.T.);
#25303=EDGE_CURVE('',#20798,#20799,#10441,.T.);
#25304=EDGE_CURVE('',#20799,#20800,#10442,.T.);
#25305=EDGE_CURVE('',#20800,#20801,#10443,.T.);
#25306=EDGE_CURVE('',#20801,#20796,#10444,.T.);
#25307=EDGE_CURVE('',#20802,#20803,#10445,.T.);
#25308=EDGE_CURVE('',#20803,#20804,#10446,.T.);
#25309=EDGE_CURVE('',#20804,#20805,#10447,.T.);
#25310=EDGE_CURVE('',#20805,#20806,#10448,.T.);
#25311=EDGE_CURVE('',#20806,#20807,#10449,.T.);
#25312=EDGE_CURVE('',#20807,#20802,#10450,.T.);
#25313=EDGE_CURVE('',#20808,#20809,#10451,.T.);
#25314=EDGE_CURVE('',#20809,#20810,#10452,.T.);
#25315=EDGE_CURVE('',#20810,#20811,#10453,.T.);
#25316=EDGE_CURVE('',#20811,#20812,#10454,.T.);
#25317=EDGE_CURVE('',#20812,#20813,#10455,.T.);
#25318=EDGE_CURVE('',#20813,#20808,#10456,.T.);
#25319=EDGE_CURVE('',#20814,#20815,#10457,.T.);
#25320=EDGE_CURVE('',#20815,#20816,#10458,.T.);
#25321=EDGE_CURVE('',#20816,#20817,#10459,.T.);
#25322=EDGE_CURVE('',#20817,#20818,#10460,.T.);
#25323=EDGE_CURVE('',#20818,#20819,#10461,.T.);
#25324=EDGE_CURVE('',#20819,#20814,#10462,.T.);
#25325=EDGE_CURVE('',#20820,#20821,#10463,.T.);
#25326=EDGE_CURVE('',#20821,#20822,#10464,.T.);
#25327=EDGE_CURVE('',#20822,#20823,#10465,.T.);
#25328=EDGE_CURVE('',#20823,#20824,#10466,.T.);
#25329=EDGE_CURVE('',#20824,#20825,#10467,.T.);
#25330=EDGE_CURVE('',#20825,#20820,#10468,.T.);
#25331=EDGE_CURVE('',#20826,#20827,#10469,.T.);
#25332=EDGE_CURVE('',#20827,#20828,#10470,.T.);
#25333=EDGE_CURVE('',#20828,#20829,#10471,.T.);
#25334=EDGE_CURVE('',#20829,#20830,#10472,.T.);
#25335=EDGE_CURVE('',#20830,#20831,#10473,.T.);
#25336=EDGE_CURVE('',#20831,#20826,#10474,.T.);
#25337=EDGE_CURVE('',#20832,#20833,#10475,.T.);
#25338=EDGE_CURVE('',#20833,#20834,#10476,.T.);
#25339=EDGE_CURVE('',#20834,#20835,#10477,.T.);
#25340=EDGE_CURVE('',#20835,#20836,#10478,.T.);
#25341=EDGE_CURVE('',#20836,#20837,#10479,.T.);
#25342=EDGE_CURVE('',#20837,#20832,#10480,.T.);
#25343=EDGE_CURVE('',#20838,#20839,#10481,.T.);
#25344=EDGE_CURVE('',#20839,#20840,#10482,.T.);
#25345=EDGE_CURVE('',#20840,#20841,#10483,.T.);
#25346=EDGE_CURVE('',#20841,#20842,#10484,.T.);
#25347=EDGE_CURVE('',#20842,#20843,#10485,.T.);
#25348=EDGE_CURVE('',#20843,#20838,#10486,.T.);
#25349=EDGE_CURVE('',#20844,#20845,#10487,.T.);
#25350=EDGE_CURVE('',#20845,#20846,#10488,.T.);
#25351=EDGE_CURVE('',#20846,#20847,#10489,.T.);
#25352=EDGE_CURVE('',#20847,#20848,#10490,.T.);
#25353=EDGE_CURVE('',#20848,#20849,#10491,.T.);
#25354=EDGE_CURVE('',#20849,#20844,#10492,.T.);
#25355=EDGE_CURVE('',#20850,#20851,#10493,.T.);
#25356=EDGE_CURVE('',#20851,#20852,#10494,.T.);
#25357=EDGE_CURVE('',#20852,#20853,#10495,.T.);
#25358=EDGE_CURVE('',#20853,#20854,#10496,.T.);
#25359=EDGE_CURVE('',#20854,#20855,#10497,.T.);
#25360=EDGE_CURVE('',#20855,#20850,#10498,.T.);
#25361=EDGE_CURVE('',#20851,#19734,#10499,.T.);
#25362=EDGE_CURVE('',#20852,#19735,#10500,.T.);
#25363=EDGE_CURVE('',#20850,#19736,#10501,.T.);
#25364=EDGE_CURVE('',#20855,#19737,#10502,.T.);
#25365=EDGE_CURVE('',#20854,#19738,#10503,.T.);
#25366=EDGE_CURVE('',#20853,#19739,#10504,.T.);
#25367=EDGE_CURVE('',#20845,#19728,#10505,.T.);
#25368=EDGE_CURVE('',#20846,#19729,#10506,.T.);
#25369=EDGE_CURVE('',#20844,#19730,#10507,.T.);
#25370=EDGE_CURVE('',#20849,#19731,#10508,.T.);
#25371=EDGE_CURVE('',#20848,#19732,#10509,.T.);
#25372=EDGE_CURVE('',#20847,#19733,#10510,.T.);
#25373=EDGE_CURVE('',#20839,#19722,#10511,.T.);
#25374=EDGE_CURVE('',#20840,#19723,#10512,.T.);
#25375=EDGE_CURVE('',#20838,#19724,#10513,.T.);
#25376=EDGE_CURVE('',#20843,#19725,#10514,.T.);
#25377=EDGE_CURVE('',#20842,#19726,#10515,.T.);
#25378=EDGE_CURVE('',#20841,#19727,#10516,.T.);
#25379=EDGE_CURVE('',#20833,#19716,#10517,.T.);
#25380=EDGE_CURVE('',#20834,#19717,#10518,.T.);
#25381=EDGE_CURVE('',#20832,#19718,#10519,.T.);
#25382=EDGE_CURVE('',#20837,#19719,#10520,.T.);
#25383=EDGE_CURVE('',#20836,#19720,#10521,.T.);
#25384=EDGE_CURVE('',#20835,#19721,#10522,.T.);
#25385=EDGE_CURVE('',#20827,#19710,#10523,.T.);
#25386=EDGE_CURVE('',#20828,#19711,#10524,.T.);
#25387=EDGE_CURVE('',#20826,#19712,#10525,.T.);
#25388=EDGE_CURVE('',#20831,#19713,#10526,.T.);
#25389=EDGE_CURVE('',#20830,#19714,#10527,.T.);
#25390=EDGE_CURVE('',#20829,#19715,#10528,.T.);
#25391=EDGE_CURVE('',#20821,#19704,#10529,.T.);
#25392=EDGE_CURVE('',#20822,#19705,#10530,.T.);
#25393=EDGE_CURVE('',#20820,#19706,#10531,.T.);
#25394=EDGE_CURVE('',#20825,#19707,#10532,.T.);
#25395=EDGE_CURVE('',#20824,#19708,#10533,.T.);
#25396=EDGE_CURVE('',#20823,#19709,#10534,.T.);
#25397=EDGE_CURVE('',#20815,#19698,#10535,.T.);
#25398=EDGE_CURVE('',#20816,#19699,#10536,.T.);
#25399=EDGE_CURVE('',#20814,#19700,#10537,.T.);
#25400=EDGE_CURVE('',#20819,#19701,#10538,.T.);
#25401=EDGE_CURVE('',#20818,#19702,#10539,.T.);
#25402=EDGE_CURVE('',#20817,#19703,#10540,.T.);
#25403=EDGE_CURVE('',#20809,#19692,#10541,.T.);
#25404=EDGE_CURVE('',#20810,#19693,#10542,.T.);
#25405=EDGE_CURVE('',#20808,#19694,#10543,.T.);
#25406=EDGE_CURVE('',#20813,#19695,#10544,.T.);
#25407=EDGE_CURVE('',#20812,#19696,#10545,.T.);
#25408=EDGE_CURVE('',#20811,#19697,#10546,.T.);
#25409=EDGE_CURVE('',#20803,#19686,#10547,.T.);
#25410=EDGE_CURVE('',#20804,#19687,#10548,.T.);
#25411=EDGE_CURVE('',#20802,#19688,#10549,.T.);
#25412=EDGE_CURVE('',#20807,#19689,#10550,.T.);
#25413=EDGE_CURVE('',#20806,#19690,#10551,.T.);
#25414=EDGE_CURVE('',#20805,#19691,#10552,.T.);
#25415=EDGE_CURVE('',#20797,#19680,#10553,.T.);
#25416=EDGE_CURVE('',#20798,#19681,#10554,.T.);
#25417=EDGE_CURVE('',#20796,#19682,#10555,.T.);
#25418=EDGE_CURVE('',#20801,#19683,#10556,.T.);
#25419=EDGE_CURVE('',#20800,#19684,#10557,.T.);
#25420=EDGE_CURVE('',#20799,#19685,#10558,.T.);
#25421=EDGE_CURVE('',#20791,#19674,#10559,.T.);
#25422=EDGE_CURVE('',#20792,#19675,#10560,.T.);
#25423=EDGE_CURVE('',#20790,#19676,#10561,.T.);
#25424=EDGE_CURVE('',#20795,#19677,#10562,.T.);
#25425=EDGE_CURVE('',#20794,#19678,#10563,.T.);
#25426=EDGE_CURVE('',#20793,#19679,#10564,.T.);
#25427=EDGE_CURVE('',#20785,#19668,#10565,.T.);
#25428=EDGE_CURVE('',#20786,#19669,#10566,.T.);
#25429=EDGE_CURVE('',#20784,#19670,#10567,.T.);
#25430=EDGE_CURVE('',#20789,#19671,#10568,.T.);
#25431=EDGE_CURVE('',#20788,#19672,#10569,.T.);
#25432=EDGE_CURVE('',#20787,#19673,#10570,.T.);
#25433=EDGE_CURVE('',#20779,#19662,#10571,.T.);
#25434=EDGE_CURVE('',#20780,#19663,#10572,.T.);
#25435=EDGE_CURVE('',#20778,#19664,#10573,.T.);
#25436=EDGE_CURVE('',#20783,#19665,#10574,.T.);
#25437=EDGE_CURVE('',#20782,#19666,#10575,.T.);
#25438=EDGE_CURVE('',#20781,#19667,#10576,.T.);
#25439=EDGE_CURVE('',#20773,#19656,#10577,.T.);
#25440=EDGE_CURVE('',#20774,#19657,#10578,.T.);
#25441=EDGE_CURVE('',#20772,#19658,#10579,.T.);
#25442=EDGE_CURVE('',#20777,#19659,#10580,.T.);
#25443=EDGE_CURVE('',#20776,#19660,#10581,.T.);
#25444=EDGE_CURVE('',#20775,#19661,#10582,.T.);
#25445=EDGE_CURVE('',#20767,#19650,#10583,.T.);
#25446=EDGE_CURVE('',#20768,#19651,#10584,.T.);
#25447=EDGE_CURVE('',#20766,#19652,#10585,.T.);
#25448=EDGE_CURVE('',#20771,#19653,#10586,.T.);
#25449=EDGE_CURVE('',#20770,#19654,#10587,.T.);
#25450=EDGE_CURVE('',#20769,#19655,#10588,.T.);
#25451=EDGE_CURVE('',#20761,#19644,#10589,.T.);
#25452=EDGE_CURVE('',#20762,#19645,#10590,.T.);
#25453=EDGE_CURVE('',#20760,#19646,#10591,.T.);
#25454=EDGE_CURVE('',#20765,#19647,#10592,.T.);
#25455=EDGE_CURVE('',#20764,#19648,#10593,.T.);
#25456=EDGE_CURVE('',#20763,#19649,#10594,.T.);
#25457=EDGE_CURVE('',#20755,#19638,#10595,.T.);
#25458=EDGE_CURVE('',#20756,#19639,#10596,.T.);
#25459=EDGE_CURVE('',#20754,#19640,#10597,.T.);
#25460=EDGE_CURVE('',#20759,#19641,#10598,.T.);
#25461=EDGE_CURVE('',#20758,#19642,#10599,.T.);
#25462=EDGE_CURVE('',#20757,#19643,#10600,.T.);
#25463=EDGE_CURVE('',#20749,#19632,#10601,.T.);
#25464=EDGE_CURVE('',#20750,#19633,#10602,.T.);
#25465=EDGE_CURVE('',#20748,#19634,#10603,.T.);
#25466=EDGE_CURVE('',#20753,#19635,#10604,.T.);
#25467=EDGE_CURVE('',#20752,#19636,#10605,.T.);
#25468=EDGE_CURVE('',#20751,#19637,#10606,.T.);
#25469=EDGE_CURVE('',#20743,#19626,#10607,.T.);
#25470=EDGE_CURVE('',#20744,#19627,#10608,.T.);
#25471=EDGE_CURVE('',#20742,#19628,#10609,.T.);
#25472=EDGE_CURVE('',#20747,#19629,#10610,.T.);
#25473=EDGE_CURVE('',#20746,#19630,#10611,.T.);
#25474=EDGE_CURVE('',#20745,#19631,#10612,.T.);
#25475=EDGE_CURVE('',#20737,#19620,#10613,.T.);
#25476=EDGE_CURVE('',#20738,#19621,#10614,.T.);
#25477=EDGE_CURVE('',#20736,#19622,#10615,.T.);
#25478=EDGE_CURVE('',#20741,#19623,#10616,.T.);
#25479=EDGE_CURVE('',#20740,#19624,#10617,.T.);
#25480=EDGE_CURVE('',#20739,#19625,#10618,.T.);
#25481=EDGE_CURVE('',#20731,#19614,#10619,.T.);
#25482=EDGE_CURVE('',#20732,#19615,#10620,.T.);
#25483=EDGE_CURVE('',#20730,#19616,#10621,.T.);
#25484=EDGE_CURVE('',#20735,#19617,#10622,.T.);
#25485=EDGE_CURVE('',#20734,#19618,#10623,.T.);
#25486=EDGE_CURVE('',#20733,#19619,#10624,.T.);
#25487=EDGE_CURVE('',#20725,#19608,#10625,.T.);
#25488=EDGE_CURVE('',#20726,#19609,#10626,.T.);
#25489=EDGE_CURVE('',#20724,#19610,#10627,.T.);
#25490=EDGE_CURVE('',#20729,#19611,#10628,.T.);
#25491=EDGE_CURVE('',#20728,#19612,#10629,.T.);
#25492=EDGE_CURVE('',#20727,#19613,#10630,.T.);
#25493=EDGE_CURVE('',#20719,#19602,#10631,.T.);
#25494=EDGE_CURVE('',#20720,#19603,#10632,.T.);
#25495=EDGE_CURVE('',#20718,#19604,#10633,.T.);
#25496=EDGE_CURVE('',#20723,#19605,#10634,.T.);
#25497=EDGE_CURVE('',#20722,#19606,#10635,.T.);
#25498=EDGE_CURVE('',#20721,#19607,#10636,.T.);
#25499=EDGE_CURVE('',#20713,#19596,#10637,.T.);
#25500=EDGE_CURVE('',#20714,#19597,#10638,.T.);
#25501=EDGE_CURVE('',#20712,#19598,#10639,.T.);
#25502=EDGE_CURVE('',#20717,#19599,#10640,.T.);
#25503=EDGE_CURVE('',#20716,#19600,#10641,.T.);
#25504=EDGE_CURVE('',#20715,#19601,#10642,.T.);
#25505=EDGE_CURVE('',#20707,#19590,#10643,.T.);
#25506=EDGE_CURVE('',#20708,#19591,#10644,.T.);
#25507=EDGE_CURVE('',#20706,#19592,#10645,.T.);
#25508=EDGE_CURVE('',#20711,#19593,#10646,.T.);
#25509=EDGE_CURVE('',#20710,#19594,#10647,.T.);
#25510=EDGE_CURVE('',#20709,#19595,#10648,.T.);
#25511=EDGE_CURVE('',#20701,#19584,#10649,.T.);
#25512=EDGE_CURVE('',#20702,#19585,#10650,.T.);
#25513=EDGE_CURVE('',#20700,#19586,#10651,.T.);
#25514=EDGE_CURVE('',#20705,#19587,#10652,.T.);
#25515=EDGE_CURVE('',#20704,#19588,#10653,.T.);
#25516=EDGE_CURVE('',#20703,#19589,#10654,.T.);
#25517=EDGE_CURVE('',#20695,#19578,#10655,.T.);
#25518=EDGE_CURVE('',#20696,#19579,#10656,.T.);
#25519=EDGE_CURVE('',#20694,#19580,#10657,.T.);
#25520=EDGE_CURVE('',#20699,#19581,#10658,.T.);
#25521=EDGE_CURVE('',#20698,#19582,#10659,.T.);
#25522=EDGE_CURVE('',#20697,#19583,#10660,.T.);
#25523=EDGE_CURVE('',#20689,#19572,#10661,.T.);
#25524=EDGE_CURVE('',#20690,#19573,#10662,.T.);
#25525=EDGE_CURVE('',#20688,#19574,#10663,.T.);
#25526=EDGE_CURVE('',#20693,#19575,#10664,.T.);
#25527=EDGE_CURVE('',#20692,#19576,#10665,.T.);
#25528=EDGE_CURVE('',#20691,#19577,#10666,.T.);
#25529=EDGE_CURVE('',#20683,#19566,#10667,.T.);
#25530=EDGE_CURVE('',#20684,#19567,#10668,.T.);
#25531=EDGE_CURVE('',#20682,#19568,#10669,.T.);
#25532=EDGE_CURVE('',#20687,#19569,#10670,.T.);
#25533=EDGE_CURVE('',#20686,#19570,#10671,.T.);
#25534=EDGE_CURVE('',#20685,#19571,#10672,.T.);
#25535=EDGE_CURVE('',#20677,#19560,#10673,.T.);
#25536=EDGE_CURVE('',#20678,#19561,#10674,.T.);
#25537=EDGE_CURVE('',#20676,#19562,#10675,.T.);
#25538=EDGE_CURVE('',#20681,#19563,#10676,.T.);
#25539=EDGE_CURVE('',#20680,#19564,#10677,.T.);
#25540=EDGE_CURVE('',#20679,#19565,#10678,.T.);
#25541=EDGE_CURVE('',#20671,#19554,#10679,.T.);
#25542=EDGE_CURVE('',#20672,#19555,#10680,.T.);
#25543=EDGE_CURVE('',#20670,#19556,#10681,.T.);
#25544=EDGE_CURVE('',#20675,#19557,#10682,.T.);
#25545=EDGE_CURVE('',#20674,#19558,#10683,.T.);
#25546=EDGE_CURVE('',#20673,#19559,#10684,.T.);
#25547=EDGE_CURVE('',#20665,#19548,#10685,.T.);
#25548=EDGE_CURVE('',#20666,#19549,#10686,.T.);
#25549=EDGE_CURVE('',#20664,#19550,#10687,.T.);
#25550=EDGE_CURVE('',#20669,#19551,#10688,.T.);
#25551=EDGE_CURVE('',#20668,#19552,#10689,.T.);
#25552=EDGE_CURVE('',#20667,#19553,#10690,.T.);
#25553=EDGE_CURVE('',#20659,#19542,#10691,.T.);
#25554=EDGE_CURVE('',#20660,#19543,#10692,.T.);
#25555=EDGE_CURVE('',#20658,#19544,#10693,.T.);
#25556=EDGE_CURVE('',#20663,#19545,#10694,.T.);
#25557=EDGE_CURVE('',#20662,#19546,#10695,.T.);
#25558=EDGE_CURVE('',#20661,#19547,#10696,.T.);
#25559=EDGE_CURVE('',#20653,#19536,#10697,.T.);
#25560=EDGE_CURVE('',#20654,#19537,#10698,.T.);
#25561=EDGE_CURVE('',#20652,#19538,#10699,.T.);
#25562=EDGE_CURVE('',#20657,#19539,#10700,.T.);
#25563=EDGE_CURVE('',#20656,#19540,#10701,.T.);
#25564=EDGE_CURVE('',#20655,#19541,#10702,.T.);
#25565=EDGE_CURVE('',#20647,#19530,#10703,.T.);
#25566=EDGE_CURVE('',#20648,#19531,#10704,.T.);
#25567=EDGE_CURVE('',#20646,#19532,#10705,.T.);
#25568=EDGE_CURVE('',#20651,#19533,#10706,.T.);
#25569=EDGE_CURVE('',#20650,#19534,#10707,.T.);
#25570=EDGE_CURVE('',#20649,#19535,#10708,.T.);
#25571=EDGE_CURVE('',#20641,#19524,#10709,.T.);
#25572=EDGE_CURVE('',#20642,#19525,#10710,.T.);
#25573=EDGE_CURVE('',#20640,#19526,#10711,.T.);
#25574=EDGE_CURVE('',#20645,#19527,#10712,.T.);
#25575=EDGE_CURVE('',#20644,#19528,#10713,.T.);
#25576=EDGE_CURVE('',#20643,#19529,#10714,.T.);
#25577=EDGE_CURVE('',#20635,#19518,#10715,.T.);
#25578=EDGE_CURVE('',#20636,#19519,#10716,.T.);
#25579=EDGE_CURVE('',#20634,#19520,#10717,.T.);
#25580=EDGE_CURVE('',#20639,#19521,#10718,.T.);
#25581=EDGE_CURVE('',#20638,#19522,#10719,.T.);
#25582=EDGE_CURVE('',#20637,#19523,#10720,.T.);
#25583=EDGE_CURVE('',#20629,#19512,#10721,.T.);
#25584=EDGE_CURVE('',#20630,#19513,#10722,.T.);
#25585=EDGE_CURVE('',#20628,#19514,#10723,.T.);
#25586=EDGE_CURVE('',#20633,#19515,#10724,.T.);
#25587=EDGE_CURVE('',#20632,#19516,#10725,.T.);
#25588=EDGE_CURVE('',#20631,#19517,#10726,.T.);
#25589=EDGE_CURVE('',#20623,#19506,#10727,.T.);
#25590=EDGE_CURVE('',#20624,#19507,#10728,.T.);
#25591=EDGE_CURVE('',#20622,#19508,#10729,.T.);
#25592=EDGE_CURVE('',#20627,#19509,#10730,.T.);
#25593=EDGE_CURVE('',#20626,#19510,#10731,.T.);
#25594=EDGE_CURVE('',#20625,#19511,#10732,.T.);
#25595=EDGE_CURVE('',#20617,#19500,#10733,.T.);
#25596=EDGE_CURVE('',#20618,#19501,#10734,.T.);
#25597=EDGE_CURVE('',#20616,#19502,#10735,.T.);
#25598=EDGE_CURVE('',#20621,#19503,#10736,.T.);
#25599=EDGE_CURVE('',#20620,#19504,#10737,.T.);
#25600=EDGE_CURVE('',#20619,#19505,#10738,.T.);
#25601=EDGE_CURVE('',#20611,#19494,#10739,.T.);
#25602=EDGE_CURVE('',#20612,#19495,#10740,.T.);
#25603=EDGE_CURVE('',#20610,#19496,#10741,.T.);
#25604=EDGE_CURVE('',#20615,#19497,#10742,.T.);
#25605=EDGE_CURVE('',#20614,#19498,#10743,.T.);
#25606=EDGE_CURVE('',#20613,#19499,#10744,.T.);
#25607=EDGE_CURVE('',#20605,#19488,#10745,.T.);
#25608=EDGE_CURVE('',#20606,#19489,#10746,.T.);
#25609=EDGE_CURVE('',#20604,#19490,#10747,.T.);
#25610=EDGE_CURVE('',#20609,#19491,#10748,.T.);
#25611=EDGE_CURVE('',#20608,#19492,#10749,.T.);
#25612=EDGE_CURVE('',#20607,#19493,#10750,.T.);
#25613=EDGE_CURVE('',#20599,#19482,#10751,.T.);
#25614=EDGE_CURVE('',#20600,#19483,#10752,.T.);
#25615=EDGE_CURVE('',#20598,#19484,#10753,.T.);
#25616=EDGE_CURVE('',#20603,#19485,#10754,.T.);
#25617=EDGE_CURVE('',#20602,#19486,#10755,.T.);
#25618=EDGE_CURVE('',#20601,#19487,#10756,.T.);
#25619=EDGE_CURVE('',#20593,#19476,#10757,.T.);
#25620=EDGE_CURVE('',#20594,#19477,#10758,.T.);
#25621=EDGE_CURVE('',#20592,#19478,#10759,.T.);
#25622=EDGE_CURVE('',#20597,#19479,#10760,.T.);
#25623=EDGE_CURVE('',#20596,#19480,#10761,.T.);
#25624=EDGE_CURVE('',#20595,#19481,#10762,.T.);
#25625=EDGE_CURVE('',#20587,#19470,#10763,.T.);
#25626=EDGE_CURVE('',#20588,#19471,#10764,.T.);
#25627=EDGE_CURVE('',#20586,#19472,#10765,.T.);
#25628=EDGE_CURVE('',#20591,#19473,#10766,.T.);
#25629=EDGE_CURVE('',#20590,#19474,#10767,.T.);
#25630=EDGE_CURVE('',#20589,#19475,#10768,.T.);
#25631=EDGE_CURVE('',#20581,#19464,#10769,.T.);
#25632=EDGE_CURVE('',#20582,#19465,#10770,.T.);
#25633=EDGE_CURVE('',#20580,#19466,#10771,.T.);
#25634=EDGE_CURVE('',#20585,#19467,#10772,.T.);
#25635=EDGE_CURVE('',#20584,#19468,#10773,.T.);
#25636=EDGE_CURVE('',#20583,#19469,#10774,.T.);
#25637=EDGE_CURVE('',#20575,#19458,#10775,.T.);
#25638=EDGE_CURVE('',#20576,#19459,#10776,.T.);
#25639=EDGE_CURVE('',#20574,#19460,#10777,.T.);
#25640=EDGE_CURVE('',#20579,#19461,#10778,.T.);
#25641=EDGE_CURVE('',#20578,#19462,#10779,.T.);
#25642=EDGE_CURVE('',#20577,#19463,#10780,.T.);
#25643=EDGE_CURVE('',#20569,#19452,#10781,.T.);
#25644=EDGE_CURVE('',#20570,#19453,#10782,.T.);
#25645=EDGE_CURVE('',#20568,#19454,#10783,.T.);
#25646=EDGE_CURVE('',#20573,#19455,#10784,.T.);
#25647=EDGE_CURVE('',#20572,#19456,#10785,.T.);
#25648=EDGE_CURVE('',#20571,#19457,#10786,.T.);
#25649=EDGE_CURVE('',#20563,#19446,#10787,.T.);
#25650=EDGE_CURVE('',#20564,#19447,#10788,.T.);
#25651=EDGE_CURVE('',#20562,#19448,#10789,.T.);
#25652=EDGE_CURVE('',#20567,#19449,#10790,.T.);
#25653=EDGE_CURVE('',#20566,#19450,#10791,.T.);
#25654=EDGE_CURVE('',#20565,#19451,#10792,.T.);
#25655=EDGE_CURVE('',#20557,#19440,#10793,.T.);
#25656=EDGE_CURVE('',#20558,#19441,#10794,.T.);
#25657=EDGE_CURVE('',#20556,#19442,#10795,.T.);
#25658=EDGE_CURVE('',#20561,#19443,#10796,.T.);
#25659=EDGE_CURVE('',#20560,#19444,#10797,.T.);
#25660=EDGE_CURVE('',#20559,#19445,#10798,.T.);
#25661=EDGE_CURVE('',#20551,#19434,#10799,.T.);
#25662=EDGE_CURVE('',#20552,#19435,#10800,.T.);
#25663=EDGE_CURVE('',#20550,#19436,#10801,.T.);
#25664=EDGE_CURVE('',#20555,#19437,#10802,.T.);
#25665=EDGE_CURVE('',#20554,#19438,#10803,.T.);
#25666=EDGE_CURVE('',#20553,#19439,#10804,.T.);
#25667=EDGE_CURVE('',#20545,#19428,#10805,.T.);
#25668=EDGE_CURVE('',#20546,#19429,#10806,.T.);
#25669=EDGE_CURVE('',#20544,#19430,#10807,.T.);
#25670=EDGE_CURVE('',#20549,#19431,#10808,.T.);
#25671=EDGE_CURVE('',#20548,#19432,#10809,.T.);
#25672=EDGE_CURVE('',#20547,#19433,#10810,.T.);
#25673=EDGE_CURVE('',#20539,#19422,#10811,.T.);
#25674=EDGE_CURVE('',#20540,#19423,#10812,.T.);
#25675=EDGE_CURVE('',#20538,#19424,#10813,.T.);
#25676=EDGE_CURVE('',#20543,#19425,#10814,.T.);
#25677=EDGE_CURVE('',#20542,#19426,#10815,.T.);
#25678=EDGE_CURVE('',#20541,#19427,#10816,.T.);
#25679=EDGE_CURVE('',#20533,#19416,#10817,.T.);
#25680=EDGE_CURVE('',#20534,#19417,#10818,.T.);
#25681=EDGE_CURVE('',#20532,#19418,#10819,.T.);
#25682=EDGE_CURVE('',#20537,#19419,#10820,.T.);
#25683=EDGE_CURVE('',#20536,#19420,#10821,.T.);
#25684=EDGE_CURVE('',#20535,#19421,#10822,.T.);
#25685=EDGE_CURVE('',#20527,#19410,#10823,.T.);
#25686=EDGE_CURVE('',#20528,#19411,#10824,.T.);
#25687=EDGE_CURVE('',#20526,#19412,#10825,.T.);
#25688=EDGE_CURVE('',#20531,#19413,#10826,.T.);
#25689=EDGE_CURVE('',#20530,#19414,#10827,.T.);
#25690=EDGE_CURVE('',#20529,#19415,#10828,.T.);
#25691=EDGE_CURVE('',#20521,#19404,#10829,.T.);
#25692=EDGE_CURVE('',#20522,#19405,#10830,.T.);
#25693=EDGE_CURVE('',#20520,#19406,#10831,.T.);
#25694=EDGE_CURVE('',#20525,#19407,#10832,.T.);
#25695=EDGE_CURVE('',#20524,#19408,#10833,.T.);
#25696=EDGE_CURVE('',#20523,#19409,#10834,.T.);
#25697=EDGE_CURVE('',#20515,#19398,#10835,.T.);
#25698=EDGE_CURVE('',#20516,#19399,#10836,.T.);
#25699=EDGE_CURVE('',#20514,#19400,#10837,.T.);
#25700=EDGE_CURVE('',#20519,#19401,#10838,.T.);
#25701=EDGE_CURVE('',#20518,#19402,#10839,.T.);
#25702=EDGE_CURVE('',#20517,#19403,#10840,.T.);
#25703=EDGE_CURVE('',#20509,#19392,#10841,.T.);
#25704=EDGE_CURVE('',#20510,#19393,#10842,.T.);
#25705=EDGE_CURVE('',#20508,#19394,#10843,.T.);
#25706=EDGE_CURVE('',#20513,#19395,#10844,.T.);
#25707=EDGE_CURVE('',#20512,#19396,#10845,.T.);
#25708=EDGE_CURVE('',#20511,#19397,#10846,.T.);
#25709=EDGE_CURVE('',#20503,#19386,#10847,.T.);
#25710=EDGE_CURVE('',#20504,#19387,#10848,.T.);
#25711=EDGE_CURVE('',#20502,#19388,#10849,.T.);
#25712=EDGE_CURVE('',#20507,#19389,#10850,.T.);
#25713=EDGE_CURVE('',#20506,#19390,#10851,.T.);
#25714=EDGE_CURVE('',#20505,#19391,#10852,.T.);
#25715=EDGE_CURVE('',#20497,#19380,#10853,.T.);
#25716=EDGE_CURVE('',#20498,#19381,#10854,.T.);
#25717=EDGE_CURVE('',#20496,#19382,#10855,.T.);
#25718=EDGE_CURVE('',#20501,#19383,#10856,.T.);
#25719=EDGE_CURVE('',#20500,#19384,#10857,.T.);
#25720=EDGE_CURVE('',#20499,#19385,#10858,.T.);
#25721=EDGE_CURVE('',#20491,#19374,#10859,.T.);
#25722=EDGE_CURVE('',#20492,#19375,#10860,.T.);
#25723=EDGE_CURVE('',#20490,#19376,#10861,.T.);
#25724=EDGE_CURVE('',#20495,#19377,#10862,.T.);
#25725=EDGE_CURVE('',#20494,#19378,#10863,.T.);
#25726=EDGE_CURVE('',#20493,#19379,#10864,.T.);
#25727=EDGE_CURVE('',#20485,#19368,#10865,.T.);
#25728=EDGE_CURVE('',#20486,#19369,#10866,.T.);
#25729=EDGE_CURVE('',#20484,#19370,#10867,.T.);
#25730=EDGE_CURVE('',#20489,#19371,#10868,.T.);
#25731=EDGE_CURVE('',#20488,#19372,#10869,.T.);
#25732=EDGE_CURVE('',#20487,#19373,#10870,.T.);
#25733=EDGE_CURVE('',#20479,#19362,#10871,.T.);
#25734=EDGE_CURVE('',#20480,#19363,#10872,.T.);
#25735=EDGE_CURVE('',#20478,#19364,#10873,.T.);
#25736=EDGE_CURVE('',#20483,#19365,#10874,.T.);
#25737=EDGE_CURVE('',#20482,#19366,#10875,.T.);
#25738=EDGE_CURVE('',#20481,#19367,#10876,.T.);
#25739=EDGE_CURVE('',#20473,#19356,#10877,.T.);
#25740=EDGE_CURVE('',#20474,#19357,#10878,.T.);
#25741=EDGE_CURVE('',#20472,#19358,#10879,.T.);
#25742=EDGE_CURVE('',#20477,#19359,#10880,.T.);
#25743=EDGE_CURVE('',#20476,#19360,#10881,.T.);
#25744=EDGE_CURVE('',#20475,#19361,#10882,.T.);
#25745=EDGE_CURVE('',#20467,#19350,#10883,.T.);
#25746=EDGE_CURVE('',#20468,#19351,#10884,.T.);
#25747=EDGE_CURVE('',#20466,#19352,#10885,.T.);
#25748=EDGE_CURVE('',#20471,#19353,#10886,.T.);
#25749=EDGE_CURVE('',#20470,#19354,#10887,.T.);
#25750=EDGE_CURVE('',#20469,#19355,#10888,.T.);
#25751=EDGE_CURVE('',#20461,#19344,#10889,.T.);
#25752=EDGE_CURVE('',#20462,#19345,#10890,.T.);
#25753=EDGE_CURVE('',#20460,#19346,#10891,.T.);
#25754=EDGE_CURVE('',#20465,#19347,#10892,.T.);
#25755=EDGE_CURVE('',#20464,#19348,#10893,.T.);
#25756=EDGE_CURVE('',#20463,#19349,#10894,.T.);
#25757=EDGE_CURVE('',#20455,#19338,#10895,.T.);
#25758=EDGE_CURVE('',#20456,#19339,#10896,.T.);
#25759=EDGE_CURVE('',#20454,#19340,#10897,.T.);
#25760=EDGE_CURVE('',#20459,#19341,#10898,.T.);
#25761=EDGE_CURVE('',#20458,#19342,#10899,.T.);
#25762=EDGE_CURVE('',#20457,#19343,#10900,.T.);
#25763=EDGE_CURVE('',#20449,#19332,#10901,.T.);
#25764=EDGE_CURVE('',#20450,#19333,#10902,.T.);
#25765=EDGE_CURVE('',#20448,#19334,#10903,.T.);
#25766=EDGE_CURVE('',#20453,#19335,#10904,.T.);
#25767=EDGE_CURVE('',#20452,#19336,#10905,.T.);
#25768=EDGE_CURVE('',#20451,#19337,#10906,.T.);
#25769=EDGE_CURVE('',#20443,#19326,#10907,.T.);
#25770=EDGE_CURVE('',#20444,#19327,#10908,.T.);
#25771=EDGE_CURVE('',#20442,#19328,#10909,.T.);
#25772=EDGE_CURVE('',#20447,#19329,#10910,.T.);
#25773=EDGE_CURVE('',#20446,#19330,#10911,.T.);
#25774=EDGE_CURVE('',#20445,#19331,#10912,.T.);
#25775=EDGE_CURVE('',#20437,#19320,#10913,.T.);
#25776=EDGE_CURVE('',#20438,#19321,#10914,.T.);
#25777=EDGE_CURVE('',#20436,#19322,#10915,.T.);
#25778=EDGE_CURVE('',#20441,#19323,#10916,.T.);
#25779=EDGE_CURVE('',#20440,#19324,#10917,.T.);
#25780=EDGE_CURVE('',#20439,#19325,#10918,.T.);
#25781=EDGE_CURVE('',#20431,#19314,#10919,.T.);
#25782=EDGE_CURVE('',#20432,#19315,#10920,.T.);
#25783=EDGE_CURVE('',#20430,#19316,#10921,.T.);
#25784=EDGE_CURVE('',#20435,#19317,#10922,.T.);
#25785=EDGE_CURVE('',#20434,#19318,#10923,.T.);
#25786=EDGE_CURVE('',#20433,#19319,#10924,.T.);
#25787=EDGE_CURVE('',#20425,#19308,#10925,.T.);
#25788=EDGE_CURVE('',#20426,#19309,#10926,.T.);
#25789=EDGE_CURVE('',#20424,#19310,#10927,.T.);
#25790=EDGE_CURVE('',#20429,#19311,#10928,.T.);
#25791=EDGE_CURVE('',#20428,#19312,#10929,.T.);
#25792=EDGE_CURVE('',#20427,#19313,#10930,.T.);
#25793=EDGE_CURVE('',#20419,#19302,#10931,.T.);
#25794=EDGE_CURVE('',#20420,#19303,#10932,.T.);
#25795=EDGE_CURVE('',#20418,#19304,#10933,.T.);
#25796=EDGE_CURVE('',#20423,#19305,#10934,.T.);
#25797=EDGE_CURVE('',#20422,#19306,#10935,.T.);
#25798=EDGE_CURVE('',#20421,#19307,#10936,.T.);
#25799=EDGE_CURVE('',#20413,#19296,#10937,.T.);
#25800=EDGE_CURVE('',#20414,#19297,#10938,.T.);
#25801=EDGE_CURVE('',#20412,#19298,#10939,.T.);
#25802=EDGE_CURVE('',#20417,#19299,#10940,.T.);
#25803=EDGE_CURVE('',#20416,#19300,#10941,.T.);
#25804=EDGE_CURVE('',#20415,#19301,#10942,.T.);
#25805=EDGE_CURVE('',#20407,#19290,#10943,.T.);
#25806=EDGE_CURVE('',#20408,#19291,#10944,.T.);
#25807=EDGE_CURVE('',#20406,#19292,#10945,.T.);
#25808=EDGE_CURVE('',#20411,#19293,#10946,.T.);
#25809=EDGE_CURVE('',#20410,#19294,#10947,.T.);
#25810=EDGE_CURVE('',#20409,#19295,#10948,.T.);
#25811=EDGE_CURVE('',#20401,#19284,#10949,.T.);
#25812=EDGE_CURVE('',#20402,#19285,#10950,.T.);
#25813=EDGE_CURVE('',#20400,#19286,#10951,.T.);
#25814=EDGE_CURVE('',#20405,#19287,#10952,.T.);
#25815=EDGE_CURVE('',#20404,#19288,#10953,.T.);
#25816=EDGE_CURVE('',#20403,#19289,#10954,.T.);
#25817=EDGE_CURVE('',#20395,#19278,#10955,.T.);
#25818=EDGE_CURVE('',#20396,#19279,#10956,.T.);
#25819=EDGE_CURVE('',#20394,#19280,#10957,.T.);
#25820=EDGE_CURVE('',#20399,#19281,#10958,.T.);
#25821=EDGE_CURVE('',#20398,#19282,#10959,.T.);
#25822=EDGE_CURVE('',#20397,#19283,#10960,.T.);
#25823=EDGE_CURVE('',#20389,#19272,#10961,.T.);
#25824=EDGE_CURVE('',#20390,#19273,#10962,.T.);
#25825=EDGE_CURVE('',#20388,#19274,#10963,.T.);
#25826=EDGE_CURVE('',#20393,#19275,#10964,.T.);
#25827=EDGE_CURVE('',#20392,#19276,#10965,.T.);
#25828=EDGE_CURVE('',#20391,#19277,#10966,.T.);
#25829=EDGE_CURVE('',#20383,#19266,#10967,.T.);
#25830=EDGE_CURVE('',#20384,#19267,#10968,.T.);
#25831=EDGE_CURVE('',#20382,#19268,#10969,.T.);
#25832=EDGE_CURVE('',#20387,#19269,#10970,.T.);
#25833=EDGE_CURVE('',#20386,#19270,#10971,.T.);
#25834=EDGE_CURVE('',#20385,#19271,#10972,.T.);
#25835=EDGE_CURVE('',#20377,#19260,#10973,.T.);
#25836=EDGE_CURVE('',#20378,#19261,#10974,.T.);
#25837=EDGE_CURVE('',#20376,#19262,#10975,.T.);
#25838=EDGE_CURVE('',#20381,#19263,#10976,.T.);
#25839=EDGE_CURVE('',#20380,#19264,#10977,.T.);
#25840=EDGE_CURVE('',#20379,#19265,#10978,.T.);
#25841=EDGE_CURVE('',#20371,#19254,#10979,.T.);
#25842=EDGE_CURVE('',#20372,#19255,#10980,.T.);
#25843=EDGE_CURVE('',#20370,#19256,#10981,.T.);
#25844=EDGE_CURVE('',#20375,#19257,#10982,.T.);
#25845=EDGE_CURVE('',#20374,#19258,#10983,.T.);
#25846=EDGE_CURVE('',#20373,#19259,#10984,.T.);
#25847=EDGE_CURVE('',#20365,#19248,#10985,.T.);
#25848=EDGE_CURVE('',#20366,#19249,#10986,.T.);
#25849=EDGE_CURVE('',#20364,#19250,#10987,.T.);
#25850=EDGE_CURVE('',#20369,#19251,#10988,.T.);
#25851=EDGE_CURVE('',#20368,#19252,#10989,.T.);
#25852=EDGE_CURVE('',#20367,#19253,#10990,.T.);
#25853=EDGE_CURVE('',#20359,#19242,#10991,.T.);
#25854=EDGE_CURVE('',#20360,#19243,#10992,.T.);
#25855=EDGE_CURVE('',#20358,#19244,#10993,.T.);
#25856=EDGE_CURVE('',#20363,#19245,#10994,.T.);
#25857=EDGE_CURVE('',#20362,#19246,#10995,.T.);
#25858=EDGE_CURVE('',#20361,#19247,#10996,.T.);
#25859=EDGE_CURVE('',#20353,#19236,#10997,.T.);
#25860=EDGE_CURVE('',#20354,#19237,#10998,.T.);
#25861=EDGE_CURVE('',#20352,#19238,#10999,.T.);
#25862=EDGE_CURVE('',#20357,#19239,#11000,.T.);
#25863=EDGE_CURVE('',#20356,#19240,#11001,.T.);
#25864=EDGE_CURVE('',#20355,#19241,#11002,.T.);
#25865=EDGE_CURVE('',#20347,#19230,#11003,.T.);
#25866=EDGE_CURVE('',#20348,#19231,#11004,.T.);
#25867=EDGE_CURVE('',#20346,#19232,#11005,.T.);
#25868=EDGE_CURVE('',#20351,#19233,#11006,.T.);
#25869=EDGE_CURVE('',#20350,#19234,#11007,.T.);
#25870=EDGE_CURVE('',#20349,#19235,#11008,.T.);
#25871=EDGE_CURVE('',#20341,#19224,#11009,.T.);
#25872=EDGE_CURVE('',#20342,#19225,#11010,.T.);
#25873=EDGE_CURVE('',#20340,#19226,#11011,.T.);
#25874=EDGE_CURVE('',#20345,#19227,#11012,.T.);
#25875=EDGE_CURVE('',#20344,#19228,#11013,.T.);
#25876=EDGE_CURVE('',#20343,#19229,#11014,.T.);
#25877=EDGE_CURVE('',#20335,#19218,#11015,.T.);
#25878=EDGE_CURVE('',#20336,#19219,#11016,.T.);
#25879=EDGE_CURVE('',#20334,#19220,#11017,.T.);
#25880=EDGE_CURVE('',#20339,#19221,#11018,.T.);
#25881=EDGE_CURVE('',#20338,#19222,#11019,.T.);
#25882=EDGE_CURVE('',#20337,#19223,#11020,.T.);
#25883=EDGE_CURVE('',#20329,#19212,#11021,.T.);
#25884=EDGE_CURVE('',#20330,#19213,#11022,.T.);
#25885=EDGE_CURVE('',#20328,#19214,#11023,.T.);
#25886=EDGE_CURVE('',#20333,#19215,#11024,.T.);
#25887=EDGE_CURVE('',#20332,#19216,#11025,.T.);
#25888=EDGE_CURVE('',#20331,#19217,#11026,.T.);
#25889=EDGE_CURVE('',#20323,#19206,#11027,.T.);
#25890=EDGE_CURVE('',#20324,#19207,#11028,.T.);
#25891=EDGE_CURVE('',#20322,#19208,#11029,.T.);
#25892=EDGE_CURVE('',#20327,#19209,#11030,.T.);
#25893=EDGE_CURVE('',#20326,#19210,#11031,.T.);
#25894=EDGE_CURVE('',#20325,#19211,#11032,.T.);
#25895=EDGE_CURVE('',#20317,#19200,#11033,.T.);
#25896=EDGE_CURVE('',#20318,#19201,#11034,.T.);
#25897=EDGE_CURVE('',#20316,#19202,#11035,.T.);
#25898=EDGE_CURVE('',#20321,#19203,#11036,.T.);
#25899=EDGE_CURVE('',#20320,#19204,#11037,.T.);
#25900=EDGE_CURVE('',#20319,#19205,#11038,.T.);
#25901=EDGE_CURVE('',#20311,#19194,#11039,.T.);
#25902=EDGE_CURVE('',#20312,#19195,#11040,.T.);
#25903=EDGE_CURVE('',#20310,#19196,#11041,.T.);
#25904=EDGE_CURVE('',#20315,#19197,#11042,.T.);
#25905=EDGE_CURVE('',#20314,#19198,#11043,.T.);
#25906=EDGE_CURVE('',#20313,#19199,#11044,.T.);
#25907=EDGE_CURVE('',#20305,#19188,#11045,.T.);
#25908=EDGE_CURVE('',#20306,#19189,#11046,.T.);
#25909=EDGE_CURVE('',#20304,#19190,#11047,.T.);
#25910=EDGE_CURVE('',#20309,#19191,#11048,.T.);
#25911=EDGE_CURVE('',#20308,#19192,#11049,.T.);
#25912=EDGE_CURVE('',#20307,#19193,#11050,.T.);
#25913=EDGE_CURVE('',#20299,#19182,#11051,.T.);
#25914=EDGE_CURVE('',#20300,#19183,#11052,.T.);
#25915=EDGE_CURVE('',#20298,#19184,#11053,.T.);
#25916=EDGE_CURVE('',#20303,#19185,#11054,.T.);
#25917=EDGE_CURVE('',#20302,#19186,#11055,.T.);
#25918=EDGE_CURVE('',#20301,#19187,#11056,.T.);
#25919=EDGE_CURVE('',#20293,#19176,#11057,.T.);
#25920=EDGE_CURVE('',#20294,#19177,#11058,.T.);
#25921=EDGE_CURVE('',#20292,#19178,#11059,.T.);
#25922=EDGE_CURVE('',#20297,#19179,#11060,.T.);
#25923=EDGE_CURVE('',#20296,#19180,#11061,.T.);
#25924=EDGE_CURVE('',#20295,#19181,#11062,.T.);
#25925=EDGE_CURVE('',#20287,#19170,#11063,.T.);
#25926=EDGE_CURVE('',#20288,#19171,#11064,.T.);
#25927=EDGE_CURVE('',#20286,#19172,#11065,.T.);
#25928=EDGE_CURVE('',#20291,#19173,#11066,.T.);
#25929=EDGE_CURVE('',#20290,#19174,#11067,.T.);
#25930=EDGE_CURVE('',#20289,#19175,#11068,.T.);
#25931=EDGE_CURVE('',#20281,#19164,#11069,.T.);
#25932=EDGE_CURVE('',#20282,#19165,#11070,.T.);
#25933=EDGE_CURVE('',#20280,#19166,#11071,.T.);
#25934=EDGE_CURVE('',#20285,#19167,#11072,.T.);
#25935=EDGE_CURVE('',#20284,#19168,#11073,.T.);
#25936=EDGE_CURVE('',#20283,#19169,#11074,.T.);
#25937=EDGE_CURVE('',#20275,#19158,#11075,.T.);
#25938=EDGE_CURVE('',#20276,#19159,#11076,.T.);
#25939=EDGE_CURVE('',#20274,#19160,#11077,.T.);
#25940=EDGE_CURVE('',#20279,#19161,#11078,.T.);
#25941=EDGE_CURVE('',#20278,#19162,#11079,.T.);
#25942=EDGE_CURVE('',#20277,#19163,#11080,.T.);
#25943=EDGE_CURVE('',#20269,#19152,#11081,.T.);
#25944=EDGE_CURVE('',#20270,#19153,#11082,.T.);
#25945=EDGE_CURVE('',#20268,#19154,#11083,.T.);
#25946=EDGE_CURVE('',#20273,#19155,#11084,.T.);
#25947=EDGE_CURVE('',#20272,#19156,#11085,.T.);
#25948=EDGE_CURVE('',#20271,#19157,#11086,.T.);
#25949=EDGE_CURVE('',#20263,#19146,#11087,.T.);
#25950=EDGE_CURVE('',#20264,#19147,#11088,.T.);
#25951=EDGE_CURVE('',#20262,#19148,#11089,.T.);
#25952=EDGE_CURVE('',#20267,#19149,#11090,.T.);
#25953=EDGE_CURVE('',#20266,#19150,#11091,.T.);
#25954=EDGE_CURVE('',#20265,#19151,#11092,.T.);
#25955=EDGE_CURVE('',#20257,#19140,#11093,.T.);
#25956=EDGE_CURVE('',#20258,#19141,#11094,.T.);
#25957=EDGE_CURVE('',#20256,#19142,#11095,.T.);
#25958=EDGE_CURVE('',#20261,#19143,#11096,.T.);
#25959=EDGE_CURVE('',#20260,#19144,#11097,.T.);
#25960=EDGE_CURVE('',#20259,#19145,#11098,.T.);
#25961=EDGE_CURVE('',#20251,#19134,#11099,.T.);
#25962=EDGE_CURVE('',#20252,#19135,#11100,.T.);
#25963=EDGE_CURVE('',#20250,#19136,#11101,.T.);
#25964=EDGE_CURVE('',#20255,#19137,#11102,.T.);
#25965=EDGE_CURVE('',#20254,#19138,#11103,.T.);
#25966=EDGE_CURVE('',#20253,#19139,#11104,.T.);
#25967=EDGE_CURVE('',#20245,#19128,#11105,.T.);
#25968=EDGE_CURVE('',#20246,#19129,#11106,.T.);
#25969=EDGE_CURVE('',#20244,#19130,#11107,.T.);
#25970=EDGE_CURVE('',#20249,#19131,#11108,.T.);
#25971=EDGE_CURVE('',#20248,#19132,#11109,.T.);
#25972=EDGE_CURVE('',#20247,#19133,#11110,.T.);
#25973=EDGE_CURVE('',#20239,#19122,#11111,.T.);
#25974=EDGE_CURVE('',#20240,#19123,#11112,.T.);
#25975=EDGE_CURVE('',#20238,#19124,#11113,.T.);
#25976=EDGE_CURVE('',#20243,#19125,#11114,.T.);
#25977=EDGE_CURVE('',#20242,#19126,#11115,.T.);
#25978=EDGE_CURVE('',#20241,#19127,#11116,.T.);
#25979=EDGE_CURVE('',#20233,#19116,#11117,.T.);
#25980=EDGE_CURVE('',#20234,#19117,#11118,.T.);
#25981=EDGE_CURVE('',#20232,#19118,#11119,.T.);
#25982=EDGE_CURVE('',#20237,#19119,#11120,.T.);
#25983=EDGE_CURVE('',#20236,#19120,#11121,.T.);
#25984=EDGE_CURVE('',#20235,#19121,#11122,.T.);
#25985=EDGE_CURVE('',#20227,#19110,#11123,.T.);
#25986=EDGE_CURVE('',#20228,#19111,#11124,.T.);
#25987=EDGE_CURVE('',#20226,#19112,#11125,.T.);
#25988=EDGE_CURVE('',#20231,#19113,#11126,.T.);
#25989=EDGE_CURVE('',#20230,#19114,#11127,.T.);
#25990=EDGE_CURVE('',#20229,#19115,#11128,.T.);
#25991=EDGE_CURVE('',#20221,#19104,#11129,.T.);
#25992=EDGE_CURVE('',#20222,#19105,#11130,.T.);
#25993=EDGE_CURVE('',#20220,#19106,#11131,.T.);
#25994=EDGE_CURVE('',#20225,#19107,#11132,.T.);
#25995=EDGE_CURVE('',#20224,#19108,#11133,.T.);
#25996=EDGE_CURVE('',#20223,#19109,#11134,.T.);
#25997=EDGE_CURVE('',#20215,#19098,#11135,.T.);
#25998=EDGE_CURVE('',#20216,#19099,#11136,.T.);
#25999=EDGE_CURVE('',#20214,#19100,#11137,.T.);
#26000=EDGE_CURVE('',#20219,#19101,#11138,.T.);
#26001=EDGE_CURVE('',#20218,#19102,#11139,.T.);
#26002=EDGE_CURVE('',#20217,#19103,#11140,.T.);
#26003=EDGE_CURVE('',#20209,#19092,#11141,.T.);
#26004=EDGE_CURVE('',#20210,#19093,#11142,.T.);
#26005=EDGE_CURVE('',#20208,#19094,#11143,.T.);
#26006=EDGE_CURVE('',#20213,#19095,#11144,.T.);
#26007=EDGE_CURVE('',#20212,#19096,#11145,.T.);
#26008=EDGE_CURVE('',#20211,#19097,#11146,.T.);
#26009=EDGE_CURVE('',#20203,#19086,#11147,.T.);
#26010=EDGE_CURVE('',#20204,#19087,#11148,.T.);
#26011=EDGE_CURVE('',#20202,#19088,#11149,.T.);
#26012=EDGE_CURVE('',#20207,#19089,#11150,.T.);
#26013=EDGE_CURVE('',#20206,#19090,#11151,.T.);
#26014=EDGE_CURVE('',#20205,#19091,#11152,.T.);
#26015=EDGE_CURVE('',#20197,#19080,#11153,.T.);
#26016=EDGE_CURVE('',#20198,#19081,#11154,.T.);
#26017=EDGE_CURVE('',#20196,#19082,#11155,.T.);
#26018=EDGE_CURVE('',#20201,#19083,#11156,.T.);
#26019=EDGE_CURVE('',#20200,#19084,#11157,.T.);
#26020=EDGE_CURVE('',#20199,#19085,#11158,.T.);
#26021=EDGE_CURVE('',#20191,#19074,#11159,.T.);
#26022=EDGE_CURVE('',#20192,#19075,#11160,.T.);
#26023=EDGE_CURVE('',#20190,#19076,#11161,.T.);
#26024=EDGE_CURVE('',#20195,#19077,#11162,.T.);
#26025=EDGE_CURVE('',#20194,#19078,#11163,.T.);
#26026=EDGE_CURVE('',#20193,#19079,#11164,.T.);
#26027=EDGE_CURVE('',#20185,#19068,#11165,.T.);
#26028=EDGE_CURVE('',#20186,#19069,#11166,.T.);
#26029=EDGE_CURVE('',#20184,#19070,#11167,.T.);
#26030=EDGE_CURVE('',#20189,#19071,#11168,.T.);
#26031=EDGE_CURVE('',#20188,#19072,#11169,.T.);
#26032=EDGE_CURVE('',#20187,#19073,#11170,.T.);
#26033=EDGE_CURVE('',#20179,#19062,#11171,.T.);
#26034=EDGE_CURVE('',#20180,#19063,#11172,.T.);
#26035=EDGE_CURVE('',#20178,#19064,#11173,.T.);
#26036=EDGE_CURVE('',#20183,#19065,#11174,.T.);
#26037=EDGE_CURVE('',#20182,#19066,#11175,.T.);
#26038=EDGE_CURVE('',#20181,#19067,#11176,.T.);
#26039=EDGE_CURVE('',#20173,#19056,#11177,.T.);
#26040=EDGE_CURVE('',#20174,#19057,#11178,.T.);
#26041=EDGE_CURVE('',#20172,#19058,#11179,.T.);
#26042=EDGE_CURVE('',#20177,#19059,#11180,.T.);
#26043=EDGE_CURVE('',#20176,#19060,#11181,.T.);
#26044=EDGE_CURVE('',#20175,#19061,#11182,.T.);
#26045=EDGE_CURVE('',#20167,#19050,#11183,.T.);
#26046=EDGE_CURVE('',#20168,#19051,#11184,.T.);
#26047=EDGE_CURVE('',#20166,#19052,#11185,.T.);
#26048=EDGE_CURVE('',#20171,#19053,#11186,.T.);
#26049=EDGE_CURVE('',#20170,#19054,#11187,.T.);
#26050=EDGE_CURVE('',#20169,#19055,#11188,.T.);
#26051=EDGE_CURVE('',#20161,#19044,#11189,.T.);
#26052=EDGE_CURVE('',#20162,#19045,#11190,.T.);
#26053=EDGE_CURVE('',#20160,#19046,#11191,.T.);
#26054=EDGE_CURVE('',#20165,#19047,#11192,.T.);
#26055=EDGE_CURVE('',#20164,#19048,#11193,.T.);
#26056=EDGE_CURVE('',#20163,#19049,#11194,.T.);
#26057=EDGE_CURVE('',#20155,#19038,#11195,.T.);
#26058=EDGE_CURVE('',#20156,#19039,#11196,.T.);
#26059=EDGE_CURVE('',#20154,#19040,#11197,.T.);
#26060=EDGE_CURVE('',#20159,#19041,#11198,.T.);
#26061=EDGE_CURVE('',#20158,#19042,#11199,.T.);
#26062=EDGE_CURVE('',#20157,#19043,#11200,.T.);
#26063=EDGE_CURVE('',#20149,#19032,#11201,.T.);
#26064=EDGE_CURVE('',#20150,#19033,#11202,.T.);
#26065=EDGE_CURVE('',#20148,#19034,#11203,.T.);
#26066=EDGE_CURVE('',#20153,#19035,#11204,.T.);
#26067=EDGE_CURVE('',#20152,#19036,#11205,.T.);
#26068=EDGE_CURVE('',#20151,#19037,#11206,.T.);
#26069=EDGE_CURVE('',#20143,#19026,#11207,.T.);
#26070=EDGE_CURVE('',#20144,#19027,#11208,.T.);
#26071=EDGE_CURVE('',#20142,#19028,#11209,.T.);
#26072=EDGE_CURVE('',#20147,#19029,#11210,.T.);
#26073=EDGE_CURVE('',#20146,#19030,#11211,.T.);
#26074=EDGE_CURVE('',#20145,#19031,#11212,.T.);
#26075=EDGE_CURVE('',#20137,#19020,#11213,.T.);
#26076=EDGE_CURVE('',#20138,#19021,#11214,.T.);
#26077=EDGE_CURVE('',#20136,#19022,#11215,.T.);
#26078=EDGE_CURVE('',#20141,#19023,#11216,.T.);
#26079=EDGE_CURVE('',#20140,#19024,#11217,.T.);
#26080=EDGE_CURVE('',#20139,#19025,#11218,.T.);
#26081=EDGE_CURVE('',#20131,#19014,#11219,.T.);
#26082=EDGE_CURVE('',#20132,#19015,#11220,.T.);
#26083=EDGE_CURVE('',#20130,#19016,#11221,.T.);
#26084=EDGE_CURVE('',#20135,#19017,#11222,.T.);
#26085=EDGE_CURVE('',#20134,#19018,#11223,.T.);
#26086=EDGE_CURVE('',#20133,#19019,#11224,.T.);
#26087=EDGE_CURVE('',#20125,#19008,#11225,.T.);
#26088=EDGE_CURVE('',#20126,#19009,#11226,.T.);
#26089=EDGE_CURVE('',#20124,#19010,#11227,.T.);
#26090=EDGE_CURVE('',#20129,#19011,#11228,.T.);
#26091=EDGE_CURVE('',#20128,#19012,#11229,.T.);
#26092=EDGE_CURVE('',#20127,#19013,#11230,.T.);
#26093=EDGE_CURVE('',#20119,#19002,#11231,.T.);
#26094=EDGE_CURVE('',#20120,#19003,#11232,.T.);
#26095=EDGE_CURVE('',#20118,#19004,#11233,.T.);
#26096=EDGE_CURVE('',#20123,#19005,#11234,.T.);
#26097=EDGE_CURVE('',#20122,#19006,#11235,.T.);
#26098=EDGE_CURVE('',#20121,#19007,#11236,.T.);
#26099=EDGE_CURVE('',#20113,#18996,#11237,.T.);
#26100=EDGE_CURVE('',#20114,#18997,#11238,.T.);
#26101=EDGE_CURVE('',#20112,#18998,#11239,.T.);
#26102=EDGE_CURVE('',#20117,#18999,#11240,.T.);
#26103=EDGE_CURVE('',#20116,#19000,#11241,.T.);
#26104=EDGE_CURVE('',#20115,#19001,#11242,.T.);
#26105=EDGE_CURVE('',#20107,#18990,#11243,.T.);
#26106=EDGE_CURVE('',#20108,#18991,#11244,.T.);
#26107=EDGE_CURVE('',#20106,#18992,#11245,.T.);
#26108=EDGE_CURVE('',#20111,#18993,#11246,.T.);
#26109=EDGE_CURVE('',#20110,#18994,#11247,.T.);
#26110=EDGE_CURVE('',#20109,#18995,#11248,.T.);
#26111=EDGE_CURVE('',#20101,#18984,#11249,.T.);
#26112=EDGE_CURVE('',#20102,#18985,#11250,.T.);
#26113=EDGE_CURVE('',#20100,#18986,#11251,.T.);
#26114=EDGE_CURVE('',#20105,#18987,#11252,.T.);
#26115=EDGE_CURVE('',#20104,#18988,#11253,.T.);
#26116=EDGE_CURVE('',#20103,#18989,#11254,.T.);
#26117=EDGE_CURVE('',#20095,#18978,#11255,.T.);
#26118=EDGE_CURVE('',#20096,#18979,#11256,.T.);
#26119=EDGE_CURVE('',#20094,#18980,#11257,.T.);
#26120=EDGE_CURVE('',#20099,#18981,#11258,.T.);
#26121=EDGE_CURVE('',#20098,#18982,#11259,.T.);
#26122=EDGE_CURVE('',#20097,#18983,#11260,.T.);
#26123=EDGE_CURVE('',#20089,#18972,#11261,.T.);
#26124=EDGE_CURVE('',#20090,#18973,#11262,.T.);
#26125=EDGE_CURVE('',#20088,#18974,#11263,.T.);
#26126=EDGE_CURVE('',#20093,#18975,#11264,.T.);
#26127=EDGE_CURVE('',#20092,#18976,#11265,.T.);
#26128=EDGE_CURVE('',#20091,#18977,#11266,.T.);
#26129=EDGE_CURVE('',#20083,#18966,#11267,.T.);
#26130=EDGE_CURVE('',#20084,#18967,#11268,.T.);
#26131=EDGE_CURVE('',#20082,#18968,#11269,.T.);
#26132=EDGE_CURVE('',#20087,#18969,#11270,.T.);
#26133=EDGE_CURVE('',#20086,#18970,#11271,.T.);
#26134=EDGE_CURVE('',#20085,#18971,#11272,.T.);
#26135=EDGE_CURVE('',#20077,#18960,#11273,.T.);
#26136=EDGE_CURVE('',#20078,#18961,#11274,.T.);
#26137=EDGE_CURVE('',#20076,#18962,#11275,.T.);
#26138=EDGE_CURVE('',#20081,#18963,#11276,.T.);
#26139=EDGE_CURVE('',#20080,#18964,#11277,.T.);
#26140=EDGE_CURVE('',#20079,#18965,#11278,.T.);
#26141=EDGE_CURVE('',#20071,#18954,#11279,.T.);
#26142=EDGE_CURVE('',#20072,#18955,#11280,.T.);
#26143=EDGE_CURVE('',#20070,#18956,#11281,.T.);
#26144=EDGE_CURVE('',#20075,#18957,#11282,.T.);
#26145=EDGE_CURVE('',#20074,#18958,#11283,.T.);
#26146=EDGE_CURVE('',#20073,#18959,#11284,.T.);
#26147=EDGE_CURVE('',#20065,#18948,#11285,.T.);
#26148=EDGE_CURVE('',#20066,#18949,#11286,.T.);
#26149=EDGE_CURVE('',#20064,#18950,#11287,.T.);
#26150=EDGE_CURVE('',#20069,#18951,#11288,.T.);
#26151=EDGE_CURVE('',#20068,#18952,#11289,.T.);
#26152=EDGE_CURVE('',#20067,#18953,#11290,.T.);
#26153=EDGE_CURVE('',#20059,#18942,#11291,.T.);
#26154=EDGE_CURVE('',#20060,#18943,#11292,.T.);
#26155=EDGE_CURVE('',#20058,#18944,#11293,.T.);
#26156=EDGE_CURVE('',#20063,#18945,#11294,.T.);
#26157=EDGE_CURVE('',#20062,#18946,#11295,.T.);
#26158=EDGE_CURVE('',#20061,#18947,#11296,.T.);
#26159=EDGE_CURVE('',#20053,#18936,#11297,.T.);
#26160=EDGE_CURVE('',#20054,#18937,#11298,.T.);
#26161=EDGE_CURVE('',#20052,#18938,#11299,.T.);
#26162=EDGE_CURVE('',#20057,#18939,#11300,.T.);
#26163=EDGE_CURVE('',#20056,#18940,#11301,.T.);
#26164=EDGE_CURVE('',#20055,#18941,#11302,.T.);
#26165=EDGE_CURVE('',#20047,#18930,#11303,.T.);
#26166=EDGE_CURVE('',#20048,#18931,#11304,.T.);
#26167=EDGE_CURVE('',#20046,#18932,#11305,.T.);
#26168=EDGE_CURVE('',#20051,#18933,#11306,.T.);
#26169=EDGE_CURVE('',#20050,#18934,#11307,.T.);
#26170=EDGE_CURVE('',#20049,#18935,#11308,.T.);
#26171=EDGE_CURVE('',#20041,#18924,#11309,.T.);
#26172=EDGE_CURVE('',#20042,#18925,#11310,.T.);
#26173=EDGE_CURVE('',#20040,#18926,#11311,.T.);
#26174=EDGE_CURVE('',#20045,#18927,#11312,.T.);
#26175=EDGE_CURVE('',#20044,#18928,#11313,.T.);
#26176=EDGE_CURVE('',#20043,#18929,#11314,.T.);
#26177=EDGE_CURVE('',#20035,#18918,#11315,.T.);
#26178=EDGE_CURVE('',#20036,#18919,#11316,.T.);
#26179=EDGE_CURVE('',#20034,#18920,#11317,.T.);
#26180=EDGE_CURVE('',#20039,#18921,#11318,.T.);
#26181=EDGE_CURVE('',#20038,#18922,#11319,.T.);
#26182=EDGE_CURVE('',#20037,#18923,#11320,.T.);
#26183=EDGE_CURVE('',#20029,#18912,#11321,.T.);
#26184=EDGE_CURVE('',#20030,#18913,#11322,.T.);
#26185=EDGE_CURVE('',#20028,#18914,#11323,.T.);
#26186=EDGE_CURVE('',#20033,#18915,#11324,.T.);
#26187=EDGE_CURVE('',#20032,#18916,#11325,.T.);
#26188=EDGE_CURVE('',#20031,#18917,#11326,.T.);
#26189=EDGE_CURVE('',#20023,#18906,#11327,.T.);
#26190=EDGE_CURVE('',#20024,#18907,#11328,.T.);
#26191=EDGE_CURVE('',#20022,#18908,#11329,.T.);
#26192=EDGE_CURVE('',#20027,#18909,#11330,.T.);
#26193=EDGE_CURVE('',#20026,#18910,#11331,.T.);
#26194=EDGE_CURVE('',#20025,#18911,#11332,.T.);
#26195=EDGE_CURVE('',#20017,#18900,#11333,.T.);
#26196=EDGE_CURVE('',#20018,#18901,#11334,.T.);
#26197=EDGE_CURVE('',#20016,#18902,#11335,.T.);
#26198=EDGE_CURVE('',#20021,#18903,#11336,.T.);
#26199=EDGE_CURVE('',#20020,#18904,#11337,.T.);
#26200=EDGE_CURVE('',#20019,#18905,#11338,.T.);
#26201=EDGE_CURVE('',#20011,#18894,#11339,.T.);
#26202=EDGE_CURVE('',#20012,#18895,#11340,.T.);
#26203=EDGE_CURVE('',#20010,#18896,#11341,.T.);
#26204=EDGE_CURVE('',#20015,#18897,#11342,.T.);
#26205=EDGE_CURVE('',#20014,#18898,#11343,.T.);
#26206=EDGE_CURVE('',#20013,#18899,#11344,.T.);
#26207=EDGE_CURVE('',#20005,#18888,#11345,.T.);
#26208=EDGE_CURVE('',#20006,#18889,#11346,.T.);
#26209=EDGE_CURVE('',#20004,#18890,#11347,.T.);
#26210=EDGE_CURVE('',#20009,#18891,#11348,.T.);
#26211=EDGE_CURVE('',#20008,#18892,#11349,.T.);
#26212=EDGE_CURVE('',#20007,#18893,#11350,.T.);
#26213=EDGE_CURVE('',#19999,#18882,#11351,.T.);
#26214=EDGE_CURVE('',#20000,#18883,#11352,.T.);
#26215=EDGE_CURVE('',#19998,#18884,#11353,.T.);
#26216=EDGE_CURVE('',#20003,#18885,#11354,.T.);
#26217=EDGE_CURVE('',#20002,#18886,#11355,.T.);
#26218=EDGE_CURVE('',#20001,#18887,#11356,.T.);
#26219=EDGE_CURVE('',#19993,#18876,#11357,.T.);
#26220=EDGE_CURVE('',#19994,#18877,#11358,.T.);
#26221=EDGE_CURVE('',#19992,#18878,#11359,.T.);
#26222=EDGE_CURVE('',#19997,#18879,#11360,.T.);
#26223=EDGE_CURVE('',#19996,#18880,#11361,.T.);
#26224=EDGE_CURVE('',#19995,#18881,#11362,.T.);
#26225=EDGE_CURVE('',#19987,#18870,#11363,.T.);
#26226=EDGE_CURVE('',#19988,#18871,#11364,.T.);
#26227=EDGE_CURVE('',#19986,#18872,#11365,.T.);
#26228=EDGE_CURVE('',#19991,#18873,#11366,.T.);
#26229=EDGE_CURVE('',#19990,#18874,#11367,.T.);
#26230=EDGE_CURVE('',#19989,#18875,#11368,.T.);
#26231=EDGE_CURVE('',#19981,#18864,#11369,.T.);
#26232=EDGE_CURVE('',#19982,#18865,#11370,.T.);
#26233=EDGE_CURVE('',#19980,#18866,#11371,.T.);
#26234=EDGE_CURVE('',#19985,#18867,#11372,.T.);
#26235=EDGE_CURVE('',#19984,#18868,#11373,.T.);
#26236=EDGE_CURVE('',#19983,#18869,#11374,.T.);
#26237=EDGE_CURVE('',#19975,#18858,#11375,.T.);
#26238=EDGE_CURVE('',#19976,#18859,#11376,.T.);
#26239=EDGE_CURVE('',#19974,#18860,#11377,.T.);
#26240=EDGE_CURVE('',#19979,#18861,#11378,.T.);
#26241=EDGE_CURVE('',#19978,#18862,#11379,.T.);
#26242=EDGE_CURVE('',#19977,#18863,#11380,.T.);
#26243=EDGE_CURVE('',#19969,#18852,#11381,.T.);
#26244=EDGE_CURVE('',#19970,#18853,#11382,.T.);
#26245=EDGE_CURVE('',#19968,#18854,#11383,.T.);
#26246=EDGE_CURVE('',#19973,#18855,#11384,.T.);
#26247=EDGE_CURVE('',#19972,#18856,#11385,.T.);
#26248=EDGE_CURVE('',#19971,#18857,#11386,.T.);
#26249=EDGE_CURVE('',#19963,#18846,#11387,.T.);
#26250=EDGE_CURVE('',#19964,#18847,#11388,.T.);
#26251=EDGE_CURVE('',#19962,#18848,#11389,.T.);
#26252=EDGE_CURVE('',#19967,#18849,#11390,.T.);
#26253=EDGE_CURVE('',#19966,#18850,#11391,.T.);
#26254=EDGE_CURVE('',#19965,#18851,#11392,.T.);
#26255=EDGE_CURVE('',#19957,#18840,#11393,.T.);
#26256=EDGE_CURVE('',#19958,#18841,#11394,.T.);
#26257=EDGE_CURVE('',#19956,#18842,#11395,.T.);
#26258=EDGE_CURVE('',#19961,#18843,#11396,.T.);
#26259=EDGE_CURVE('',#19960,#18844,#11397,.T.);
#26260=EDGE_CURVE('',#19959,#18845,#11398,.T.);
#26261=EDGE_CURVE('',#19951,#18834,#11399,.T.);
#26262=EDGE_CURVE('',#19952,#18835,#11400,.T.);
#26263=EDGE_CURVE('',#19950,#18836,#11401,.T.);
#26264=EDGE_CURVE('',#19955,#18837,#11402,.T.);
#26265=EDGE_CURVE('',#19954,#18838,#11403,.T.);
#26266=EDGE_CURVE('',#19953,#18839,#11404,.T.);
#26267=EDGE_CURVE('',#19945,#18828,#11405,.T.);
#26268=EDGE_CURVE('',#19946,#18829,#11406,.T.);
#26269=EDGE_CURVE('',#19944,#18830,#11407,.T.);
#26270=EDGE_CURVE('',#19949,#18831,#11408,.T.);
#26271=EDGE_CURVE('',#19948,#18832,#11409,.T.);
#26272=EDGE_CURVE('',#19947,#18833,#11410,.T.);
#26273=EDGE_CURVE('',#19939,#18822,#11411,.T.);
#26274=EDGE_CURVE('',#19940,#18823,#11412,.T.);
#26275=EDGE_CURVE('',#19938,#18824,#11413,.T.);
#26276=EDGE_CURVE('',#19943,#18825,#11414,.T.);
#26277=EDGE_CURVE('',#19942,#18826,#11415,.T.);
#26278=EDGE_CURVE('',#19941,#18827,#11416,.T.);
#26279=EDGE_CURVE('',#19933,#18816,#11417,.T.);
#26280=EDGE_CURVE('',#19934,#18817,#11418,.T.);
#26281=EDGE_CURVE('',#19932,#18818,#11419,.T.);
#26282=EDGE_CURVE('',#19937,#18819,#11420,.T.);
#26283=EDGE_CURVE('',#19936,#18820,#11421,.T.);
#26284=EDGE_CURVE('',#19935,#18821,#11422,.T.);
#26285=EDGE_CURVE('',#19927,#18810,#11423,.T.);
#26286=EDGE_CURVE('',#19928,#18811,#11424,.T.);
#26287=EDGE_CURVE('',#19926,#18812,#11425,.T.);
#26288=EDGE_CURVE('',#19931,#18813,#11426,.T.);
#26289=EDGE_CURVE('',#19930,#18814,#11427,.T.);
#26290=EDGE_CURVE('',#19929,#18815,#11428,.T.);
#26291=EDGE_CURVE('',#19921,#18804,#11429,.T.);
#26292=EDGE_CURVE('',#19922,#18805,#11430,.T.);
#26293=EDGE_CURVE('',#19920,#18806,#11431,.T.);
#26294=EDGE_CURVE('',#19925,#18807,#11432,.T.);
#26295=EDGE_CURVE('',#19924,#18808,#11433,.T.);
#26296=EDGE_CURVE('',#19923,#18809,#11434,.T.);
#26297=EDGE_CURVE('',#19915,#18798,#11435,.T.);
#26298=EDGE_CURVE('',#19916,#18799,#11436,.T.);
#26299=EDGE_CURVE('',#19914,#18800,#11437,.T.);
#26300=EDGE_CURVE('',#19919,#18801,#11438,.T.);
#26301=EDGE_CURVE('',#19918,#18802,#11439,.T.);
#26302=EDGE_CURVE('',#19917,#18803,#11440,.T.);
#26303=EDGE_CURVE('',#19909,#18792,#11441,.T.);
#26304=EDGE_CURVE('',#19910,#18793,#11442,.T.);
#26305=EDGE_CURVE('',#19908,#18794,#11443,.T.);
#26306=EDGE_CURVE('',#19913,#18795,#11444,.T.);
#26307=EDGE_CURVE('',#19912,#18796,#11445,.T.);
#26308=EDGE_CURVE('',#19911,#18797,#11446,.T.);
#26309=EDGE_CURVE('',#19903,#18786,#11447,.T.);
#26310=EDGE_CURVE('',#19904,#18787,#11448,.T.);
#26311=EDGE_CURVE('',#19902,#18788,#11449,.T.);
#26312=EDGE_CURVE('',#19907,#18789,#11450,.T.);
#26313=EDGE_CURVE('',#19906,#18790,#11451,.T.);
#26314=EDGE_CURVE('',#19905,#18791,#11452,.T.);
#26315=EDGE_CURVE('',#19897,#18780,#11453,.T.);
#26316=EDGE_CURVE('',#19898,#18781,#11454,.T.);
#26317=EDGE_CURVE('',#19896,#18782,#11455,.T.);
#26318=EDGE_CURVE('',#19901,#18783,#11456,.T.);
#26319=EDGE_CURVE('',#19900,#18784,#11457,.T.);
#26320=EDGE_CURVE('',#19899,#18785,#11458,.T.);
#26321=EDGE_CURVE('',#19891,#18774,#11459,.T.);
#26322=EDGE_CURVE('',#19892,#18775,#11460,.T.);
#26323=EDGE_CURVE('',#19890,#18776,#11461,.T.);
#26324=EDGE_CURVE('',#19895,#18777,#11462,.T.);
#26325=EDGE_CURVE('',#19894,#18778,#11463,.T.);
#26326=EDGE_CURVE('',#19893,#18779,#11464,.T.);
#26327=EDGE_CURVE('',#19885,#18768,#11465,.T.);
#26328=EDGE_CURVE('',#19886,#18769,#11466,.T.);
#26329=EDGE_CURVE('',#19884,#18770,#11467,.T.);
#26330=EDGE_CURVE('',#19889,#18771,#11468,.T.);
#26331=EDGE_CURVE('',#19888,#18772,#11469,.T.);
#26332=EDGE_CURVE('',#19887,#18773,#11470,.T.);
#26333=EDGE_CURVE('',#19879,#18762,#11471,.T.);
#26334=EDGE_CURVE('',#19880,#18763,#11472,.T.);
#26335=EDGE_CURVE('',#19878,#18764,#11473,.T.);
#26336=EDGE_CURVE('',#19883,#18765,#11474,.T.);
#26337=EDGE_CURVE('',#19882,#18766,#11475,.T.);
#26338=EDGE_CURVE('',#19881,#18767,#11476,.T.);
#26339=EDGE_CURVE('',#19873,#18756,#11477,.T.);
#26340=EDGE_CURVE('',#19874,#18757,#11478,.T.);
#26341=EDGE_CURVE('',#19872,#18758,#11479,.T.);
#26342=EDGE_CURVE('',#19877,#18759,#11480,.T.);
#26343=EDGE_CURVE('',#19876,#18760,#11481,.T.);
#26344=EDGE_CURVE('',#19875,#18761,#11482,.T.);
#26345=EDGE_CURVE('',#19867,#18750,#11483,.T.);
#26346=EDGE_CURVE('',#19868,#18751,#11484,.T.);
#26347=EDGE_CURVE('',#19866,#18752,#11485,.T.);
#26348=EDGE_CURVE('',#19871,#18753,#11486,.T.);
#26349=EDGE_CURVE('',#19870,#18754,#11487,.T.);
#26350=EDGE_CURVE('',#19869,#18755,#11488,.T.);
#26351=EDGE_CURVE('',#19861,#18744,#11489,.T.);
#26352=EDGE_CURVE('',#19862,#18745,#11490,.T.);
#26353=EDGE_CURVE('',#19860,#18746,#11491,.T.);
#26354=EDGE_CURVE('',#19865,#18747,#11492,.T.);
#26355=EDGE_CURVE('',#19864,#18748,#11493,.T.);
#26356=EDGE_CURVE('',#19863,#18749,#11494,.T.);
#26357=EDGE_CURVE('',#19855,#18738,#11495,.T.);
#26358=EDGE_CURVE('',#19856,#18739,#11496,.T.);
#26359=EDGE_CURVE('',#19854,#18740,#11497,.T.);
#26360=EDGE_CURVE('',#19859,#18741,#11498,.T.);
#26361=EDGE_CURVE('',#19858,#18742,#11499,.T.);
#26362=EDGE_CURVE('',#19857,#18743,#11500,.T.);
#26363=EDGE_CURVE('',#19849,#18732,#11501,.T.);
#26364=EDGE_CURVE('',#19850,#18733,#11502,.T.);
#26365=EDGE_CURVE('',#19848,#18734,#11503,.T.);
#26366=EDGE_CURVE('',#19853,#18735,#11504,.T.);
#26367=EDGE_CURVE('',#19852,#18736,#11505,.T.);
#26368=EDGE_CURVE('',#19851,#18737,#11506,.T.);
#26369=EDGE_CURVE('',#19843,#18726,#11507,.T.);
#26370=EDGE_CURVE('',#19844,#18727,#11508,.T.);
#26371=EDGE_CURVE('',#19842,#18728,#11509,.T.);
#26372=EDGE_CURVE('',#19847,#18729,#11510,.T.);
#26373=EDGE_CURVE('',#19846,#18730,#11511,.T.);
#26374=EDGE_CURVE('',#19845,#18731,#11512,.T.);
#26375=EDGE_CURVE('',#19837,#18720,#11513,.T.);
#26376=EDGE_CURVE('',#19838,#18721,#11514,.T.);
#26377=EDGE_CURVE('',#19836,#18722,#11515,.T.);
#26378=EDGE_CURVE('',#19841,#18723,#11516,.T.);
#26379=EDGE_CURVE('',#19840,#18724,#11517,.T.);
#26380=EDGE_CURVE('',#19839,#18725,#11518,.T.);
#26381=EDGE_CURVE('',#19831,#18714,#11519,.T.);
#26382=EDGE_CURVE('',#19832,#18715,#11520,.T.);
#26383=EDGE_CURVE('',#19830,#18716,#11521,.T.);
#26384=EDGE_CURVE('',#19835,#18717,#11522,.T.);
#26385=EDGE_CURVE('',#19834,#18718,#11523,.T.);
#26386=EDGE_CURVE('',#19833,#18719,#11524,.T.);
#26387=EDGE_CURVE('',#19825,#18708,#11525,.T.);
#26388=EDGE_CURVE('',#19826,#18709,#11526,.T.);
#26389=EDGE_CURVE('',#19824,#18710,#11527,.T.);
#26390=EDGE_CURVE('',#19829,#18711,#11528,.T.);
#26391=EDGE_CURVE('',#19828,#18712,#11529,.T.);
#26392=EDGE_CURVE('',#19827,#18713,#11530,.T.);
#26393=EDGE_CURVE('',#19819,#18702,#11531,.T.);
#26394=EDGE_CURVE('',#19820,#18703,#11532,.T.);
#26395=EDGE_CURVE('',#19818,#18704,#11533,.T.);
#26396=EDGE_CURVE('',#19823,#18705,#11534,.T.);
#26397=EDGE_CURVE('',#19822,#18706,#11535,.T.);
#26398=EDGE_CURVE('',#19821,#18707,#11536,.T.);
#26399=EDGE_CURVE('',#19813,#18696,#11537,.T.);
#26400=EDGE_CURVE('',#19814,#18697,#11538,.T.);
#26401=EDGE_CURVE('',#19812,#18698,#11539,.T.);
#26402=EDGE_CURVE('',#19817,#18699,#11540,.T.);
#26403=EDGE_CURVE('',#19816,#18700,#11541,.T.);
#26404=EDGE_CURVE('',#19815,#18701,#11542,.T.);
#26405=EDGE_CURVE('',#19807,#18690,#11543,.T.);
#26406=EDGE_CURVE('',#19808,#18691,#11544,.T.);
#26407=EDGE_CURVE('',#19806,#18692,#11545,.T.);
#26408=EDGE_CURVE('',#19811,#18693,#11546,.T.);
#26409=EDGE_CURVE('',#19810,#18694,#11547,.T.);
#26410=EDGE_CURVE('',#19809,#18695,#11548,.T.);
#26411=EDGE_CURVE('',#19801,#18684,#11549,.T.);
#26412=EDGE_CURVE('',#19802,#18685,#11550,.T.);
#26413=EDGE_CURVE('',#19800,#18686,#11551,.T.);
#26414=EDGE_CURVE('',#19805,#18687,#11552,.T.);
#26415=EDGE_CURVE('',#19804,#18688,#11553,.T.);
#26416=EDGE_CURVE('',#19803,#18689,#11554,.T.);
#26417=EDGE_CURVE('',#19795,#18678,#11555,.T.);
#26418=EDGE_CURVE('',#19796,#18679,#11556,.T.);
#26419=EDGE_CURVE('',#19794,#18680,#11557,.T.);
#26420=EDGE_CURVE('',#19799,#18681,#11558,.T.);
#26421=EDGE_CURVE('',#19798,#18682,#11559,.T.);
#26422=EDGE_CURVE('',#19797,#18683,#11560,.T.);
#26423=EDGE_CURVE('',#19789,#18672,#11561,.T.);
#26424=EDGE_CURVE('',#19790,#18673,#11562,.T.);
#26425=EDGE_CURVE('',#19788,#18674,#11563,.T.);
#26426=EDGE_CURVE('',#19793,#18675,#11564,.T.);
#26427=EDGE_CURVE('',#19792,#18676,#11565,.T.);
#26428=EDGE_CURVE('',#19791,#18677,#11566,.T.);
#26429=EDGE_CURVE('',#19783,#18666,#11567,.T.);
#26430=EDGE_CURVE('',#19784,#18667,#11568,.T.);
#26431=EDGE_CURVE('',#19782,#18668,#11569,.T.);
#26432=EDGE_CURVE('',#19787,#18669,#11570,.T.);
#26433=EDGE_CURVE('',#19786,#18670,#11571,.T.);
#26434=EDGE_CURVE('',#19785,#18671,#11572,.T.);
#26435=EDGE_CURVE('',#19777,#18660,#11573,.T.);
#26436=EDGE_CURVE('',#19778,#18661,#11574,.T.);
#26437=EDGE_CURVE('',#19776,#18662,#11575,.T.);
#26438=EDGE_CURVE('',#19781,#18663,#11576,.T.);
#26439=EDGE_CURVE('',#19780,#18664,#11577,.T.);
#26440=EDGE_CURVE('',#19779,#18665,#11578,.T.);
#26441=EDGE_CURVE('',#19771,#18654,#11579,.T.);
#26442=EDGE_CURVE('',#19772,#18655,#11580,.T.);
#26443=EDGE_CURVE('',#19770,#18656,#11581,.T.);
#26444=EDGE_CURVE('',#19775,#18657,#11582,.T.);
#26445=EDGE_CURVE('',#19774,#18658,#11583,.T.);
#26446=EDGE_CURVE('',#19773,#18659,#11584,.T.);
#26447=EDGE_CURVE('',#19765,#18648,#11585,.T.);
#26448=EDGE_CURVE('',#19766,#18649,#11586,.T.);
#26449=EDGE_CURVE('',#19764,#18650,#11587,.T.);
#26450=EDGE_CURVE('',#19769,#18651,#11588,.T.);
#26451=EDGE_CURVE('',#19768,#18652,#11589,.T.);
#26452=EDGE_CURVE('',#19767,#18653,#11590,.T.);
#26453=EDGE_CURVE('',#19759,#18642,#11591,.T.);
#26454=EDGE_CURVE('',#19760,#18643,#11592,.T.);
#26455=EDGE_CURVE('',#19758,#18644,#11593,.T.);
#26456=EDGE_CURVE('',#19763,#18645,#11594,.T.);
#26457=EDGE_CURVE('',#19762,#18646,#11595,.T.);
#26458=EDGE_CURVE('',#19761,#18647,#11596,.T.);
#26459=EDGE_CURVE('',#19753,#18636,#11597,.T.);
#26460=EDGE_CURVE('',#19754,#18637,#11598,.T.);
#26461=EDGE_CURVE('',#19752,#18638,#11599,.T.);
#26462=EDGE_CURVE('',#19757,#18639,#11600,.T.);
#26463=EDGE_CURVE('',#19756,#18640,#11601,.T.);
#26464=EDGE_CURVE('',#19755,#18641,#11602,.T.);
#26465=EDGE_CURVE('',#19747,#18630,#11603,.T.);
#26466=EDGE_CURVE('',#19748,#18631,#11604,.T.);
#26467=EDGE_CURVE('',#19746,#18632,#11605,.T.);
#26468=EDGE_CURVE('',#19751,#18633,#11606,.T.);
#26469=EDGE_CURVE('',#19750,#18634,#11607,.T.);
#26470=EDGE_CURVE('',#19749,#18635,#11608,.T.);
#26471=EDGE_CURVE('',#19741,#18624,#11609,.T.);
#26472=EDGE_CURVE('',#19742,#18625,#11610,.T.);
#26473=EDGE_CURVE('',#19740,#18626,#11611,.T.);
#26474=EDGE_CURVE('',#19745,#18627,#11612,.T.);
#26475=EDGE_CURVE('',#19744,#18628,#11613,.T.);
#26476=EDGE_CURVE('',#19743,#18629,#11614,.T.);
#30779=ORIENTED_EDGE('',*,*,#23007,.F.);
#30780=ORIENTED_EDGE('',*,*,#23008,.T.);
#30781=ORIENTED_EDGE('',*,*,#23009,.T.);
#30782=ORIENTED_EDGE('',*,*,#23008,.F.);
#30783=ORIENTED_EDGE('',*,*,#23010,.F.);
#30784=ORIENTED_EDGE('',*,*,#23011,.T.);
#30785=ORIENTED_EDGE('',*,*,#23012,.T.);
#30786=ORIENTED_EDGE('',*,*,#23011,.F.);
#30787=ORIENTED_EDGE('',*,*,#23013,.F.);
#30788=ORIENTED_EDGE('',*,*,#23014,.T.);
#30789=ORIENTED_EDGE('',*,*,#23010,.T.);
#30790=ORIENTED_EDGE('',*,*,#23014,.F.);
#30791=ORIENTED_EDGE('',*,*,#23015,.T.);
#30792=ORIENTED_EDGE('',*,*,#23016,.T.);
#30793=ORIENTED_EDGE('',*,*,#23007,.T.);
#30794=ORIENTED_EDGE('',*,*,#23016,.F.);
#30795=ORIENTED_EDGE('',*,*,#23017,.F.);
#30796=ORIENTED_EDGE('',*,*,#23018,.F.);
#30797=ORIENTED_EDGE('',*,*,#23019,.T.);
#30798=ORIENTED_EDGE('',*,*,#23020,.F.);
#30799=ORIENTED_EDGE('',*,*,#23021,.T.);
#30800=ORIENTED_EDGE('',*,*,#23022,.T.);
#30801=ORIENTED_EDGE('',*,*,#23023,.F.);
#30802=ORIENTED_EDGE('',*,*,#23024,.T.);
#30803=ORIENTED_EDGE('',*,*,#23025,.T.);
#30804=ORIENTED_EDGE('',*,*,#23026,.T.);
#30805=ORIENTED_EDGE('',*,*,#23027,.F.);
#30806=ORIENTED_EDGE('',*,*,#23028,.F.);
#30807=ORIENTED_EDGE('',*,*,#23015,.F.);
#30808=ORIENTED_EDGE('',*,*,#23029,.F.);
#30809=ORIENTED_EDGE('',*,*,#23030,.F.);
#30810=ORIENTED_EDGE('',*,*,#23031,.T.);
#30811=ORIENTED_EDGE('',*,*,#23032,.T.);
#30812=ORIENTED_EDGE('',*,*,#23033,.F.);
#30813=ORIENTED_EDGE('',*,*,#23034,.T.);
#30814=ORIENTED_EDGE('',*,*,#23035,.T.);
#30815=ORIENTED_EDGE('',*,*,#23036,.F.);
#30816=ORIENTED_EDGE('',*,*,#23037,.F.);
#30817=ORIENTED_EDGE('',*,*,#23038,.F.);
#30818=ORIENTED_EDGE('',*,*,#23039,.T.);
#30819=ORIENTED_EDGE('',*,*,#23040,.T.);
#30820=ORIENTED_EDGE('',*,*,#23012,.F.);
#30821=ORIENTED_EDGE('',*,*,#23027,.T.);
#30822=ORIENTED_EDGE('',*,*,#23041,.T.);
#30823=ORIENTED_EDGE('',*,*,#23032,.F.);
#30824=ORIENTED_EDGE('',*,*,#23042,.T.);
#30825=ORIENTED_EDGE('',*,*,#23021,.F.);
#30826=ORIENTED_EDGE('',*,*,#23043,.T.);
#30827=ORIENTED_EDGE('',*,*,#23038,.T.);
#30828=ORIENTED_EDGE('',*,*,#23044,.T.);
#30829=ORIENTED_EDGE('',*,*,#23045,.F.);
#30830=ORIENTED_EDGE('',*,*,#23030,.T.);
#30831=ORIENTED_EDGE('',*,*,#23046,.F.);
#30832=ORIENTED_EDGE('',*,*,#23017,.T.);
#30833=ORIENTED_EDGE('',*,*,#23047,.F.);
#30834=ORIENTED_EDGE('',*,*,#23019,.F.);
#30835=ORIENTED_EDGE('',*,*,#23048,.T.);
#30836=ORIENTED_EDGE('',*,*,#23040,.F.);
#30837=ORIENTED_EDGE('',*,*,#23018,.T.);
#30838=ORIENTED_EDGE('',*,*,#23046,.T.);
#30839=ORIENTED_EDGE('',*,*,#23029,.T.);
#30840=ORIENTED_EDGE('',*,*,#23048,.F.);
#30841=ORIENTED_EDGE('',*,*,#23049,.F.);
#30842=ORIENTED_EDGE('',*,*,#23025,.F.);
#30843=ORIENTED_EDGE('',*,*,#23050,.T.);
#30844=ORIENTED_EDGE('',*,*,#23034,.F.);
#30845=ORIENTED_EDGE('',*,*,#23051,.T.);
#30846=ORIENTED_EDGE('',*,*,#23035,.F.);
#30847=ORIENTED_EDGE('',*,*,#23050,.F.);
#30848=ORIENTED_EDGE('',*,*,#23024,.F.);
#30849=ORIENTED_EDGE('',*,*,#23052,.F.);
#30850=ORIENTED_EDGE('',*,*,#23036,.T.);
#30851=ORIENTED_EDGE('',*,*,#23051,.F.);
#30852=ORIENTED_EDGE('',*,*,#23023,.T.);
#30853=ORIENTED_EDGE('',*,*,#23053,.T.);
#30854=ORIENTED_EDGE('',*,*,#23054,.T.);
#30855=ORIENTED_EDGE('',*,*,#23049,.T.);
#30856=ORIENTED_EDGE('',*,*,#23055,.F.);
#30857=ORIENTED_EDGE('',*,*,#23056,.T.);
#30858=ORIENTED_EDGE('',*,*,#23057,.F.);
#30859=ORIENTED_EDGE('',*,*,#23058,.F.);
#30860=ORIENTED_EDGE('',*,*,#23041,.F.);
#30861=ORIENTED_EDGE('',*,*,#23033,.T.);
#30862=ORIENTED_EDGE('',*,*,#23058,.T.);
#30863=ORIENTED_EDGE('',*,*,#23059,.F.);
#30864=ORIENTED_EDGE('',*,*,#23055,.T.);
#30865=ORIENTED_EDGE('',*,*,#23026,.F.);
#30866=ORIENTED_EDGE('',*,*,#23054,.F.);
#30867=ORIENTED_EDGE('',*,*,#23060,.T.);
#30868=ORIENTED_EDGE('',*,*,#23056,.F.);
#30869=ORIENTED_EDGE('',*,*,#23052,.T.);
#30870=ORIENTED_EDGE('',*,*,#23061,.T.);
#30871=ORIENTED_EDGE('',*,*,#23062,.T.);
#30872=ORIENTED_EDGE('',*,*,#23063,.F.);
#30873=ORIENTED_EDGE('',*,*,#23064,.F.);
#30874=ORIENTED_EDGE('',*,*,#23065,.T.);
#30875=ORIENTED_EDGE('',*,*,#23044,.F.);
#30876=ORIENTED_EDGE('',*,*,#23066,.F.);
#30877=ORIENTED_EDGE('',*,*,#23066,.T.);
#30878=ORIENTED_EDGE('',*,*,#23037,.T.);
#30879=ORIENTED_EDGE('',*,*,#23063,.T.);
#30880=ORIENTED_EDGE('',*,*,#23067,.F.);
#30881=ORIENTED_EDGE('',*,*,#23065,.F.);
#30882=ORIENTED_EDGE('',*,*,#23068,.T.);
#30883=ORIENTED_EDGE('',*,*,#23061,.F.);
#30884=ORIENTED_EDGE('',*,*,#23022,.F.);
#30885=ORIENTED_EDGE('',*,*,#23069,.F.);
#30886=ORIENTED_EDGE('',*,*,#23070,.F.);
#30887=ORIENTED_EDGE('',*,*,#23071,.F.);
#30888=ORIENTED_EDGE('',*,*,#23072,.F.);
#30889=ORIENTED_EDGE('',*,*,#23073,.T.);
#30890=ORIENTED_EDGE('',*,*,#23074,.T.);
#30891=ORIENTED_EDGE('',*,*,#23075,.T.);
#30892=ORIENTED_EDGE('',*,*,#23076,.F.);
#30893=ORIENTED_EDGE('',*,*,#23077,.F.);
#30894=ORIENTED_EDGE('',*,*,#23078,.F.);
#30895=ORIENTED_EDGE('',*,*,#23079,.F.);
#30896=ORIENTED_EDGE('',*,*,#23080,.F.);
#30897=ORIENTED_EDGE('',*,*,#23081,.F.);
#30898=ORIENTED_EDGE('',*,*,#23078,.T.);
#30899=ORIENTED_EDGE('',*,*,#23082,.T.);
#30900=ORIENTED_EDGE('',*,*,#23072,.T.);
#30901=ORIENTED_EDGE('',*,*,#23082,.F.);
#30902=ORIENTED_EDGE('',*,*,#23077,.T.);
#30903=ORIENTED_EDGE('',*,*,#23083,.F.);
#30904=ORIENTED_EDGE('',*,*,#23067,.T.);
#30905=ORIENTED_EDGE('',*,*,#23084,.F.);
#30906=ORIENTED_EDGE('',*,*,#23075,.F.);
#30907=ORIENTED_EDGE('',*,*,#23085,.T.);
#30908=ORIENTED_EDGE('',*,*,#23059,.T.);
#30909=ORIENTED_EDGE('',*,*,#23086,.T.);
#30910=ORIENTED_EDGE('',*,*,#23069,.T.);
#30911=ORIENTED_EDGE('',*,*,#23062,.F.);
#30912=ORIENTED_EDGE('',*,*,#23087,.T.);
#30913=ORIENTED_EDGE('',*,*,#23076,.T.);
#30914=ORIENTED_EDGE('',*,*,#23084,.T.);
#30915=ORIENTED_EDGE('',*,*,#23088,.T.);
#30916=ORIENTED_EDGE('',*,*,#23079,.T.);
#30917=ORIENTED_EDGE('',*,*,#23081,.T.);
#30918=ORIENTED_EDGE('',*,*,#23071,.T.);
#30919=ORIENTED_EDGE('',*,*,#23089,.F.);
#30920=ORIENTED_EDGE('',*,*,#23060,.F.);
#30921=ORIENTED_EDGE('',*,*,#23090,.T.);
#30922=ORIENTED_EDGE('',*,*,#23073,.F.);
#30923=ORIENTED_EDGE('',*,*,#23087,.F.);
#30924=ORIENTED_EDGE('',*,*,#23068,.F.);
#30925=ORIENTED_EDGE('',*,*,#23083,.T.);
#30926=ORIENTED_EDGE('',*,*,#23080,.T.);
#30927=ORIENTED_EDGE('',*,*,#23088,.F.);
#30928=ORIENTED_EDGE('',*,*,#23064,.T.);
#30929=ORIENTED_EDGE('',*,*,#23089,.T.);
#30930=ORIENTED_EDGE('',*,*,#23070,.T.);
#30931=ORIENTED_EDGE('',*,*,#23086,.F.);
#30932=ORIENTED_EDGE('',*,*,#23057,.T.);
#30933=ORIENTED_EDGE('',*,*,#23053,.F.);
#30934=ORIENTED_EDGE('',*,*,#23085,.F.);
#30935=ORIENTED_EDGE('',*,*,#23074,.F.);
#30936=ORIENTED_EDGE('',*,*,#23090,.F.);
#30937=ORIENTED_EDGE('',*,*,#23091,.T.);
#30938=ORIENTED_EDGE('',*,*,#23092,.T.);
#30939=ORIENTED_EDGE('',*,*,#23047,.T.);
#30940=ORIENTED_EDGE('',*,*,#23093,.F.);
#30941=ORIENTED_EDGE('',*,*,#23094,.T.);
#30942=ORIENTED_EDGE('',*,*,#23095,.F.);
#30943=ORIENTED_EDGE('',*,*,#23096,.F.);
#30944=ORIENTED_EDGE('',*,*,#23043,.F.);
#30945=ORIENTED_EDGE('',*,*,#23039,.F.);
#30946=ORIENTED_EDGE('',*,*,#23096,.T.);
#30947=ORIENTED_EDGE('',*,*,#23097,.T.);
#30948=ORIENTED_EDGE('',*,*,#23093,.T.);
#30949=ORIENTED_EDGE('',*,*,#23020,.T.);
#30950=ORIENTED_EDGE('',*,*,#23092,.F.);
#30951=ORIENTED_EDGE('',*,*,#23098,.F.);
#30952=ORIENTED_EDGE('',*,*,#23094,.F.);
#30953=ORIENTED_EDGE('',*,*,#23045,.T.);
#30954=ORIENTED_EDGE('',*,*,#23099,.T.);
#30955=ORIENTED_EDGE('',*,*,#23100,.T.);
#30956=ORIENTED_EDGE('',*,*,#23101,.F.);
#30957=ORIENTED_EDGE('',*,*,#23102,.F.);
#30958=ORIENTED_EDGE('',*,*,#23103,.T.);
#30959=ORIENTED_EDGE('',*,*,#23042,.F.);
#30960=ORIENTED_EDGE('',*,*,#23104,.F.);
#30961=ORIENTED_EDGE('',*,*,#23104,.T.);
#30962=ORIENTED_EDGE('',*,*,#23031,.F.);
#30963=ORIENTED_EDGE('',*,*,#23101,.T.);
#30964=ORIENTED_EDGE('',*,*,#23105,.T.);
#30965=ORIENTED_EDGE('',*,*,#23103,.F.);
#30966=ORIENTED_EDGE('',*,*,#23106,.F.);
#30967=ORIENTED_EDGE('',*,*,#23099,.F.);
#30968=ORIENTED_EDGE('',*,*,#23028,.T.);
#30969=ORIENTED_EDGE('',*,*,#23107,.F.);
#30970=ORIENTED_EDGE('',*,*,#23108,.F.);
#30971=ORIENTED_EDGE('',*,*,#23109,.F.);
#30972=ORIENTED_EDGE('',*,*,#23110,.F.);
#30973=ORIENTED_EDGE('',*,*,#23111,.T.);
#30974=ORIENTED_EDGE('',*,*,#23112,.F.);
#30975=ORIENTED_EDGE('',*,*,#23113,.F.);
#30976=ORIENTED_EDGE('',*,*,#23114,.F.);
#30977=ORIENTED_EDGE('',*,*,#23115,.F.);
#30978=ORIENTED_EDGE('',*,*,#23116,.F.);
#30979=ORIENTED_EDGE('',*,*,#23117,.F.);
#30980=ORIENTED_EDGE('',*,*,#23118,.F.);
#30981=ORIENTED_EDGE('',*,*,#23119,.T.);
#30982=ORIENTED_EDGE('',*,*,#23118,.T.);
#30983=ORIENTED_EDGE('',*,*,#23120,.F.);
#30984=ORIENTED_EDGE('',*,*,#23108,.T.);
#30985=ORIENTED_EDGE('',*,*,#23120,.T.);
#30986=ORIENTED_EDGE('',*,*,#23117,.T.);
#30987=ORIENTED_EDGE('',*,*,#23121,.T.);
#30988=ORIENTED_EDGE('',*,*,#23105,.F.);
#30989=ORIENTED_EDGE('',*,*,#23122,.F.);
#30990=ORIENTED_EDGE('',*,*,#23112,.T.);
#30991=ORIENTED_EDGE('',*,*,#23123,.T.);
#30992=ORIENTED_EDGE('',*,*,#23097,.F.);
#30993=ORIENTED_EDGE('',*,*,#23124,.F.);
#30994=ORIENTED_EDGE('',*,*,#23109,.T.);
#30995=ORIENTED_EDGE('',*,*,#23100,.F.);
#30996=ORIENTED_EDGE('',*,*,#23125,.T.);
#30997=ORIENTED_EDGE('',*,*,#23113,.T.);
#30998=ORIENTED_EDGE('',*,*,#23122,.T.);
#30999=ORIENTED_EDGE('',*,*,#23126,.F.);
#31000=ORIENTED_EDGE('',*,*,#23115,.T.);
#31001=ORIENTED_EDGE('',*,*,#23119,.F.);
#31002=ORIENTED_EDGE('',*,*,#23107,.T.);
#31003=ORIENTED_EDGE('',*,*,#23127,.T.);
#31004=ORIENTED_EDGE('',*,*,#23098,.T.);
#31005=ORIENTED_EDGE('',*,*,#23128,.T.);
#31006=ORIENTED_EDGE('',*,*,#23114,.T.);
#31007=ORIENTED_EDGE('',*,*,#23125,.F.);
#31008=ORIENTED_EDGE('',*,*,#23106,.T.);
#31009=ORIENTED_EDGE('',*,*,#23121,.F.);
#31010=ORIENTED_EDGE('',*,*,#23116,.T.);
#31011=ORIENTED_EDGE('',*,*,#23126,.T.);
#31012=ORIENTED_EDGE('',*,*,#23102,.T.);
#31013=ORIENTED_EDGE('',*,*,#23127,.F.);
#31014=ORIENTED_EDGE('',*,*,#23110,.T.);
#31015=ORIENTED_EDGE('',*,*,#23124,.T.);
#31016=ORIENTED_EDGE('',*,*,#23095,.T.);
#31017=ORIENTED_EDGE('',*,*,#23091,.F.);
#31018=ORIENTED_EDGE('',*,*,#23123,.F.);
#31019=ORIENTED_EDGE('',*,*,#23111,.F.);
#31020=ORIENTED_EDGE('',*,*,#23128,.F.);
#31021=ORIENTED_EDGE('',*,*,#23013,.T.);
#31022=ORIENTED_EDGE('',*,*,#23129,.F.);
#31023=ORIENTED_EDGE('',*,*,#23130,.F.);
#31024=ORIENTED_EDGE('',*,*,#23131,.F.);
#31025=ORIENTED_EDGE('',*,*,#23132,.F.);
#31026=ORIENTED_EDGE('',*,*,#23133,.F.);
#31027=ORIENTED_EDGE('',*,*,#23134,.F.);
#31028=ORIENTED_EDGE('',*,*,#23135,.F.);
#31029=ORIENTED_EDGE('',*,*,#23136,.F.);
#31030=ORIENTED_EDGE('',*,*,#23137,.F.);
#31031=ORIENTED_EDGE('',*,*,#23138,.F.);
#31032=ORIENTED_EDGE('',*,*,#23139,.F.);
#31033=ORIENTED_EDGE('',*,*,#23140,.F.);
#31034=ORIENTED_EDGE('',*,*,#23141,.F.);
#31035=ORIENTED_EDGE('',*,*,#23142,.F.);
#31036=ORIENTED_EDGE('',*,*,#23143,.F.);
#31037=ORIENTED_EDGE('',*,*,#23144,.F.);
#31038=ORIENTED_EDGE('',*,*,#23145,.F.);
#31039=ORIENTED_EDGE('',*,*,#23146,.F.);
#31040=ORIENTED_EDGE('',*,*,#23147,.F.);
#31041=ORIENTED_EDGE('',*,*,#23148,.F.);
#31042=ORIENTED_EDGE('',*,*,#23149,.F.);
#31043=ORIENTED_EDGE('',*,*,#23150,.F.);
#31044=ORIENTED_EDGE('',*,*,#23151,.F.);
#31045=ORIENTED_EDGE('',*,*,#23152,.F.);
#31046=ORIENTED_EDGE('',*,*,#23153,.F.);
#31047=ORIENTED_EDGE('',*,*,#23154,.F.);
#31048=ORIENTED_EDGE('',*,*,#23155,.F.);
#31049=ORIENTED_EDGE('',*,*,#23156,.F.);
#31050=ORIENTED_EDGE('',*,*,#23157,.F.);
#31051=ORIENTED_EDGE('',*,*,#23158,.F.);
#31052=ORIENTED_EDGE('',*,*,#23159,.F.);
#31053=ORIENTED_EDGE('',*,*,#23160,.F.);
#31054=ORIENTED_EDGE('',*,*,#23161,.F.);
#31055=ORIENTED_EDGE('',*,*,#23162,.F.);
#31056=ORIENTED_EDGE('',*,*,#23163,.F.);
#31057=ORIENTED_EDGE('',*,*,#23164,.F.);
#31058=ORIENTED_EDGE('',*,*,#23165,.F.);
#31059=ORIENTED_EDGE('',*,*,#23166,.F.);
#31060=ORIENTED_EDGE('',*,*,#23167,.F.);
#31061=ORIENTED_EDGE('',*,*,#23168,.F.);
#31062=ORIENTED_EDGE('',*,*,#23169,.F.);
#31063=ORIENTED_EDGE('',*,*,#23170,.F.);
#31064=ORIENTED_EDGE('',*,*,#23171,.F.);
#31065=ORIENTED_EDGE('',*,*,#23172,.F.);
#31066=ORIENTED_EDGE('',*,*,#23173,.F.);
#31067=ORIENTED_EDGE('',*,*,#23174,.F.);
#31068=ORIENTED_EDGE('',*,*,#23175,.F.);
#31069=ORIENTED_EDGE('',*,*,#23176,.F.);
#31070=ORIENTED_EDGE('',*,*,#23177,.F.);
#31071=ORIENTED_EDGE('',*,*,#23178,.F.);
#31072=ORIENTED_EDGE('',*,*,#23179,.F.);
#31073=ORIENTED_EDGE('',*,*,#23180,.F.);
#31074=ORIENTED_EDGE('',*,*,#23181,.F.);
#31075=ORIENTED_EDGE('',*,*,#23182,.F.);
#31076=ORIENTED_EDGE('',*,*,#23183,.F.);
#31077=ORIENTED_EDGE('',*,*,#23184,.F.);
#31078=ORIENTED_EDGE('',*,*,#23185,.F.);
#31079=ORIENTED_EDGE('',*,*,#23186,.F.);
#31080=ORIENTED_EDGE('',*,*,#23187,.F.);
#31081=ORIENTED_EDGE('',*,*,#23188,.F.);
#31082=ORIENTED_EDGE('',*,*,#23189,.F.);
#31083=ORIENTED_EDGE('',*,*,#23190,.F.);
#31084=ORIENTED_EDGE('',*,*,#23191,.F.);
#31085=ORIENTED_EDGE('',*,*,#23192,.F.);
#31086=ORIENTED_EDGE('',*,*,#23193,.F.);
#31087=ORIENTED_EDGE('',*,*,#23194,.F.);
#31088=ORIENTED_EDGE('',*,*,#23195,.F.);
#31089=ORIENTED_EDGE('',*,*,#23196,.F.);
#31090=ORIENTED_EDGE('',*,*,#23197,.F.);
#31091=ORIENTED_EDGE('',*,*,#23198,.F.);
#31092=ORIENTED_EDGE('',*,*,#23199,.F.);
#31093=ORIENTED_EDGE('',*,*,#23200,.F.);
#31094=ORIENTED_EDGE('',*,*,#23201,.F.);
#31095=ORIENTED_EDGE('',*,*,#23202,.F.);
#31096=ORIENTED_EDGE('',*,*,#23203,.F.);
#31097=ORIENTED_EDGE('',*,*,#23204,.F.);
#31098=ORIENTED_EDGE('',*,*,#23205,.F.);
#31099=ORIENTED_EDGE('',*,*,#23206,.F.);
#31100=ORIENTED_EDGE('',*,*,#23207,.F.);
#31101=ORIENTED_EDGE('',*,*,#23208,.F.);
#31102=ORIENTED_EDGE('',*,*,#23209,.F.);
#31103=ORIENTED_EDGE('',*,*,#23210,.F.);
#31104=ORIENTED_EDGE('',*,*,#23211,.F.);
#31105=ORIENTED_EDGE('',*,*,#23212,.F.);
#31106=ORIENTED_EDGE('',*,*,#23213,.F.);
#31107=ORIENTED_EDGE('',*,*,#23214,.F.);
#31108=ORIENTED_EDGE('',*,*,#23215,.F.);
#31109=ORIENTED_EDGE('',*,*,#23216,.F.);
#31110=ORIENTED_EDGE('',*,*,#23217,.F.);
#31111=ORIENTED_EDGE('',*,*,#23218,.F.);
#31112=ORIENTED_EDGE('',*,*,#23219,.F.);
#31113=ORIENTED_EDGE('',*,*,#23220,.F.);
#31114=ORIENTED_EDGE('',*,*,#23221,.F.);
#31115=ORIENTED_EDGE('',*,*,#23222,.F.);
#31116=ORIENTED_EDGE('',*,*,#23223,.F.);
#31117=ORIENTED_EDGE('',*,*,#23224,.F.);
#31118=ORIENTED_EDGE('',*,*,#23225,.F.);
#31119=ORIENTED_EDGE('',*,*,#23226,.F.);
#31120=ORIENTED_EDGE('',*,*,#23227,.F.);
#31121=ORIENTED_EDGE('',*,*,#23228,.F.);
#31122=ORIENTED_EDGE('',*,*,#23229,.F.);
#31123=ORIENTED_EDGE('',*,*,#23230,.F.);
#31124=ORIENTED_EDGE('',*,*,#23231,.F.);
#31125=ORIENTED_EDGE('',*,*,#23232,.F.);
#31126=ORIENTED_EDGE('',*,*,#23233,.F.);
#31127=ORIENTED_EDGE('',*,*,#23234,.F.);
#31128=ORIENTED_EDGE('',*,*,#23235,.F.);
#31129=ORIENTED_EDGE('',*,*,#23236,.F.);
#31130=ORIENTED_EDGE('',*,*,#23237,.F.);
#31131=ORIENTED_EDGE('',*,*,#23238,.F.);
#31132=ORIENTED_EDGE('',*,*,#23239,.F.);
#31133=ORIENTED_EDGE('',*,*,#23240,.F.);
#31134=ORIENTED_EDGE('',*,*,#23241,.F.);
#31135=ORIENTED_EDGE('',*,*,#23242,.F.);
#31136=ORIENTED_EDGE('',*,*,#23243,.F.);
#31137=ORIENTED_EDGE('',*,*,#23244,.F.);
#31138=ORIENTED_EDGE('',*,*,#23245,.F.);
#31139=ORIENTED_EDGE('',*,*,#23246,.F.);
#31140=ORIENTED_EDGE('',*,*,#23247,.F.);
#31141=ORIENTED_EDGE('',*,*,#23248,.F.);
#31142=ORIENTED_EDGE('',*,*,#23249,.F.);
#31143=ORIENTED_EDGE('',*,*,#23250,.F.);
#31144=ORIENTED_EDGE('',*,*,#23251,.F.);
#31145=ORIENTED_EDGE('',*,*,#23252,.F.);
#31146=ORIENTED_EDGE('',*,*,#23253,.F.);
#31147=ORIENTED_EDGE('',*,*,#23254,.F.);
#31148=ORIENTED_EDGE('',*,*,#23255,.F.);
#31149=ORIENTED_EDGE('',*,*,#23256,.F.);
#31150=ORIENTED_EDGE('',*,*,#23257,.F.);
#31151=ORIENTED_EDGE('',*,*,#23258,.F.);
#31152=ORIENTED_EDGE('',*,*,#23259,.F.);
#31153=ORIENTED_EDGE('',*,*,#23260,.F.);
#31154=ORIENTED_EDGE('',*,*,#23261,.F.);
#31155=ORIENTED_EDGE('',*,*,#23262,.F.);
#31156=ORIENTED_EDGE('',*,*,#23263,.F.);
#31157=ORIENTED_EDGE('',*,*,#23264,.F.);
#31158=ORIENTED_EDGE('',*,*,#23265,.F.);
#31159=ORIENTED_EDGE('',*,*,#23266,.F.);
#31160=ORIENTED_EDGE('',*,*,#23267,.F.);
#31161=ORIENTED_EDGE('',*,*,#23268,.F.);
#31162=ORIENTED_EDGE('',*,*,#23269,.F.);
#31163=ORIENTED_EDGE('',*,*,#23270,.F.);
#31164=ORIENTED_EDGE('',*,*,#23271,.F.);
#31165=ORIENTED_EDGE('',*,*,#23272,.F.);
#31166=ORIENTED_EDGE('',*,*,#23273,.F.);
#31167=ORIENTED_EDGE('',*,*,#23274,.F.);
#31168=ORIENTED_EDGE('',*,*,#23275,.F.);
#31169=ORIENTED_EDGE('',*,*,#23276,.F.);
#31170=ORIENTED_EDGE('',*,*,#23277,.F.);
#31171=ORIENTED_EDGE('',*,*,#23278,.F.);
#31172=ORIENTED_EDGE('',*,*,#23279,.F.);
#31173=ORIENTED_EDGE('',*,*,#23280,.F.);
#31174=ORIENTED_EDGE('',*,*,#23281,.F.);
#31175=ORIENTED_EDGE('',*,*,#23282,.F.);
#31176=ORIENTED_EDGE('',*,*,#23283,.F.);
#31177=ORIENTED_EDGE('',*,*,#23284,.F.);
#31178=ORIENTED_EDGE('',*,*,#23285,.F.);
#31179=ORIENTED_EDGE('',*,*,#23286,.F.);
#31180=ORIENTED_EDGE('',*,*,#23287,.F.);
#31181=ORIENTED_EDGE('',*,*,#23288,.F.);
#31182=ORIENTED_EDGE('',*,*,#23289,.F.);
#31183=ORIENTED_EDGE('',*,*,#23290,.F.);
#31184=ORIENTED_EDGE('',*,*,#23291,.F.);
#31185=ORIENTED_EDGE('',*,*,#23292,.F.);
#31186=ORIENTED_EDGE('',*,*,#23293,.F.);
#31187=ORIENTED_EDGE('',*,*,#23294,.F.);
#31188=ORIENTED_EDGE('',*,*,#23295,.F.);
#31189=ORIENTED_EDGE('',*,*,#23296,.F.);
#31190=ORIENTED_EDGE('',*,*,#23297,.F.);
#31191=ORIENTED_EDGE('',*,*,#23298,.F.);
#31192=ORIENTED_EDGE('',*,*,#23299,.F.);
#31193=ORIENTED_EDGE('',*,*,#23300,.F.);
#31194=ORIENTED_EDGE('',*,*,#23301,.F.);
#31195=ORIENTED_EDGE('',*,*,#23302,.F.);
#31196=ORIENTED_EDGE('',*,*,#23303,.F.);
#31197=ORIENTED_EDGE('',*,*,#23304,.F.);
#31198=ORIENTED_EDGE('',*,*,#23305,.F.);
#31199=ORIENTED_EDGE('',*,*,#23306,.F.);
#31200=ORIENTED_EDGE('',*,*,#23307,.F.);
#31201=ORIENTED_EDGE('',*,*,#23308,.F.);
#31202=ORIENTED_EDGE('',*,*,#23309,.F.);
#31203=ORIENTED_EDGE('',*,*,#23310,.F.);
#31204=ORIENTED_EDGE('',*,*,#23311,.F.);
#31205=ORIENTED_EDGE('',*,*,#23312,.F.);
#31206=ORIENTED_EDGE('',*,*,#23313,.F.);
#31207=ORIENTED_EDGE('',*,*,#23314,.F.);
#31208=ORIENTED_EDGE('',*,*,#23315,.F.);
#31209=ORIENTED_EDGE('',*,*,#23316,.F.);
#31210=ORIENTED_EDGE('',*,*,#23317,.F.);
#31211=ORIENTED_EDGE('',*,*,#23318,.F.);
#31212=ORIENTED_EDGE('',*,*,#23319,.F.);
#31213=ORIENTED_EDGE('',*,*,#23320,.F.);
#31214=ORIENTED_EDGE('',*,*,#23321,.F.);
#31215=ORIENTED_EDGE('',*,*,#23322,.F.);
#31216=ORIENTED_EDGE('',*,*,#23323,.F.);
#31217=ORIENTED_EDGE('',*,*,#23324,.F.);
#31218=ORIENTED_EDGE('',*,*,#23325,.F.);
#31219=ORIENTED_EDGE('',*,*,#23326,.F.);
#31220=ORIENTED_EDGE('',*,*,#23327,.F.);
#31221=ORIENTED_EDGE('',*,*,#23328,.F.);
#31222=ORIENTED_EDGE('',*,*,#23329,.F.);
#31223=ORIENTED_EDGE('',*,*,#23330,.F.);
#31224=ORIENTED_EDGE('',*,*,#23331,.F.);
#31225=ORIENTED_EDGE('',*,*,#23332,.F.);
#31226=ORIENTED_EDGE('',*,*,#23333,.F.);
#31227=ORIENTED_EDGE('',*,*,#23334,.F.);
#31228=ORIENTED_EDGE('',*,*,#23335,.F.);
#31229=ORIENTED_EDGE('',*,*,#23336,.F.);
#31230=ORIENTED_EDGE('',*,*,#23337,.F.);
#31231=ORIENTED_EDGE('',*,*,#23338,.F.);
#31232=ORIENTED_EDGE('',*,*,#23339,.F.);
#31233=ORIENTED_EDGE('',*,*,#23340,.F.);
#31234=ORIENTED_EDGE('',*,*,#23341,.F.);
#31235=ORIENTED_EDGE('',*,*,#23342,.F.);
#31236=ORIENTED_EDGE('',*,*,#23343,.F.);
#31237=ORIENTED_EDGE('',*,*,#23344,.F.);
#31238=ORIENTED_EDGE('',*,*,#23345,.F.);
#31239=ORIENTED_EDGE('',*,*,#23346,.F.);
#31240=ORIENTED_EDGE('',*,*,#23347,.F.);
#31241=ORIENTED_EDGE('',*,*,#23348,.F.);
#31242=ORIENTED_EDGE('',*,*,#23349,.F.);
#31243=ORIENTED_EDGE('',*,*,#23350,.F.);
#31244=ORIENTED_EDGE('',*,*,#23351,.F.);
#31245=ORIENTED_EDGE('',*,*,#23352,.F.);
#31246=ORIENTED_EDGE('',*,*,#23353,.F.);
#31247=ORIENTED_EDGE('',*,*,#23354,.F.);
#31248=ORIENTED_EDGE('',*,*,#23355,.F.);
#31249=ORIENTED_EDGE('',*,*,#23356,.F.);
#31250=ORIENTED_EDGE('',*,*,#23357,.F.);
#31251=ORIENTED_EDGE('',*,*,#23358,.F.);
#31252=ORIENTED_EDGE('',*,*,#23359,.F.);
#31253=ORIENTED_EDGE('',*,*,#23360,.F.);
#31254=ORIENTED_EDGE('',*,*,#23361,.F.);
#31255=ORIENTED_EDGE('',*,*,#23362,.F.);
#31256=ORIENTED_EDGE('',*,*,#23363,.F.);
#31257=ORIENTED_EDGE('',*,*,#23364,.F.);
#31258=ORIENTED_EDGE('',*,*,#23365,.F.);
#31259=ORIENTED_EDGE('',*,*,#23366,.F.);
#31260=ORIENTED_EDGE('',*,*,#23367,.F.);
#31261=ORIENTED_EDGE('',*,*,#23368,.F.);
#31262=ORIENTED_EDGE('',*,*,#23369,.F.);
#31263=ORIENTED_EDGE('',*,*,#23370,.F.);
#31264=ORIENTED_EDGE('',*,*,#23371,.F.);
#31265=ORIENTED_EDGE('',*,*,#23372,.F.);
#31266=ORIENTED_EDGE('',*,*,#23373,.F.);
#31267=ORIENTED_EDGE('',*,*,#23374,.F.);
#31268=ORIENTED_EDGE('',*,*,#23375,.F.);
#31269=ORIENTED_EDGE('',*,*,#23376,.F.);
#31270=ORIENTED_EDGE('',*,*,#23377,.F.);
#31271=ORIENTED_EDGE('',*,*,#23378,.F.);
#31272=ORIENTED_EDGE('',*,*,#23379,.F.);
#31273=ORIENTED_EDGE('',*,*,#23380,.F.);
#31274=ORIENTED_EDGE('',*,*,#23381,.F.);
#31275=ORIENTED_EDGE('',*,*,#23382,.F.);
#31276=ORIENTED_EDGE('',*,*,#23383,.F.);
#31277=ORIENTED_EDGE('',*,*,#23384,.F.);
#31278=ORIENTED_EDGE('',*,*,#23385,.F.);
#31279=ORIENTED_EDGE('',*,*,#23386,.F.);
#31280=ORIENTED_EDGE('',*,*,#23387,.F.);
#31281=ORIENTED_EDGE('',*,*,#23388,.F.);
#31282=ORIENTED_EDGE('',*,*,#23389,.F.);
#31283=ORIENTED_EDGE('',*,*,#23390,.F.);
#31284=ORIENTED_EDGE('',*,*,#23391,.F.);
#31285=ORIENTED_EDGE('',*,*,#23392,.F.);
#31286=ORIENTED_EDGE('',*,*,#23393,.F.);
#31287=ORIENTED_EDGE('',*,*,#23394,.F.);
#31288=ORIENTED_EDGE('',*,*,#23395,.F.);
#31289=ORIENTED_EDGE('',*,*,#23396,.F.);
#31290=ORIENTED_EDGE('',*,*,#23397,.F.);
#31291=ORIENTED_EDGE('',*,*,#23398,.F.);
#31292=ORIENTED_EDGE('',*,*,#23399,.F.);
#31293=ORIENTED_EDGE('',*,*,#23400,.F.);
#31294=ORIENTED_EDGE('',*,*,#23401,.F.);
#31295=ORIENTED_EDGE('',*,*,#23402,.F.);
#31296=ORIENTED_EDGE('',*,*,#23403,.F.);
#31297=ORIENTED_EDGE('',*,*,#23404,.F.);
#31298=ORIENTED_EDGE('',*,*,#23405,.F.);
#31299=ORIENTED_EDGE('',*,*,#23406,.F.);
#31300=ORIENTED_EDGE('',*,*,#23407,.F.);
#31301=ORIENTED_EDGE('',*,*,#23408,.F.);
#31302=ORIENTED_EDGE('',*,*,#23409,.F.);
#31303=ORIENTED_EDGE('',*,*,#23410,.F.);
#31304=ORIENTED_EDGE('',*,*,#23411,.F.);
#31305=ORIENTED_EDGE('',*,*,#23412,.F.);
#31306=ORIENTED_EDGE('',*,*,#23413,.F.);
#31307=ORIENTED_EDGE('',*,*,#23414,.F.);
#31308=ORIENTED_EDGE('',*,*,#23415,.F.);
#31309=ORIENTED_EDGE('',*,*,#23416,.F.);
#31310=ORIENTED_EDGE('',*,*,#23417,.F.);
#31311=ORIENTED_EDGE('',*,*,#23418,.F.);
#31312=ORIENTED_EDGE('',*,*,#23419,.F.);
#31313=ORIENTED_EDGE('',*,*,#23420,.F.);
#31314=ORIENTED_EDGE('',*,*,#23421,.F.);
#31315=ORIENTED_EDGE('',*,*,#23422,.F.);
#31316=ORIENTED_EDGE('',*,*,#23423,.F.);
#31317=ORIENTED_EDGE('',*,*,#23424,.F.);
#31318=ORIENTED_EDGE('',*,*,#23425,.F.);
#31319=ORIENTED_EDGE('',*,*,#23426,.F.);
#31320=ORIENTED_EDGE('',*,*,#23427,.F.);
#31321=ORIENTED_EDGE('',*,*,#23428,.F.);
#31322=ORIENTED_EDGE('',*,*,#23429,.F.);
#31323=ORIENTED_EDGE('',*,*,#23430,.F.);
#31324=ORIENTED_EDGE('',*,*,#23431,.F.);
#31325=ORIENTED_EDGE('',*,*,#23432,.F.);
#31326=ORIENTED_EDGE('',*,*,#23433,.F.);
#31327=ORIENTED_EDGE('',*,*,#23434,.F.);
#31328=ORIENTED_EDGE('',*,*,#23435,.F.);
#31329=ORIENTED_EDGE('',*,*,#23436,.F.);
#31330=ORIENTED_EDGE('',*,*,#23437,.F.);
#31331=ORIENTED_EDGE('',*,*,#23438,.F.);
#31332=ORIENTED_EDGE('',*,*,#23439,.F.);
#31333=ORIENTED_EDGE('',*,*,#23440,.F.);
#31334=ORIENTED_EDGE('',*,*,#23441,.F.);
#31335=ORIENTED_EDGE('',*,*,#23442,.F.);
#31336=ORIENTED_EDGE('',*,*,#23443,.F.);
#31337=ORIENTED_EDGE('',*,*,#23444,.F.);
#31338=ORIENTED_EDGE('',*,*,#23445,.F.);
#31339=ORIENTED_EDGE('',*,*,#23446,.F.);
#31340=ORIENTED_EDGE('',*,*,#23447,.F.);
#31341=ORIENTED_EDGE('',*,*,#23448,.F.);
#31342=ORIENTED_EDGE('',*,*,#23449,.F.);
#31343=ORIENTED_EDGE('',*,*,#23450,.F.);
#31344=ORIENTED_EDGE('',*,*,#23451,.F.);
#31345=ORIENTED_EDGE('',*,*,#23452,.F.);
#31346=ORIENTED_EDGE('',*,*,#23453,.F.);
#31347=ORIENTED_EDGE('',*,*,#23454,.F.);
#31348=ORIENTED_EDGE('',*,*,#23455,.F.);
#31349=ORIENTED_EDGE('',*,*,#23456,.F.);
#31350=ORIENTED_EDGE('',*,*,#23457,.F.);
#31351=ORIENTED_EDGE('',*,*,#23458,.F.);
#31352=ORIENTED_EDGE('',*,*,#23459,.F.);
#31353=ORIENTED_EDGE('',*,*,#23460,.F.);
#31354=ORIENTED_EDGE('',*,*,#23461,.F.);
#31355=ORIENTED_EDGE('',*,*,#23462,.F.);
#31356=ORIENTED_EDGE('',*,*,#23463,.F.);
#31357=ORIENTED_EDGE('',*,*,#23464,.F.);
#31358=ORIENTED_EDGE('',*,*,#23465,.F.);
#31359=ORIENTED_EDGE('',*,*,#23466,.F.);
#31360=ORIENTED_EDGE('',*,*,#23467,.F.);
#31361=ORIENTED_EDGE('',*,*,#23468,.F.);
#31362=ORIENTED_EDGE('',*,*,#23469,.F.);
#31363=ORIENTED_EDGE('',*,*,#23470,.F.);
#31364=ORIENTED_EDGE('',*,*,#23471,.F.);
#31365=ORIENTED_EDGE('',*,*,#23472,.F.);
#31366=ORIENTED_EDGE('',*,*,#23473,.F.);
#31367=ORIENTED_EDGE('',*,*,#23474,.F.);
#31368=ORIENTED_EDGE('',*,*,#23475,.F.);
#31369=ORIENTED_EDGE('',*,*,#23476,.F.);
#31370=ORIENTED_EDGE('',*,*,#23477,.F.);
#31371=ORIENTED_EDGE('',*,*,#23478,.F.);
#31372=ORIENTED_EDGE('',*,*,#23479,.F.);
#31373=ORIENTED_EDGE('',*,*,#23480,.F.);
#31374=ORIENTED_EDGE('',*,*,#23481,.F.);
#31375=ORIENTED_EDGE('',*,*,#23482,.F.);
#31376=ORIENTED_EDGE('',*,*,#23483,.F.);
#31377=ORIENTED_EDGE('',*,*,#23484,.F.);
#31378=ORIENTED_EDGE('',*,*,#23485,.F.);
#31379=ORIENTED_EDGE('',*,*,#23486,.F.);
#31380=ORIENTED_EDGE('',*,*,#23487,.F.);
#31381=ORIENTED_EDGE('',*,*,#23488,.F.);
#31382=ORIENTED_EDGE('',*,*,#23489,.F.);
#31383=ORIENTED_EDGE('',*,*,#23490,.F.);
#31384=ORIENTED_EDGE('',*,*,#23491,.F.);
#31385=ORIENTED_EDGE('',*,*,#23492,.F.);
#31386=ORIENTED_EDGE('',*,*,#23493,.F.);
#31387=ORIENTED_EDGE('',*,*,#23494,.F.);
#31388=ORIENTED_EDGE('',*,*,#23495,.F.);
#31389=ORIENTED_EDGE('',*,*,#23496,.F.);
#31390=ORIENTED_EDGE('',*,*,#23497,.F.);
#31391=ORIENTED_EDGE('',*,*,#23498,.F.);
#31392=ORIENTED_EDGE('',*,*,#23499,.F.);
#31393=ORIENTED_EDGE('',*,*,#23500,.F.);
#31394=ORIENTED_EDGE('',*,*,#23501,.F.);
#31395=ORIENTED_EDGE('',*,*,#23502,.F.);
#31396=ORIENTED_EDGE('',*,*,#23503,.F.);
#31397=ORIENTED_EDGE('',*,*,#23504,.F.);
#31398=ORIENTED_EDGE('',*,*,#23505,.F.);
#31399=ORIENTED_EDGE('',*,*,#23506,.F.);
#31400=ORIENTED_EDGE('',*,*,#23507,.F.);
#31401=ORIENTED_EDGE('',*,*,#23508,.F.);
#31402=ORIENTED_EDGE('',*,*,#23509,.F.);
#31403=ORIENTED_EDGE('',*,*,#23510,.F.);
#31404=ORIENTED_EDGE('',*,*,#23511,.F.);
#31405=ORIENTED_EDGE('',*,*,#23512,.F.);
#31406=ORIENTED_EDGE('',*,*,#23513,.F.);
#31407=ORIENTED_EDGE('',*,*,#23514,.F.);
#31408=ORIENTED_EDGE('',*,*,#23515,.F.);
#31409=ORIENTED_EDGE('',*,*,#23516,.F.);
#31410=ORIENTED_EDGE('',*,*,#23517,.F.);
#31411=ORIENTED_EDGE('',*,*,#23518,.F.);
#31412=ORIENTED_EDGE('',*,*,#23519,.F.);
#31413=ORIENTED_EDGE('',*,*,#23520,.F.);
#31414=ORIENTED_EDGE('',*,*,#23521,.F.);
#31415=ORIENTED_EDGE('',*,*,#23522,.F.);
#31416=ORIENTED_EDGE('',*,*,#23523,.F.);
#31417=ORIENTED_EDGE('',*,*,#23524,.F.);
#31418=ORIENTED_EDGE('',*,*,#23525,.F.);
#31419=ORIENTED_EDGE('',*,*,#23526,.F.);
#31420=ORIENTED_EDGE('',*,*,#23527,.F.);
#31421=ORIENTED_EDGE('',*,*,#23528,.F.);
#31422=ORIENTED_EDGE('',*,*,#23529,.F.);
#31423=ORIENTED_EDGE('',*,*,#23530,.F.);
#31424=ORIENTED_EDGE('',*,*,#23531,.F.);
#31425=ORIENTED_EDGE('',*,*,#23532,.F.);
#31426=ORIENTED_EDGE('',*,*,#23533,.F.);
#31427=ORIENTED_EDGE('',*,*,#23534,.F.);
#31428=ORIENTED_EDGE('',*,*,#23535,.F.);
#31429=ORIENTED_EDGE('',*,*,#23536,.F.);
#31430=ORIENTED_EDGE('',*,*,#23537,.F.);
#31431=ORIENTED_EDGE('',*,*,#23538,.F.);
#31432=ORIENTED_EDGE('',*,*,#23539,.F.);
#31433=ORIENTED_EDGE('',*,*,#23540,.F.);
#31434=ORIENTED_EDGE('',*,*,#23541,.F.);
#31435=ORIENTED_EDGE('',*,*,#23542,.F.);
#31436=ORIENTED_EDGE('',*,*,#23543,.F.);
#31437=ORIENTED_EDGE('',*,*,#23544,.F.);
#31438=ORIENTED_EDGE('',*,*,#23545,.F.);
#31439=ORIENTED_EDGE('',*,*,#23546,.F.);
#31440=ORIENTED_EDGE('',*,*,#23547,.F.);
#31441=ORIENTED_EDGE('',*,*,#23548,.F.);
#31442=ORIENTED_EDGE('',*,*,#23549,.F.);
#31443=ORIENTED_EDGE('',*,*,#23550,.F.);
#31444=ORIENTED_EDGE('',*,*,#23551,.F.);
#31445=ORIENTED_EDGE('',*,*,#23552,.F.);
#31446=ORIENTED_EDGE('',*,*,#23553,.F.);
#31447=ORIENTED_EDGE('',*,*,#23554,.F.);
#31448=ORIENTED_EDGE('',*,*,#23555,.F.);
#31449=ORIENTED_EDGE('',*,*,#23556,.F.);
#31450=ORIENTED_EDGE('',*,*,#23557,.F.);
#31451=ORIENTED_EDGE('',*,*,#23558,.F.);
#31452=ORIENTED_EDGE('',*,*,#23559,.F.);
#31453=ORIENTED_EDGE('',*,*,#23560,.F.);
#31454=ORIENTED_EDGE('',*,*,#23561,.F.);
#31455=ORIENTED_EDGE('',*,*,#23562,.F.);
#31456=ORIENTED_EDGE('',*,*,#23563,.F.);
#31457=ORIENTED_EDGE('',*,*,#23564,.F.);
#31458=ORIENTED_EDGE('',*,*,#23565,.F.);
#31459=ORIENTED_EDGE('',*,*,#23566,.F.);
#31460=ORIENTED_EDGE('',*,*,#23567,.F.);
#31461=ORIENTED_EDGE('',*,*,#23568,.F.);
#31462=ORIENTED_EDGE('',*,*,#23569,.F.);
#31463=ORIENTED_EDGE('',*,*,#23570,.F.);
#31464=ORIENTED_EDGE('',*,*,#23571,.F.);
#31465=ORIENTED_EDGE('',*,*,#23572,.F.);
#31466=ORIENTED_EDGE('',*,*,#23573,.F.);
#31467=ORIENTED_EDGE('',*,*,#23574,.F.);
#31468=ORIENTED_EDGE('',*,*,#23575,.F.);
#31469=ORIENTED_EDGE('',*,*,#23576,.F.);
#31470=ORIENTED_EDGE('',*,*,#23577,.F.);
#31471=ORIENTED_EDGE('',*,*,#23578,.F.);
#31472=ORIENTED_EDGE('',*,*,#23579,.F.);
#31473=ORIENTED_EDGE('',*,*,#23580,.F.);
#31474=ORIENTED_EDGE('',*,*,#23581,.F.);
#31475=ORIENTED_EDGE('',*,*,#23582,.F.);
#31476=ORIENTED_EDGE('',*,*,#23583,.F.);
#31477=ORIENTED_EDGE('',*,*,#23584,.F.);
#31478=ORIENTED_EDGE('',*,*,#23585,.F.);
#31479=ORIENTED_EDGE('',*,*,#23586,.F.);
#31480=ORIENTED_EDGE('',*,*,#23587,.F.);
#31481=ORIENTED_EDGE('',*,*,#23588,.F.);
#31482=ORIENTED_EDGE('',*,*,#23589,.F.);
#31483=ORIENTED_EDGE('',*,*,#23590,.F.);
#31484=ORIENTED_EDGE('',*,*,#23591,.F.);
#31485=ORIENTED_EDGE('',*,*,#23592,.F.);
#31486=ORIENTED_EDGE('',*,*,#23593,.F.);
#31487=ORIENTED_EDGE('',*,*,#23594,.F.);
#31488=ORIENTED_EDGE('',*,*,#23595,.F.);
#31489=ORIENTED_EDGE('',*,*,#23596,.F.);
#31490=ORIENTED_EDGE('',*,*,#23597,.F.);
#31491=ORIENTED_EDGE('',*,*,#23598,.F.);
#31492=ORIENTED_EDGE('',*,*,#23599,.F.);
#31493=ORIENTED_EDGE('',*,*,#23600,.F.);
#31494=ORIENTED_EDGE('',*,*,#23601,.F.);
#31495=ORIENTED_EDGE('',*,*,#23602,.F.);
#31496=ORIENTED_EDGE('',*,*,#23603,.F.);
#31497=ORIENTED_EDGE('',*,*,#23604,.F.);
#31498=ORIENTED_EDGE('',*,*,#23605,.F.);
#31499=ORIENTED_EDGE('',*,*,#23606,.F.);
#31500=ORIENTED_EDGE('',*,*,#23607,.F.);
#31501=ORIENTED_EDGE('',*,*,#23608,.F.);
#31502=ORIENTED_EDGE('',*,*,#23609,.F.);
#31503=ORIENTED_EDGE('',*,*,#23610,.F.);
#31504=ORIENTED_EDGE('',*,*,#23611,.F.);
#31505=ORIENTED_EDGE('',*,*,#23612,.F.);
#31506=ORIENTED_EDGE('',*,*,#23613,.F.);
#31507=ORIENTED_EDGE('',*,*,#23614,.F.);
#31508=ORIENTED_EDGE('',*,*,#23615,.F.);
#31509=ORIENTED_EDGE('',*,*,#23616,.F.);
#31510=ORIENTED_EDGE('',*,*,#23617,.F.);
#31511=ORIENTED_EDGE('',*,*,#23618,.F.);
#31512=ORIENTED_EDGE('',*,*,#23619,.F.);
#31513=ORIENTED_EDGE('',*,*,#23620,.F.);
#31514=ORIENTED_EDGE('',*,*,#23621,.F.);
#31515=ORIENTED_EDGE('',*,*,#23622,.F.);
#31516=ORIENTED_EDGE('',*,*,#23623,.F.);
#31517=ORIENTED_EDGE('',*,*,#23624,.F.);
#31518=ORIENTED_EDGE('',*,*,#23625,.F.);
#31519=ORIENTED_EDGE('',*,*,#23626,.F.);
#31520=ORIENTED_EDGE('',*,*,#23627,.F.);
#31521=ORIENTED_EDGE('',*,*,#23628,.F.);
#31522=ORIENTED_EDGE('',*,*,#23629,.F.);
#31523=ORIENTED_EDGE('',*,*,#23630,.F.);
#31524=ORIENTED_EDGE('',*,*,#23631,.F.);
#31525=ORIENTED_EDGE('',*,*,#23632,.F.);
#31526=ORIENTED_EDGE('',*,*,#23633,.F.);
#31527=ORIENTED_EDGE('',*,*,#23634,.F.);
#31528=ORIENTED_EDGE('',*,*,#23635,.F.);
#31529=ORIENTED_EDGE('',*,*,#23636,.F.);
#31530=ORIENTED_EDGE('',*,*,#23637,.F.);
#31531=ORIENTED_EDGE('',*,*,#23638,.F.);
#31532=ORIENTED_EDGE('',*,*,#23639,.F.);
#31533=ORIENTED_EDGE('',*,*,#23640,.F.);
#31534=ORIENTED_EDGE('',*,*,#23641,.F.);
#31535=ORIENTED_EDGE('',*,*,#23642,.F.);
#31536=ORIENTED_EDGE('',*,*,#23643,.F.);
#31537=ORIENTED_EDGE('',*,*,#23644,.F.);
#31538=ORIENTED_EDGE('',*,*,#23645,.F.);
#31539=ORIENTED_EDGE('',*,*,#23646,.F.);
#31540=ORIENTED_EDGE('',*,*,#23647,.F.);
#31541=ORIENTED_EDGE('',*,*,#23648,.F.);
#31542=ORIENTED_EDGE('',*,*,#23649,.F.);
#31543=ORIENTED_EDGE('',*,*,#23650,.F.);
#31544=ORIENTED_EDGE('',*,*,#23651,.F.);
#31545=ORIENTED_EDGE('',*,*,#23652,.F.);
#31546=ORIENTED_EDGE('',*,*,#23653,.F.);
#31547=ORIENTED_EDGE('',*,*,#23654,.F.);
#31548=ORIENTED_EDGE('',*,*,#23655,.F.);
#31549=ORIENTED_EDGE('',*,*,#23656,.F.);
#31550=ORIENTED_EDGE('',*,*,#23657,.F.);
#31551=ORIENTED_EDGE('',*,*,#23658,.F.);
#31552=ORIENTED_EDGE('',*,*,#23659,.F.);
#31553=ORIENTED_EDGE('',*,*,#23660,.F.);
#31554=ORIENTED_EDGE('',*,*,#23661,.F.);
#31555=ORIENTED_EDGE('',*,*,#23662,.F.);
#31556=ORIENTED_EDGE('',*,*,#23663,.F.);
#31557=ORIENTED_EDGE('',*,*,#23664,.F.);
#31558=ORIENTED_EDGE('',*,*,#23665,.F.);
#31559=ORIENTED_EDGE('',*,*,#23666,.F.);
#31560=ORIENTED_EDGE('',*,*,#23667,.F.);
#31561=ORIENTED_EDGE('',*,*,#23668,.F.);
#31562=ORIENTED_EDGE('',*,*,#23669,.F.);
#31563=ORIENTED_EDGE('',*,*,#23670,.F.);
#31564=ORIENTED_EDGE('',*,*,#23671,.F.);
#31565=ORIENTED_EDGE('',*,*,#23672,.F.);
#31566=ORIENTED_EDGE('',*,*,#23673,.F.);
#31567=ORIENTED_EDGE('',*,*,#23674,.F.);
#31568=ORIENTED_EDGE('',*,*,#23675,.F.);
#31569=ORIENTED_EDGE('',*,*,#23676,.F.);
#31570=ORIENTED_EDGE('',*,*,#23677,.F.);
#31571=ORIENTED_EDGE('',*,*,#23678,.F.);
#31572=ORIENTED_EDGE('',*,*,#23679,.F.);
#31573=ORIENTED_EDGE('',*,*,#23680,.F.);
#31574=ORIENTED_EDGE('',*,*,#23681,.F.);
#31575=ORIENTED_EDGE('',*,*,#23682,.F.);
#31576=ORIENTED_EDGE('',*,*,#23683,.F.);
#31577=ORIENTED_EDGE('',*,*,#23684,.F.);
#31578=ORIENTED_EDGE('',*,*,#23685,.F.);
#31579=ORIENTED_EDGE('',*,*,#23686,.F.);
#31580=ORIENTED_EDGE('',*,*,#23687,.F.);
#31581=ORIENTED_EDGE('',*,*,#23688,.F.);
#31582=ORIENTED_EDGE('',*,*,#23689,.F.);
#31583=ORIENTED_EDGE('',*,*,#23690,.F.);
#31584=ORIENTED_EDGE('',*,*,#23691,.F.);
#31585=ORIENTED_EDGE('',*,*,#23692,.F.);
#31586=ORIENTED_EDGE('',*,*,#23693,.F.);
#31587=ORIENTED_EDGE('',*,*,#23694,.F.);
#31588=ORIENTED_EDGE('',*,*,#23695,.F.);
#31589=ORIENTED_EDGE('',*,*,#23696,.F.);
#31590=ORIENTED_EDGE('',*,*,#23697,.F.);
#31591=ORIENTED_EDGE('',*,*,#23698,.F.);
#31592=ORIENTED_EDGE('',*,*,#23699,.F.);
#31593=ORIENTED_EDGE('',*,*,#23700,.F.);
#31594=ORIENTED_EDGE('',*,*,#23701,.F.);
#31595=ORIENTED_EDGE('',*,*,#23702,.F.);
#31596=ORIENTED_EDGE('',*,*,#23703,.F.);
#31597=ORIENTED_EDGE('',*,*,#23704,.F.);
#31598=ORIENTED_EDGE('',*,*,#23705,.F.);
#31599=ORIENTED_EDGE('',*,*,#23706,.F.);
#31600=ORIENTED_EDGE('',*,*,#23707,.F.);
#31601=ORIENTED_EDGE('',*,*,#23708,.F.);
#31602=ORIENTED_EDGE('',*,*,#23709,.F.);
#31603=ORIENTED_EDGE('',*,*,#23710,.F.);
#31604=ORIENTED_EDGE('',*,*,#23711,.F.);
#31605=ORIENTED_EDGE('',*,*,#23712,.F.);
#31606=ORIENTED_EDGE('',*,*,#23713,.F.);
#31607=ORIENTED_EDGE('',*,*,#23714,.F.);
#31608=ORIENTED_EDGE('',*,*,#23715,.F.);
#31609=ORIENTED_EDGE('',*,*,#23716,.F.);
#31610=ORIENTED_EDGE('',*,*,#23717,.F.);
#31611=ORIENTED_EDGE('',*,*,#23718,.F.);
#31612=ORIENTED_EDGE('',*,*,#23719,.F.);
#31613=ORIENTED_EDGE('',*,*,#23720,.F.);
#31614=ORIENTED_EDGE('',*,*,#23721,.F.);
#31615=ORIENTED_EDGE('',*,*,#23722,.F.);
#31616=ORIENTED_EDGE('',*,*,#23723,.F.);
#31617=ORIENTED_EDGE('',*,*,#23724,.F.);
#31618=ORIENTED_EDGE('',*,*,#23725,.F.);
#31619=ORIENTED_EDGE('',*,*,#23726,.F.);
#31620=ORIENTED_EDGE('',*,*,#23727,.F.);
#31621=ORIENTED_EDGE('',*,*,#23728,.F.);
#31622=ORIENTED_EDGE('',*,*,#23729,.F.);
#31623=ORIENTED_EDGE('',*,*,#23730,.F.);
#31624=ORIENTED_EDGE('',*,*,#23731,.F.);
#31625=ORIENTED_EDGE('',*,*,#23732,.F.);
#31626=ORIENTED_EDGE('',*,*,#23733,.F.);
#31627=ORIENTED_EDGE('',*,*,#23734,.F.);
#31628=ORIENTED_EDGE('',*,*,#23735,.F.);
#31629=ORIENTED_EDGE('',*,*,#23736,.F.);
#31630=ORIENTED_EDGE('',*,*,#23737,.F.);
#31631=ORIENTED_EDGE('',*,*,#23738,.F.);
#31632=ORIENTED_EDGE('',*,*,#23739,.F.);
#31633=ORIENTED_EDGE('',*,*,#23740,.F.);
#31634=ORIENTED_EDGE('',*,*,#23741,.F.);
#31635=ORIENTED_EDGE('',*,*,#23742,.F.);
#31636=ORIENTED_EDGE('',*,*,#23743,.F.);
#31637=ORIENTED_EDGE('',*,*,#23744,.F.);
#31638=ORIENTED_EDGE('',*,*,#23745,.F.);
#31639=ORIENTED_EDGE('',*,*,#23746,.F.);
#31640=ORIENTED_EDGE('',*,*,#23747,.F.);
#31641=ORIENTED_EDGE('',*,*,#23748,.F.);
#31642=ORIENTED_EDGE('',*,*,#23749,.F.);
#31643=ORIENTED_EDGE('',*,*,#23750,.F.);
#31644=ORIENTED_EDGE('',*,*,#23751,.F.);
#31645=ORIENTED_EDGE('',*,*,#23752,.F.);
#31646=ORIENTED_EDGE('',*,*,#23753,.F.);
#31647=ORIENTED_EDGE('',*,*,#23754,.F.);
#31648=ORIENTED_EDGE('',*,*,#23755,.F.);
#31649=ORIENTED_EDGE('',*,*,#23756,.F.);
#31650=ORIENTED_EDGE('',*,*,#23757,.F.);
#31651=ORIENTED_EDGE('',*,*,#23758,.F.);
#31652=ORIENTED_EDGE('',*,*,#23759,.F.);
#31653=ORIENTED_EDGE('',*,*,#23760,.F.);
#31654=ORIENTED_EDGE('',*,*,#23761,.F.);
#31655=ORIENTED_EDGE('',*,*,#23762,.F.);
#31656=ORIENTED_EDGE('',*,*,#23763,.F.);
#31657=ORIENTED_EDGE('',*,*,#23764,.F.);
#31658=ORIENTED_EDGE('',*,*,#23765,.F.);
#31659=ORIENTED_EDGE('',*,*,#23766,.F.);
#31660=ORIENTED_EDGE('',*,*,#23767,.F.);
#31661=ORIENTED_EDGE('',*,*,#23768,.F.);
#31662=ORIENTED_EDGE('',*,*,#23769,.F.);
#31663=ORIENTED_EDGE('',*,*,#23770,.F.);
#31664=ORIENTED_EDGE('',*,*,#23771,.F.);
#31665=ORIENTED_EDGE('',*,*,#23772,.F.);
#31666=ORIENTED_EDGE('',*,*,#23773,.F.);
#31667=ORIENTED_EDGE('',*,*,#23774,.F.);
#31668=ORIENTED_EDGE('',*,*,#23775,.F.);
#31669=ORIENTED_EDGE('',*,*,#23776,.F.);
#31670=ORIENTED_EDGE('',*,*,#23777,.F.);
#31671=ORIENTED_EDGE('',*,*,#23778,.F.);
#31672=ORIENTED_EDGE('',*,*,#23779,.F.);
#31673=ORIENTED_EDGE('',*,*,#23780,.F.);
#31674=ORIENTED_EDGE('',*,*,#23781,.F.);
#31675=ORIENTED_EDGE('',*,*,#23782,.F.);
#31676=ORIENTED_EDGE('',*,*,#23783,.F.);
#31677=ORIENTED_EDGE('',*,*,#23784,.F.);
#31678=ORIENTED_EDGE('',*,*,#23785,.F.);
#31679=ORIENTED_EDGE('',*,*,#23786,.F.);
#31680=ORIENTED_EDGE('',*,*,#23787,.F.);
#31681=ORIENTED_EDGE('',*,*,#23788,.F.);
#31682=ORIENTED_EDGE('',*,*,#23789,.F.);
#31683=ORIENTED_EDGE('',*,*,#23790,.F.);
#31684=ORIENTED_EDGE('',*,*,#23791,.F.);
#31685=ORIENTED_EDGE('',*,*,#23792,.F.);
#31686=ORIENTED_EDGE('',*,*,#23793,.F.);
#31687=ORIENTED_EDGE('',*,*,#23794,.F.);
#31688=ORIENTED_EDGE('',*,*,#23795,.F.);
#31689=ORIENTED_EDGE('',*,*,#23796,.F.);
#31690=ORIENTED_EDGE('',*,*,#23797,.F.);
#31691=ORIENTED_EDGE('',*,*,#23798,.F.);
#31692=ORIENTED_EDGE('',*,*,#23799,.F.);
#31693=ORIENTED_EDGE('',*,*,#23800,.F.);
#31694=ORIENTED_EDGE('',*,*,#23801,.F.);
#31695=ORIENTED_EDGE('',*,*,#23802,.F.);
#31696=ORIENTED_EDGE('',*,*,#23803,.F.);
#31697=ORIENTED_EDGE('',*,*,#23804,.F.);
#31698=ORIENTED_EDGE('',*,*,#23805,.F.);
#31699=ORIENTED_EDGE('',*,*,#23806,.F.);
#31700=ORIENTED_EDGE('',*,*,#23807,.F.);
#31701=ORIENTED_EDGE('',*,*,#23808,.F.);
#31702=ORIENTED_EDGE('',*,*,#23809,.F.);
#31703=ORIENTED_EDGE('',*,*,#23810,.F.);
#31704=ORIENTED_EDGE('',*,*,#23811,.F.);
#31705=ORIENTED_EDGE('',*,*,#23812,.F.);
#31706=ORIENTED_EDGE('',*,*,#23813,.F.);
#31707=ORIENTED_EDGE('',*,*,#23814,.F.);
#31708=ORIENTED_EDGE('',*,*,#23815,.F.);
#31709=ORIENTED_EDGE('',*,*,#23816,.F.);
#31710=ORIENTED_EDGE('',*,*,#23817,.F.);
#31711=ORIENTED_EDGE('',*,*,#23818,.F.);
#31712=ORIENTED_EDGE('',*,*,#23819,.F.);
#31713=ORIENTED_EDGE('',*,*,#23820,.F.);
#31714=ORIENTED_EDGE('',*,*,#23821,.F.);
#31715=ORIENTED_EDGE('',*,*,#23822,.F.);
#31716=ORIENTED_EDGE('',*,*,#23823,.F.);
#31717=ORIENTED_EDGE('',*,*,#23824,.F.);
#31718=ORIENTED_EDGE('',*,*,#23825,.F.);
#31719=ORIENTED_EDGE('',*,*,#23826,.F.);
#31720=ORIENTED_EDGE('',*,*,#23827,.F.);
#31721=ORIENTED_EDGE('',*,*,#23828,.F.);
#31722=ORIENTED_EDGE('',*,*,#23829,.F.);
#31723=ORIENTED_EDGE('',*,*,#23830,.F.);
#31724=ORIENTED_EDGE('',*,*,#23831,.F.);
#31725=ORIENTED_EDGE('',*,*,#23832,.F.);
#31726=ORIENTED_EDGE('',*,*,#23833,.F.);
#31727=ORIENTED_EDGE('',*,*,#23834,.F.);
#31728=ORIENTED_EDGE('',*,*,#23835,.F.);
#31729=ORIENTED_EDGE('',*,*,#23836,.F.);
#31730=ORIENTED_EDGE('',*,*,#23837,.F.);
#31731=ORIENTED_EDGE('',*,*,#23838,.F.);
#31732=ORIENTED_EDGE('',*,*,#23839,.F.);
#31733=ORIENTED_EDGE('',*,*,#23840,.F.);
#31734=ORIENTED_EDGE('',*,*,#23841,.F.);
#31735=ORIENTED_EDGE('',*,*,#23842,.F.);
#31736=ORIENTED_EDGE('',*,*,#23843,.F.);
#31737=ORIENTED_EDGE('',*,*,#23844,.F.);
#31738=ORIENTED_EDGE('',*,*,#23845,.F.);
#31739=ORIENTED_EDGE('',*,*,#23846,.F.);
#31740=ORIENTED_EDGE('',*,*,#23847,.F.);
#31741=ORIENTED_EDGE('',*,*,#23848,.F.);
#31742=ORIENTED_EDGE('',*,*,#23849,.F.);
#31743=ORIENTED_EDGE('',*,*,#23850,.F.);
#31744=ORIENTED_EDGE('',*,*,#23851,.F.);
#31745=ORIENTED_EDGE('',*,*,#23852,.F.);
#31746=ORIENTED_EDGE('',*,*,#23853,.F.);
#31747=ORIENTED_EDGE('',*,*,#23854,.F.);
#31748=ORIENTED_EDGE('',*,*,#23855,.F.);
#31749=ORIENTED_EDGE('',*,*,#23856,.F.);
#31750=ORIENTED_EDGE('',*,*,#23857,.F.);
#31751=ORIENTED_EDGE('',*,*,#23858,.F.);
#31752=ORIENTED_EDGE('',*,*,#23859,.F.);
#31753=ORIENTED_EDGE('',*,*,#23860,.F.);
#31754=ORIENTED_EDGE('',*,*,#23861,.F.);
#31755=ORIENTED_EDGE('',*,*,#23862,.F.);
#31756=ORIENTED_EDGE('',*,*,#23863,.F.);
#31757=ORIENTED_EDGE('',*,*,#23864,.F.);
#31758=ORIENTED_EDGE('',*,*,#23865,.F.);
#31759=ORIENTED_EDGE('',*,*,#23866,.F.);
#31760=ORIENTED_EDGE('',*,*,#23867,.F.);
#31761=ORIENTED_EDGE('',*,*,#23868,.F.);
#31762=ORIENTED_EDGE('',*,*,#23869,.F.);
#31763=ORIENTED_EDGE('',*,*,#23870,.F.);
#31764=ORIENTED_EDGE('',*,*,#23871,.F.);
#31765=ORIENTED_EDGE('',*,*,#23872,.F.);
#31766=ORIENTED_EDGE('',*,*,#23873,.F.);
#31767=ORIENTED_EDGE('',*,*,#23874,.F.);
#31768=ORIENTED_EDGE('',*,*,#23875,.F.);
#31769=ORIENTED_EDGE('',*,*,#23876,.F.);
#31770=ORIENTED_EDGE('',*,*,#23877,.F.);
#31771=ORIENTED_EDGE('',*,*,#23878,.F.);
#31772=ORIENTED_EDGE('',*,*,#23879,.F.);
#31773=ORIENTED_EDGE('',*,*,#23880,.F.);
#31774=ORIENTED_EDGE('',*,*,#23881,.F.);
#31775=ORIENTED_EDGE('',*,*,#23882,.F.);
#31776=ORIENTED_EDGE('',*,*,#23883,.F.);
#31777=ORIENTED_EDGE('',*,*,#23884,.F.);
#31778=ORIENTED_EDGE('',*,*,#23885,.F.);
#31779=ORIENTED_EDGE('',*,*,#23886,.F.);
#31780=ORIENTED_EDGE('',*,*,#23887,.F.);
#31781=ORIENTED_EDGE('',*,*,#23888,.F.);
#31782=ORIENTED_EDGE('',*,*,#23889,.F.);
#31783=ORIENTED_EDGE('',*,*,#23890,.F.);
#31784=ORIENTED_EDGE('',*,*,#23891,.F.);
#31785=ORIENTED_EDGE('',*,*,#23892,.F.);
#31786=ORIENTED_EDGE('',*,*,#23893,.F.);
#31787=ORIENTED_EDGE('',*,*,#23894,.F.);
#31788=ORIENTED_EDGE('',*,*,#23895,.F.);
#31789=ORIENTED_EDGE('',*,*,#23896,.F.);
#31790=ORIENTED_EDGE('',*,*,#23897,.F.);
#31791=ORIENTED_EDGE('',*,*,#23898,.F.);
#31792=ORIENTED_EDGE('',*,*,#23899,.F.);
#31793=ORIENTED_EDGE('',*,*,#23900,.F.);
#31794=ORIENTED_EDGE('',*,*,#23901,.F.);
#31795=ORIENTED_EDGE('',*,*,#23902,.F.);
#31796=ORIENTED_EDGE('',*,*,#23903,.F.);
#31797=ORIENTED_EDGE('',*,*,#23904,.F.);
#31798=ORIENTED_EDGE('',*,*,#23905,.F.);
#31799=ORIENTED_EDGE('',*,*,#23906,.F.);
#31800=ORIENTED_EDGE('',*,*,#23907,.F.);
#31801=ORIENTED_EDGE('',*,*,#23908,.F.);
#31802=ORIENTED_EDGE('',*,*,#23909,.F.);
#31803=ORIENTED_EDGE('',*,*,#23910,.F.);
#31804=ORIENTED_EDGE('',*,*,#23911,.F.);
#31805=ORIENTED_EDGE('',*,*,#23912,.F.);
#31806=ORIENTED_EDGE('',*,*,#23913,.F.);
#31807=ORIENTED_EDGE('',*,*,#23914,.F.);
#31808=ORIENTED_EDGE('',*,*,#23915,.F.);
#31809=ORIENTED_EDGE('',*,*,#23916,.F.);
#31810=ORIENTED_EDGE('',*,*,#23917,.F.);
#31811=ORIENTED_EDGE('',*,*,#23918,.F.);
#31812=ORIENTED_EDGE('',*,*,#23919,.F.);
#31813=ORIENTED_EDGE('',*,*,#23920,.F.);
#31814=ORIENTED_EDGE('',*,*,#23921,.F.);
#31815=ORIENTED_EDGE('',*,*,#23922,.F.);
#31816=ORIENTED_EDGE('',*,*,#23923,.F.);
#31817=ORIENTED_EDGE('',*,*,#23924,.F.);
#31818=ORIENTED_EDGE('',*,*,#23925,.F.);
#31819=ORIENTED_EDGE('',*,*,#23926,.F.);
#31820=ORIENTED_EDGE('',*,*,#23927,.F.);
#31821=ORIENTED_EDGE('',*,*,#23928,.F.);
#31822=ORIENTED_EDGE('',*,*,#23929,.F.);
#31823=ORIENTED_EDGE('',*,*,#23930,.F.);
#31824=ORIENTED_EDGE('',*,*,#23931,.F.);
#31825=ORIENTED_EDGE('',*,*,#23932,.F.);
#31826=ORIENTED_EDGE('',*,*,#23933,.F.);
#31827=ORIENTED_EDGE('',*,*,#23934,.F.);
#31828=ORIENTED_EDGE('',*,*,#23935,.F.);
#31829=ORIENTED_EDGE('',*,*,#23936,.F.);
#31830=ORIENTED_EDGE('',*,*,#23937,.F.);
#31831=ORIENTED_EDGE('',*,*,#23938,.F.);
#31832=ORIENTED_EDGE('',*,*,#23939,.F.);
#31833=ORIENTED_EDGE('',*,*,#23940,.F.);
#31834=ORIENTED_EDGE('',*,*,#23941,.F.);
#31835=ORIENTED_EDGE('',*,*,#23942,.F.);
#31836=ORIENTED_EDGE('',*,*,#23943,.F.);
#31837=ORIENTED_EDGE('',*,*,#23944,.F.);
#31838=ORIENTED_EDGE('',*,*,#23945,.F.);
#31839=ORIENTED_EDGE('',*,*,#23946,.F.);
#31840=ORIENTED_EDGE('',*,*,#23947,.F.);
#31841=ORIENTED_EDGE('',*,*,#23948,.F.);
#31842=ORIENTED_EDGE('',*,*,#23949,.F.);
#31843=ORIENTED_EDGE('',*,*,#23950,.F.);
#31844=ORIENTED_EDGE('',*,*,#23951,.F.);
#31845=ORIENTED_EDGE('',*,*,#23952,.F.);
#31846=ORIENTED_EDGE('',*,*,#23953,.F.);
#31847=ORIENTED_EDGE('',*,*,#23954,.F.);
#31848=ORIENTED_EDGE('',*,*,#23955,.F.);
#31849=ORIENTED_EDGE('',*,*,#23956,.F.);
#31850=ORIENTED_EDGE('',*,*,#23957,.F.);
#31851=ORIENTED_EDGE('',*,*,#23958,.F.);
#31852=ORIENTED_EDGE('',*,*,#23959,.F.);
#31853=ORIENTED_EDGE('',*,*,#23960,.F.);
#31854=ORIENTED_EDGE('',*,*,#23961,.F.);
#31855=ORIENTED_EDGE('',*,*,#23962,.F.);
#31856=ORIENTED_EDGE('',*,*,#23963,.F.);
#31857=ORIENTED_EDGE('',*,*,#23964,.F.);
#31858=ORIENTED_EDGE('',*,*,#23965,.F.);
#31859=ORIENTED_EDGE('',*,*,#23966,.F.);
#31860=ORIENTED_EDGE('',*,*,#23967,.F.);
#31861=ORIENTED_EDGE('',*,*,#23968,.F.);
#31862=ORIENTED_EDGE('',*,*,#23969,.F.);
#31863=ORIENTED_EDGE('',*,*,#23970,.F.);
#31864=ORIENTED_EDGE('',*,*,#23971,.F.);
#31865=ORIENTED_EDGE('',*,*,#23972,.F.);
#31866=ORIENTED_EDGE('',*,*,#23973,.F.);
#31867=ORIENTED_EDGE('',*,*,#23974,.F.);
#31868=ORIENTED_EDGE('',*,*,#23975,.F.);
#31869=ORIENTED_EDGE('',*,*,#23976,.F.);
#31870=ORIENTED_EDGE('',*,*,#23977,.F.);
#31871=ORIENTED_EDGE('',*,*,#23978,.F.);
#31872=ORIENTED_EDGE('',*,*,#23979,.F.);
#31873=ORIENTED_EDGE('',*,*,#23980,.F.);
#31874=ORIENTED_EDGE('',*,*,#23981,.F.);
#31875=ORIENTED_EDGE('',*,*,#23982,.F.);
#31876=ORIENTED_EDGE('',*,*,#23983,.F.);
#31877=ORIENTED_EDGE('',*,*,#23984,.F.);
#31878=ORIENTED_EDGE('',*,*,#23985,.F.);
#31879=ORIENTED_EDGE('',*,*,#23986,.F.);
#31880=ORIENTED_EDGE('',*,*,#23987,.F.);
#31881=ORIENTED_EDGE('',*,*,#23988,.F.);
#31882=ORIENTED_EDGE('',*,*,#23989,.F.);
#31883=ORIENTED_EDGE('',*,*,#23990,.F.);
#31884=ORIENTED_EDGE('',*,*,#23991,.F.);
#31885=ORIENTED_EDGE('',*,*,#23992,.F.);
#31886=ORIENTED_EDGE('',*,*,#23993,.F.);
#31887=ORIENTED_EDGE('',*,*,#23994,.F.);
#31888=ORIENTED_EDGE('',*,*,#23995,.F.);
#31889=ORIENTED_EDGE('',*,*,#23996,.F.);
#31890=ORIENTED_EDGE('',*,*,#23997,.F.);
#31891=ORIENTED_EDGE('',*,*,#23998,.F.);
#31892=ORIENTED_EDGE('',*,*,#23999,.F.);
#31893=ORIENTED_EDGE('',*,*,#24000,.F.);
#31894=ORIENTED_EDGE('',*,*,#24001,.F.);
#31895=ORIENTED_EDGE('',*,*,#24002,.F.);
#31896=ORIENTED_EDGE('',*,*,#24003,.F.);
#31897=ORIENTED_EDGE('',*,*,#24004,.F.);
#31898=ORIENTED_EDGE('',*,*,#24005,.F.);
#31899=ORIENTED_EDGE('',*,*,#24006,.F.);
#31900=ORIENTED_EDGE('',*,*,#24007,.F.);
#31901=ORIENTED_EDGE('',*,*,#24008,.F.);
#31902=ORIENTED_EDGE('',*,*,#24009,.F.);
#31903=ORIENTED_EDGE('',*,*,#24010,.F.);
#31904=ORIENTED_EDGE('',*,*,#24011,.F.);
#31905=ORIENTED_EDGE('',*,*,#24012,.F.);
#31906=ORIENTED_EDGE('',*,*,#24013,.F.);
#31907=ORIENTED_EDGE('',*,*,#24014,.F.);
#31908=ORIENTED_EDGE('',*,*,#24015,.F.);
#31909=ORIENTED_EDGE('',*,*,#24016,.F.);
#31910=ORIENTED_EDGE('',*,*,#24017,.F.);
#31911=ORIENTED_EDGE('',*,*,#24018,.F.);
#31912=ORIENTED_EDGE('',*,*,#24019,.F.);
#31913=ORIENTED_EDGE('',*,*,#24020,.F.);
#31914=ORIENTED_EDGE('',*,*,#24021,.F.);
#31915=ORIENTED_EDGE('',*,*,#24022,.F.);
#31916=ORIENTED_EDGE('',*,*,#24023,.F.);
#31917=ORIENTED_EDGE('',*,*,#24024,.F.);
#31918=ORIENTED_EDGE('',*,*,#24025,.F.);
#31919=ORIENTED_EDGE('',*,*,#24026,.F.);
#31920=ORIENTED_EDGE('',*,*,#24027,.F.);
#31921=ORIENTED_EDGE('',*,*,#24028,.F.);
#31922=ORIENTED_EDGE('',*,*,#24029,.F.);
#31923=ORIENTED_EDGE('',*,*,#24030,.F.);
#31924=ORIENTED_EDGE('',*,*,#24031,.F.);
#31925=ORIENTED_EDGE('',*,*,#24032,.F.);
#31926=ORIENTED_EDGE('',*,*,#24033,.F.);
#31927=ORIENTED_EDGE('',*,*,#24034,.F.);
#31928=ORIENTED_EDGE('',*,*,#24035,.F.);
#31929=ORIENTED_EDGE('',*,*,#24036,.F.);
#31930=ORIENTED_EDGE('',*,*,#24037,.F.);
#31931=ORIENTED_EDGE('',*,*,#24038,.F.);
#31932=ORIENTED_EDGE('',*,*,#24039,.F.);
#31933=ORIENTED_EDGE('',*,*,#24040,.F.);
#31934=ORIENTED_EDGE('',*,*,#24041,.F.);
#31935=ORIENTED_EDGE('',*,*,#24042,.F.);
#31936=ORIENTED_EDGE('',*,*,#24043,.F.);
#31937=ORIENTED_EDGE('',*,*,#24044,.F.);
#31938=ORIENTED_EDGE('',*,*,#24045,.F.);
#31939=ORIENTED_EDGE('',*,*,#24046,.F.);
#31940=ORIENTED_EDGE('',*,*,#24047,.F.);
#31941=ORIENTED_EDGE('',*,*,#24048,.F.);
#31942=ORIENTED_EDGE('',*,*,#24049,.F.);
#31943=ORIENTED_EDGE('',*,*,#24050,.F.);
#31944=ORIENTED_EDGE('',*,*,#24051,.F.);
#31945=ORIENTED_EDGE('',*,*,#24052,.F.);
#31946=ORIENTED_EDGE('',*,*,#24053,.F.);
#31947=ORIENTED_EDGE('',*,*,#24054,.F.);
#31948=ORIENTED_EDGE('',*,*,#24055,.F.);
#31949=ORIENTED_EDGE('',*,*,#24056,.F.);
#31950=ORIENTED_EDGE('',*,*,#24057,.F.);
#31951=ORIENTED_EDGE('',*,*,#24058,.F.);
#31952=ORIENTED_EDGE('',*,*,#24059,.F.);
#31953=ORIENTED_EDGE('',*,*,#24060,.F.);
#31954=ORIENTED_EDGE('',*,*,#24061,.F.);
#31955=ORIENTED_EDGE('',*,*,#24062,.F.);
#31956=ORIENTED_EDGE('',*,*,#24063,.F.);
#31957=ORIENTED_EDGE('',*,*,#24064,.F.);
#31958=ORIENTED_EDGE('',*,*,#24065,.F.);
#31959=ORIENTED_EDGE('',*,*,#24066,.F.);
#31960=ORIENTED_EDGE('',*,*,#24067,.F.);
#31961=ORIENTED_EDGE('',*,*,#24068,.F.);
#31962=ORIENTED_EDGE('',*,*,#24069,.F.);
#31963=ORIENTED_EDGE('',*,*,#24070,.F.);
#31964=ORIENTED_EDGE('',*,*,#24071,.F.);
#31965=ORIENTED_EDGE('',*,*,#24072,.F.);
#31966=ORIENTED_EDGE('',*,*,#24073,.F.);
#31967=ORIENTED_EDGE('',*,*,#24074,.F.);
#31968=ORIENTED_EDGE('',*,*,#24075,.F.);
#31969=ORIENTED_EDGE('',*,*,#24076,.F.);
#31970=ORIENTED_EDGE('',*,*,#24077,.F.);
#31971=ORIENTED_EDGE('',*,*,#24078,.F.);
#31972=ORIENTED_EDGE('',*,*,#24079,.F.);
#31973=ORIENTED_EDGE('',*,*,#24080,.F.);
#31974=ORIENTED_EDGE('',*,*,#24081,.F.);
#31975=ORIENTED_EDGE('',*,*,#24082,.F.);
#31976=ORIENTED_EDGE('',*,*,#24083,.F.);
#31977=ORIENTED_EDGE('',*,*,#24084,.F.);
#31978=ORIENTED_EDGE('',*,*,#24085,.F.);
#31979=ORIENTED_EDGE('',*,*,#24086,.F.);
#31980=ORIENTED_EDGE('',*,*,#24087,.F.);
#31981=ORIENTED_EDGE('',*,*,#24088,.F.);
#31982=ORIENTED_EDGE('',*,*,#24089,.F.);
#31983=ORIENTED_EDGE('',*,*,#24090,.F.);
#31984=ORIENTED_EDGE('',*,*,#24091,.F.);
#31985=ORIENTED_EDGE('',*,*,#24092,.F.);
#31986=ORIENTED_EDGE('',*,*,#24093,.F.);
#31987=ORIENTED_EDGE('',*,*,#24094,.F.);
#31988=ORIENTED_EDGE('',*,*,#24095,.F.);
#31989=ORIENTED_EDGE('',*,*,#24096,.F.);
#31990=ORIENTED_EDGE('',*,*,#24097,.F.);
#31991=ORIENTED_EDGE('',*,*,#24098,.F.);
#31992=ORIENTED_EDGE('',*,*,#24099,.F.);
#31993=ORIENTED_EDGE('',*,*,#24100,.F.);
#31994=ORIENTED_EDGE('',*,*,#24101,.F.);
#31995=ORIENTED_EDGE('',*,*,#24102,.F.);
#31996=ORIENTED_EDGE('',*,*,#24103,.F.);
#31997=ORIENTED_EDGE('',*,*,#24104,.F.);
#31998=ORIENTED_EDGE('',*,*,#24105,.F.);
#31999=ORIENTED_EDGE('',*,*,#24106,.F.);
#32000=ORIENTED_EDGE('',*,*,#24107,.F.);
#32001=ORIENTED_EDGE('',*,*,#24108,.F.);
#32002=ORIENTED_EDGE('',*,*,#24109,.F.);
#32003=ORIENTED_EDGE('',*,*,#24110,.F.);
#32004=ORIENTED_EDGE('',*,*,#24111,.F.);
#32005=ORIENTED_EDGE('',*,*,#24112,.F.);
#32006=ORIENTED_EDGE('',*,*,#24113,.F.);
#32007=ORIENTED_EDGE('',*,*,#24114,.F.);
#32008=ORIENTED_EDGE('',*,*,#24115,.F.);
#32009=ORIENTED_EDGE('',*,*,#24116,.F.);
#32010=ORIENTED_EDGE('',*,*,#24117,.F.);
#32011=ORIENTED_EDGE('',*,*,#24118,.F.);
#32012=ORIENTED_EDGE('',*,*,#24119,.F.);
#32013=ORIENTED_EDGE('',*,*,#24120,.F.);
#32014=ORIENTED_EDGE('',*,*,#24121,.F.);
#32015=ORIENTED_EDGE('',*,*,#24122,.F.);
#32016=ORIENTED_EDGE('',*,*,#24123,.F.);
#32017=ORIENTED_EDGE('',*,*,#24124,.F.);
#32018=ORIENTED_EDGE('',*,*,#24125,.F.);
#32019=ORIENTED_EDGE('',*,*,#24126,.F.);
#32020=ORIENTED_EDGE('',*,*,#24127,.F.);
#32021=ORIENTED_EDGE('',*,*,#24128,.F.);
#32022=ORIENTED_EDGE('',*,*,#24129,.F.);
#32023=ORIENTED_EDGE('',*,*,#24130,.F.);
#32024=ORIENTED_EDGE('',*,*,#24131,.F.);
#32025=ORIENTED_EDGE('',*,*,#24132,.F.);
#32026=ORIENTED_EDGE('',*,*,#24133,.F.);
#32027=ORIENTED_EDGE('',*,*,#24134,.F.);
#32028=ORIENTED_EDGE('',*,*,#24135,.F.);
#32029=ORIENTED_EDGE('',*,*,#24136,.F.);
#32030=ORIENTED_EDGE('',*,*,#24137,.F.);
#32031=ORIENTED_EDGE('',*,*,#24138,.F.);
#32032=ORIENTED_EDGE('',*,*,#24139,.F.);
#32033=ORIENTED_EDGE('',*,*,#24140,.F.);
#32034=ORIENTED_EDGE('',*,*,#24141,.F.);
#32035=ORIENTED_EDGE('',*,*,#24142,.F.);
#32036=ORIENTED_EDGE('',*,*,#24143,.F.);
#32037=ORIENTED_EDGE('',*,*,#24144,.F.);
#32038=ORIENTED_EDGE('',*,*,#24145,.F.);
#32039=ORIENTED_EDGE('',*,*,#24146,.F.);
#32040=ORIENTED_EDGE('',*,*,#24147,.F.);
#32041=ORIENTED_EDGE('',*,*,#24148,.F.);
#32042=ORIENTED_EDGE('',*,*,#24149,.F.);
#32043=ORIENTED_EDGE('',*,*,#24150,.F.);
#32044=ORIENTED_EDGE('',*,*,#24151,.F.);
#32045=ORIENTED_EDGE('',*,*,#24152,.F.);
#32046=ORIENTED_EDGE('',*,*,#24153,.F.);
#32047=ORIENTED_EDGE('',*,*,#24154,.F.);
#32048=ORIENTED_EDGE('',*,*,#24155,.F.);
#32049=ORIENTED_EDGE('',*,*,#24156,.F.);
#32050=ORIENTED_EDGE('',*,*,#24157,.F.);
#32051=ORIENTED_EDGE('',*,*,#24158,.F.);
#32052=ORIENTED_EDGE('',*,*,#24159,.F.);
#32053=ORIENTED_EDGE('',*,*,#24160,.F.);
#32054=ORIENTED_EDGE('',*,*,#24161,.F.);
#32055=ORIENTED_EDGE('',*,*,#24162,.F.);
#32056=ORIENTED_EDGE('',*,*,#24163,.F.);
#32057=ORIENTED_EDGE('',*,*,#24164,.F.);
#32058=ORIENTED_EDGE('',*,*,#24165,.F.);
#32059=ORIENTED_EDGE('',*,*,#24166,.F.);
#32060=ORIENTED_EDGE('',*,*,#24167,.F.);
#32061=ORIENTED_EDGE('',*,*,#24168,.F.);
#32062=ORIENTED_EDGE('',*,*,#24169,.F.);
#32063=ORIENTED_EDGE('',*,*,#24170,.F.);
#32064=ORIENTED_EDGE('',*,*,#24171,.F.);
#32065=ORIENTED_EDGE('',*,*,#24172,.F.);
#32066=ORIENTED_EDGE('',*,*,#24173,.F.);
#32067=ORIENTED_EDGE('',*,*,#24174,.F.);
#32068=ORIENTED_EDGE('',*,*,#24175,.F.);
#32069=ORIENTED_EDGE('',*,*,#24176,.F.);
#32070=ORIENTED_EDGE('',*,*,#24177,.F.);
#32071=ORIENTED_EDGE('',*,*,#24178,.F.);
#32072=ORIENTED_EDGE('',*,*,#24179,.F.);
#32073=ORIENTED_EDGE('',*,*,#24180,.F.);
#32074=ORIENTED_EDGE('',*,*,#24181,.F.);
#32075=ORIENTED_EDGE('',*,*,#24182,.F.);
#32076=ORIENTED_EDGE('',*,*,#24183,.F.);
#32077=ORIENTED_EDGE('',*,*,#24184,.F.);
#32078=ORIENTED_EDGE('',*,*,#24185,.F.);
#32079=ORIENTED_EDGE('',*,*,#24186,.F.);
#32080=ORIENTED_EDGE('',*,*,#24187,.F.);
#32081=ORIENTED_EDGE('',*,*,#24188,.F.);
#32082=ORIENTED_EDGE('',*,*,#24189,.F.);
#32083=ORIENTED_EDGE('',*,*,#24190,.F.);
#32084=ORIENTED_EDGE('',*,*,#24191,.F.);
#32085=ORIENTED_EDGE('',*,*,#24192,.F.);
#32086=ORIENTED_EDGE('',*,*,#24193,.F.);
#32087=ORIENTED_EDGE('',*,*,#24194,.F.);
#32088=ORIENTED_EDGE('',*,*,#24195,.F.);
#32089=ORIENTED_EDGE('',*,*,#24196,.F.);
#32090=ORIENTED_EDGE('',*,*,#24197,.F.);
#32091=ORIENTED_EDGE('',*,*,#24198,.F.);
#32092=ORIENTED_EDGE('',*,*,#24199,.F.);
#32093=ORIENTED_EDGE('',*,*,#24200,.F.);
#32094=ORIENTED_EDGE('',*,*,#24201,.F.);
#32095=ORIENTED_EDGE('',*,*,#24202,.F.);
#32096=ORIENTED_EDGE('',*,*,#24203,.F.);
#32097=ORIENTED_EDGE('',*,*,#24204,.F.);
#32098=ORIENTED_EDGE('',*,*,#24205,.F.);
#32099=ORIENTED_EDGE('',*,*,#24206,.F.);
#32100=ORIENTED_EDGE('',*,*,#24207,.F.);
#32101=ORIENTED_EDGE('',*,*,#24208,.F.);
#32102=ORIENTED_EDGE('',*,*,#24209,.F.);
#32103=ORIENTED_EDGE('',*,*,#24210,.F.);
#32104=ORIENTED_EDGE('',*,*,#24211,.F.);
#32105=ORIENTED_EDGE('',*,*,#24212,.F.);
#32106=ORIENTED_EDGE('',*,*,#24213,.F.);
#32107=ORIENTED_EDGE('',*,*,#24214,.F.);
#32108=ORIENTED_EDGE('',*,*,#24215,.F.);
#32109=ORIENTED_EDGE('',*,*,#24216,.F.);
#32110=ORIENTED_EDGE('',*,*,#24217,.F.);
#32111=ORIENTED_EDGE('',*,*,#24218,.F.);
#32112=ORIENTED_EDGE('',*,*,#24219,.F.);
#32113=ORIENTED_EDGE('',*,*,#24220,.F.);
#32114=ORIENTED_EDGE('',*,*,#24221,.F.);
#32115=ORIENTED_EDGE('',*,*,#24222,.F.);
#32116=ORIENTED_EDGE('',*,*,#24223,.F.);
#32117=ORIENTED_EDGE('',*,*,#24224,.F.);
#32118=ORIENTED_EDGE('',*,*,#24225,.F.);
#32119=ORIENTED_EDGE('',*,*,#24226,.F.);
#32120=ORIENTED_EDGE('',*,*,#24227,.F.);
#32121=ORIENTED_EDGE('',*,*,#24228,.F.);
#32122=ORIENTED_EDGE('',*,*,#24229,.F.);
#32123=ORIENTED_EDGE('',*,*,#24230,.F.);
#32124=ORIENTED_EDGE('',*,*,#24231,.F.);
#32125=ORIENTED_EDGE('',*,*,#24232,.F.);
#32126=ORIENTED_EDGE('',*,*,#24233,.F.);
#32127=ORIENTED_EDGE('',*,*,#24234,.F.);
#32128=ORIENTED_EDGE('',*,*,#24235,.F.);
#32129=ORIENTED_EDGE('',*,*,#24236,.F.);
#32130=ORIENTED_EDGE('',*,*,#24237,.F.);
#32131=ORIENTED_EDGE('',*,*,#24238,.F.);
#32132=ORIENTED_EDGE('',*,*,#24239,.F.);
#32133=ORIENTED_EDGE('',*,*,#24240,.F.);
#32134=ORIENTED_EDGE('',*,*,#24241,.F.);
#32135=ORIENTED_EDGE('',*,*,#24242,.F.);
#32136=ORIENTED_EDGE('',*,*,#24243,.F.);
#32137=ORIENTED_EDGE('',*,*,#24244,.F.);
#32138=ORIENTED_EDGE('',*,*,#23009,.F.);
#32139=ORIENTED_EDGE('',*,*,#24245,.T.);
#32140=ORIENTED_EDGE('',*,*,#24246,.T.);
#32141=ORIENTED_EDGE('',*,*,#24247,.T.);
#32142=ORIENTED_EDGE('',*,*,#24248,.T.);
#32143=ORIENTED_EDGE('',*,*,#24249,.T.);
#32144=ORIENTED_EDGE('',*,*,#24250,.T.);
#32145=ORIENTED_EDGE('',*,*,#24251,.T.);
#32146=ORIENTED_EDGE('',*,*,#24252,.T.);
#32147=ORIENTED_EDGE('',*,*,#24253,.T.);
#32148=ORIENTED_EDGE('',*,*,#24254,.T.);
#32149=ORIENTED_EDGE('',*,*,#24255,.T.);
#32150=ORIENTED_EDGE('',*,*,#24256,.T.);
#32151=ORIENTED_EDGE('',*,*,#24257,.T.);
#32152=ORIENTED_EDGE('',*,*,#24258,.T.);
#32153=ORIENTED_EDGE('',*,*,#24259,.T.);
#32154=ORIENTED_EDGE('',*,*,#24260,.T.);
#32155=ORIENTED_EDGE('',*,*,#24261,.T.);
#32156=ORIENTED_EDGE('',*,*,#24262,.T.);
#32157=ORIENTED_EDGE('',*,*,#24263,.T.);
#32158=ORIENTED_EDGE('',*,*,#24264,.T.);
#32159=ORIENTED_EDGE('',*,*,#24265,.T.);
#32160=ORIENTED_EDGE('',*,*,#24266,.T.);
#32161=ORIENTED_EDGE('',*,*,#24267,.T.);
#32162=ORIENTED_EDGE('',*,*,#24268,.T.);
#32163=ORIENTED_EDGE('',*,*,#24269,.T.);
#32164=ORIENTED_EDGE('',*,*,#24270,.T.);
#32165=ORIENTED_EDGE('',*,*,#24271,.T.);
#32166=ORIENTED_EDGE('',*,*,#24272,.T.);
#32167=ORIENTED_EDGE('',*,*,#24273,.T.);
#32168=ORIENTED_EDGE('',*,*,#24274,.T.);
#32169=ORIENTED_EDGE('',*,*,#24275,.T.);
#32170=ORIENTED_EDGE('',*,*,#24276,.T.);
#32171=ORIENTED_EDGE('',*,*,#24277,.T.);
#32172=ORIENTED_EDGE('',*,*,#24278,.T.);
#32173=ORIENTED_EDGE('',*,*,#24279,.T.);
#32174=ORIENTED_EDGE('',*,*,#24280,.T.);
#32175=ORIENTED_EDGE('',*,*,#24281,.T.);
#32176=ORIENTED_EDGE('',*,*,#24282,.T.);
#32177=ORIENTED_EDGE('',*,*,#24283,.T.);
#32178=ORIENTED_EDGE('',*,*,#24284,.T.);
#32179=ORIENTED_EDGE('',*,*,#24285,.T.);
#32180=ORIENTED_EDGE('',*,*,#24286,.T.);
#32181=ORIENTED_EDGE('',*,*,#24287,.T.);
#32182=ORIENTED_EDGE('',*,*,#24288,.T.);
#32183=ORIENTED_EDGE('',*,*,#24289,.T.);
#32184=ORIENTED_EDGE('',*,*,#24290,.T.);
#32185=ORIENTED_EDGE('',*,*,#24291,.T.);
#32186=ORIENTED_EDGE('',*,*,#24292,.T.);
#32187=ORIENTED_EDGE('',*,*,#24293,.T.);
#32188=ORIENTED_EDGE('',*,*,#24294,.T.);
#32189=ORIENTED_EDGE('',*,*,#24295,.T.);
#32190=ORIENTED_EDGE('',*,*,#24296,.T.);
#32191=ORIENTED_EDGE('',*,*,#24297,.T.);
#32192=ORIENTED_EDGE('',*,*,#24298,.T.);
#32193=ORIENTED_EDGE('',*,*,#24299,.T.);
#32194=ORIENTED_EDGE('',*,*,#24300,.T.);
#32195=ORIENTED_EDGE('',*,*,#24301,.T.);
#32196=ORIENTED_EDGE('',*,*,#24302,.T.);
#32197=ORIENTED_EDGE('',*,*,#24303,.T.);
#32198=ORIENTED_EDGE('',*,*,#24304,.T.);
#32199=ORIENTED_EDGE('',*,*,#24305,.T.);
#32200=ORIENTED_EDGE('',*,*,#24306,.T.);
#32201=ORIENTED_EDGE('',*,*,#24307,.T.);
#32202=ORIENTED_EDGE('',*,*,#24308,.T.);
#32203=ORIENTED_EDGE('',*,*,#24309,.T.);
#32204=ORIENTED_EDGE('',*,*,#24310,.T.);
#32205=ORIENTED_EDGE('',*,*,#24311,.T.);
#32206=ORIENTED_EDGE('',*,*,#24312,.T.);
#32207=ORIENTED_EDGE('',*,*,#24313,.T.);
#32208=ORIENTED_EDGE('',*,*,#24314,.T.);
#32209=ORIENTED_EDGE('',*,*,#24315,.T.);
#32210=ORIENTED_EDGE('',*,*,#24316,.T.);
#32211=ORIENTED_EDGE('',*,*,#24317,.T.);
#32212=ORIENTED_EDGE('',*,*,#24318,.T.);
#32213=ORIENTED_EDGE('',*,*,#24319,.T.);
#32214=ORIENTED_EDGE('',*,*,#24320,.T.);
#32215=ORIENTED_EDGE('',*,*,#24321,.T.);
#32216=ORIENTED_EDGE('',*,*,#24322,.T.);
#32217=ORIENTED_EDGE('',*,*,#24323,.T.);
#32218=ORIENTED_EDGE('',*,*,#24324,.T.);
#32219=ORIENTED_EDGE('',*,*,#24325,.T.);
#32220=ORIENTED_EDGE('',*,*,#24326,.T.);
#32221=ORIENTED_EDGE('',*,*,#24327,.T.);
#32222=ORIENTED_EDGE('',*,*,#24328,.T.);
#32223=ORIENTED_EDGE('',*,*,#24329,.T.);
#32224=ORIENTED_EDGE('',*,*,#24330,.T.);
#32225=ORIENTED_EDGE('',*,*,#24331,.T.);
#32226=ORIENTED_EDGE('',*,*,#24332,.T.);
#32227=ORIENTED_EDGE('',*,*,#24333,.T.);
#32228=ORIENTED_EDGE('',*,*,#24334,.T.);
#32229=ORIENTED_EDGE('',*,*,#24335,.T.);
#32230=ORIENTED_EDGE('',*,*,#24336,.T.);
#32231=ORIENTED_EDGE('',*,*,#24337,.T.);
#32232=ORIENTED_EDGE('',*,*,#24338,.T.);
#32233=ORIENTED_EDGE('',*,*,#24339,.T.);
#32234=ORIENTED_EDGE('',*,*,#24340,.T.);
#32235=ORIENTED_EDGE('',*,*,#24341,.T.);
#32236=ORIENTED_EDGE('',*,*,#24342,.T.);
#32237=ORIENTED_EDGE('',*,*,#24343,.T.);
#32238=ORIENTED_EDGE('',*,*,#24344,.T.);
#32239=ORIENTED_EDGE('',*,*,#24345,.T.);
#32240=ORIENTED_EDGE('',*,*,#24346,.T.);
#32241=ORIENTED_EDGE('',*,*,#24347,.T.);
#32242=ORIENTED_EDGE('',*,*,#24348,.T.);
#32243=ORIENTED_EDGE('',*,*,#24349,.T.);
#32244=ORIENTED_EDGE('',*,*,#24350,.T.);
#32245=ORIENTED_EDGE('',*,*,#24351,.T.);
#32246=ORIENTED_EDGE('',*,*,#24352,.T.);
#32247=ORIENTED_EDGE('',*,*,#24353,.T.);
#32248=ORIENTED_EDGE('',*,*,#24354,.T.);
#32249=ORIENTED_EDGE('',*,*,#24355,.T.);
#32250=ORIENTED_EDGE('',*,*,#24356,.T.);
#32251=ORIENTED_EDGE('',*,*,#24357,.T.);
#32252=ORIENTED_EDGE('',*,*,#24358,.T.);
#32253=ORIENTED_EDGE('',*,*,#24359,.T.);
#32254=ORIENTED_EDGE('',*,*,#24360,.T.);
#32255=ORIENTED_EDGE('',*,*,#24361,.T.);
#32256=ORIENTED_EDGE('',*,*,#24362,.T.);
#32257=ORIENTED_EDGE('',*,*,#24363,.T.);
#32258=ORIENTED_EDGE('',*,*,#24364,.T.);
#32259=ORIENTED_EDGE('',*,*,#24365,.T.);
#32260=ORIENTED_EDGE('',*,*,#24366,.T.);
#32261=ORIENTED_EDGE('',*,*,#24367,.T.);
#32262=ORIENTED_EDGE('',*,*,#24368,.T.);
#32263=ORIENTED_EDGE('',*,*,#24369,.T.);
#32264=ORIENTED_EDGE('',*,*,#24370,.T.);
#32265=ORIENTED_EDGE('',*,*,#24371,.T.);
#32266=ORIENTED_EDGE('',*,*,#24372,.T.);
#32267=ORIENTED_EDGE('',*,*,#24373,.T.);
#32268=ORIENTED_EDGE('',*,*,#24374,.T.);
#32269=ORIENTED_EDGE('',*,*,#24375,.T.);
#32270=ORIENTED_EDGE('',*,*,#24376,.T.);
#32271=ORIENTED_EDGE('',*,*,#24377,.T.);
#32272=ORIENTED_EDGE('',*,*,#24378,.T.);
#32273=ORIENTED_EDGE('',*,*,#24379,.T.);
#32274=ORIENTED_EDGE('',*,*,#24380,.T.);
#32275=ORIENTED_EDGE('',*,*,#24381,.T.);
#32276=ORIENTED_EDGE('',*,*,#24382,.T.);
#32277=ORIENTED_EDGE('',*,*,#24383,.T.);
#32278=ORIENTED_EDGE('',*,*,#24384,.T.);
#32279=ORIENTED_EDGE('',*,*,#24385,.T.);
#32280=ORIENTED_EDGE('',*,*,#24386,.T.);
#32281=ORIENTED_EDGE('',*,*,#24387,.T.);
#32282=ORIENTED_EDGE('',*,*,#24388,.T.);
#32283=ORIENTED_EDGE('',*,*,#24389,.T.);
#32284=ORIENTED_EDGE('',*,*,#24390,.T.);
#32285=ORIENTED_EDGE('',*,*,#24391,.T.);
#32286=ORIENTED_EDGE('',*,*,#24392,.T.);
#32287=ORIENTED_EDGE('',*,*,#24393,.T.);
#32288=ORIENTED_EDGE('',*,*,#24394,.T.);
#32289=ORIENTED_EDGE('',*,*,#24395,.T.);
#32290=ORIENTED_EDGE('',*,*,#24396,.T.);
#32291=ORIENTED_EDGE('',*,*,#24397,.T.);
#32292=ORIENTED_EDGE('',*,*,#24398,.T.);
#32293=ORIENTED_EDGE('',*,*,#24399,.T.);
#32294=ORIENTED_EDGE('',*,*,#24400,.T.);
#32295=ORIENTED_EDGE('',*,*,#24401,.T.);
#32296=ORIENTED_EDGE('',*,*,#24402,.T.);
#32297=ORIENTED_EDGE('',*,*,#24403,.T.);
#32298=ORIENTED_EDGE('',*,*,#24404,.T.);
#32299=ORIENTED_EDGE('',*,*,#24405,.T.);
#32300=ORIENTED_EDGE('',*,*,#24406,.T.);
#32301=ORIENTED_EDGE('',*,*,#24407,.T.);
#32302=ORIENTED_EDGE('',*,*,#24408,.T.);
#32303=ORIENTED_EDGE('',*,*,#24409,.T.);
#32304=ORIENTED_EDGE('',*,*,#24410,.T.);
#32305=ORIENTED_EDGE('',*,*,#24411,.T.);
#32306=ORIENTED_EDGE('',*,*,#24412,.T.);
#32307=ORIENTED_EDGE('',*,*,#24413,.T.);
#32308=ORIENTED_EDGE('',*,*,#24414,.T.);
#32309=ORIENTED_EDGE('',*,*,#24415,.T.);
#32310=ORIENTED_EDGE('',*,*,#24416,.T.);
#32311=ORIENTED_EDGE('',*,*,#24417,.T.);
#32312=ORIENTED_EDGE('',*,*,#24418,.T.);
#32313=ORIENTED_EDGE('',*,*,#24419,.T.);
#32314=ORIENTED_EDGE('',*,*,#24420,.T.);
#32315=ORIENTED_EDGE('',*,*,#24421,.T.);
#32316=ORIENTED_EDGE('',*,*,#24422,.T.);
#32317=ORIENTED_EDGE('',*,*,#24423,.T.);
#32318=ORIENTED_EDGE('',*,*,#24424,.T.);
#32319=ORIENTED_EDGE('',*,*,#24425,.T.);
#32320=ORIENTED_EDGE('',*,*,#24426,.T.);
#32321=ORIENTED_EDGE('',*,*,#24427,.T.);
#32322=ORIENTED_EDGE('',*,*,#24428,.T.);
#32323=ORIENTED_EDGE('',*,*,#24429,.T.);
#32324=ORIENTED_EDGE('',*,*,#24430,.T.);
#32325=ORIENTED_EDGE('',*,*,#24431,.T.);
#32326=ORIENTED_EDGE('',*,*,#24432,.T.);
#32327=ORIENTED_EDGE('',*,*,#24433,.T.);
#32328=ORIENTED_EDGE('',*,*,#24434,.T.);
#32329=ORIENTED_EDGE('',*,*,#24435,.T.);
#32330=ORIENTED_EDGE('',*,*,#24436,.T.);
#32331=ORIENTED_EDGE('',*,*,#24437,.T.);
#32332=ORIENTED_EDGE('',*,*,#24438,.T.);
#32333=ORIENTED_EDGE('',*,*,#24439,.T.);
#32334=ORIENTED_EDGE('',*,*,#24440,.T.);
#32335=ORIENTED_EDGE('',*,*,#24441,.T.);
#32336=ORIENTED_EDGE('',*,*,#24442,.T.);
#32337=ORIENTED_EDGE('',*,*,#24443,.T.);
#32338=ORIENTED_EDGE('',*,*,#24444,.T.);
#32339=ORIENTED_EDGE('',*,*,#24445,.T.);
#32340=ORIENTED_EDGE('',*,*,#24446,.T.);
#32341=ORIENTED_EDGE('',*,*,#24447,.T.);
#32342=ORIENTED_EDGE('',*,*,#24448,.T.);
#32343=ORIENTED_EDGE('',*,*,#24449,.T.);
#32344=ORIENTED_EDGE('',*,*,#24450,.T.);
#32345=ORIENTED_EDGE('',*,*,#24451,.T.);
#32346=ORIENTED_EDGE('',*,*,#24452,.T.);
#32347=ORIENTED_EDGE('',*,*,#24453,.T.);
#32348=ORIENTED_EDGE('',*,*,#24454,.T.);
#32349=ORIENTED_EDGE('',*,*,#24455,.T.);
#32350=ORIENTED_EDGE('',*,*,#24456,.T.);
#32351=ORIENTED_EDGE('',*,*,#24457,.T.);
#32352=ORIENTED_EDGE('',*,*,#24458,.T.);
#32353=ORIENTED_EDGE('',*,*,#24459,.T.);
#32354=ORIENTED_EDGE('',*,*,#24460,.T.);
#32355=ORIENTED_EDGE('',*,*,#24461,.T.);
#32356=ORIENTED_EDGE('',*,*,#24462,.T.);
#32357=ORIENTED_EDGE('',*,*,#24463,.T.);
#32358=ORIENTED_EDGE('',*,*,#24464,.T.);
#32359=ORIENTED_EDGE('',*,*,#24465,.T.);
#32360=ORIENTED_EDGE('',*,*,#24466,.T.);
#32361=ORIENTED_EDGE('',*,*,#24467,.T.);
#32362=ORIENTED_EDGE('',*,*,#24468,.T.);
#32363=ORIENTED_EDGE('',*,*,#24469,.T.);
#32364=ORIENTED_EDGE('',*,*,#24470,.T.);
#32365=ORIENTED_EDGE('',*,*,#24471,.T.);
#32366=ORIENTED_EDGE('',*,*,#24472,.T.);
#32367=ORIENTED_EDGE('',*,*,#24473,.T.);
#32368=ORIENTED_EDGE('',*,*,#24474,.T.);
#32369=ORIENTED_EDGE('',*,*,#24475,.T.);
#32370=ORIENTED_EDGE('',*,*,#24476,.T.);
#32371=ORIENTED_EDGE('',*,*,#24477,.T.);
#32372=ORIENTED_EDGE('',*,*,#24478,.T.);
#32373=ORIENTED_EDGE('',*,*,#24479,.T.);
#32374=ORIENTED_EDGE('',*,*,#24480,.T.);
#32375=ORIENTED_EDGE('',*,*,#24481,.T.);
#32376=ORIENTED_EDGE('',*,*,#24482,.T.);
#32377=ORIENTED_EDGE('',*,*,#24483,.T.);
#32378=ORIENTED_EDGE('',*,*,#24484,.T.);
#32379=ORIENTED_EDGE('',*,*,#24485,.T.);
#32380=ORIENTED_EDGE('',*,*,#24486,.T.);
#32381=ORIENTED_EDGE('',*,*,#24487,.T.);
#32382=ORIENTED_EDGE('',*,*,#24488,.T.);
#32383=ORIENTED_EDGE('',*,*,#24489,.T.);
#32384=ORIENTED_EDGE('',*,*,#24490,.T.);
#32385=ORIENTED_EDGE('',*,*,#24491,.T.);
#32386=ORIENTED_EDGE('',*,*,#24492,.T.);
#32387=ORIENTED_EDGE('',*,*,#24493,.T.);
#32388=ORIENTED_EDGE('',*,*,#24494,.T.);
#32389=ORIENTED_EDGE('',*,*,#24495,.T.);
#32390=ORIENTED_EDGE('',*,*,#24496,.T.);
#32391=ORIENTED_EDGE('',*,*,#24497,.T.);
#32392=ORIENTED_EDGE('',*,*,#24498,.T.);
#32393=ORIENTED_EDGE('',*,*,#24499,.T.);
#32394=ORIENTED_EDGE('',*,*,#24500,.T.);
#32395=ORIENTED_EDGE('',*,*,#24501,.T.);
#32396=ORIENTED_EDGE('',*,*,#24502,.T.);
#32397=ORIENTED_EDGE('',*,*,#24503,.T.);
#32398=ORIENTED_EDGE('',*,*,#24504,.T.);
#32399=ORIENTED_EDGE('',*,*,#24505,.T.);
#32400=ORIENTED_EDGE('',*,*,#24506,.T.);
#32401=ORIENTED_EDGE('',*,*,#24507,.T.);
#32402=ORIENTED_EDGE('',*,*,#24508,.T.);
#32403=ORIENTED_EDGE('',*,*,#24509,.T.);
#32404=ORIENTED_EDGE('',*,*,#24510,.T.);
#32405=ORIENTED_EDGE('',*,*,#24511,.T.);
#32406=ORIENTED_EDGE('',*,*,#24512,.T.);
#32407=ORIENTED_EDGE('',*,*,#24513,.T.);
#32408=ORIENTED_EDGE('',*,*,#24514,.T.);
#32409=ORIENTED_EDGE('',*,*,#24515,.T.);
#32410=ORIENTED_EDGE('',*,*,#24516,.T.);
#32411=ORIENTED_EDGE('',*,*,#24517,.T.);
#32412=ORIENTED_EDGE('',*,*,#24518,.T.);
#32413=ORIENTED_EDGE('',*,*,#24519,.T.);
#32414=ORIENTED_EDGE('',*,*,#24520,.T.);
#32415=ORIENTED_EDGE('',*,*,#24521,.T.);
#32416=ORIENTED_EDGE('',*,*,#24522,.T.);
#32417=ORIENTED_EDGE('',*,*,#24523,.T.);
#32418=ORIENTED_EDGE('',*,*,#24524,.T.);
#32419=ORIENTED_EDGE('',*,*,#24525,.T.);
#32420=ORIENTED_EDGE('',*,*,#24526,.T.);
#32421=ORIENTED_EDGE('',*,*,#24527,.T.);
#32422=ORIENTED_EDGE('',*,*,#24528,.T.);
#32423=ORIENTED_EDGE('',*,*,#24529,.T.);
#32424=ORIENTED_EDGE('',*,*,#24530,.T.);
#32425=ORIENTED_EDGE('',*,*,#24531,.T.);
#32426=ORIENTED_EDGE('',*,*,#24532,.T.);
#32427=ORIENTED_EDGE('',*,*,#24533,.T.);
#32428=ORIENTED_EDGE('',*,*,#24534,.T.);
#32429=ORIENTED_EDGE('',*,*,#24535,.T.);
#32430=ORIENTED_EDGE('',*,*,#24536,.T.);
#32431=ORIENTED_EDGE('',*,*,#24537,.T.);
#32432=ORIENTED_EDGE('',*,*,#24538,.T.);
#32433=ORIENTED_EDGE('',*,*,#24539,.T.);
#32434=ORIENTED_EDGE('',*,*,#24540,.T.);
#32435=ORIENTED_EDGE('',*,*,#24541,.T.);
#32436=ORIENTED_EDGE('',*,*,#24542,.T.);
#32437=ORIENTED_EDGE('',*,*,#24543,.T.);
#32438=ORIENTED_EDGE('',*,*,#24544,.T.);
#32439=ORIENTED_EDGE('',*,*,#24545,.T.);
#32440=ORIENTED_EDGE('',*,*,#24546,.T.);
#32441=ORIENTED_EDGE('',*,*,#24547,.T.);
#32442=ORIENTED_EDGE('',*,*,#24548,.T.);
#32443=ORIENTED_EDGE('',*,*,#24549,.T.);
#32444=ORIENTED_EDGE('',*,*,#24550,.T.);
#32445=ORIENTED_EDGE('',*,*,#24551,.T.);
#32446=ORIENTED_EDGE('',*,*,#24552,.T.);
#32447=ORIENTED_EDGE('',*,*,#24553,.T.);
#32448=ORIENTED_EDGE('',*,*,#24554,.T.);
#32449=ORIENTED_EDGE('',*,*,#24555,.T.);
#32450=ORIENTED_EDGE('',*,*,#24556,.T.);
#32451=ORIENTED_EDGE('',*,*,#24557,.T.);
#32452=ORIENTED_EDGE('',*,*,#24558,.T.);
#32453=ORIENTED_EDGE('',*,*,#24559,.T.);
#32454=ORIENTED_EDGE('',*,*,#24560,.T.);
#32455=ORIENTED_EDGE('',*,*,#24561,.T.);
#32456=ORIENTED_EDGE('',*,*,#24562,.T.);
#32457=ORIENTED_EDGE('',*,*,#24563,.T.);
#32458=ORIENTED_EDGE('',*,*,#24564,.T.);
#32459=ORIENTED_EDGE('',*,*,#24565,.T.);
#32460=ORIENTED_EDGE('',*,*,#24566,.T.);
#32461=ORIENTED_EDGE('',*,*,#24567,.T.);
#32462=ORIENTED_EDGE('',*,*,#24568,.T.);
#32463=ORIENTED_EDGE('',*,*,#24569,.T.);
#32464=ORIENTED_EDGE('',*,*,#24570,.T.);
#32465=ORIENTED_EDGE('',*,*,#24571,.T.);
#32466=ORIENTED_EDGE('',*,*,#24572,.T.);
#32467=ORIENTED_EDGE('',*,*,#24573,.T.);
#32468=ORIENTED_EDGE('',*,*,#24574,.T.);
#32469=ORIENTED_EDGE('',*,*,#24575,.T.);
#32470=ORIENTED_EDGE('',*,*,#24576,.T.);
#32471=ORIENTED_EDGE('',*,*,#24577,.T.);
#32472=ORIENTED_EDGE('',*,*,#24578,.T.);
#32473=ORIENTED_EDGE('',*,*,#24579,.T.);
#32474=ORIENTED_EDGE('',*,*,#24580,.T.);
#32475=ORIENTED_EDGE('',*,*,#24581,.T.);
#32476=ORIENTED_EDGE('',*,*,#24582,.T.);
#32477=ORIENTED_EDGE('',*,*,#24583,.T.);
#32478=ORIENTED_EDGE('',*,*,#24584,.T.);
#32479=ORIENTED_EDGE('',*,*,#24585,.T.);
#32480=ORIENTED_EDGE('',*,*,#24586,.T.);
#32481=ORIENTED_EDGE('',*,*,#24587,.T.);
#32482=ORIENTED_EDGE('',*,*,#24588,.T.);
#32483=ORIENTED_EDGE('',*,*,#24589,.T.);
#32484=ORIENTED_EDGE('',*,*,#24590,.T.);
#32485=ORIENTED_EDGE('',*,*,#24591,.T.);
#32486=ORIENTED_EDGE('',*,*,#24592,.T.);
#32487=ORIENTED_EDGE('',*,*,#24593,.T.);
#32488=ORIENTED_EDGE('',*,*,#24594,.T.);
#32489=ORIENTED_EDGE('',*,*,#24595,.T.);
#32490=ORIENTED_EDGE('',*,*,#24596,.T.);
#32491=ORIENTED_EDGE('',*,*,#24597,.T.);
#32492=ORIENTED_EDGE('',*,*,#24598,.T.);
#32493=ORIENTED_EDGE('',*,*,#24599,.T.);
#32494=ORIENTED_EDGE('',*,*,#24600,.T.);
#32495=ORIENTED_EDGE('',*,*,#24601,.T.);
#32496=ORIENTED_EDGE('',*,*,#24602,.T.);
#32497=ORIENTED_EDGE('',*,*,#24603,.T.);
#32498=ORIENTED_EDGE('',*,*,#24604,.T.);
#32499=ORIENTED_EDGE('',*,*,#24605,.T.);
#32500=ORIENTED_EDGE('',*,*,#24606,.T.);
#32501=ORIENTED_EDGE('',*,*,#24607,.T.);
#32502=ORIENTED_EDGE('',*,*,#24608,.T.);
#32503=ORIENTED_EDGE('',*,*,#24609,.T.);
#32504=ORIENTED_EDGE('',*,*,#24610,.T.);
#32505=ORIENTED_EDGE('',*,*,#24611,.T.);
#32506=ORIENTED_EDGE('',*,*,#24612,.T.);
#32507=ORIENTED_EDGE('',*,*,#24613,.T.);
#32508=ORIENTED_EDGE('',*,*,#24614,.T.);
#32509=ORIENTED_EDGE('',*,*,#24615,.T.);
#32510=ORIENTED_EDGE('',*,*,#24616,.T.);
#32511=ORIENTED_EDGE('',*,*,#24617,.T.);
#32512=ORIENTED_EDGE('',*,*,#24618,.T.);
#32513=ORIENTED_EDGE('',*,*,#24619,.T.);
#32514=ORIENTED_EDGE('',*,*,#24620,.T.);
#32515=ORIENTED_EDGE('',*,*,#24621,.T.);
#32516=ORIENTED_EDGE('',*,*,#24622,.T.);
#32517=ORIENTED_EDGE('',*,*,#24623,.T.);
#32518=ORIENTED_EDGE('',*,*,#24624,.T.);
#32519=ORIENTED_EDGE('',*,*,#24625,.T.);
#32520=ORIENTED_EDGE('',*,*,#24626,.T.);
#32521=ORIENTED_EDGE('',*,*,#24627,.T.);
#32522=ORIENTED_EDGE('',*,*,#24628,.T.);
#32523=ORIENTED_EDGE('',*,*,#24629,.T.);
#32524=ORIENTED_EDGE('',*,*,#24630,.T.);
#32525=ORIENTED_EDGE('',*,*,#24631,.T.);
#32526=ORIENTED_EDGE('',*,*,#24632,.T.);
#32527=ORIENTED_EDGE('',*,*,#24633,.T.);
#32528=ORIENTED_EDGE('',*,*,#24634,.T.);
#32529=ORIENTED_EDGE('',*,*,#24635,.T.);
#32530=ORIENTED_EDGE('',*,*,#24636,.T.);
#32531=ORIENTED_EDGE('',*,*,#24637,.T.);
#32532=ORIENTED_EDGE('',*,*,#24638,.T.);
#32533=ORIENTED_EDGE('',*,*,#24639,.T.);
#32534=ORIENTED_EDGE('',*,*,#24640,.T.);
#32535=ORIENTED_EDGE('',*,*,#24641,.T.);
#32536=ORIENTED_EDGE('',*,*,#24642,.T.);
#32537=ORIENTED_EDGE('',*,*,#24643,.T.);
#32538=ORIENTED_EDGE('',*,*,#24644,.T.);
#32539=ORIENTED_EDGE('',*,*,#24645,.T.);
#32540=ORIENTED_EDGE('',*,*,#24646,.T.);
#32541=ORIENTED_EDGE('',*,*,#24647,.T.);
#32542=ORIENTED_EDGE('',*,*,#24648,.T.);
#32543=ORIENTED_EDGE('',*,*,#24649,.T.);
#32544=ORIENTED_EDGE('',*,*,#24650,.T.);
#32545=ORIENTED_EDGE('',*,*,#24651,.T.);
#32546=ORIENTED_EDGE('',*,*,#24652,.T.);
#32547=ORIENTED_EDGE('',*,*,#24653,.T.);
#32548=ORIENTED_EDGE('',*,*,#24654,.T.);
#32549=ORIENTED_EDGE('',*,*,#24655,.T.);
#32550=ORIENTED_EDGE('',*,*,#24656,.T.);
#32551=ORIENTED_EDGE('',*,*,#24657,.T.);
#32552=ORIENTED_EDGE('',*,*,#24658,.T.);
#32553=ORIENTED_EDGE('',*,*,#24659,.T.);
#32554=ORIENTED_EDGE('',*,*,#24660,.T.);
#32555=ORIENTED_EDGE('',*,*,#24661,.T.);
#32556=ORIENTED_EDGE('',*,*,#24662,.T.);
#32557=ORIENTED_EDGE('',*,*,#24663,.T.);
#32558=ORIENTED_EDGE('',*,*,#24664,.T.);
#32559=ORIENTED_EDGE('',*,*,#24665,.T.);
#32560=ORIENTED_EDGE('',*,*,#24666,.T.);
#32561=ORIENTED_EDGE('',*,*,#24667,.T.);
#32562=ORIENTED_EDGE('',*,*,#24668,.T.);
#32563=ORIENTED_EDGE('',*,*,#24669,.T.);
#32564=ORIENTED_EDGE('',*,*,#24670,.T.);
#32565=ORIENTED_EDGE('',*,*,#24671,.T.);
#32566=ORIENTED_EDGE('',*,*,#24672,.T.);
#32567=ORIENTED_EDGE('',*,*,#24673,.T.);
#32568=ORIENTED_EDGE('',*,*,#24674,.T.);
#32569=ORIENTED_EDGE('',*,*,#24675,.T.);
#32570=ORIENTED_EDGE('',*,*,#24676,.T.);
#32571=ORIENTED_EDGE('',*,*,#24677,.T.);
#32572=ORIENTED_EDGE('',*,*,#24678,.T.);
#32573=ORIENTED_EDGE('',*,*,#24679,.T.);
#32574=ORIENTED_EDGE('',*,*,#24680,.T.);
#32575=ORIENTED_EDGE('',*,*,#24681,.T.);
#32576=ORIENTED_EDGE('',*,*,#24682,.T.);
#32577=ORIENTED_EDGE('',*,*,#24683,.T.);
#32578=ORIENTED_EDGE('',*,*,#24684,.T.);
#32579=ORIENTED_EDGE('',*,*,#24685,.T.);
#32580=ORIENTED_EDGE('',*,*,#24686,.T.);
#32581=ORIENTED_EDGE('',*,*,#24687,.T.);
#32582=ORIENTED_EDGE('',*,*,#24688,.T.);
#32583=ORIENTED_EDGE('',*,*,#24689,.T.);
#32584=ORIENTED_EDGE('',*,*,#24690,.T.);
#32585=ORIENTED_EDGE('',*,*,#24691,.T.);
#32586=ORIENTED_EDGE('',*,*,#24692,.T.);
#32587=ORIENTED_EDGE('',*,*,#24693,.T.);
#32588=ORIENTED_EDGE('',*,*,#24694,.T.);
#32589=ORIENTED_EDGE('',*,*,#24695,.T.);
#32590=ORIENTED_EDGE('',*,*,#24696,.T.);
#32591=ORIENTED_EDGE('',*,*,#24697,.T.);
#32592=ORIENTED_EDGE('',*,*,#24698,.T.);
#32593=ORIENTED_EDGE('',*,*,#24699,.T.);
#32594=ORIENTED_EDGE('',*,*,#24700,.T.);
#32595=ORIENTED_EDGE('',*,*,#24701,.T.);
#32596=ORIENTED_EDGE('',*,*,#24702,.T.);
#32597=ORIENTED_EDGE('',*,*,#24703,.T.);
#32598=ORIENTED_EDGE('',*,*,#24704,.T.);
#32599=ORIENTED_EDGE('',*,*,#24705,.T.);
#32600=ORIENTED_EDGE('',*,*,#24706,.T.);
#32601=ORIENTED_EDGE('',*,*,#24707,.T.);
#32602=ORIENTED_EDGE('',*,*,#24708,.T.);
#32603=ORIENTED_EDGE('',*,*,#24709,.T.);
#32604=ORIENTED_EDGE('',*,*,#24710,.T.);
#32605=ORIENTED_EDGE('',*,*,#24711,.T.);
#32606=ORIENTED_EDGE('',*,*,#24712,.T.);
#32607=ORIENTED_EDGE('',*,*,#24713,.T.);
#32608=ORIENTED_EDGE('',*,*,#24714,.T.);
#32609=ORIENTED_EDGE('',*,*,#24715,.T.);
#32610=ORIENTED_EDGE('',*,*,#24716,.T.);
#32611=ORIENTED_EDGE('',*,*,#24717,.T.);
#32612=ORIENTED_EDGE('',*,*,#24718,.T.);
#32613=ORIENTED_EDGE('',*,*,#24719,.T.);
#32614=ORIENTED_EDGE('',*,*,#24720,.T.);
#32615=ORIENTED_EDGE('',*,*,#24721,.T.);
#32616=ORIENTED_EDGE('',*,*,#24722,.T.);
#32617=ORIENTED_EDGE('',*,*,#24723,.T.);
#32618=ORIENTED_EDGE('',*,*,#24724,.T.);
#32619=ORIENTED_EDGE('',*,*,#24725,.T.);
#32620=ORIENTED_EDGE('',*,*,#24726,.T.);
#32621=ORIENTED_EDGE('',*,*,#24727,.T.);
#32622=ORIENTED_EDGE('',*,*,#24728,.T.);
#32623=ORIENTED_EDGE('',*,*,#24729,.T.);
#32624=ORIENTED_EDGE('',*,*,#24730,.T.);
#32625=ORIENTED_EDGE('',*,*,#24731,.T.);
#32626=ORIENTED_EDGE('',*,*,#24732,.T.);
#32627=ORIENTED_EDGE('',*,*,#24733,.T.);
#32628=ORIENTED_EDGE('',*,*,#24734,.T.);
#32629=ORIENTED_EDGE('',*,*,#24735,.T.);
#32630=ORIENTED_EDGE('',*,*,#24736,.T.);
#32631=ORIENTED_EDGE('',*,*,#24737,.T.);
#32632=ORIENTED_EDGE('',*,*,#24738,.T.);
#32633=ORIENTED_EDGE('',*,*,#24739,.T.);
#32634=ORIENTED_EDGE('',*,*,#24740,.T.);
#32635=ORIENTED_EDGE('',*,*,#24741,.T.);
#32636=ORIENTED_EDGE('',*,*,#24742,.T.);
#32637=ORIENTED_EDGE('',*,*,#24743,.T.);
#32638=ORIENTED_EDGE('',*,*,#24744,.T.);
#32639=ORIENTED_EDGE('',*,*,#24745,.T.);
#32640=ORIENTED_EDGE('',*,*,#24746,.T.);
#32641=ORIENTED_EDGE('',*,*,#24747,.T.);
#32642=ORIENTED_EDGE('',*,*,#24748,.T.);
#32643=ORIENTED_EDGE('',*,*,#24749,.T.);
#32644=ORIENTED_EDGE('',*,*,#24750,.T.);
#32645=ORIENTED_EDGE('',*,*,#24751,.T.);
#32646=ORIENTED_EDGE('',*,*,#24752,.T.);
#32647=ORIENTED_EDGE('',*,*,#24753,.T.);
#32648=ORIENTED_EDGE('',*,*,#24754,.T.);
#32649=ORIENTED_EDGE('',*,*,#24755,.T.);
#32650=ORIENTED_EDGE('',*,*,#24756,.T.);
#32651=ORIENTED_EDGE('',*,*,#24757,.T.);
#32652=ORIENTED_EDGE('',*,*,#24758,.T.);
#32653=ORIENTED_EDGE('',*,*,#24759,.T.);
#32654=ORIENTED_EDGE('',*,*,#24760,.T.);
#32655=ORIENTED_EDGE('',*,*,#24761,.T.);
#32656=ORIENTED_EDGE('',*,*,#24762,.T.);
#32657=ORIENTED_EDGE('',*,*,#24763,.T.);
#32658=ORIENTED_EDGE('',*,*,#24764,.T.);
#32659=ORIENTED_EDGE('',*,*,#24765,.T.);
#32660=ORIENTED_EDGE('',*,*,#24766,.T.);
#32661=ORIENTED_EDGE('',*,*,#24767,.T.);
#32662=ORIENTED_EDGE('',*,*,#24768,.T.);
#32663=ORIENTED_EDGE('',*,*,#24769,.T.);
#32664=ORIENTED_EDGE('',*,*,#24770,.T.);
#32665=ORIENTED_EDGE('',*,*,#24771,.T.);
#32666=ORIENTED_EDGE('',*,*,#24772,.T.);
#32667=ORIENTED_EDGE('',*,*,#24773,.T.);
#32668=ORIENTED_EDGE('',*,*,#24774,.T.);
#32669=ORIENTED_EDGE('',*,*,#24775,.T.);
#32670=ORIENTED_EDGE('',*,*,#24776,.T.);
#32671=ORIENTED_EDGE('',*,*,#24777,.T.);
#32672=ORIENTED_EDGE('',*,*,#24778,.T.);
#32673=ORIENTED_EDGE('',*,*,#24779,.T.);
#32674=ORIENTED_EDGE('',*,*,#24780,.T.);
#32675=ORIENTED_EDGE('',*,*,#24781,.T.);
#32676=ORIENTED_EDGE('',*,*,#24782,.T.);
#32677=ORIENTED_EDGE('',*,*,#24783,.T.);
#32678=ORIENTED_EDGE('',*,*,#24784,.T.);
#32679=ORIENTED_EDGE('',*,*,#24785,.T.);
#32680=ORIENTED_EDGE('',*,*,#24786,.T.);
#32681=ORIENTED_EDGE('',*,*,#24787,.T.);
#32682=ORIENTED_EDGE('',*,*,#24788,.T.);
#32683=ORIENTED_EDGE('',*,*,#24789,.T.);
#32684=ORIENTED_EDGE('',*,*,#24790,.T.);
#32685=ORIENTED_EDGE('',*,*,#24791,.T.);
#32686=ORIENTED_EDGE('',*,*,#24792,.T.);
#32687=ORIENTED_EDGE('',*,*,#24793,.T.);
#32688=ORIENTED_EDGE('',*,*,#24794,.T.);
#32689=ORIENTED_EDGE('',*,*,#24795,.T.);
#32690=ORIENTED_EDGE('',*,*,#24796,.T.);
#32691=ORIENTED_EDGE('',*,*,#24797,.T.);
#32692=ORIENTED_EDGE('',*,*,#24798,.T.);
#32693=ORIENTED_EDGE('',*,*,#24799,.T.);
#32694=ORIENTED_EDGE('',*,*,#24800,.T.);
#32695=ORIENTED_EDGE('',*,*,#24801,.T.);
#32696=ORIENTED_EDGE('',*,*,#24802,.T.);
#32697=ORIENTED_EDGE('',*,*,#24803,.T.);
#32698=ORIENTED_EDGE('',*,*,#24804,.T.);
#32699=ORIENTED_EDGE('',*,*,#24805,.T.);
#32700=ORIENTED_EDGE('',*,*,#24806,.T.);
#32701=ORIENTED_EDGE('',*,*,#24807,.T.);
#32702=ORIENTED_EDGE('',*,*,#24808,.T.);
#32703=ORIENTED_EDGE('',*,*,#24809,.T.);
#32704=ORIENTED_EDGE('',*,*,#24810,.T.);
#32705=ORIENTED_EDGE('',*,*,#24811,.T.);
#32706=ORIENTED_EDGE('',*,*,#24812,.T.);
#32707=ORIENTED_EDGE('',*,*,#24813,.T.);
#32708=ORIENTED_EDGE('',*,*,#24814,.T.);
#32709=ORIENTED_EDGE('',*,*,#24815,.T.);
#32710=ORIENTED_EDGE('',*,*,#24816,.T.);
#32711=ORIENTED_EDGE('',*,*,#24817,.T.);
#32712=ORIENTED_EDGE('',*,*,#24818,.T.);
#32713=ORIENTED_EDGE('',*,*,#24819,.T.);
#32714=ORIENTED_EDGE('',*,*,#24820,.T.);
#32715=ORIENTED_EDGE('',*,*,#24821,.T.);
#32716=ORIENTED_EDGE('',*,*,#24822,.T.);
#32717=ORIENTED_EDGE('',*,*,#24823,.T.);
#32718=ORIENTED_EDGE('',*,*,#24824,.T.);
#32719=ORIENTED_EDGE('',*,*,#24825,.T.);
#32720=ORIENTED_EDGE('',*,*,#24826,.T.);
#32721=ORIENTED_EDGE('',*,*,#24827,.T.);
#32722=ORIENTED_EDGE('',*,*,#24828,.T.);
#32723=ORIENTED_EDGE('',*,*,#24829,.T.);
#32724=ORIENTED_EDGE('',*,*,#24830,.T.);
#32725=ORIENTED_EDGE('',*,*,#24831,.T.);
#32726=ORIENTED_EDGE('',*,*,#24832,.T.);
#32727=ORIENTED_EDGE('',*,*,#24833,.T.);
#32728=ORIENTED_EDGE('',*,*,#24834,.T.);
#32729=ORIENTED_EDGE('',*,*,#24835,.T.);
#32730=ORIENTED_EDGE('',*,*,#24836,.T.);
#32731=ORIENTED_EDGE('',*,*,#24837,.T.);
#32732=ORIENTED_EDGE('',*,*,#24838,.T.);
#32733=ORIENTED_EDGE('',*,*,#24839,.T.);
#32734=ORIENTED_EDGE('',*,*,#24840,.T.);
#32735=ORIENTED_EDGE('',*,*,#24841,.T.);
#32736=ORIENTED_EDGE('',*,*,#24842,.T.);
#32737=ORIENTED_EDGE('',*,*,#24843,.T.);
#32738=ORIENTED_EDGE('',*,*,#24844,.T.);
#32739=ORIENTED_EDGE('',*,*,#24845,.T.);
#32740=ORIENTED_EDGE('',*,*,#24846,.T.);
#32741=ORIENTED_EDGE('',*,*,#24847,.T.);
#32742=ORIENTED_EDGE('',*,*,#24848,.T.);
#32743=ORIENTED_EDGE('',*,*,#24849,.T.);
#32744=ORIENTED_EDGE('',*,*,#24850,.T.);
#32745=ORIENTED_EDGE('',*,*,#24851,.T.);
#32746=ORIENTED_EDGE('',*,*,#24852,.T.);
#32747=ORIENTED_EDGE('',*,*,#24853,.T.);
#32748=ORIENTED_EDGE('',*,*,#24854,.T.);
#32749=ORIENTED_EDGE('',*,*,#24855,.T.);
#32750=ORIENTED_EDGE('',*,*,#24856,.T.);
#32751=ORIENTED_EDGE('',*,*,#24857,.T.);
#32752=ORIENTED_EDGE('',*,*,#24858,.T.);
#32753=ORIENTED_EDGE('',*,*,#24859,.T.);
#32754=ORIENTED_EDGE('',*,*,#24860,.T.);
#32755=ORIENTED_EDGE('',*,*,#24861,.T.);
#32756=ORIENTED_EDGE('',*,*,#24862,.T.);
#32757=ORIENTED_EDGE('',*,*,#24863,.T.);
#32758=ORIENTED_EDGE('',*,*,#24864,.T.);
#32759=ORIENTED_EDGE('',*,*,#24865,.T.);
#32760=ORIENTED_EDGE('',*,*,#24866,.T.);
#32761=ORIENTED_EDGE('',*,*,#24867,.T.);
#32762=ORIENTED_EDGE('',*,*,#24868,.T.);
#32763=ORIENTED_EDGE('',*,*,#24869,.T.);
#32764=ORIENTED_EDGE('',*,*,#24870,.T.);
#32765=ORIENTED_EDGE('',*,*,#24871,.T.);
#32766=ORIENTED_EDGE('',*,*,#24872,.T.);
#32767=ORIENTED_EDGE('',*,*,#24873,.T.);
#32768=ORIENTED_EDGE('',*,*,#24874,.T.);
#32769=ORIENTED_EDGE('',*,*,#24875,.T.);
#32770=ORIENTED_EDGE('',*,*,#24876,.T.);
#32771=ORIENTED_EDGE('',*,*,#24877,.T.);
#32772=ORIENTED_EDGE('',*,*,#24878,.T.);
#32773=ORIENTED_EDGE('',*,*,#24879,.T.);
#32774=ORIENTED_EDGE('',*,*,#24880,.T.);
#32775=ORIENTED_EDGE('',*,*,#24881,.T.);
#32776=ORIENTED_EDGE('',*,*,#24882,.T.);
#32777=ORIENTED_EDGE('',*,*,#24883,.T.);
#32778=ORIENTED_EDGE('',*,*,#24884,.T.);
#32779=ORIENTED_EDGE('',*,*,#24885,.T.);
#32780=ORIENTED_EDGE('',*,*,#24886,.T.);
#32781=ORIENTED_EDGE('',*,*,#24887,.T.);
#32782=ORIENTED_EDGE('',*,*,#24888,.T.);
#32783=ORIENTED_EDGE('',*,*,#24889,.T.);
#32784=ORIENTED_EDGE('',*,*,#24890,.T.);
#32785=ORIENTED_EDGE('',*,*,#24891,.T.);
#32786=ORIENTED_EDGE('',*,*,#24892,.T.);
#32787=ORIENTED_EDGE('',*,*,#24893,.T.);
#32788=ORIENTED_EDGE('',*,*,#24894,.T.);
#32789=ORIENTED_EDGE('',*,*,#24895,.T.);
#32790=ORIENTED_EDGE('',*,*,#24896,.T.);
#32791=ORIENTED_EDGE('',*,*,#24897,.T.);
#32792=ORIENTED_EDGE('',*,*,#24898,.T.);
#32793=ORIENTED_EDGE('',*,*,#24899,.T.);
#32794=ORIENTED_EDGE('',*,*,#24900,.T.);
#32795=ORIENTED_EDGE('',*,*,#24901,.T.);
#32796=ORIENTED_EDGE('',*,*,#24902,.T.);
#32797=ORIENTED_EDGE('',*,*,#24903,.T.);
#32798=ORIENTED_EDGE('',*,*,#24904,.T.);
#32799=ORIENTED_EDGE('',*,*,#24905,.T.);
#32800=ORIENTED_EDGE('',*,*,#24906,.T.);
#32801=ORIENTED_EDGE('',*,*,#24907,.T.);
#32802=ORIENTED_EDGE('',*,*,#24908,.T.);
#32803=ORIENTED_EDGE('',*,*,#24909,.T.);
#32804=ORIENTED_EDGE('',*,*,#24910,.T.);
#32805=ORIENTED_EDGE('',*,*,#24911,.T.);
#32806=ORIENTED_EDGE('',*,*,#24912,.T.);
#32807=ORIENTED_EDGE('',*,*,#24913,.T.);
#32808=ORIENTED_EDGE('',*,*,#24914,.T.);
#32809=ORIENTED_EDGE('',*,*,#24915,.T.);
#32810=ORIENTED_EDGE('',*,*,#24916,.T.);
#32811=ORIENTED_EDGE('',*,*,#24917,.T.);
#32812=ORIENTED_EDGE('',*,*,#24918,.T.);
#32813=ORIENTED_EDGE('',*,*,#24919,.T.);
#32814=ORIENTED_EDGE('',*,*,#24920,.T.);
#32815=ORIENTED_EDGE('',*,*,#24921,.T.);
#32816=ORIENTED_EDGE('',*,*,#24922,.T.);
#32817=ORIENTED_EDGE('',*,*,#24923,.T.);
#32818=ORIENTED_EDGE('',*,*,#24924,.T.);
#32819=ORIENTED_EDGE('',*,*,#24925,.T.);
#32820=ORIENTED_EDGE('',*,*,#24926,.T.);
#32821=ORIENTED_EDGE('',*,*,#24927,.T.);
#32822=ORIENTED_EDGE('',*,*,#24928,.T.);
#32823=ORIENTED_EDGE('',*,*,#24929,.T.);
#32824=ORIENTED_EDGE('',*,*,#24930,.T.);
#32825=ORIENTED_EDGE('',*,*,#24931,.T.);
#32826=ORIENTED_EDGE('',*,*,#24932,.T.);
#32827=ORIENTED_EDGE('',*,*,#24933,.T.);
#32828=ORIENTED_EDGE('',*,*,#24934,.T.);
#32829=ORIENTED_EDGE('',*,*,#24935,.T.);
#32830=ORIENTED_EDGE('',*,*,#24936,.T.);
#32831=ORIENTED_EDGE('',*,*,#24937,.T.);
#32832=ORIENTED_EDGE('',*,*,#24938,.T.);
#32833=ORIENTED_EDGE('',*,*,#24939,.T.);
#32834=ORIENTED_EDGE('',*,*,#24940,.T.);
#32835=ORIENTED_EDGE('',*,*,#24941,.T.);
#32836=ORIENTED_EDGE('',*,*,#24942,.T.);
#32837=ORIENTED_EDGE('',*,*,#24943,.T.);
#32838=ORIENTED_EDGE('',*,*,#24944,.T.);
#32839=ORIENTED_EDGE('',*,*,#24945,.T.);
#32840=ORIENTED_EDGE('',*,*,#24946,.T.);
#32841=ORIENTED_EDGE('',*,*,#24947,.T.);
#32842=ORIENTED_EDGE('',*,*,#24948,.T.);
#32843=ORIENTED_EDGE('',*,*,#24949,.T.);
#32844=ORIENTED_EDGE('',*,*,#24950,.T.);
#32845=ORIENTED_EDGE('',*,*,#24951,.T.);
#32846=ORIENTED_EDGE('',*,*,#24952,.T.);
#32847=ORIENTED_EDGE('',*,*,#24953,.T.);
#32848=ORIENTED_EDGE('',*,*,#24954,.T.);
#32849=ORIENTED_EDGE('',*,*,#24955,.T.);
#32850=ORIENTED_EDGE('',*,*,#24956,.T.);
#32851=ORIENTED_EDGE('',*,*,#24957,.T.);
#32852=ORIENTED_EDGE('',*,*,#24958,.T.);
#32853=ORIENTED_EDGE('',*,*,#24959,.T.);
#32854=ORIENTED_EDGE('',*,*,#24960,.T.);
#32855=ORIENTED_EDGE('',*,*,#24961,.T.);
#32856=ORIENTED_EDGE('',*,*,#24962,.T.);
#32857=ORIENTED_EDGE('',*,*,#24963,.T.);
#32858=ORIENTED_EDGE('',*,*,#24964,.T.);
#32859=ORIENTED_EDGE('',*,*,#24965,.T.);
#32860=ORIENTED_EDGE('',*,*,#24966,.T.);
#32861=ORIENTED_EDGE('',*,*,#24967,.T.);
#32862=ORIENTED_EDGE('',*,*,#24968,.T.);
#32863=ORIENTED_EDGE('',*,*,#24969,.T.);
#32864=ORIENTED_EDGE('',*,*,#24970,.T.);
#32865=ORIENTED_EDGE('',*,*,#24971,.T.);
#32866=ORIENTED_EDGE('',*,*,#24972,.T.);
#32867=ORIENTED_EDGE('',*,*,#24973,.T.);
#32868=ORIENTED_EDGE('',*,*,#24974,.T.);
#32869=ORIENTED_EDGE('',*,*,#24975,.T.);
#32870=ORIENTED_EDGE('',*,*,#24976,.T.);
#32871=ORIENTED_EDGE('',*,*,#24977,.T.);
#32872=ORIENTED_EDGE('',*,*,#24978,.T.);
#32873=ORIENTED_EDGE('',*,*,#24979,.T.);
#32874=ORIENTED_EDGE('',*,*,#24980,.T.);
#32875=ORIENTED_EDGE('',*,*,#24981,.T.);
#32876=ORIENTED_EDGE('',*,*,#24982,.T.);
#32877=ORIENTED_EDGE('',*,*,#24983,.T.);
#32878=ORIENTED_EDGE('',*,*,#24984,.T.);
#32879=ORIENTED_EDGE('',*,*,#24985,.T.);
#32880=ORIENTED_EDGE('',*,*,#24986,.T.);
#32881=ORIENTED_EDGE('',*,*,#24987,.T.);
#32882=ORIENTED_EDGE('',*,*,#24988,.T.);
#32883=ORIENTED_EDGE('',*,*,#24989,.T.);
#32884=ORIENTED_EDGE('',*,*,#24990,.T.);
#32885=ORIENTED_EDGE('',*,*,#24991,.T.);
#32886=ORIENTED_EDGE('',*,*,#24992,.T.);
#32887=ORIENTED_EDGE('',*,*,#24993,.T.);
#32888=ORIENTED_EDGE('',*,*,#24994,.T.);
#32889=ORIENTED_EDGE('',*,*,#24995,.T.);
#32890=ORIENTED_EDGE('',*,*,#24996,.T.);
#32891=ORIENTED_EDGE('',*,*,#24997,.T.);
#32892=ORIENTED_EDGE('',*,*,#24998,.T.);
#32893=ORIENTED_EDGE('',*,*,#24999,.T.);
#32894=ORIENTED_EDGE('',*,*,#25000,.T.);
#32895=ORIENTED_EDGE('',*,*,#25001,.T.);
#32896=ORIENTED_EDGE('',*,*,#25002,.T.);
#32897=ORIENTED_EDGE('',*,*,#25003,.T.);
#32898=ORIENTED_EDGE('',*,*,#25004,.T.);
#32899=ORIENTED_EDGE('',*,*,#25005,.T.);
#32900=ORIENTED_EDGE('',*,*,#25006,.T.);
#32901=ORIENTED_EDGE('',*,*,#25007,.T.);
#32902=ORIENTED_EDGE('',*,*,#25008,.T.);
#32903=ORIENTED_EDGE('',*,*,#25009,.T.);
#32904=ORIENTED_EDGE('',*,*,#25010,.T.);
#32905=ORIENTED_EDGE('',*,*,#25011,.T.);
#32906=ORIENTED_EDGE('',*,*,#25012,.T.);
#32907=ORIENTED_EDGE('',*,*,#25013,.T.);
#32908=ORIENTED_EDGE('',*,*,#25014,.T.);
#32909=ORIENTED_EDGE('',*,*,#25015,.T.);
#32910=ORIENTED_EDGE('',*,*,#25016,.T.);
#32911=ORIENTED_EDGE('',*,*,#25017,.T.);
#32912=ORIENTED_EDGE('',*,*,#25018,.T.);
#32913=ORIENTED_EDGE('',*,*,#25019,.T.);
#32914=ORIENTED_EDGE('',*,*,#25020,.T.);
#32915=ORIENTED_EDGE('',*,*,#25021,.T.);
#32916=ORIENTED_EDGE('',*,*,#25022,.T.);
#32917=ORIENTED_EDGE('',*,*,#25023,.T.);
#32918=ORIENTED_EDGE('',*,*,#25024,.T.);
#32919=ORIENTED_EDGE('',*,*,#25025,.T.);
#32920=ORIENTED_EDGE('',*,*,#25026,.T.);
#32921=ORIENTED_EDGE('',*,*,#25027,.T.);
#32922=ORIENTED_EDGE('',*,*,#25028,.T.);
#32923=ORIENTED_EDGE('',*,*,#25029,.T.);
#32924=ORIENTED_EDGE('',*,*,#25030,.T.);
#32925=ORIENTED_EDGE('',*,*,#25031,.T.);
#32926=ORIENTED_EDGE('',*,*,#25032,.T.);
#32927=ORIENTED_EDGE('',*,*,#25033,.T.);
#32928=ORIENTED_EDGE('',*,*,#25034,.T.);
#32929=ORIENTED_EDGE('',*,*,#25035,.T.);
#32930=ORIENTED_EDGE('',*,*,#25036,.T.);
#32931=ORIENTED_EDGE('',*,*,#25037,.T.);
#32932=ORIENTED_EDGE('',*,*,#25038,.T.);
#32933=ORIENTED_EDGE('',*,*,#25039,.T.);
#32934=ORIENTED_EDGE('',*,*,#25040,.T.);
#32935=ORIENTED_EDGE('',*,*,#25041,.T.);
#32936=ORIENTED_EDGE('',*,*,#25042,.T.);
#32937=ORIENTED_EDGE('',*,*,#25043,.T.);
#32938=ORIENTED_EDGE('',*,*,#25044,.T.);
#32939=ORIENTED_EDGE('',*,*,#25045,.T.);
#32940=ORIENTED_EDGE('',*,*,#25046,.T.);
#32941=ORIENTED_EDGE('',*,*,#25047,.T.);
#32942=ORIENTED_EDGE('',*,*,#25048,.T.);
#32943=ORIENTED_EDGE('',*,*,#25049,.T.);
#32944=ORIENTED_EDGE('',*,*,#25050,.T.);
#32945=ORIENTED_EDGE('',*,*,#25051,.T.);
#32946=ORIENTED_EDGE('',*,*,#25052,.T.);
#32947=ORIENTED_EDGE('',*,*,#25053,.T.);
#32948=ORIENTED_EDGE('',*,*,#25054,.T.);
#32949=ORIENTED_EDGE('',*,*,#25055,.T.);
#32950=ORIENTED_EDGE('',*,*,#25056,.T.);
#32951=ORIENTED_EDGE('',*,*,#25057,.T.);
#32952=ORIENTED_EDGE('',*,*,#25058,.T.);
#32953=ORIENTED_EDGE('',*,*,#25059,.T.);
#32954=ORIENTED_EDGE('',*,*,#25060,.T.);
#32955=ORIENTED_EDGE('',*,*,#25061,.T.);
#32956=ORIENTED_EDGE('',*,*,#25062,.T.);
#32957=ORIENTED_EDGE('',*,*,#25063,.T.);
#32958=ORIENTED_EDGE('',*,*,#25064,.T.);
#32959=ORIENTED_EDGE('',*,*,#25065,.T.);
#32960=ORIENTED_EDGE('',*,*,#25066,.T.);
#32961=ORIENTED_EDGE('',*,*,#25067,.T.);
#32962=ORIENTED_EDGE('',*,*,#25068,.T.);
#32963=ORIENTED_EDGE('',*,*,#25069,.T.);
#32964=ORIENTED_EDGE('',*,*,#25070,.T.);
#32965=ORIENTED_EDGE('',*,*,#25071,.T.);
#32966=ORIENTED_EDGE('',*,*,#25072,.T.);
#32967=ORIENTED_EDGE('',*,*,#25073,.T.);
#32968=ORIENTED_EDGE('',*,*,#25074,.T.);
#32969=ORIENTED_EDGE('',*,*,#25075,.T.);
#32970=ORIENTED_EDGE('',*,*,#25076,.T.);
#32971=ORIENTED_EDGE('',*,*,#25077,.T.);
#32972=ORIENTED_EDGE('',*,*,#25078,.T.);
#32973=ORIENTED_EDGE('',*,*,#25079,.T.);
#32974=ORIENTED_EDGE('',*,*,#25080,.T.);
#32975=ORIENTED_EDGE('',*,*,#25081,.T.);
#32976=ORIENTED_EDGE('',*,*,#25082,.T.);
#32977=ORIENTED_EDGE('',*,*,#25083,.T.);
#32978=ORIENTED_EDGE('',*,*,#25084,.T.);
#32979=ORIENTED_EDGE('',*,*,#25085,.T.);
#32980=ORIENTED_EDGE('',*,*,#25086,.T.);
#32981=ORIENTED_EDGE('',*,*,#25087,.T.);
#32982=ORIENTED_EDGE('',*,*,#25088,.T.);
#32983=ORIENTED_EDGE('',*,*,#25089,.T.);
#32984=ORIENTED_EDGE('',*,*,#25090,.T.);
#32985=ORIENTED_EDGE('',*,*,#25091,.T.);
#32986=ORIENTED_EDGE('',*,*,#25092,.T.);
#32987=ORIENTED_EDGE('',*,*,#25093,.T.);
#32988=ORIENTED_EDGE('',*,*,#25094,.T.);
#32989=ORIENTED_EDGE('',*,*,#25095,.T.);
#32990=ORIENTED_EDGE('',*,*,#25096,.T.);
#32991=ORIENTED_EDGE('',*,*,#25097,.T.);
#32992=ORIENTED_EDGE('',*,*,#25098,.T.);
#32993=ORIENTED_EDGE('',*,*,#25099,.T.);
#32994=ORIENTED_EDGE('',*,*,#25100,.T.);
#32995=ORIENTED_EDGE('',*,*,#25101,.T.);
#32996=ORIENTED_EDGE('',*,*,#25102,.T.);
#32997=ORIENTED_EDGE('',*,*,#25103,.T.);
#32998=ORIENTED_EDGE('',*,*,#25104,.T.);
#32999=ORIENTED_EDGE('',*,*,#25105,.T.);
#33000=ORIENTED_EDGE('',*,*,#25106,.T.);
#33001=ORIENTED_EDGE('',*,*,#25107,.T.);
#33002=ORIENTED_EDGE('',*,*,#25108,.T.);
#33003=ORIENTED_EDGE('',*,*,#25109,.T.);
#33004=ORIENTED_EDGE('',*,*,#25110,.T.);
#33005=ORIENTED_EDGE('',*,*,#25111,.T.);
#33006=ORIENTED_EDGE('',*,*,#25112,.T.);
#33007=ORIENTED_EDGE('',*,*,#25113,.T.);
#33008=ORIENTED_EDGE('',*,*,#25114,.T.);
#33009=ORIENTED_EDGE('',*,*,#25115,.T.);
#33010=ORIENTED_EDGE('',*,*,#25116,.T.);
#33011=ORIENTED_EDGE('',*,*,#25117,.T.);
#33012=ORIENTED_EDGE('',*,*,#25118,.T.);
#33013=ORIENTED_EDGE('',*,*,#25119,.T.);
#33014=ORIENTED_EDGE('',*,*,#25120,.T.);
#33015=ORIENTED_EDGE('',*,*,#25121,.T.);
#33016=ORIENTED_EDGE('',*,*,#25122,.T.);
#33017=ORIENTED_EDGE('',*,*,#25123,.T.);
#33018=ORIENTED_EDGE('',*,*,#25124,.T.);
#33019=ORIENTED_EDGE('',*,*,#25125,.T.);
#33020=ORIENTED_EDGE('',*,*,#25126,.T.);
#33021=ORIENTED_EDGE('',*,*,#25127,.T.);
#33022=ORIENTED_EDGE('',*,*,#25128,.T.);
#33023=ORIENTED_EDGE('',*,*,#25129,.T.);
#33024=ORIENTED_EDGE('',*,*,#25130,.T.);
#33025=ORIENTED_EDGE('',*,*,#25131,.T.);
#33026=ORIENTED_EDGE('',*,*,#25132,.T.);
#33027=ORIENTED_EDGE('',*,*,#25133,.T.);
#33028=ORIENTED_EDGE('',*,*,#25134,.T.);
#33029=ORIENTED_EDGE('',*,*,#25135,.T.);
#33030=ORIENTED_EDGE('',*,*,#25136,.T.);
#33031=ORIENTED_EDGE('',*,*,#25137,.T.);
#33032=ORIENTED_EDGE('',*,*,#25138,.T.);
#33033=ORIENTED_EDGE('',*,*,#25139,.T.);
#33034=ORIENTED_EDGE('',*,*,#25140,.T.);
#33035=ORIENTED_EDGE('',*,*,#25141,.T.);
#33036=ORIENTED_EDGE('',*,*,#25142,.T.);
#33037=ORIENTED_EDGE('',*,*,#25143,.T.);
#33038=ORIENTED_EDGE('',*,*,#25144,.T.);
#33039=ORIENTED_EDGE('',*,*,#25145,.T.);
#33040=ORIENTED_EDGE('',*,*,#25146,.T.);
#33041=ORIENTED_EDGE('',*,*,#25147,.T.);
#33042=ORIENTED_EDGE('',*,*,#25148,.T.);
#33043=ORIENTED_EDGE('',*,*,#25149,.T.);
#33044=ORIENTED_EDGE('',*,*,#25150,.T.);
#33045=ORIENTED_EDGE('',*,*,#25151,.T.);
#33046=ORIENTED_EDGE('',*,*,#25152,.T.);
#33047=ORIENTED_EDGE('',*,*,#25153,.T.);
#33048=ORIENTED_EDGE('',*,*,#25154,.T.);
#33049=ORIENTED_EDGE('',*,*,#25155,.T.);
#33050=ORIENTED_EDGE('',*,*,#25156,.T.);
#33051=ORIENTED_EDGE('',*,*,#25157,.T.);
#33052=ORIENTED_EDGE('',*,*,#25158,.T.);
#33053=ORIENTED_EDGE('',*,*,#25159,.T.);
#33054=ORIENTED_EDGE('',*,*,#25160,.T.);
#33055=ORIENTED_EDGE('',*,*,#25161,.T.);
#33056=ORIENTED_EDGE('',*,*,#25162,.T.);
#33057=ORIENTED_EDGE('',*,*,#25163,.T.);
#33058=ORIENTED_EDGE('',*,*,#25164,.T.);
#33059=ORIENTED_EDGE('',*,*,#25165,.T.);
#33060=ORIENTED_EDGE('',*,*,#25166,.T.);
#33061=ORIENTED_EDGE('',*,*,#25167,.T.);
#33062=ORIENTED_EDGE('',*,*,#25168,.T.);
#33063=ORIENTED_EDGE('',*,*,#25169,.T.);
#33064=ORIENTED_EDGE('',*,*,#25170,.T.);
#33065=ORIENTED_EDGE('',*,*,#25171,.T.);
#33066=ORIENTED_EDGE('',*,*,#25172,.T.);
#33067=ORIENTED_EDGE('',*,*,#25173,.T.);
#33068=ORIENTED_EDGE('',*,*,#25174,.T.);
#33069=ORIENTED_EDGE('',*,*,#25175,.T.);
#33070=ORIENTED_EDGE('',*,*,#25176,.T.);
#33071=ORIENTED_EDGE('',*,*,#25177,.T.);
#33072=ORIENTED_EDGE('',*,*,#25178,.T.);
#33073=ORIENTED_EDGE('',*,*,#25179,.T.);
#33074=ORIENTED_EDGE('',*,*,#25180,.T.);
#33075=ORIENTED_EDGE('',*,*,#25181,.T.);
#33076=ORIENTED_EDGE('',*,*,#25182,.T.);
#33077=ORIENTED_EDGE('',*,*,#25183,.T.);
#33078=ORIENTED_EDGE('',*,*,#25184,.T.);
#33079=ORIENTED_EDGE('',*,*,#25185,.T.);
#33080=ORIENTED_EDGE('',*,*,#25186,.T.);
#33081=ORIENTED_EDGE('',*,*,#25187,.T.);
#33082=ORIENTED_EDGE('',*,*,#25188,.T.);
#33083=ORIENTED_EDGE('',*,*,#25189,.T.);
#33084=ORIENTED_EDGE('',*,*,#25190,.T.);
#33085=ORIENTED_EDGE('',*,*,#25191,.T.);
#33086=ORIENTED_EDGE('',*,*,#25192,.T.);
#33087=ORIENTED_EDGE('',*,*,#25193,.T.);
#33088=ORIENTED_EDGE('',*,*,#25194,.T.);
#33089=ORIENTED_EDGE('',*,*,#25195,.T.);
#33090=ORIENTED_EDGE('',*,*,#25196,.T.);
#33091=ORIENTED_EDGE('',*,*,#25197,.T.);
#33092=ORIENTED_EDGE('',*,*,#25198,.T.);
#33093=ORIENTED_EDGE('',*,*,#25199,.T.);
#33094=ORIENTED_EDGE('',*,*,#25200,.T.);
#33095=ORIENTED_EDGE('',*,*,#25201,.T.);
#33096=ORIENTED_EDGE('',*,*,#25202,.T.);
#33097=ORIENTED_EDGE('',*,*,#25203,.T.);
#33098=ORIENTED_EDGE('',*,*,#25204,.T.);
#33099=ORIENTED_EDGE('',*,*,#25205,.T.);
#33100=ORIENTED_EDGE('',*,*,#25206,.T.);
#33101=ORIENTED_EDGE('',*,*,#25207,.T.);
#33102=ORIENTED_EDGE('',*,*,#25208,.T.);
#33103=ORIENTED_EDGE('',*,*,#25209,.T.);
#33104=ORIENTED_EDGE('',*,*,#25210,.T.);
#33105=ORIENTED_EDGE('',*,*,#25211,.T.);
#33106=ORIENTED_EDGE('',*,*,#25212,.T.);
#33107=ORIENTED_EDGE('',*,*,#25213,.T.);
#33108=ORIENTED_EDGE('',*,*,#25214,.T.);
#33109=ORIENTED_EDGE('',*,*,#25215,.T.);
#33110=ORIENTED_EDGE('',*,*,#25216,.T.);
#33111=ORIENTED_EDGE('',*,*,#25217,.T.);
#33112=ORIENTED_EDGE('',*,*,#25218,.T.);
#33113=ORIENTED_EDGE('',*,*,#25219,.T.);
#33114=ORIENTED_EDGE('',*,*,#25220,.T.);
#33115=ORIENTED_EDGE('',*,*,#25221,.T.);
#33116=ORIENTED_EDGE('',*,*,#25222,.T.);
#33117=ORIENTED_EDGE('',*,*,#25223,.T.);
#33118=ORIENTED_EDGE('',*,*,#25224,.T.);
#33119=ORIENTED_EDGE('',*,*,#25225,.T.);
#33120=ORIENTED_EDGE('',*,*,#25226,.T.);
#33121=ORIENTED_EDGE('',*,*,#25227,.T.);
#33122=ORIENTED_EDGE('',*,*,#25228,.T.);
#33123=ORIENTED_EDGE('',*,*,#25229,.T.);
#33124=ORIENTED_EDGE('',*,*,#25230,.T.);
#33125=ORIENTED_EDGE('',*,*,#25231,.T.);
#33126=ORIENTED_EDGE('',*,*,#25232,.T.);
#33127=ORIENTED_EDGE('',*,*,#25233,.T.);
#33128=ORIENTED_EDGE('',*,*,#25234,.T.);
#33129=ORIENTED_EDGE('',*,*,#25235,.T.);
#33130=ORIENTED_EDGE('',*,*,#25236,.T.);
#33131=ORIENTED_EDGE('',*,*,#25237,.T.);
#33132=ORIENTED_EDGE('',*,*,#25238,.T.);
#33133=ORIENTED_EDGE('',*,*,#25239,.T.);
#33134=ORIENTED_EDGE('',*,*,#25240,.T.);
#33135=ORIENTED_EDGE('',*,*,#25241,.T.);
#33136=ORIENTED_EDGE('',*,*,#25242,.T.);
#33137=ORIENTED_EDGE('',*,*,#25243,.T.);
#33138=ORIENTED_EDGE('',*,*,#25244,.T.);
#33139=ORIENTED_EDGE('',*,*,#25245,.T.);
#33140=ORIENTED_EDGE('',*,*,#25246,.T.);
#33141=ORIENTED_EDGE('',*,*,#25247,.T.);
#33142=ORIENTED_EDGE('',*,*,#25248,.T.);
#33143=ORIENTED_EDGE('',*,*,#25249,.T.);
#33144=ORIENTED_EDGE('',*,*,#25250,.T.);
#33145=ORIENTED_EDGE('',*,*,#25251,.T.);
#33146=ORIENTED_EDGE('',*,*,#25252,.T.);
#33147=ORIENTED_EDGE('',*,*,#25253,.T.);
#33148=ORIENTED_EDGE('',*,*,#25254,.T.);
#33149=ORIENTED_EDGE('',*,*,#25255,.T.);
#33150=ORIENTED_EDGE('',*,*,#25256,.T.);
#33151=ORIENTED_EDGE('',*,*,#25257,.T.);
#33152=ORIENTED_EDGE('',*,*,#25258,.T.);
#33153=ORIENTED_EDGE('',*,*,#25259,.T.);
#33154=ORIENTED_EDGE('',*,*,#25260,.T.);
#33155=ORIENTED_EDGE('',*,*,#25261,.T.);
#33156=ORIENTED_EDGE('',*,*,#25262,.T.);
#33157=ORIENTED_EDGE('',*,*,#25263,.T.);
#33158=ORIENTED_EDGE('',*,*,#25264,.T.);
#33159=ORIENTED_EDGE('',*,*,#25265,.T.);
#33160=ORIENTED_EDGE('',*,*,#25266,.T.);
#33161=ORIENTED_EDGE('',*,*,#25267,.T.);
#33162=ORIENTED_EDGE('',*,*,#25268,.T.);
#33163=ORIENTED_EDGE('',*,*,#25269,.T.);
#33164=ORIENTED_EDGE('',*,*,#25270,.T.);
#33165=ORIENTED_EDGE('',*,*,#25271,.T.);
#33166=ORIENTED_EDGE('',*,*,#25272,.T.);
#33167=ORIENTED_EDGE('',*,*,#25273,.T.);
#33168=ORIENTED_EDGE('',*,*,#25274,.T.);
#33169=ORIENTED_EDGE('',*,*,#25275,.T.);
#33170=ORIENTED_EDGE('',*,*,#25276,.T.);
#33171=ORIENTED_EDGE('',*,*,#25277,.T.);
#33172=ORIENTED_EDGE('',*,*,#25278,.T.);
#33173=ORIENTED_EDGE('',*,*,#25279,.T.);
#33174=ORIENTED_EDGE('',*,*,#25280,.T.);
#33175=ORIENTED_EDGE('',*,*,#25281,.T.);
#33176=ORIENTED_EDGE('',*,*,#25282,.T.);
#33177=ORIENTED_EDGE('',*,*,#25283,.T.);
#33178=ORIENTED_EDGE('',*,*,#25284,.T.);
#33179=ORIENTED_EDGE('',*,*,#25285,.T.);
#33180=ORIENTED_EDGE('',*,*,#25286,.T.);
#33181=ORIENTED_EDGE('',*,*,#25287,.T.);
#33182=ORIENTED_EDGE('',*,*,#25288,.T.);
#33183=ORIENTED_EDGE('',*,*,#25289,.T.);
#33184=ORIENTED_EDGE('',*,*,#25290,.T.);
#33185=ORIENTED_EDGE('',*,*,#25291,.T.);
#33186=ORIENTED_EDGE('',*,*,#25292,.T.);
#33187=ORIENTED_EDGE('',*,*,#25293,.T.);
#33188=ORIENTED_EDGE('',*,*,#25294,.T.);
#33189=ORIENTED_EDGE('',*,*,#25295,.T.);
#33190=ORIENTED_EDGE('',*,*,#25296,.T.);
#33191=ORIENTED_EDGE('',*,*,#25297,.T.);
#33192=ORIENTED_EDGE('',*,*,#25298,.T.);
#33193=ORIENTED_EDGE('',*,*,#25299,.T.);
#33194=ORIENTED_EDGE('',*,*,#25300,.T.);
#33195=ORIENTED_EDGE('',*,*,#25301,.T.);
#33196=ORIENTED_EDGE('',*,*,#25302,.T.);
#33197=ORIENTED_EDGE('',*,*,#25303,.T.);
#33198=ORIENTED_EDGE('',*,*,#25304,.T.);
#33199=ORIENTED_EDGE('',*,*,#25305,.T.);
#33200=ORIENTED_EDGE('',*,*,#25306,.T.);
#33201=ORIENTED_EDGE('',*,*,#25307,.T.);
#33202=ORIENTED_EDGE('',*,*,#25308,.T.);
#33203=ORIENTED_EDGE('',*,*,#25309,.T.);
#33204=ORIENTED_EDGE('',*,*,#25310,.T.);
#33205=ORIENTED_EDGE('',*,*,#25311,.T.);
#33206=ORIENTED_EDGE('',*,*,#25312,.T.);
#33207=ORIENTED_EDGE('',*,*,#25313,.T.);
#33208=ORIENTED_EDGE('',*,*,#25314,.T.);
#33209=ORIENTED_EDGE('',*,*,#25315,.T.);
#33210=ORIENTED_EDGE('',*,*,#25316,.T.);
#33211=ORIENTED_EDGE('',*,*,#25317,.T.);
#33212=ORIENTED_EDGE('',*,*,#25318,.T.);
#33213=ORIENTED_EDGE('',*,*,#25319,.T.);
#33214=ORIENTED_EDGE('',*,*,#25320,.T.);
#33215=ORIENTED_EDGE('',*,*,#25321,.T.);
#33216=ORIENTED_EDGE('',*,*,#25322,.T.);
#33217=ORIENTED_EDGE('',*,*,#25323,.T.);
#33218=ORIENTED_EDGE('',*,*,#25324,.T.);
#33219=ORIENTED_EDGE('',*,*,#25325,.T.);
#33220=ORIENTED_EDGE('',*,*,#25326,.T.);
#33221=ORIENTED_EDGE('',*,*,#25327,.T.);
#33222=ORIENTED_EDGE('',*,*,#25328,.T.);
#33223=ORIENTED_EDGE('',*,*,#25329,.T.);
#33224=ORIENTED_EDGE('',*,*,#25330,.T.);
#33225=ORIENTED_EDGE('',*,*,#25331,.T.);
#33226=ORIENTED_EDGE('',*,*,#25332,.T.);
#33227=ORIENTED_EDGE('',*,*,#25333,.T.);
#33228=ORIENTED_EDGE('',*,*,#25334,.T.);
#33229=ORIENTED_EDGE('',*,*,#25335,.T.);
#33230=ORIENTED_EDGE('',*,*,#25336,.T.);
#33231=ORIENTED_EDGE('',*,*,#25337,.T.);
#33232=ORIENTED_EDGE('',*,*,#25338,.T.);
#33233=ORIENTED_EDGE('',*,*,#25339,.T.);
#33234=ORIENTED_EDGE('',*,*,#25340,.T.);
#33235=ORIENTED_EDGE('',*,*,#25341,.T.);
#33236=ORIENTED_EDGE('',*,*,#25342,.T.);
#33237=ORIENTED_EDGE('',*,*,#25343,.T.);
#33238=ORIENTED_EDGE('',*,*,#25344,.T.);
#33239=ORIENTED_EDGE('',*,*,#25345,.T.);
#33240=ORIENTED_EDGE('',*,*,#25346,.T.);
#33241=ORIENTED_EDGE('',*,*,#25347,.T.);
#33242=ORIENTED_EDGE('',*,*,#25348,.T.);
#33243=ORIENTED_EDGE('',*,*,#25349,.T.);
#33244=ORIENTED_EDGE('',*,*,#25350,.T.);
#33245=ORIENTED_EDGE('',*,*,#25351,.T.);
#33246=ORIENTED_EDGE('',*,*,#25352,.T.);
#33247=ORIENTED_EDGE('',*,*,#25353,.T.);
#33248=ORIENTED_EDGE('',*,*,#25354,.T.);
#33249=ORIENTED_EDGE('',*,*,#25355,.T.);
#33250=ORIENTED_EDGE('',*,*,#25356,.T.);
#33251=ORIENTED_EDGE('',*,*,#25357,.T.);
#33252=ORIENTED_EDGE('',*,*,#25358,.T.);
#33253=ORIENTED_EDGE('',*,*,#25359,.T.);
#33254=ORIENTED_EDGE('',*,*,#25360,.T.);
#33255=ORIENTED_EDGE('',*,*,#25361,.T.);
#33256=ORIENTED_EDGE('',*,*,#24239,.T.);
#33257=ORIENTED_EDGE('',*,*,#25362,.F.);
#33258=ORIENTED_EDGE('',*,*,#25356,.F.);
#33259=ORIENTED_EDGE('',*,*,#25363,.T.);
#33260=ORIENTED_EDGE('',*,*,#24240,.T.);
#33261=ORIENTED_EDGE('',*,*,#25361,.F.);
#33262=ORIENTED_EDGE('',*,*,#25355,.F.);
#33263=ORIENTED_EDGE('',*,*,#25364,.T.);
#33264=ORIENTED_EDGE('',*,*,#24241,.T.);
#33265=ORIENTED_EDGE('',*,*,#25363,.F.);
#33266=ORIENTED_EDGE('',*,*,#25360,.F.);
#33267=ORIENTED_EDGE('',*,*,#25365,.T.);
#33268=ORIENTED_EDGE('',*,*,#24242,.T.);
#33269=ORIENTED_EDGE('',*,*,#25364,.F.);
#33270=ORIENTED_EDGE('',*,*,#25359,.F.);
#33271=ORIENTED_EDGE('',*,*,#25366,.T.);
#33272=ORIENTED_EDGE('',*,*,#24243,.T.);
#33273=ORIENTED_EDGE('',*,*,#25365,.F.);
#33274=ORIENTED_EDGE('',*,*,#25358,.F.);
#33275=ORIENTED_EDGE('',*,*,#25362,.T.);
#33276=ORIENTED_EDGE('',*,*,#24244,.T.);
#33277=ORIENTED_EDGE('',*,*,#25366,.F.);
#33278=ORIENTED_EDGE('',*,*,#25357,.F.);
#33279=ORIENTED_EDGE('',*,*,#25367,.T.);
#33280=ORIENTED_EDGE('',*,*,#24233,.T.);
#33281=ORIENTED_EDGE('',*,*,#25368,.F.);
#33282=ORIENTED_EDGE('',*,*,#25350,.F.);
#33283=ORIENTED_EDGE('',*,*,#25369,.T.);
#33284=ORIENTED_EDGE('',*,*,#24234,.T.);
#33285=ORIENTED_EDGE('',*,*,#25367,.F.);
#33286=ORIENTED_EDGE('',*,*,#25349,.F.);
#33287=ORIENTED_EDGE('',*,*,#25370,.T.);
#33288=ORIENTED_EDGE('',*,*,#24235,.T.);
#33289=ORIENTED_EDGE('',*,*,#25369,.F.);
#33290=ORIENTED_EDGE('',*,*,#25354,.F.);
#33291=ORIENTED_EDGE('',*,*,#25371,.T.);
#33292=ORIENTED_EDGE('',*,*,#24236,.T.);
#33293=ORIENTED_EDGE('',*,*,#25370,.F.);
#33294=ORIENTED_EDGE('',*,*,#25353,.F.);
#33295=ORIENTED_EDGE('',*,*,#25372,.T.);
#33296=ORIENTED_EDGE('',*,*,#24237,.T.);
#33297=ORIENTED_EDGE('',*,*,#25371,.F.);
#33298=ORIENTED_EDGE('',*,*,#25352,.F.);
#33299=ORIENTED_EDGE('',*,*,#25368,.T.);
#33300=ORIENTED_EDGE('',*,*,#24238,.T.);
#33301=ORIENTED_EDGE('',*,*,#25372,.F.);
#33302=ORIENTED_EDGE('',*,*,#25351,.F.);
#33303=ORIENTED_EDGE('',*,*,#25373,.T.);
#33304=ORIENTED_EDGE('',*,*,#24227,.T.);
#33305=ORIENTED_EDGE('',*,*,#25374,.F.);
#33306=ORIENTED_EDGE('',*,*,#25344,.F.);
#33307=ORIENTED_EDGE('',*,*,#25375,.T.);
#33308=ORIENTED_EDGE('',*,*,#24228,.T.);
#33309=ORIENTED_EDGE('',*,*,#25373,.F.);
#33310=ORIENTED_EDGE('',*,*,#25343,.F.);
#33311=ORIENTED_EDGE('',*,*,#25376,.T.);
#33312=ORIENTED_EDGE('',*,*,#24229,.T.);
#33313=ORIENTED_EDGE('',*,*,#25375,.F.);
#33314=ORIENTED_EDGE('',*,*,#25348,.F.);
#33315=ORIENTED_EDGE('',*,*,#25377,.T.);
#33316=ORIENTED_EDGE('',*,*,#24230,.T.);
#33317=ORIENTED_EDGE('',*,*,#25376,.F.);
#33318=ORIENTED_EDGE('',*,*,#25347,.F.);
#33319=ORIENTED_EDGE('',*,*,#25378,.T.);
#33320=ORIENTED_EDGE('',*,*,#24231,.T.);
#33321=ORIENTED_EDGE('',*,*,#25377,.F.);
#33322=ORIENTED_EDGE('',*,*,#25346,.F.);
#33323=ORIENTED_EDGE('',*,*,#25374,.T.);
#33324=ORIENTED_EDGE('',*,*,#24232,.T.);
#33325=ORIENTED_EDGE('',*,*,#25378,.F.);
#33326=ORIENTED_EDGE('',*,*,#25345,.F.);
#33327=ORIENTED_EDGE('',*,*,#25379,.T.);
#33328=ORIENTED_EDGE('',*,*,#24221,.T.);
#33329=ORIENTED_EDGE('',*,*,#25380,.F.);
#33330=ORIENTED_EDGE('',*,*,#25338,.F.);
#33331=ORIENTED_EDGE('',*,*,#25381,.T.);
#33332=ORIENTED_EDGE('',*,*,#24222,.T.);
#33333=ORIENTED_EDGE('',*,*,#25379,.F.);
#33334=ORIENTED_EDGE('',*,*,#25337,.F.);
#33335=ORIENTED_EDGE('',*,*,#25382,.T.);
#33336=ORIENTED_EDGE('',*,*,#24223,.T.);
#33337=ORIENTED_EDGE('',*,*,#25381,.F.);
#33338=ORIENTED_EDGE('',*,*,#25342,.F.);
#33339=ORIENTED_EDGE('',*,*,#25383,.T.);
#33340=ORIENTED_EDGE('',*,*,#24224,.T.);
#33341=ORIENTED_EDGE('',*,*,#25382,.F.);
#33342=ORIENTED_EDGE('',*,*,#25341,.F.);
#33343=ORIENTED_EDGE('',*,*,#25384,.T.);
#33344=ORIENTED_EDGE('',*,*,#24225,.T.);
#33345=ORIENTED_EDGE('',*,*,#25383,.F.);
#33346=ORIENTED_EDGE('',*,*,#25340,.F.);
#33347=ORIENTED_EDGE('',*,*,#25380,.T.);
#33348=ORIENTED_EDGE('',*,*,#24226,.T.);
#33349=ORIENTED_EDGE('',*,*,#25384,.F.);
#33350=ORIENTED_EDGE('',*,*,#25339,.F.);
#33351=ORIENTED_EDGE('',*,*,#25385,.T.);
#33352=ORIENTED_EDGE('',*,*,#24215,.T.);
#33353=ORIENTED_EDGE('',*,*,#25386,.F.);
#33354=ORIENTED_EDGE('',*,*,#25332,.F.);
#33355=ORIENTED_EDGE('',*,*,#25387,.T.);
#33356=ORIENTED_EDGE('',*,*,#24216,.T.);
#33357=ORIENTED_EDGE('',*,*,#25385,.F.);
#33358=ORIENTED_EDGE('',*,*,#25331,.F.);
#33359=ORIENTED_EDGE('',*,*,#25388,.T.);
#33360=ORIENTED_EDGE('',*,*,#24217,.T.);
#33361=ORIENTED_EDGE('',*,*,#25387,.F.);
#33362=ORIENTED_EDGE('',*,*,#25336,.F.);
#33363=ORIENTED_EDGE('',*,*,#25389,.T.);
#33364=ORIENTED_EDGE('',*,*,#24218,.T.);
#33365=ORIENTED_EDGE('',*,*,#25388,.F.);
#33366=ORIENTED_EDGE('',*,*,#25335,.F.);
#33367=ORIENTED_EDGE('',*,*,#25390,.T.);
#33368=ORIENTED_EDGE('',*,*,#24219,.T.);
#33369=ORIENTED_EDGE('',*,*,#25389,.F.);
#33370=ORIENTED_EDGE('',*,*,#25334,.F.);
#33371=ORIENTED_EDGE('',*,*,#25386,.T.);
#33372=ORIENTED_EDGE('',*,*,#24220,.T.);
#33373=ORIENTED_EDGE('',*,*,#25390,.F.);
#33374=ORIENTED_EDGE('',*,*,#25333,.F.);
#33375=ORIENTED_EDGE('',*,*,#25391,.T.);
#33376=ORIENTED_EDGE('',*,*,#24209,.T.);
#33377=ORIENTED_EDGE('',*,*,#25392,.F.);
#33378=ORIENTED_EDGE('',*,*,#25326,.F.);
#33379=ORIENTED_EDGE('',*,*,#25393,.T.);
#33380=ORIENTED_EDGE('',*,*,#24210,.T.);
#33381=ORIENTED_EDGE('',*,*,#25391,.F.);
#33382=ORIENTED_EDGE('',*,*,#25325,.F.);
#33383=ORIENTED_EDGE('',*,*,#25394,.T.);
#33384=ORIENTED_EDGE('',*,*,#24211,.T.);
#33385=ORIENTED_EDGE('',*,*,#25393,.F.);
#33386=ORIENTED_EDGE('',*,*,#25330,.F.);
#33387=ORIENTED_EDGE('',*,*,#25395,.T.);
#33388=ORIENTED_EDGE('',*,*,#24212,.T.);
#33389=ORIENTED_EDGE('',*,*,#25394,.F.);
#33390=ORIENTED_EDGE('',*,*,#25329,.F.);
#33391=ORIENTED_EDGE('',*,*,#25396,.T.);
#33392=ORIENTED_EDGE('',*,*,#24213,.T.);
#33393=ORIENTED_EDGE('',*,*,#25395,.F.);
#33394=ORIENTED_EDGE('',*,*,#25328,.F.);
#33395=ORIENTED_EDGE('',*,*,#25392,.T.);
#33396=ORIENTED_EDGE('',*,*,#24214,.T.);
#33397=ORIENTED_EDGE('',*,*,#25396,.F.);
#33398=ORIENTED_EDGE('',*,*,#25327,.F.);
#33399=ORIENTED_EDGE('',*,*,#25397,.T.);
#33400=ORIENTED_EDGE('',*,*,#24203,.T.);
#33401=ORIENTED_EDGE('',*,*,#25398,.F.);
#33402=ORIENTED_EDGE('',*,*,#25320,.F.);
#33403=ORIENTED_EDGE('',*,*,#25399,.T.);
#33404=ORIENTED_EDGE('',*,*,#24204,.T.);
#33405=ORIENTED_EDGE('',*,*,#25397,.F.);
#33406=ORIENTED_EDGE('',*,*,#25319,.F.);
#33407=ORIENTED_EDGE('',*,*,#25400,.T.);
#33408=ORIENTED_EDGE('',*,*,#24205,.T.);
#33409=ORIENTED_EDGE('',*,*,#25399,.F.);
#33410=ORIENTED_EDGE('',*,*,#25324,.F.);
#33411=ORIENTED_EDGE('',*,*,#25401,.T.);
#33412=ORIENTED_EDGE('',*,*,#24206,.T.);
#33413=ORIENTED_EDGE('',*,*,#25400,.F.);
#33414=ORIENTED_EDGE('',*,*,#25323,.F.);
#33415=ORIENTED_EDGE('',*,*,#25402,.T.);
#33416=ORIENTED_EDGE('',*,*,#24207,.T.);
#33417=ORIENTED_EDGE('',*,*,#25401,.F.);
#33418=ORIENTED_EDGE('',*,*,#25322,.F.);
#33419=ORIENTED_EDGE('',*,*,#25398,.T.);
#33420=ORIENTED_EDGE('',*,*,#24208,.T.);
#33421=ORIENTED_EDGE('',*,*,#25402,.F.);
#33422=ORIENTED_EDGE('',*,*,#25321,.F.);
#33423=ORIENTED_EDGE('',*,*,#25403,.T.);
#33424=ORIENTED_EDGE('',*,*,#24197,.T.);
#33425=ORIENTED_EDGE('',*,*,#25404,.F.);
#33426=ORIENTED_EDGE('',*,*,#25314,.F.);
#33427=ORIENTED_EDGE('',*,*,#25405,.T.);
#33428=ORIENTED_EDGE('',*,*,#24198,.T.);
#33429=ORIENTED_EDGE('',*,*,#25403,.F.);
#33430=ORIENTED_EDGE('',*,*,#25313,.F.);
#33431=ORIENTED_EDGE('',*,*,#25406,.T.);
#33432=ORIENTED_EDGE('',*,*,#24199,.T.);
#33433=ORIENTED_EDGE('',*,*,#25405,.F.);
#33434=ORIENTED_EDGE('',*,*,#25318,.F.);
#33435=ORIENTED_EDGE('',*,*,#25407,.T.);
#33436=ORIENTED_EDGE('',*,*,#24200,.T.);
#33437=ORIENTED_EDGE('',*,*,#25406,.F.);
#33438=ORIENTED_EDGE('',*,*,#25317,.F.);
#33439=ORIENTED_EDGE('',*,*,#25408,.T.);
#33440=ORIENTED_EDGE('',*,*,#24201,.T.);
#33441=ORIENTED_EDGE('',*,*,#25407,.F.);
#33442=ORIENTED_EDGE('',*,*,#25316,.F.);
#33443=ORIENTED_EDGE('',*,*,#25404,.T.);
#33444=ORIENTED_EDGE('',*,*,#24202,.T.);
#33445=ORIENTED_EDGE('',*,*,#25408,.F.);
#33446=ORIENTED_EDGE('',*,*,#25315,.F.);
#33447=ORIENTED_EDGE('',*,*,#25409,.T.);
#33448=ORIENTED_EDGE('',*,*,#24191,.T.);
#33449=ORIENTED_EDGE('',*,*,#25410,.F.);
#33450=ORIENTED_EDGE('',*,*,#25308,.F.);
#33451=ORIENTED_EDGE('',*,*,#25411,.T.);
#33452=ORIENTED_EDGE('',*,*,#24192,.T.);
#33453=ORIENTED_EDGE('',*,*,#25409,.F.);
#33454=ORIENTED_EDGE('',*,*,#25307,.F.);
#33455=ORIENTED_EDGE('',*,*,#25412,.T.);
#33456=ORIENTED_EDGE('',*,*,#24193,.T.);
#33457=ORIENTED_EDGE('',*,*,#25411,.F.);
#33458=ORIENTED_EDGE('',*,*,#25312,.F.);
#33459=ORIENTED_EDGE('',*,*,#25413,.T.);
#33460=ORIENTED_EDGE('',*,*,#24194,.T.);
#33461=ORIENTED_EDGE('',*,*,#25412,.F.);
#33462=ORIENTED_EDGE('',*,*,#25311,.F.);
#33463=ORIENTED_EDGE('',*,*,#25414,.T.);
#33464=ORIENTED_EDGE('',*,*,#24195,.T.);
#33465=ORIENTED_EDGE('',*,*,#25413,.F.);
#33466=ORIENTED_EDGE('',*,*,#25310,.F.);
#33467=ORIENTED_EDGE('',*,*,#25410,.T.);
#33468=ORIENTED_EDGE('',*,*,#24196,.T.);
#33469=ORIENTED_EDGE('',*,*,#25414,.F.);
#33470=ORIENTED_EDGE('',*,*,#25309,.F.);
#33471=ORIENTED_EDGE('',*,*,#25415,.T.);
#33472=ORIENTED_EDGE('',*,*,#24185,.T.);
#33473=ORIENTED_EDGE('',*,*,#25416,.F.);
#33474=ORIENTED_EDGE('',*,*,#25302,.F.);
#33475=ORIENTED_EDGE('',*,*,#25417,.T.);
#33476=ORIENTED_EDGE('',*,*,#24186,.T.);
#33477=ORIENTED_EDGE('',*,*,#25415,.F.);
#33478=ORIENTED_EDGE('',*,*,#25301,.F.);
#33479=ORIENTED_EDGE('',*,*,#25418,.T.);
#33480=ORIENTED_EDGE('',*,*,#24187,.T.);
#33481=ORIENTED_EDGE('',*,*,#25417,.F.);
#33482=ORIENTED_EDGE('',*,*,#25306,.F.);
#33483=ORIENTED_EDGE('',*,*,#25419,.T.);
#33484=ORIENTED_EDGE('',*,*,#24188,.T.);
#33485=ORIENTED_EDGE('',*,*,#25418,.F.);
#33486=ORIENTED_EDGE('',*,*,#25305,.F.);
#33487=ORIENTED_EDGE('',*,*,#25420,.T.);
#33488=ORIENTED_EDGE('',*,*,#24189,.T.);
#33489=ORIENTED_EDGE('',*,*,#25419,.F.);
#33490=ORIENTED_EDGE('',*,*,#25304,.F.);
#33491=ORIENTED_EDGE('',*,*,#25416,.T.);
#33492=ORIENTED_EDGE('',*,*,#24190,.T.);
#33493=ORIENTED_EDGE('',*,*,#25420,.F.);
#33494=ORIENTED_EDGE('',*,*,#25303,.F.);
#33495=ORIENTED_EDGE('',*,*,#25421,.T.);
#33496=ORIENTED_EDGE('',*,*,#24179,.T.);
#33497=ORIENTED_EDGE('',*,*,#25422,.F.);
#33498=ORIENTED_EDGE('',*,*,#25296,.F.);
#33499=ORIENTED_EDGE('',*,*,#25423,.T.);
#33500=ORIENTED_EDGE('',*,*,#24180,.T.);
#33501=ORIENTED_EDGE('',*,*,#25421,.F.);
#33502=ORIENTED_EDGE('',*,*,#25295,.F.);
#33503=ORIENTED_EDGE('',*,*,#25424,.T.);
#33504=ORIENTED_EDGE('',*,*,#24181,.T.);
#33505=ORIENTED_EDGE('',*,*,#25423,.F.);
#33506=ORIENTED_EDGE('',*,*,#25300,.F.);
#33507=ORIENTED_EDGE('',*,*,#25425,.T.);
#33508=ORIENTED_EDGE('',*,*,#24182,.T.);
#33509=ORIENTED_EDGE('',*,*,#25424,.F.);
#33510=ORIENTED_EDGE('',*,*,#25299,.F.);
#33511=ORIENTED_EDGE('',*,*,#25426,.T.);
#33512=ORIENTED_EDGE('',*,*,#24183,.T.);
#33513=ORIENTED_EDGE('',*,*,#25425,.F.);
#33514=ORIENTED_EDGE('',*,*,#25298,.F.);
#33515=ORIENTED_EDGE('',*,*,#25422,.T.);
#33516=ORIENTED_EDGE('',*,*,#24184,.T.);
#33517=ORIENTED_EDGE('',*,*,#25426,.F.);
#33518=ORIENTED_EDGE('',*,*,#25297,.F.);
#33519=ORIENTED_EDGE('',*,*,#25427,.T.);
#33520=ORIENTED_EDGE('',*,*,#24173,.T.);
#33521=ORIENTED_EDGE('',*,*,#25428,.F.);
#33522=ORIENTED_EDGE('',*,*,#25290,.F.);
#33523=ORIENTED_EDGE('',*,*,#25429,.T.);
#33524=ORIENTED_EDGE('',*,*,#24174,.T.);
#33525=ORIENTED_EDGE('',*,*,#25427,.F.);
#33526=ORIENTED_EDGE('',*,*,#25289,.F.);
#33527=ORIENTED_EDGE('',*,*,#25430,.T.);
#33528=ORIENTED_EDGE('',*,*,#24175,.T.);
#33529=ORIENTED_EDGE('',*,*,#25429,.F.);
#33530=ORIENTED_EDGE('',*,*,#25294,.F.);
#33531=ORIENTED_EDGE('',*,*,#25431,.T.);
#33532=ORIENTED_EDGE('',*,*,#24176,.T.);
#33533=ORIENTED_EDGE('',*,*,#25430,.F.);
#33534=ORIENTED_EDGE('',*,*,#25293,.F.);
#33535=ORIENTED_EDGE('',*,*,#25432,.T.);
#33536=ORIENTED_EDGE('',*,*,#24177,.T.);
#33537=ORIENTED_EDGE('',*,*,#25431,.F.);
#33538=ORIENTED_EDGE('',*,*,#25292,.F.);
#33539=ORIENTED_EDGE('',*,*,#25428,.T.);
#33540=ORIENTED_EDGE('',*,*,#24178,.T.);
#33541=ORIENTED_EDGE('',*,*,#25432,.F.);
#33542=ORIENTED_EDGE('',*,*,#25291,.F.);
#33543=ORIENTED_EDGE('',*,*,#25433,.T.);
#33544=ORIENTED_EDGE('',*,*,#24167,.T.);
#33545=ORIENTED_EDGE('',*,*,#25434,.F.);
#33546=ORIENTED_EDGE('',*,*,#25284,.F.);
#33547=ORIENTED_EDGE('',*,*,#25435,.T.);
#33548=ORIENTED_EDGE('',*,*,#24168,.T.);
#33549=ORIENTED_EDGE('',*,*,#25433,.F.);
#33550=ORIENTED_EDGE('',*,*,#25283,.F.);
#33551=ORIENTED_EDGE('',*,*,#25436,.T.);
#33552=ORIENTED_EDGE('',*,*,#24169,.T.);
#33553=ORIENTED_EDGE('',*,*,#25435,.F.);
#33554=ORIENTED_EDGE('',*,*,#25288,.F.);
#33555=ORIENTED_EDGE('',*,*,#25437,.T.);
#33556=ORIENTED_EDGE('',*,*,#24170,.T.);
#33557=ORIENTED_EDGE('',*,*,#25436,.F.);
#33558=ORIENTED_EDGE('',*,*,#25287,.F.);
#33559=ORIENTED_EDGE('',*,*,#25438,.T.);
#33560=ORIENTED_EDGE('',*,*,#24171,.T.);
#33561=ORIENTED_EDGE('',*,*,#25437,.F.);
#33562=ORIENTED_EDGE('',*,*,#25286,.F.);
#33563=ORIENTED_EDGE('',*,*,#25434,.T.);
#33564=ORIENTED_EDGE('',*,*,#24172,.T.);
#33565=ORIENTED_EDGE('',*,*,#25438,.F.);
#33566=ORIENTED_EDGE('',*,*,#25285,.F.);
#33567=ORIENTED_EDGE('',*,*,#25439,.T.);
#33568=ORIENTED_EDGE('',*,*,#24161,.T.);
#33569=ORIENTED_EDGE('',*,*,#25440,.F.);
#33570=ORIENTED_EDGE('',*,*,#25278,.F.);
#33571=ORIENTED_EDGE('',*,*,#25441,.T.);
#33572=ORIENTED_EDGE('',*,*,#24162,.T.);
#33573=ORIENTED_EDGE('',*,*,#25439,.F.);
#33574=ORIENTED_EDGE('',*,*,#25277,.F.);
#33575=ORIENTED_EDGE('',*,*,#25442,.T.);
#33576=ORIENTED_EDGE('',*,*,#24163,.T.);
#33577=ORIENTED_EDGE('',*,*,#25441,.F.);
#33578=ORIENTED_EDGE('',*,*,#25282,.F.);
#33579=ORIENTED_EDGE('',*,*,#25443,.T.);
#33580=ORIENTED_EDGE('',*,*,#24164,.T.);
#33581=ORIENTED_EDGE('',*,*,#25442,.F.);
#33582=ORIENTED_EDGE('',*,*,#25281,.F.);
#33583=ORIENTED_EDGE('',*,*,#25444,.T.);
#33584=ORIENTED_EDGE('',*,*,#24165,.T.);
#33585=ORIENTED_EDGE('',*,*,#25443,.F.);
#33586=ORIENTED_EDGE('',*,*,#25280,.F.);
#33587=ORIENTED_EDGE('',*,*,#25440,.T.);
#33588=ORIENTED_EDGE('',*,*,#24166,.T.);
#33589=ORIENTED_EDGE('',*,*,#25444,.F.);
#33590=ORIENTED_EDGE('',*,*,#25279,.F.);
#33591=ORIENTED_EDGE('',*,*,#25445,.T.);
#33592=ORIENTED_EDGE('',*,*,#24155,.T.);
#33593=ORIENTED_EDGE('',*,*,#25446,.F.);
#33594=ORIENTED_EDGE('',*,*,#25272,.F.);
#33595=ORIENTED_EDGE('',*,*,#25447,.T.);
#33596=ORIENTED_EDGE('',*,*,#24156,.T.);
#33597=ORIENTED_EDGE('',*,*,#25445,.F.);
#33598=ORIENTED_EDGE('',*,*,#25271,.F.);
#33599=ORIENTED_EDGE('',*,*,#25448,.T.);
#33600=ORIENTED_EDGE('',*,*,#24157,.T.);
#33601=ORIENTED_EDGE('',*,*,#25447,.F.);
#33602=ORIENTED_EDGE('',*,*,#25276,.F.);
#33603=ORIENTED_EDGE('',*,*,#25449,.T.);
#33604=ORIENTED_EDGE('',*,*,#24158,.T.);
#33605=ORIENTED_EDGE('',*,*,#25448,.F.);
#33606=ORIENTED_EDGE('',*,*,#25275,.F.);
#33607=ORIENTED_EDGE('',*,*,#25450,.T.);
#33608=ORIENTED_EDGE('',*,*,#24159,.T.);
#33609=ORIENTED_EDGE('',*,*,#25449,.F.);
#33610=ORIENTED_EDGE('',*,*,#25274,.F.);
#33611=ORIENTED_EDGE('',*,*,#25446,.T.);
#33612=ORIENTED_EDGE('',*,*,#24160,.T.);
#33613=ORIENTED_EDGE('',*,*,#25450,.F.);
#33614=ORIENTED_EDGE('',*,*,#25273,.F.);
#33615=ORIENTED_EDGE('',*,*,#25451,.T.);
#33616=ORIENTED_EDGE('',*,*,#24149,.T.);
#33617=ORIENTED_EDGE('',*,*,#25452,.F.);
#33618=ORIENTED_EDGE('',*,*,#25266,.F.);
#33619=ORIENTED_EDGE('',*,*,#25453,.T.);
#33620=ORIENTED_EDGE('',*,*,#24150,.T.);
#33621=ORIENTED_EDGE('',*,*,#25451,.F.);
#33622=ORIENTED_EDGE('',*,*,#25265,.F.);
#33623=ORIENTED_EDGE('',*,*,#25454,.T.);
#33624=ORIENTED_EDGE('',*,*,#24151,.T.);
#33625=ORIENTED_EDGE('',*,*,#25453,.F.);
#33626=ORIENTED_EDGE('',*,*,#25270,.F.);
#33627=ORIENTED_EDGE('',*,*,#25455,.T.);
#33628=ORIENTED_EDGE('',*,*,#24152,.T.);
#33629=ORIENTED_EDGE('',*,*,#25454,.F.);
#33630=ORIENTED_EDGE('',*,*,#25269,.F.);
#33631=ORIENTED_EDGE('',*,*,#25456,.T.);
#33632=ORIENTED_EDGE('',*,*,#24153,.T.);
#33633=ORIENTED_EDGE('',*,*,#25455,.F.);
#33634=ORIENTED_EDGE('',*,*,#25268,.F.);
#33635=ORIENTED_EDGE('',*,*,#25452,.T.);
#33636=ORIENTED_EDGE('',*,*,#24154,.T.);
#33637=ORIENTED_EDGE('',*,*,#25456,.F.);
#33638=ORIENTED_EDGE('',*,*,#25267,.F.);
#33639=ORIENTED_EDGE('',*,*,#25457,.T.);
#33640=ORIENTED_EDGE('',*,*,#24143,.T.);
#33641=ORIENTED_EDGE('',*,*,#25458,.F.);
#33642=ORIENTED_EDGE('',*,*,#25260,.F.);
#33643=ORIENTED_EDGE('',*,*,#25459,.T.);
#33644=ORIENTED_EDGE('',*,*,#24144,.T.);
#33645=ORIENTED_EDGE('',*,*,#25457,.F.);
#33646=ORIENTED_EDGE('',*,*,#25259,.F.);
#33647=ORIENTED_EDGE('',*,*,#25460,.T.);
#33648=ORIENTED_EDGE('',*,*,#24145,.T.);
#33649=ORIENTED_EDGE('',*,*,#25459,.F.);
#33650=ORIENTED_EDGE('',*,*,#25264,.F.);
#33651=ORIENTED_EDGE('',*,*,#25461,.T.);
#33652=ORIENTED_EDGE('',*,*,#24146,.T.);
#33653=ORIENTED_EDGE('',*,*,#25460,.F.);
#33654=ORIENTED_EDGE('',*,*,#25263,.F.);
#33655=ORIENTED_EDGE('',*,*,#25462,.T.);
#33656=ORIENTED_EDGE('',*,*,#24147,.T.);
#33657=ORIENTED_EDGE('',*,*,#25461,.F.);
#33658=ORIENTED_EDGE('',*,*,#25262,.F.);
#33659=ORIENTED_EDGE('',*,*,#25458,.T.);
#33660=ORIENTED_EDGE('',*,*,#24148,.T.);
#33661=ORIENTED_EDGE('',*,*,#25462,.F.);
#33662=ORIENTED_EDGE('',*,*,#25261,.F.);
#33663=ORIENTED_EDGE('',*,*,#25463,.T.);
#33664=ORIENTED_EDGE('',*,*,#24137,.T.);
#33665=ORIENTED_EDGE('',*,*,#25464,.F.);
#33666=ORIENTED_EDGE('',*,*,#25254,.F.);
#33667=ORIENTED_EDGE('',*,*,#25465,.T.);
#33668=ORIENTED_EDGE('',*,*,#24138,.T.);
#33669=ORIENTED_EDGE('',*,*,#25463,.F.);
#33670=ORIENTED_EDGE('',*,*,#25253,.F.);
#33671=ORIENTED_EDGE('',*,*,#25466,.T.);
#33672=ORIENTED_EDGE('',*,*,#24139,.T.);
#33673=ORIENTED_EDGE('',*,*,#25465,.F.);
#33674=ORIENTED_EDGE('',*,*,#25258,.F.);
#33675=ORIENTED_EDGE('',*,*,#25467,.T.);
#33676=ORIENTED_EDGE('',*,*,#24140,.T.);
#33677=ORIENTED_EDGE('',*,*,#25466,.F.);
#33678=ORIENTED_EDGE('',*,*,#25257,.F.);
#33679=ORIENTED_EDGE('',*,*,#25468,.T.);
#33680=ORIENTED_EDGE('',*,*,#24141,.T.);
#33681=ORIENTED_EDGE('',*,*,#25467,.F.);
#33682=ORIENTED_EDGE('',*,*,#25256,.F.);
#33683=ORIENTED_EDGE('',*,*,#25464,.T.);
#33684=ORIENTED_EDGE('',*,*,#24142,.T.);
#33685=ORIENTED_EDGE('',*,*,#25468,.F.);
#33686=ORIENTED_EDGE('',*,*,#25255,.F.);
#33687=ORIENTED_EDGE('',*,*,#25469,.T.);
#33688=ORIENTED_EDGE('',*,*,#24131,.T.);
#33689=ORIENTED_EDGE('',*,*,#25470,.F.);
#33690=ORIENTED_EDGE('',*,*,#25248,.F.);
#33691=ORIENTED_EDGE('',*,*,#25471,.T.);
#33692=ORIENTED_EDGE('',*,*,#24132,.T.);
#33693=ORIENTED_EDGE('',*,*,#25469,.F.);
#33694=ORIENTED_EDGE('',*,*,#25247,.F.);
#33695=ORIENTED_EDGE('',*,*,#25472,.T.);
#33696=ORIENTED_EDGE('',*,*,#24133,.T.);
#33697=ORIENTED_EDGE('',*,*,#25471,.F.);
#33698=ORIENTED_EDGE('',*,*,#25252,.F.);
#33699=ORIENTED_EDGE('',*,*,#25473,.T.);
#33700=ORIENTED_EDGE('',*,*,#24134,.T.);
#33701=ORIENTED_EDGE('',*,*,#25472,.F.);
#33702=ORIENTED_EDGE('',*,*,#25251,.F.);
#33703=ORIENTED_EDGE('',*,*,#25474,.T.);
#33704=ORIENTED_EDGE('',*,*,#24135,.T.);
#33705=ORIENTED_EDGE('',*,*,#25473,.F.);
#33706=ORIENTED_EDGE('',*,*,#25250,.F.);
#33707=ORIENTED_EDGE('',*,*,#25470,.T.);
#33708=ORIENTED_EDGE('',*,*,#24136,.T.);
#33709=ORIENTED_EDGE('',*,*,#25474,.F.);
#33710=ORIENTED_EDGE('',*,*,#25249,.F.);
#33711=ORIENTED_EDGE('',*,*,#25475,.T.);
#33712=ORIENTED_EDGE('',*,*,#24125,.T.);
#33713=ORIENTED_EDGE('',*,*,#25476,.F.);
#33714=ORIENTED_EDGE('',*,*,#25242,.F.);
#33715=ORIENTED_EDGE('',*,*,#25477,.T.);
#33716=ORIENTED_EDGE('',*,*,#24126,.T.);
#33717=ORIENTED_EDGE('',*,*,#25475,.F.);
#33718=ORIENTED_EDGE('',*,*,#25241,.F.);
#33719=ORIENTED_EDGE('',*,*,#25478,.T.);
#33720=ORIENTED_EDGE('',*,*,#24127,.T.);
#33721=ORIENTED_EDGE('',*,*,#25477,.F.);
#33722=ORIENTED_EDGE('',*,*,#25246,.F.);
#33723=ORIENTED_EDGE('',*,*,#25479,.T.);
#33724=ORIENTED_EDGE('',*,*,#24128,.T.);
#33725=ORIENTED_EDGE('',*,*,#25478,.F.);
#33726=ORIENTED_EDGE('',*,*,#25245,.F.);
#33727=ORIENTED_EDGE('',*,*,#25480,.T.);
#33728=ORIENTED_EDGE('',*,*,#24129,.T.);
#33729=ORIENTED_EDGE('',*,*,#25479,.F.);
#33730=ORIENTED_EDGE('',*,*,#25244,.F.);
#33731=ORIENTED_EDGE('',*,*,#25476,.T.);
#33732=ORIENTED_EDGE('',*,*,#24130,.T.);
#33733=ORIENTED_EDGE('',*,*,#25480,.F.);
#33734=ORIENTED_EDGE('',*,*,#25243,.F.);
#33735=ORIENTED_EDGE('',*,*,#25481,.T.);
#33736=ORIENTED_EDGE('',*,*,#24119,.T.);
#33737=ORIENTED_EDGE('',*,*,#25482,.F.);
#33738=ORIENTED_EDGE('',*,*,#25236,.F.);
#33739=ORIENTED_EDGE('',*,*,#25483,.T.);
#33740=ORIENTED_EDGE('',*,*,#24120,.T.);
#33741=ORIENTED_EDGE('',*,*,#25481,.F.);
#33742=ORIENTED_EDGE('',*,*,#25235,.F.);
#33743=ORIENTED_EDGE('',*,*,#25484,.T.);
#33744=ORIENTED_EDGE('',*,*,#24121,.T.);
#33745=ORIENTED_EDGE('',*,*,#25483,.F.);
#33746=ORIENTED_EDGE('',*,*,#25240,.F.);
#33747=ORIENTED_EDGE('',*,*,#25485,.T.);
#33748=ORIENTED_EDGE('',*,*,#24122,.T.);
#33749=ORIENTED_EDGE('',*,*,#25484,.F.);
#33750=ORIENTED_EDGE('',*,*,#25239,.F.);
#33751=ORIENTED_EDGE('',*,*,#25486,.T.);
#33752=ORIENTED_EDGE('',*,*,#24123,.T.);
#33753=ORIENTED_EDGE('',*,*,#25485,.F.);
#33754=ORIENTED_EDGE('',*,*,#25238,.F.);
#33755=ORIENTED_EDGE('',*,*,#25482,.T.);
#33756=ORIENTED_EDGE('',*,*,#24124,.T.);
#33757=ORIENTED_EDGE('',*,*,#25486,.F.);
#33758=ORIENTED_EDGE('',*,*,#25237,.F.);
#33759=ORIENTED_EDGE('',*,*,#25487,.T.);
#33760=ORIENTED_EDGE('',*,*,#24113,.T.);
#33761=ORIENTED_EDGE('',*,*,#25488,.F.);
#33762=ORIENTED_EDGE('',*,*,#25230,.F.);
#33763=ORIENTED_EDGE('',*,*,#25489,.T.);
#33764=ORIENTED_EDGE('',*,*,#24114,.T.);
#33765=ORIENTED_EDGE('',*,*,#25487,.F.);
#33766=ORIENTED_EDGE('',*,*,#25229,.F.);
#33767=ORIENTED_EDGE('',*,*,#25490,.T.);
#33768=ORIENTED_EDGE('',*,*,#24115,.T.);
#33769=ORIENTED_EDGE('',*,*,#25489,.F.);
#33770=ORIENTED_EDGE('',*,*,#25234,.F.);
#33771=ORIENTED_EDGE('',*,*,#25491,.T.);
#33772=ORIENTED_EDGE('',*,*,#24116,.T.);
#33773=ORIENTED_EDGE('',*,*,#25490,.F.);
#33774=ORIENTED_EDGE('',*,*,#25233,.F.);
#33775=ORIENTED_EDGE('',*,*,#25492,.T.);
#33776=ORIENTED_EDGE('',*,*,#24117,.T.);
#33777=ORIENTED_EDGE('',*,*,#25491,.F.);
#33778=ORIENTED_EDGE('',*,*,#25232,.F.);
#33779=ORIENTED_EDGE('',*,*,#25488,.T.);
#33780=ORIENTED_EDGE('',*,*,#24118,.T.);
#33781=ORIENTED_EDGE('',*,*,#25492,.F.);
#33782=ORIENTED_EDGE('',*,*,#25231,.F.);
#33783=ORIENTED_EDGE('',*,*,#25493,.T.);
#33784=ORIENTED_EDGE('',*,*,#24107,.T.);
#33785=ORIENTED_EDGE('',*,*,#25494,.F.);
#33786=ORIENTED_EDGE('',*,*,#25224,.F.);
#33787=ORIENTED_EDGE('',*,*,#25495,.T.);
#33788=ORIENTED_EDGE('',*,*,#24108,.T.);
#33789=ORIENTED_EDGE('',*,*,#25493,.F.);
#33790=ORIENTED_EDGE('',*,*,#25223,.F.);
#33791=ORIENTED_EDGE('',*,*,#25496,.T.);
#33792=ORIENTED_EDGE('',*,*,#24109,.T.);
#33793=ORIENTED_EDGE('',*,*,#25495,.F.);
#33794=ORIENTED_EDGE('',*,*,#25228,.F.);
#33795=ORIENTED_EDGE('',*,*,#25497,.T.);
#33796=ORIENTED_EDGE('',*,*,#24110,.T.);
#33797=ORIENTED_EDGE('',*,*,#25496,.F.);
#33798=ORIENTED_EDGE('',*,*,#25227,.F.);
#33799=ORIENTED_EDGE('',*,*,#25498,.T.);
#33800=ORIENTED_EDGE('',*,*,#24111,.T.);
#33801=ORIENTED_EDGE('',*,*,#25497,.F.);
#33802=ORIENTED_EDGE('',*,*,#25226,.F.);
#33803=ORIENTED_EDGE('',*,*,#25494,.T.);
#33804=ORIENTED_EDGE('',*,*,#24112,.T.);
#33805=ORIENTED_EDGE('',*,*,#25498,.F.);
#33806=ORIENTED_EDGE('',*,*,#25225,.F.);
#33807=ORIENTED_EDGE('',*,*,#25499,.T.);
#33808=ORIENTED_EDGE('',*,*,#24101,.T.);
#33809=ORIENTED_EDGE('',*,*,#25500,.F.);
#33810=ORIENTED_EDGE('',*,*,#25218,.F.);
#33811=ORIENTED_EDGE('',*,*,#25501,.T.);
#33812=ORIENTED_EDGE('',*,*,#24102,.T.);
#33813=ORIENTED_EDGE('',*,*,#25499,.F.);
#33814=ORIENTED_EDGE('',*,*,#25217,.F.);
#33815=ORIENTED_EDGE('',*,*,#25502,.T.);
#33816=ORIENTED_EDGE('',*,*,#24103,.T.);
#33817=ORIENTED_EDGE('',*,*,#25501,.F.);
#33818=ORIENTED_EDGE('',*,*,#25222,.F.);
#33819=ORIENTED_EDGE('',*,*,#25503,.T.);
#33820=ORIENTED_EDGE('',*,*,#24104,.T.);
#33821=ORIENTED_EDGE('',*,*,#25502,.F.);
#33822=ORIENTED_EDGE('',*,*,#25221,.F.);
#33823=ORIENTED_EDGE('',*,*,#25504,.T.);
#33824=ORIENTED_EDGE('',*,*,#24105,.T.);
#33825=ORIENTED_EDGE('',*,*,#25503,.F.);
#33826=ORIENTED_EDGE('',*,*,#25220,.F.);
#33827=ORIENTED_EDGE('',*,*,#25500,.T.);
#33828=ORIENTED_EDGE('',*,*,#24106,.T.);
#33829=ORIENTED_EDGE('',*,*,#25504,.F.);
#33830=ORIENTED_EDGE('',*,*,#25219,.F.);
#33831=ORIENTED_EDGE('',*,*,#25505,.T.);
#33832=ORIENTED_EDGE('',*,*,#24095,.T.);
#33833=ORIENTED_EDGE('',*,*,#25506,.F.);
#33834=ORIENTED_EDGE('',*,*,#25212,.F.);
#33835=ORIENTED_EDGE('',*,*,#25507,.T.);
#33836=ORIENTED_EDGE('',*,*,#24096,.T.);
#33837=ORIENTED_EDGE('',*,*,#25505,.F.);
#33838=ORIENTED_EDGE('',*,*,#25211,.F.);
#33839=ORIENTED_EDGE('',*,*,#25508,.T.);
#33840=ORIENTED_EDGE('',*,*,#24097,.T.);
#33841=ORIENTED_EDGE('',*,*,#25507,.F.);
#33842=ORIENTED_EDGE('',*,*,#25216,.F.);
#33843=ORIENTED_EDGE('',*,*,#25509,.T.);
#33844=ORIENTED_EDGE('',*,*,#24098,.T.);
#33845=ORIENTED_EDGE('',*,*,#25508,.F.);
#33846=ORIENTED_EDGE('',*,*,#25215,.F.);
#33847=ORIENTED_EDGE('',*,*,#25510,.T.);
#33848=ORIENTED_EDGE('',*,*,#24099,.T.);
#33849=ORIENTED_EDGE('',*,*,#25509,.F.);
#33850=ORIENTED_EDGE('',*,*,#25214,.F.);
#33851=ORIENTED_EDGE('',*,*,#25506,.T.);
#33852=ORIENTED_EDGE('',*,*,#24100,.T.);
#33853=ORIENTED_EDGE('',*,*,#25510,.F.);
#33854=ORIENTED_EDGE('',*,*,#25213,.F.);
#33855=ORIENTED_EDGE('',*,*,#25511,.T.);
#33856=ORIENTED_EDGE('',*,*,#24089,.T.);
#33857=ORIENTED_EDGE('',*,*,#25512,.F.);
#33858=ORIENTED_EDGE('',*,*,#25206,.F.);
#33859=ORIENTED_EDGE('',*,*,#25513,.T.);
#33860=ORIENTED_EDGE('',*,*,#24090,.T.);
#33861=ORIENTED_EDGE('',*,*,#25511,.F.);
#33862=ORIENTED_EDGE('',*,*,#25205,.F.);
#33863=ORIENTED_EDGE('',*,*,#25514,.T.);
#33864=ORIENTED_EDGE('',*,*,#24091,.T.);
#33865=ORIENTED_EDGE('',*,*,#25513,.F.);
#33866=ORIENTED_EDGE('',*,*,#25210,.F.);
#33867=ORIENTED_EDGE('',*,*,#25515,.T.);
#33868=ORIENTED_EDGE('',*,*,#24092,.T.);
#33869=ORIENTED_EDGE('',*,*,#25514,.F.);
#33870=ORIENTED_EDGE('',*,*,#25209,.F.);
#33871=ORIENTED_EDGE('',*,*,#25516,.T.);
#33872=ORIENTED_EDGE('',*,*,#24093,.T.);
#33873=ORIENTED_EDGE('',*,*,#25515,.F.);
#33874=ORIENTED_EDGE('',*,*,#25208,.F.);
#33875=ORIENTED_EDGE('',*,*,#25512,.T.);
#33876=ORIENTED_EDGE('',*,*,#24094,.T.);
#33877=ORIENTED_EDGE('',*,*,#25516,.F.);
#33878=ORIENTED_EDGE('',*,*,#25207,.F.);
#33879=ORIENTED_EDGE('',*,*,#25517,.T.);
#33880=ORIENTED_EDGE('',*,*,#24083,.T.);
#33881=ORIENTED_EDGE('',*,*,#25518,.F.);
#33882=ORIENTED_EDGE('',*,*,#25200,.F.);
#33883=ORIENTED_EDGE('',*,*,#25519,.T.);
#33884=ORIENTED_EDGE('',*,*,#24084,.T.);
#33885=ORIENTED_EDGE('',*,*,#25517,.F.);
#33886=ORIENTED_EDGE('',*,*,#25199,.F.);
#33887=ORIENTED_EDGE('',*,*,#25520,.T.);
#33888=ORIENTED_EDGE('',*,*,#24085,.T.);
#33889=ORIENTED_EDGE('',*,*,#25519,.F.);
#33890=ORIENTED_EDGE('',*,*,#25204,.F.);
#33891=ORIENTED_EDGE('',*,*,#25521,.T.);
#33892=ORIENTED_EDGE('',*,*,#24086,.T.);
#33893=ORIENTED_EDGE('',*,*,#25520,.F.);
#33894=ORIENTED_EDGE('',*,*,#25203,.F.);
#33895=ORIENTED_EDGE('',*,*,#25522,.T.);
#33896=ORIENTED_EDGE('',*,*,#24087,.T.);
#33897=ORIENTED_EDGE('',*,*,#25521,.F.);
#33898=ORIENTED_EDGE('',*,*,#25202,.F.);
#33899=ORIENTED_EDGE('',*,*,#25518,.T.);
#33900=ORIENTED_EDGE('',*,*,#24088,.T.);
#33901=ORIENTED_EDGE('',*,*,#25522,.F.);
#33902=ORIENTED_EDGE('',*,*,#25201,.F.);
#33903=ORIENTED_EDGE('',*,*,#25523,.T.);
#33904=ORIENTED_EDGE('',*,*,#24077,.T.);
#33905=ORIENTED_EDGE('',*,*,#25524,.F.);
#33906=ORIENTED_EDGE('',*,*,#25194,.F.);
#33907=ORIENTED_EDGE('',*,*,#25525,.T.);
#33908=ORIENTED_EDGE('',*,*,#24078,.T.);
#33909=ORIENTED_EDGE('',*,*,#25523,.F.);
#33910=ORIENTED_EDGE('',*,*,#25193,.F.);
#33911=ORIENTED_EDGE('',*,*,#25526,.T.);
#33912=ORIENTED_EDGE('',*,*,#24079,.T.);
#33913=ORIENTED_EDGE('',*,*,#25525,.F.);
#33914=ORIENTED_EDGE('',*,*,#25198,.F.);
#33915=ORIENTED_EDGE('',*,*,#25527,.T.);
#33916=ORIENTED_EDGE('',*,*,#24080,.T.);
#33917=ORIENTED_EDGE('',*,*,#25526,.F.);
#33918=ORIENTED_EDGE('',*,*,#25197,.F.);
#33919=ORIENTED_EDGE('',*,*,#25528,.T.);
#33920=ORIENTED_EDGE('',*,*,#24081,.T.);
#33921=ORIENTED_EDGE('',*,*,#25527,.F.);
#33922=ORIENTED_EDGE('',*,*,#25196,.F.);
#33923=ORIENTED_EDGE('',*,*,#25524,.T.);
#33924=ORIENTED_EDGE('',*,*,#24082,.T.);
#33925=ORIENTED_EDGE('',*,*,#25528,.F.);
#33926=ORIENTED_EDGE('',*,*,#25195,.F.);
#33927=ORIENTED_EDGE('',*,*,#25529,.T.);
#33928=ORIENTED_EDGE('',*,*,#24071,.T.);
#33929=ORIENTED_EDGE('',*,*,#25530,.F.);
#33930=ORIENTED_EDGE('',*,*,#25188,.F.);
#33931=ORIENTED_EDGE('',*,*,#25531,.T.);
#33932=ORIENTED_EDGE('',*,*,#24072,.T.);
#33933=ORIENTED_EDGE('',*,*,#25529,.F.);
#33934=ORIENTED_EDGE('',*,*,#25187,.F.);
#33935=ORIENTED_EDGE('',*,*,#25532,.T.);
#33936=ORIENTED_EDGE('',*,*,#24073,.T.);
#33937=ORIENTED_EDGE('',*,*,#25531,.F.);
#33938=ORIENTED_EDGE('',*,*,#25192,.F.);
#33939=ORIENTED_EDGE('',*,*,#25533,.T.);
#33940=ORIENTED_EDGE('',*,*,#24074,.T.);
#33941=ORIENTED_EDGE('',*,*,#25532,.F.);
#33942=ORIENTED_EDGE('',*,*,#25191,.F.);
#33943=ORIENTED_EDGE('',*,*,#25534,.T.);
#33944=ORIENTED_EDGE('',*,*,#24075,.T.);
#33945=ORIENTED_EDGE('',*,*,#25533,.F.);
#33946=ORIENTED_EDGE('',*,*,#25190,.F.);
#33947=ORIENTED_EDGE('',*,*,#25530,.T.);
#33948=ORIENTED_EDGE('',*,*,#24076,.T.);
#33949=ORIENTED_EDGE('',*,*,#25534,.F.);
#33950=ORIENTED_EDGE('',*,*,#25189,.F.);
#33951=ORIENTED_EDGE('',*,*,#25535,.T.);
#33952=ORIENTED_EDGE('',*,*,#24065,.T.);
#33953=ORIENTED_EDGE('',*,*,#25536,.F.);
#33954=ORIENTED_EDGE('',*,*,#25182,.F.);
#33955=ORIENTED_EDGE('',*,*,#25537,.T.);
#33956=ORIENTED_EDGE('',*,*,#24066,.T.);
#33957=ORIENTED_EDGE('',*,*,#25535,.F.);
#33958=ORIENTED_EDGE('',*,*,#25181,.F.);
#33959=ORIENTED_EDGE('',*,*,#25538,.T.);
#33960=ORIENTED_EDGE('',*,*,#24067,.T.);
#33961=ORIENTED_EDGE('',*,*,#25537,.F.);
#33962=ORIENTED_EDGE('',*,*,#25186,.F.);
#33963=ORIENTED_EDGE('',*,*,#25539,.T.);
#33964=ORIENTED_EDGE('',*,*,#24068,.T.);
#33965=ORIENTED_EDGE('',*,*,#25538,.F.);
#33966=ORIENTED_EDGE('',*,*,#25185,.F.);
#33967=ORIENTED_EDGE('',*,*,#25540,.T.);
#33968=ORIENTED_EDGE('',*,*,#24069,.T.);
#33969=ORIENTED_EDGE('',*,*,#25539,.F.);
#33970=ORIENTED_EDGE('',*,*,#25184,.F.);
#33971=ORIENTED_EDGE('',*,*,#25536,.T.);
#33972=ORIENTED_EDGE('',*,*,#24070,.T.);
#33973=ORIENTED_EDGE('',*,*,#25540,.F.);
#33974=ORIENTED_EDGE('',*,*,#25183,.F.);
#33975=ORIENTED_EDGE('',*,*,#25541,.T.);
#33976=ORIENTED_EDGE('',*,*,#24059,.T.);
#33977=ORIENTED_EDGE('',*,*,#25542,.F.);
#33978=ORIENTED_EDGE('',*,*,#25176,.F.);
#33979=ORIENTED_EDGE('',*,*,#25543,.T.);
#33980=ORIENTED_EDGE('',*,*,#24060,.T.);
#33981=ORIENTED_EDGE('',*,*,#25541,.F.);
#33982=ORIENTED_EDGE('',*,*,#25175,.F.);
#33983=ORIENTED_EDGE('',*,*,#25544,.T.);
#33984=ORIENTED_EDGE('',*,*,#24061,.T.);
#33985=ORIENTED_EDGE('',*,*,#25543,.F.);
#33986=ORIENTED_EDGE('',*,*,#25180,.F.);
#33987=ORIENTED_EDGE('',*,*,#25545,.T.);
#33988=ORIENTED_EDGE('',*,*,#24062,.T.);
#33989=ORIENTED_EDGE('',*,*,#25544,.F.);
#33990=ORIENTED_EDGE('',*,*,#25179,.F.);
#33991=ORIENTED_EDGE('',*,*,#25546,.T.);
#33992=ORIENTED_EDGE('',*,*,#24063,.T.);
#33993=ORIENTED_EDGE('',*,*,#25545,.F.);
#33994=ORIENTED_EDGE('',*,*,#25178,.F.);
#33995=ORIENTED_EDGE('',*,*,#25542,.T.);
#33996=ORIENTED_EDGE('',*,*,#24064,.T.);
#33997=ORIENTED_EDGE('',*,*,#25546,.F.);
#33998=ORIENTED_EDGE('',*,*,#25177,.F.);
#33999=ORIENTED_EDGE('',*,*,#25547,.T.);
#34000=ORIENTED_EDGE('',*,*,#24053,.T.);
#34001=ORIENTED_EDGE('',*,*,#25548,.F.);
#34002=ORIENTED_EDGE('',*,*,#25170,.F.);
#34003=ORIENTED_EDGE('',*,*,#25549,.T.);
#34004=ORIENTED_EDGE('',*,*,#24054,.T.);
#34005=ORIENTED_EDGE('',*,*,#25547,.F.);
#34006=ORIENTED_EDGE('',*,*,#25169,.F.);
#34007=ORIENTED_EDGE('',*,*,#25550,.T.);
#34008=ORIENTED_EDGE('',*,*,#24055,.T.);
#34009=ORIENTED_EDGE('',*,*,#25549,.F.);
#34010=ORIENTED_EDGE('',*,*,#25174,.F.);
#34011=ORIENTED_EDGE('',*,*,#25551,.T.);
#34012=ORIENTED_EDGE('',*,*,#24056,.T.);
#34013=ORIENTED_EDGE('',*,*,#25550,.F.);
#34014=ORIENTED_EDGE('',*,*,#25173,.F.);
#34015=ORIENTED_EDGE('',*,*,#25552,.T.);
#34016=ORIENTED_EDGE('',*,*,#24057,.T.);
#34017=ORIENTED_EDGE('',*,*,#25551,.F.);
#34018=ORIENTED_EDGE('',*,*,#25172,.F.);
#34019=ORIENTED_EDGE('',*,*,#25548,.T.);
#34020=ORIENTED_EDGE('',*,*,#24058,.T.);
#34021=ORIENTED_EDGE('',*,*,#25552,.F.);
#34022=ORIENTED_EDGE('',*,*,#25171,.F.);
#34023=ORIENTED_EDGE('',*,*,#25553,.T.);
#34024=ORIENTED_EDGE('',*,*,#24047,.T.);
#34025=ORIENTED_EDGE('',*,*,#25554,.F.);
#34026=ORIENTED_EDGE('',*,*,#25164,.F.);
#34027=ORIENTED_EDGE('',*,*,#25555,.T.);
#34028=ORIENTED_EDGE('',*,*,#24048,.T.);
#34029=ORIENTED_EDGE('',*,*,#25553,.F.);
#34030=ORIENTED_EDGE('',*,*,#25163,.F.);
#34031=ORIENTED_EDGE('',*,*,#25556,.T.);
#34032=ORIENTED_EDGE('',*,*,#24049,.T.);
#34033=ORIENTED_EDGE('',*,*,#25555,.F.);
#34034=ORIENTED_EDGE('',*,*,#25168,.F.);
#34035=ORIENTED_EDGE('',*,*,#25557,.T.);
#34036=ORIENTED_EDGE('',*,*,#24050,.T.);
#34037=ORIENTED_EDGE('',*,*,#25556,.F.);
#34038=ORIENTED_EDGE('',*,*,#25167,.F.);
#34039=ORIENTED_EDGE('',*,*,#25558,.T.);
#34040=ORIENTED_EDGE('',*,*,#24051,.T.);
#34041=ORIENTED_EDGE('',*,*,#25557,.F.);
#34042=ORIENTED_EDGE('',*,*,#25166,.F.);
#34043=ORIENTED_EDGE('',*,*,#25554,.T.);
#34044=ORIENTED_EDGE('',*,*,#24052,.T.);
#34045=ORIENTED_EDGE('',*,*,#25558,.F.);
#34046=ORIENTED_EDGE('',*,*,#25165,.F.);
#34047=ORIENTED_EDGE('',*,*,#25559,.T.);
#34048=ORIENTED_EDGE('',*,*,#24041,.T.);
#34049=ORIENTED_EDGE('',*,*,#25560,.F.);
#34050=ORIENTED_EDGE('',*,*,#25158,.F.);
#34051=ORIENTED_EDGE('',*,*,#25561,.T.);
#34052=ORIENTED_EDGE('',*,*,#24042,.T.);
#34053=ORIENTED_EDGE('',*,*,#25559,.F.);
#34054=ORIENTED_EDGE('',*,*,#25157,.F.);
#34055=ORIENTED_EDGE('',*,*,#25562,.T.);
#34056=ORIENTED_EDGE('',*,*,#24043,.T.);
#34057=ORIENTED_EDGE('',*,*,#25561,.F.);
#34058=ORIENTED_EDGE('',*,*,#25162,.F.);
#34059=ORIENTED_EDGE('',*,*,#25563,.T.);
#34060=ORIENTED_EDGE('',*,*,#24044,.T.);
#34061=ORIENTED_EDGE('',*,*,#25562,.F.);
#34062=ORIENTED_EDGE('',*,*,#25161,.F.);
#34063=ORIENTED_EDGE('',*,*,#25564,.T.);
#34064=ORIENTED_EDGE('',*,*,#24045,.T.);
#34065=ORIENTED_EDGE('',*,*,#25563,.F.);
#34066=ORIENTED_EDGE('',*,*,#25160,.F.);
#34067=ORIENTED_EDGE('',*,*,#25560,.T.);
#34068=ORIENTED_EDGE('',*,*,#24046,.T.);
#34069=ORIENTED_EDGE('',*,*,#25564,.F.);
#34070=ORIENTED_EDGE('',*,*,#25159,.F.);
#34071=ORIENTED_EDGE('',*,*,#25565,.T.);
#34072=ORIENTED_EDGE('',*,*,#24035,.T.);
#34073=ORIENTED_EDGE('',*,*,#25566,.F.);
#34074=ORIENTED_EDGE('',*,*,#25152,.F.);
#34075=ORIENTED_EDGE('',*,*,#25567,.T.);
#34076=ORIENTED_EDGE('',*,*,#24036,.T.);
#34077=ORIENTED_EDGE('',*,*,#25565,.F.);
#34078=ORIENTED_EDGE('',*,*,#25151,.F.);
#34079=ORIENTED_EDGE('',*,*,#25568,.T.);
#34080=ORIENTED_EDGE('',*,*,#24037,.T.);
#34081=ORIENTED_EDGE('',*,*,#25567,.F.);
#34082=ORIENTED_EDGE('',*,*,#25156,.F.);
#34083=ORIENTED_EDGE('',*,*,#25569,.T.);
#34084=ORIENTED_EDGE('',*,*,#24038,.T.);
#34085=ORIENTED_EDGE('',*,*,#25568,.F.);
#34086=ORIENTED_EDGE('',*,*,#25155,.F.);
#34087=ORIENTED_EDGE('',*,*,#25570,.T.);
#34088=ORIENTED_EDGE('',*,*,#24039,.T.);
#34089=ORIENTED_EDGE('',*,*,#25569,.F.);
#34090=ORIENTED_EDGE('',*,*,#25154,.F.);
#34091=ORIENTED_EDGE('',*,*,#25566,.T.);
#34092=ORIENTED_EDGE('',*,*,#24040,.T.);
#34093=ORIENTED_EDGE('',*,*,#25570,.F.);
#34094=ORIENTED_EDGE('',*,*,#25153,.F.);
#34095=ORIENTED_EDGE('',*,*,#25571,.T.);
#34096=ORIENTED_EDGE('',*,*,#24029,.T.);
#34097=ORIENTED_EDGE('',*,*,#25572,.F.);
#34098=ORIENTED_EDGE('',*,*,#25146,.F.);
#34099=ORIENTED_EDGE('',*,*,#25573,.T.);
#34100=ORIENTED_EDGE('',*,*,#24030,.T.);
#34101=ORIENTED_EDGE('',*,*,#25571,.F.);
#34102=ORIENTED_EDGE('',*,*,#25145,.F.);
#34103=ORIENTED_EDGE('',*,*,#25574,.T.);
#34104=ORIENTED_EDGE('',*,*,#24031,.T.);
#34105=ORIENTED_EDGE('',*,*,#25573,.F.);
#34106=ORIENTED_EDGE('',*,*,#25150,.F.);
#34107=ORIENTED_EDGE('',*,*,#25575,.T.);
#34108=ORIENTED_EDGE('',*,*,#24032,.T.);
#34109=ORIENTED_EDGE('',*,*,#25574,.F.);
#34110=ORIENTED_EDGE('',*,*,#25149,.F.);
#34111=ORIENTED_EDGE('',*,*,#25576,.T.);
#34112=ORIENTED_EDGE('',*,*,#24033,.T.);
#34113=ORIENTED_EDGE('',*,*,#25575,.F.);
#34114=ORIENTED_EDGE('',*,*,#25148,.F.);
#34115=ORIENTED_EDGE('',*,*,#25572,.T.);
#34116=ORIENTED_EDGE('',*,*,#24034,.T.);
#34117=ORIENTED_EDGE('',*,*,#25576,.F.);
#34118=ORIENTED_EDGE('',*,*,#25147,.F.);
#34119=ORIENTED_EDGE('',*,*,#25577,.T.);
#34120=ORIENTED_EDGE('',*,*,#24023,.T.);
#34121=ORIENTED_EDGE('',*,*,#25578,.F.);
#34122=ORIENTED_EDGE('',*,*,#25140,.F.);
#34123=ORIENTED_EDGE('',*,*,#25579,.T.);
#34124=ORIENTED_EDGE('',*,*,#24024,.T.);
#34125=ORIENTED_EDGE('',*,*,#25577,.F.);
#34126=ORIENTED_EDGE('',*,*,#25139,.F.);
#34127=ORIENTED_EDGE('',*,*,#25580,.T.);
#34128=ORIENTED_EDGE('',*,*,#24025,.T.);
#34129=ORIENTED_EDGE('',*,*,#25579,.F.);
#34130=ORIENTED_EDGE('',*,*,#25144,.F.);
#34131=ORIENTED_EDGE('',*,*,#25581,.T.);
#34132=ORIENTED_EDGE('',*,*,#24026,.T.);
#34133=ORIENTED_EDGE('',*,*,#25580,.F.);
#34134=ORIENTED_EDGE('',*,*,#25143,.F.);
#34135=ORIENTED_EDGE('',*,*,#25582,.T.);
#34136=ORIENTED_EDGE('',*,*,#24027,.T.);
#34137=ORIENTED_EDGE('',*,*,#25581,.F.);
#34138=ORIENTED_EDGE('',*,*,#25142,.F.);
#34139=ORIENTED_EDGE('',*,*,#25578,.T.);
#34140=ORIENTED_EDGE('',*,*,#24028,.T.);
#34141=ORIENTED_EDGE('',*,*,#25582,.F.);
#34142=ORIENTED_EDGE('',*,*,#25141,.F.);
#34143=ORIENTED_EDGE('',*,*,#25583,.T.);
#34144=ORIENTED_EDGE('',*,*,#24017,.T.);
#34145=ORIENTED_EDGE('',*,*,#25584,.F.);
#34146=ORIENTED_EDGE('',*,*,#25134,.F.);
#34147=ORIENTED_EDGE('',*,*,#25585,.T.);
#34148=ORIENTED_EDGE('',*,*,#24018,.T.);
#34149=ORIENTED_EDGE('',*,*,#25583,.F.);
#34150=ORIENTED_EDGE('',*,*,#25133,.F.);
#34151=ORIENTED_EDGE('',*,*,#25586,.T.);
#34152=ORIENTED_EDGE('',*,*,#24019,.T.);
#34153=ORIENTED_EDGE('',*,*,#25585,.F.);
#34154=ORIENTED_EDGE('',*,*,#25138,.F.);
#34155=ORIENTED_EDGE('',*,*,#25587,.T.);
#34156=ORIENTED_EDGE('',*,*,#24020,.T.);
#34157=ORIENTED_EDGE('',*,*,#25586,.F.);
#34158=ORIENTED_EDGE('',*,*,#25137,.F.);
#34159=ORIENTED_EDGE('',*,*,#25588,.T.);
#34160=ORIENTED_EDGE('',*,*,#24021,.T.);
#34161=ORIENTED_EDGE('',*,*,#25587,.F.);
#34162=ORIENTED_EDGE('',*,*,#25136,.F.);
#34163=ORIENTED_EDGE('',*,*,#25584,.T.);
#34164=ORIENTED_EDGE('',*,*,#24022,.T.);
#34165=ORIENTED_EDGE('',*,*,#25588,.F.);
#34166=ORIENTED_EDGE('',*,*,#25135,.F.);
#34167=ORIENTED_EDGE('',*,*,#25589,.T.);
#34168=ORIENTED_EDGE('',*,*,#24011,.T.);
#34169=ORIENTED_EDGE('',*,*,#25590,.F.);
#34170=ORIENTED_EDGE('',*,*,#25128,.F.);
#34171=ORIENTED_EDGE('',*,*,#25591,.T.);
#34172=ORIENTED_EDGE('',*,*,#24012,.T.);
#34173=ORIENTED_EDGE('',*,*,#25589,.F.);
#34174=ORIENTED_EDGE('',*,*,#25127,.F.);
#34175=ORIENTED_EDGE('',*,*,#25592,.T.);
#34176=ORIENTED_EDGE('',*,*,#24013,.T.);
#34177=ORIENTED_EDGE('',*,*,#25591,.F.);
#34178=ORIENTED_EDGE('',*,*,#25132,.F.);
#34179=ORIENTED_EDGE('',*,*,#25593,.T.);
#34180=ORIENTED_EDGE('',*,*,#24014,.T.);
#34181=ORIENTED_EDGE('',*,*,#25592,.F.);
#34182=ORIENTED_EDGE('',*,*,#25131,.F.);
#34183=ORIENTED_EDGE('',*,*,#25594,.T.);
#34184=ORIENTED_EDGE('',*,*,#24015,.T.);
#34185=ORIENTED_EDGE('',*,*,#25593,.F.);
#34186=ORIENTED_EDGE('',*,*,#25130,.F.);
#34187=ORIENTED_EDGE('',*,*,#25590,.T.);
#34188=ORIENTED_EDGE('',*,*,#24016,.T.);
#34189=ORIENTED_EDGE('',*,*,#25594,.F.);
#34190=ORIENTED_EDGE('',*,*,#25129,.F.);
#34191=ORIENTED_EDGE('',*,*,#25595,.T.);
#34192=ORIENTED_EDGE('',*,*,#24005,.T.);
#34193=ORIENTED_EDGE('',*,*,#25596,.F.);
#34194=ORIENTED_EDGE('',*,*,#25122,.F.);
#34195=ORIENTED_EDGE('',*,*,#25597,.T.);
#34196=ORIENTED_EDGE('',*,*,#24006,.T.);
#34197=ORIENTED_EDGE('',*,*,#25595,.F.);
#34198=ORIENTED_EDGE('',*,*,#25121,.F.);
#34199=ORIENTED_EDGE('',*,*,#25598,.T.);
#34200=ORIENTED_EDGE('',*,*,#24007,.T.);
#34201=ORIENTED_EDGE('',*,*,#25597,.F.);
#34202=ORIENTED_EDGE('',*,*,#25126,.F.);
#34203=ORIENTED_EDGE('',*,*,#25599,.T.);
#34204=ORIENTED_EDGE('',*,*,#24008,.T.);
#34205=ORIENTED_EDGE('',*,*,#25598,.F.);
#34206=ORIENTED_EDGE('',*,*,#25125,.F.);
#34207=ORIENTED_EDGE('',*,*,#25600,.T.);
#34208=ORIENTED_EDGE('',*,*,#24009,.T.);
#34209=ORIENTED_EDGE('',*,*,#25599,.F.);
#34210=ORIENTED_EDGE('',*,*,#25124,.F.);
#34211=ORIENTED_EDGE('',*,*,#25596,.T.);
#34212=ORIENTED_EDGE('',*,*,#24010,.T.);
#34213=ORIENTED_EDGE('',*,*,#25600,.F.);
#34214=ORIENTED_EDGE('',*,*,#25123,.F.);
#34215=ORIENTED_EDGE('',*,*,#25601,.T.);
#34216=ORIENTED_EDGE('',*,*,#23999,.T.);
#34217=ORIENTED_EDGE('',*,*,#25602,.F.);
#34218=ORIENTED_EDGE('',*,*,#25116,.F.);
#34219=ORIENTED_EDGE('',*,*,#25603,.T.);
#34220=ORIENTED_EDGE('',*,*,#24000,.T.);
#34221=ORIENTED_EDGE('',*,*,#25601,.F.);
#34222=ORIENTED_EDGE('',*,*,#25115,.F.);
#34223=ORIENTED_EDGE('',*,*,#25604,.T.);
#34224=ORIENTED_EDGE('',*,*,#24001,.T.);
#34225=ORIENTED_EDGE('',*,*,#25603,.F.);
#34226=ORIENTED_EDGE('',*,*,#25120,.F.);
#34227=ORIENTED_EDGE('',*,*,#25605,.T.);
#34228=ORIENTED_EDGE('',*,*,#24002,.T.);
#34229=ORIENTED_EDGE('',*,*,#25604,.F.);
#34230=ORIENTED_EDGE('',*,*,#25119,.F.);
#34231=ORIENTED_EDGE('',*,*,#25606,.T.);
#34232=ORIENTED_EDGE('',*,*,#24003,.T.);
#34233=ORIENTED_EDGE('',*,*,#25605,.F.);
#34234=ORIENTED_EDGE('',*,*,#25118,.F.);
#34235=ORIENTED_EDGE('',*,*,#25602,.T.);
#34236=ORIENTED_EDGE('',*,*,#24004,.T.);
#34237=ORIENTED_EDGE('',*,*,#25606,.F.);
#34238=ORIENTED_EDGE('',*,*,#25117,.F.);
#34239=ORIENTED_EDGE('',*,*,#25607,.T.);
#34240=ORIENTED_EDGE('',*,*,#23993,.T.);
#34241=ORIENTED_EDGE('',*,*,#25608,.F.);
#34242=ORIENTED_EDGE('',*,*,#25110,.F.);
#34243=ORIENTED_EDGE('',*,*,#25609,.T.);
#34244=ORIENTED_EDGE('',*,*,#23994,.T.);
#34245=ORIENTED_EDGE('',*,*,#25607,.F.);
#34246=ORIENTED_EDGE('',*,*,#25109,.F.);
#34247=ORIENTED_EDGE('',*,*,#25610,.T.);
#34248=ORIENTED_EDGE('',*,*,#23995,.T.);
#34249=ORIENTED_EDGE('',*,*,#25609,.F.);
#34250=ORIENTED_EDGE('',*,*,#25114,.F.);
#34251=ORIENTED_EDGE('',*,*,#25611,.T.);
#34252=ORIENTED_EDGE('',*,*,#23996,.T.);
#34253=ORIENTED_EDGE('',*,*,#25610,.F.);
#34254=ORIENTED_EDGE('',*,*,#25113,.F.);
#34255=ORIENTED_EDGE('',*,*,#25612,.T.);
#34256=ORIENTED_EDGE('',*,*,#23997,.T.);
#34257=ORIENTED_EDGE('',*,*,#25611,.F.);
#34258=ORIENTED_EDGE('',*,*,#25112,.F.);
#34259=ORIENTED_EDGE('',*,*,#25608,.T.);
#34260=ORIENTED_EDGE('',*,*,#23998,.T.);
#34261=ORIENTED_EDGE('',*,*,#25612,.F.);
#34262=ORIENTED_EDGE('',*,*,#25111,.F.);
#34263=ORIENTED_EDGE('',*,*,#25613,.T.);
#34264=ORIENTED_EDGE('',*,*,#23987,.T.);
#34265=ORIENTED_EDGE('',*,*,#25614,.F.);
#34266=ORIENTED_EDGE('',*,*,#25104,.F.);
#34267=ORIENTED_EDGE('',*,*,#25615,.T.);
#34268=ORIENTED_EDGE('',*,*,#23988,.T.);
#34269=ORIENTED_EDGE('',*,*,#25613,.F.);
#34270=ORIENTED_EDGE('',*,*,#25103,.F.);
#34271=ORIENTED_EDGE('',*,*,#25616,.T.);
#34272=ORIENTED_EDGE('',*,*,#23989,.T.);
#34273=ORIENTED_EDGE('',*,*,#25615,.F.);
#34274=ORIENTED_EDGE('',*,*,#25108,.F.);
#34275=ORIENTED_EDGE('',*,*,#25617,.T.);
#34276=ORIENTED_EDGE('',*,*,#23990,.T.);
#34277=ORIENTED_EDGE('',*,*,#25616,.F.);
#34278=ORIENTED_EDGE('',*,*,#25107,.F.);
#34279=ORIENTED_EDGE('',*,*,#25618,.T.);
#34280=ORIENTED_EDGE('',*,*,#23991,.T.);
#34281=ORIENTED_EDGE('',*,*,#25617,.F.);
#34282=ORIENTED_EDGE('',*,*,#25106,.F.);
#34283=ORIENTED_EDGE('',*,*,#25614,.T.);
#34284=ORIENTED_EDGE('',*,*,#23992,.T.);
#34285=ORIENTED_EDGE('',*,*,#25618,.F.);
#34286=ORIENTED_EDGE('',*,*,#25105,.F.);
#34287=ORIENTED_EDGE('',*,*,#25619,.T.);
#34288=ORIENTED_EDGE('',*,*,#23981,.T.);
#34289=ORIENTED_EDGE('',*,*,#25620,.F.);
#34290=ORIENTED_EDGE('',*,*,#25098,.F.);
#34291=ORIENTED_EDGE('',*,*,#25621,.T.);
#34292=ORIENTED_EDGE('',*,*,#23982,.T.);
#34293=ORIENTED_EDGE('',*,*,#25619,.F.);
#34294=ORIENTED_EDGE('',*,*,#25097,.F.);
#34295=ORIENTED_EDGE('',*,*,#25622,.T.);
#34296=ORIENTED_EDGE('',*,*,#23983,.T.);
#34297=ORIENTED_EDGE('',*,*,#25621,.F.);
#34298=ORIENTED_EDGE('',*,*,#25102,.F.);
#34299=ORIENTED_EDGE('',*,*,#25623,.T.);
#34300=ORIENTED_EDGE('',*,*,#23984,.T.);
#34301=ORIENTED_EDGE('',*,*,#25622,.F.);
#34302=ORIENTED_EDGE('',*,*,#25101,.F.);
#34303=ORIENTED_EDGE('',*,*,#25624,.T.);
#34304=ORIENTED_EDGE('',*,*,#23985,.T.);
#34305=ORIENTED_EDGE('',*,*,#25623,.F.);
#34306=ORIENTED_EDGE('',*,*,#25100,.F.);
#34307=ORIENTED_EDGE('',*,*,#25620,.T.);
#34308=ORIENTED_EDGE('',*,*,#23986,.T.);
#34309=ORIENTED_EDGE('',*,*,#25624,.F.);
#34310=ORIENTED_EDGE('',*,*,#25099,.F.);
#34311=ORIENTED_EDGE('',*,*,#25625,.T.);
#34312=ORIENTED_EDGE('',*,*,#23975,.T.);
#34313=ORIENTED_EDGE('',*,*,#25626,.F.);
#34314=ORIENTED_EDGE('',*,*,#25092,.F.);
#34315=ORIENTED_EDGE('',*,*,#25627,.T.);
#34316=ORIENTED_EDGE('',*,*,#23976,.T.);
#34317=ORIENTED_EDGE('',*,*,#25625,.F.);
#34318=ORIENTED_EDGE('',*,*,#25091,.F.);
#34319=ORIENTED_EDGE('',*,*,#25628,.T.);
#34320=ORIENTED_EDGE('',*,*,#23977,.T.);
#34321=ORIENTED_EDGE('',*,*,#25627,.F.);
#34322=ORIENTED_EDGE('',*,*,#25096,.F.);
#34323=ORIENTED_EDGE('',*,*,#25629,.T.);
#34324=ORIENTED_EDGE('',*,*,#23978,.T.);
#34325=ORIENTED_EDGE('',*,*,#25628,.F.);
#34326=ORIENTED_EDGE('',*,*,#25095,.F.);
#34327=ORIENTED_EDGE('',*,*,#25630,.T.);
#34328=ORIENTED_EDGE('',*,*,#23979,.T.);
#34329=ORIENTED_EDGE('',*,*,#25629,.F.);
#34330=ORIENTED_EDGE('',*,*,#25094,.F.);
#34331=ORIENTED_EDGE('',*,*,#25626,.T.);
#34332=ORIENTED_EDGE('',*,*,#23980,.T.);
#34333=ORIENTED_EDGE('',*,*,#25630,.F.);
#34334=ORIENTED_EDGE('',*,*,#25093,.F.);
#34335=ORIENTED_EDGE('',*,*,#25631,.T.);
#34336=ORIENTED_EDGE('',*,*,#23969,.T.);
#34337=ORIENTED_EDGE('',*,*,#25632,.F.);
#34338=ORIENTED_EDGE('',*,*,#25086,.F.);
#34339=ORIENTED_EDGE('',*,*,#25633,.T.);
#34340=ORIENTED_EDGE('',*,*,#23970,.T.);
#34341=ORIENTED_EDGE('',*,*,#25631,.F.);
#34342=ORIENTED_EDGE('',*,*,#25085,.F.);
#34343=ORIENTED_EDGE('',*,*,#25634,.T.);
#34344=ORIENTED_EDGE('',*,*,#23971,.T.);
#34345=ORIENTED_EDGE('',*,*,#25633,.F.);
#34346=ORIENTED_EDGE('',*,*,#25090,.F.);
#34347=ORIENTED_EDGE('',*,*,#25635,.T.);
#34348=ORIENTED_EDGE('',*,*,#23972,.T.);
#34349=ORIENTED_EDGE('',*,*,#25634,.F.);
#34350=ORIENTED_EDGE('',*,*,#25089,.F.);
#34351=ORIENTED_EDGE('',*,*,#25636,.T.);
#34352=ORIENTED_EDGE('',*,*,#23973,.T.);
#34353=ORIENTED_EDGE('',*,*,#25635,.F.);
#34354=ORIENTED_EDGE('',*,*,#25088,.F.);
#34355=ORIENTED_EDGE('',*,*,#25632,.T.);
#34356=ORIENTED_EDGE('',*,*,#23974,.T.);
#34357=ORIENTED_EDGE('',*,*,#25636,.F.);
#34358=ORIENTED_EDGE('',*,*,#25087,.F.);
#34359=ORIENTED_EDGE('',*,*,#25637,.T.);
#34360=ORIENTED_EDGE('',*,*,#23963,.T.);
#34361=ORIENTED_EDGE('',*,*,#25638,.F.);
#34362=ORIENTED_EDGE('',*,*,#25080,.F.);
#34363=ORIENTED_EDGE('',*,*,#25639,.T.);
#34364=ORIENTED_EDGE('',*,*,#23964,.T.);
#34365=ORIENTED_EDGE('',*,*,#25637,.F.);
#34366=ORIENTED_EDGE('',*,*,#25079,.F.);
#34367=ORIENTED_EDGE('',*,*,#25640,.T.);
#34368=ORIENTED_EDGE('',*,*,#23965,.T.);
#34369=ORIENTED_EDGE('',*,*,#25639,.F.);
#34370=ORIENTED_EDGE('',*,*,#25084,.F.);
#34371=ORIENTED_EDGE('',*,*,#25641,.T.);
#34372=ORIENTED_EDGE('',*,*,#23966,.T.);
#34373=ORIENTED_EDGE('',*,*,#25640,.F.);
#34374=ORIENTED_EDGE('',*,*,#25083,.F.);
#34375=ORIENTED_EDGE('',*,*,#25642,.T.);
#34376=ORIENTED_EDGE('',*,*,#23967,.T.);
#34377=ORIENTED_EDGE('',*,*,#25641,.F.);
#34378=ORIENTED_EDGE('',*,*,#25082,.F.);
#34379=ORIENTED_EDGE('',*,*,#25638,.T.);
#34380=ORIENTED_EDGE('',*,*,#23968,.T.);
#34381=ORIENTED_EDGE('',*,*,#25642,.F.);
#34382=ORIENTED_EDGE('',*,*,#25081,.F.);
#34383=ORIENTED_EDGE('',*,*,#25643,.T.);
#34384=ORIENTED_EDGE('',*,*,#23957,.T.);
#34385=ORIENTED_EDGE('',*,*,#25644,.F.);
#34386=ORIENTED_EDGE('',*,*,#25074,.F.);
#34387=ORIENTED_EDGE('',*,*,#25645,.T.);
#34388=ORIENTED_EDGE('',*,*,#23958,.T.);
#34389=ORIENTED_EDGE('',*,*,#25643,.F.);
#34390=ORIENTED_EDGE('',*,*,#25073,.F.);
#34391=ORIENTED_EDGE('',*,*,#25646,.T.);
#34392=ORIENTED_EDGE('',*,*,#23959,.T.);
#34393=ORIENTED_EDGE('',*,*,#25645,.F.);
#34394=ORIENTED_EDGE('',*,*,#25078,.F.);
#34395=ORIENTED_EDGE('',*,*,#25647,.T.);
#34396=ORIENTED_EDGE('',*,*,#23960,.T.);
#34397=ORIENTED_EDGE('',*,*,#25646,.F.);
#34398=ORIENTED_EDGE('',*,*,#25077,.F.);
#34399=ORIENTED_EDGE('',*,*,#25648,.T.);
#34400=ORIENTED_EDGE('',*,*,#23961,.T.);
#34401=ORIENTED_EDGE('',*,*,#25647,.F.);
#34402=ORIENTED_EDGE('',*,*,#25076,.F.);
#34403=ORIENTED_EDGE('',*,*,#25644,.T.);
#34404=ORIENTED_EDGE('',*,*,#23962,.T.);
#34405=ORIENTED_EDGE('',*,*,#25648,.F.);
#34406=ORIENTED_EDGE('',*,*,#25075,.F.);
#34407=ORIENTED_EDGE('',*,*,#25649,.T.);
#34408=ORIENTED_EDGE('',*,*,#23951,.T.);
#34409=ORIENTED_EDGE('',*,*,#25650,.F.);
#34410=ORIENTED_EDGE('',*,*,#25068,.F.);
#34411=ORIENTED_EDGE('',*,*,#25651,.T.);
#34412=ORIENTED_EDGE('',*,*,#23952,.T.);
#34413=ORIENTED_EDGE('',*,*,#25649,.F.);
#34414=ORIENTED_EDGE('',*,*,#25067,.F.);
#34415=ORIENTED_EDGE('',*,*,#25652,.T.);
#34416=ORIENTED_EDGE('',*,*,#23953,.T.);
#34417=ORIENTED_EDGE('',*,*,#25651,.F.);
#34418=ORIENTED_EDGE('',*,*,#25072,.F.);
#34419=ORIENTED_EDGE('',*,*,#25653,.T.);
#34420=ORIENTED_EDGE('',*,*,#23954,.T.);
#34421=ORIENTED_EDGE('',*,*,#25652,.F.);
#34422=ORIENTED_EDGE('',*,*,#25071,.F.);
#34423=ORIENTED_EDGE('',*,*,#25654,.T.);
#34424=ORIENTED_EDGE('',*,*,#23955,.T.);
#34425=ORIENTED_EDGE('',*,*,#25653,.F.);
#34426=ORIENTED_EDGE('',*,*,#25070,.F.);
#34427=ORIENTED_EDGE('',*,*,#25650,.T.);
#34428=ORIENTED_EDGE('',*,*,#23956,.T.);
#34429=ORIENTED_EDGE('',*,*,#25654,.F.);
#34430=ORIENTED_EDGE('',*,*,#25069,.F.);
#34431=ORIENTED_EDGE('',*,*,#25655,.T.);
#34432=ORIENTED_EDGE('',*,*,#23945,.T.);
#34433=ORIENTED_EDGE('',*,*,#25656,.F.);
#34434=ORIENTED_EDGE('',*,*,#25062,.F.);
#34435=ORIENTED_EDGE('',*,*,#25657,.T.);
#34436=ORIENTED_EDGE('',*,*,#23946,.T.);
#34437=ORIENTED_EDGE('',*,*,#25655,.F.);
#34438=ORIENTED_EDGE('',*,*,#25061,.F.);
#34439=ORIENTED_EDGE('',*,*,#25658,.T.);
#34440=ORIENTED_EDGE('',*,*,#23947,.T.);
#34441=ORIENTED_EDGE('',*,*,#25657,.F.);
#34442=ORIENTED_EDGE('',*,*,#25066,.F.);
#34443=ORIENTED_EDGE('',*,*,#25659,.T.);
#34444=ORIENTED_EDGE('',*,*,#23948,.T.);
#34445=ORIENTED_EDGE('',*,*,#25658,.F.);
#34446=ORIENTED_EDGE('',*,*,#25065,.F.);
#34447=ORIENTED_EDGE('',*,*,#25660,.T.);
#34448=ORIENTED_EDGE('',*,*,#23949,.T.);
#34449=ORIENTED_EDGE('',*,*,#25659,.F.);
#34450=ORIENTED_EDGE('',*,*,#25064,.F.);
#34451=ORIENTED_EDGE('',*,*,#25656,.T.);
#34452=ORIENTED_EDGE('',*,*,#23950,.T.);
#34453=ORIENTED_EDGE('',*,*,#25660,.F.);
#34454=ORIENTED_EDGE('',*,*,#25063,.F.);
#34455=ORIENTED_EDGE('',*,*,#25661,.T.);
#34456=ORIENTED_EDGE('',*,*,#23939,.T.);
#34457=ORIENTED_EDGE('',*,*,#25662,.F.);
#34458=ORIENTED_EDGE('',*,*,#25056,.F.);
#34459=ORIENTED_EDGE('',*,*,#25663,.T.);
#34460=ORIENTED_EDGE('',*,*,#23940,.T.);
#34461=ORIENTED_EDGE('',*,*,#25661,.F.);
#34462=ORIENTED_EDGE('',*,*,#25055,.F.);
#34463=ORIENTED_EDGE('',*,*,#25664,.T.);
#34464=ORIENTED_EDGE('',*,*,#23941,.T.);
#34465=ORIENTED_EDGE('',*,*,#25663,.F.);
#34466=ORIENTED_EDGE('',*,*,#25060,.F.);
#34467=ORIENTED_EDGE('',*,*,#25665,.T.);
#34468=ORIENTED_EDGE('',*,*,#23942,.T.);
#34469=ORIENTED_EDGE('',*,*,#25664,.F.);
#34470=ORIENTED_EDGE('',*,*,#25059,.F.);
#34471=ORIENTED_EDGE('',*,*,#25666,.T.);
#34472=ORIENTED_EDGE('',*,*,#23943,.T.);
#34473=ORIENTED_EDGE('',*,*,#25665,.F.);
#34474=ORIENTED_EDGE('',*,*,#25058,.F.);
#34475=ORIENTED_EDGE('',*,*,#25662,.T.);
#34476=ORIENTED_EDGE('',*,*,#23944,.T.);
#34477=ORIENTED_EDGE('',*,*,#25666,.F.);
#34478=ORIENTED_EDGE('',*,*,#25057,.F.);
#34479=ORIENTED_EDGE('',*,*,#25667,.T.);
#34480=ORIENTED_EDGE('',*,*,#23933,.T.);
#34481=ORIENTED_EDGE('',*,*,#25668,.F.);
#34482=ORIENTED_EDGE('',*,*,#25050,.F.);
#34483=ORIENTED_EDGE('',*,*,#25669,.T.);
#34484=ORIENTED_EDGE('',*,*,#23934,.T.);
#34485=ORIENTED_EDGE('',*,*,#25667,.F.);
#34486=ORIENTED_EDGE('',*,*,#25049,.F.);
#34487=ORIENTED_EDGE('',*,*,#25670,.T.);
#34488=ORIENTED_EDGE('',*,*,#23935,.T.);
#34489=ORIENTED_EDGE('',*,*,#25669,.F.);
#34490=ORIENTED_EDGE('',*,*,#25054,.F.);
#34491=ORIENTED_EDGE('',*,*,#25671,.T.);
#34492=ORIENTED_EDGE('',*,*,#23936,.T.);
#34493=ORIENTED_EDGE('',*,*,#25670,.F.);
#34494=ORIENTED_EDGE('',*,*,#25053,.F.);
#34495=ORIENTED_EDGE('',*,*,#25672,.T.);
#34496=ORIENTED_EDGE('',*,*,#23937,.T.);
#34497=ORIENTED_EDGE('',*,*,#25671,.F.);
#34498=ORIENTED_EDGE('',*,*,#25052,.F.);
#34499=ORIENTED_EDGE('',*,*,#25668,.T.);
#34500=ORIENTED_EDGE('',*,*,#23938,.T.);
#34501=ORIENTED_EDGE('',*,*,#25672,.F.);
#34502=ORIENTED_EDGE('',*,*,#25051,.F.);
#34503=ORIENTED_EDGE('',*,*,#25673,.T.);
#34504=ORIENTED_EDGE('',*,*,#23927,.T.);
#34505=ORIENTED_EDGE('',*,*,#25674,.F.);
#34506=ORIENTED_EDGE('',*,*,#25044,.F.);
#34507=ORIENTED_EDGE('',*,*,#25675,.T.);
#34508=ORIENTED_EDGE('',*,*,#23928,.T.);
#34509=ORIENTED_EDGE('',*,*,#25673,.F.);
#34510=ORIENTED_EDGE('',*,*,#25043,.F.);
#34511=ORIENTED_EDGE('',*,*,#25676,.T.);
#34512=ORIENTED_EDGE('',*,*,#23929,.T.);
#34513=ORIENTED_EDGE('',*,*,#25675,.F.);
#34514=ORIENTED_EDGE('',*,*,#25048,.F.);
#34515=ORIENTED_EDGE('',*,*,#25677,.T.);
#34516=ORIENTED_EDGE('',*,*,#23930,.T.);
#34517=ORIENTED_EDGE('',*,*,#25676,.F.);
#34518=ORIENTED_EDGE('',*,*,#25047,.F.);
#34519=ORIENTED_EDGE('',*,*,#25678,.T.);
#34520=ORIENTED_EDGE('',*,*,#23931,.T.);
#34521=ORIENTED_EDGE('',*,*,#25677,.F.);
#34522=ORIENTED_EDGE('',*,*,#25046,.F.);
#34523=ORIENTED_EDGE('',*,*,#25674,.T.);
#34524=ORIENTED_EDGE('',*,*,#23932,.T.);
#34525=ORIENTED_EDGE('',*,*,#25678,.F.);
#34526=ORIENTED_EDGE('',*,*,#25045,.F.);
#34527=ORIENTED_EDGE('',*,*,#25679,.T.);
#34528=ORIENTED_EDGE('',*,*,#23921,.T.);
#34529=ORIENTED_EDGE('',*,*,#25680,.F.);
#34530=ORIENTED_EDGE('',*,*,#25038,.F.);
#34531=ORIENTED_EDGE('',*,*,#25681,.T.);
#34532=ORIENTED_EDGE('',*,*,#23922,.T.);
#34533=ORIENTED_EDGE('',*,*,#25679,.F.);
#34534=ORIENTED_EDGE('',*,*,#25037,.F.);
#34535=ORIENTED_EDGE('',*,*,#25682,.T.);
#34536=ORIENTED_EDGE('',*,*,#23923,.T.);
#34537=ORIENTED_EDGE('',*,*,#25681,.F.);
#34538=ORIENTED_EDGE('',*,*,#25042,.F.);
#34539=ORIENTED_EDGE('',*,*,#25683,.T.);
#34540=ORIENTED_EDGE('',*,*,#23924,.T.);
#34541=ORIENTED_EDGE('',*,*,#25682,.F.);
#34542=ORIENTED_EDGE('',*,*,#25041,.F.);
#34543=ORIENTED_EDGE('',*,*,#25684,.T.);
#34544=ORIENTED_EDGE('',*,*,#23925,.T.);
#34545=ORIENTED_EDGE('',*,*,#25683,.F.);
#34546=ORIENTED_EDGE('',*,*,#25040,.F.);
#34547=ORIENTED_EDGE('',*,*,#25680,.T.);
#34548=ORIENTED_EDGE('',*,*,#23926,.T.);
#34549=ORIENTED_EDGE('',*,*,#25684,.F.);
#34550=ORIENTED_EDGE('',*,*,#25039,.F.);
#34551=ORIENTED_EDGE('',*,*,#25685,.T.);
#34552=ORIENTED_EDGE('',*,*,#23915,.T.);
#34553=ORIENTED_EDGE('',*,*,#25686,.F.);
#34554=ORIENTED_EDGE('',*,*,#25032,.F.);
#34555=ORIENTED_EDGE('',*,*,#25687,.T.);
#34556=ORIENTED_EDGE('',*,*,#23916,.T.);
#34557=ORIENTED_EDGE('',*,*,#25685,.F.);
#34558=ORIENTED_EDGE('',*,*,#25031,.F.);
#34559=ORIENTED_EDGE('',*,*,#25688,.T.);
#34560=ORIENTED_EDGE('',*,*,#23917,.T.);
#34561=ORIENTED_EDGE('',*,*,#25687,.F.);
#34562=ORIENTED_EDGE('',*,*,#25036,.F.);
#34563=ORIENTED_EDGE('',*,*,#25689,.T.);
#34564=ORIENTED_EDGE('',*,*,#23918,.T.);
#34565=ORIENTED_EDGE('',*,*,#25688,.F.);
#34566=ORIENTED_EDGE('',*,*,#25035,.F.);
#34567=ORIENTED_EDGE('',*,*,#25690,.T.);
#34568=ORIENTED_EDGE('',*,*,#23919,.T.);
#34569=ORIENTED_EDGE('',*,*,#25689,.F.);
#34570=ORIENTED_EDGE('',*,*,#25034,.F.);
#34571=ORIENTED_EDGE('',*,*,#25686,.T.);
#34572=ORIENTED_EDGE('',*,*,#23920,.T.);
#34573=ORIENTED_EDGE('',*,*,#25690,.F.);
#34574=ORIENTED_EDGE('',*,*,#25033,.F.);
#34575=ORIENTED_EDGE('',*,*,#25691,.T.);
#34576=ORIENTED_EDGE('',*,*,#23909,.T.);
#34577=ORIENTED_EDGE('',*,*,#25692,.F.);
#34578=ORIENTED_EDGE('',*,*,#25026,.F.);
#34579=ORIENTED_EDGE('',*,*,#25693,.T.);
#34580=ORIENTED_EDGE('',*,*,#23910,.T.);
#34581=ORIENTED_EDGE('',*,*,#25691,.F.);
#34582=ORIENTED_EDGE('',*,*,#25025,.F.);
#34583=ORIENTED_EDGE('',*,*,#25694,.T.);
#34584=ORIENTED_EDGE('',*,*,#23911,.T.);
#34585=ORIENTED_EDGE('',*,*,#25693,.F.);
#34586=ORIENTED_EDGE('',*,*,#25030,.F.);
#34587=ORIENTED_EDGE('',*,*,#25695,.T.);
#34588=ORIENTED_EDGE('',*,*,#23912,.T.);
#34589=ORIENTED_EDGE('',*,*,#25694,.F.);
#34590=ORIENTED_EDGE('',*,*,#25029,.F.);
#34591=ORIENTED_EDGE('',*,*,#25696,.T.);
#34592=ORIENTED_EDGE('',*,*,#23913,.T.);
#34593=ORIENTED_EDGE('',*,*,#25695,.F.);
#34594=ORIENTED_EDGE('',*,*,#25028,.F.);
#34595=ORIENTED_EDGE('',*,*,#25692,.T.);
#34596=ORIENTED_EDGE('',*,*,#23914,.T.);
#34597=ORIENTED_EDGE('',*,*,#25696,.F.);
#34598=ORIENTED_EDGE('',*,*,#25027,.F.);
#34599=ORIENTED_EDGE('',*,*,#25697,.T.);
#34600=ORIENTED_EDGE('',*,*,#23903,.T.);
#34601=ORIENTED_EDGE('',*,*,#25698,.F.);
#34602=ORIENTED_EDGE('',*,*,#25020,.F.);
#34603=ORIENTED_EDGE('',*,*,#25699,.T.);
#34604=ORIENTED_EDGE('',*,*,#23904,.T.);
#34605=ORIENTED_EDGE('',*,*,#25697,.F.);
#34606=ORIENTED_EDGE('',*,*,#25019,.F.);
#34607=ORIENTED_EDGE('',*,*,#25700,.T.);
#34608=ORIENTED_EDGE('',*,*,#23905,.T.);
#34609=ORIENTED_EDGE('',*,*,#25699,.F.);
#34610=ORIENTED_EDGE('',*,*,#25024,.F.);
#34611=ORIENTED_EDGE('',*,*,#25701,.T.);
#34612=ORIENTED_EDGE('',*,*,#23906,.T.);
#34613=ORIENTED_EDGE('',*,*,#25700,.F.);
#34614=ORIENTED_EDGE('',*,*,#25023,.F.);
#34615=ORIENTED_EDGE('',*,*,#25702,.T.);
#34616=ORIENTED_EDGE('',*,*,#23907,.T.);
#34617=ORIENTED_EDGE('',*,*,#25701,.F.);
#34618=ORIENTED_EDGE('',*,*,#25022,.F.);
#34619=ORIENTED_EDGE('',*,*,#25698,.T.);
#34620=ORIENTED_EDGE('',*,*,#23908,.T.);
#34621=ORIENTED_EDGE('',*,*,#25702,.F.);
#34622=ORIENTED_EDGE('',*,*,#25021,.F.);
#34623=ORIENTED_EDGE('',*,*,#25703,.T.);
#34624=ORIENTED_EDGE('',*,*,#23897,.T.);
#34625=ORIENTED_EDGE('',*,*,#25704,.F.);
#34626=ORIENTED_EDGE('',*,*,#25014,.F.);
#34627=ORIENTED_EDGE('',*,*,#25705,.T.);
#34628=ORIENTED_EDGE('',*,*,#23898,.T.);
#34629=ORIENTED_EDGE('',*,*,#25703,.F.);
#34630=ORIENTED_EDGE('',*,*,#25013,.F.);
#34631=ORIENTED_EDGE('',*,*,#25706,.T.);
#34632=ORIENTED_EDGE('',*,*,#23899,.T.);
#34633=ORIENTED_EDGE('',*,*,#25705,.F.);
#34634=ORIENTED_EDGE('',*,*,#25018,.F.);
#34635=ORIENTED_EDGE('',*,*,#25707,.T.);
#34636=ORIENTED_EDGE('',*,*,#23900,.T.);
#34637=ORIENTED_EDGE('',*,*,#25706,.F.);
#34638=ORIENTED_EDGE('',*,*,#25017,.F.);
#34639=ORIENTED_EDGE('',*,*,#25708,.T.);
#34640=ORIENTED_EDGE('',*,*,#23901,.T.);
#34641=ORIENTED_EDGE('',*,*,#25707,.F.);
#34642=ORIENTED_EDGE('',*,*,#25016,.F.);
#34643=ORIENTED_EDGE('',*,*,#25704,.T.);
#34644=ORIENTED_EDGE('',*,*,#23902,.T.);
#34645=ORIENTED_EDGE('',*,*,#25708,.F.);
#34646=ORIENTED_EDGE('',*,*,#25015,.F.);
#34647=ORIENTED_EDGE('',*,*,#25709,.T.);
#34648=ORIENTED_EDGE('',*,*,#23891,.T.);
#34649=ORIENTED_EDGE('',*,*,#25710,.F.);
#34650=ORIENTED_EDGE('',*,*,#25008,.F.);
#34651=ORIENTED_EDGE('',*,*,#25711,.T.);
#34652=ORIENTED_EDGE('',*,*,#23892,.T.);
#34653=ORIENTED_EDGE('',*,*,#25709,.F.);
#34654=ORIENTED_EDGE('',*,*,#25007,.F.);
#34655=ORIENTED_EDGE('',*,*,#25712,.T.);
#34656=ORIENTED_EDGE('',*,*,#23893,.T.);
#34657=ORIENTED_EDGE('',*,*,#25711,.F.);
#34658=ORIENTED_EDGE('',*,*,#25012,.F.);
#34659=ORIENTED_EDGE('',*,*,#25713,.T.);
#34660=ORIENTED_EDGE('',*,*,#23894,.T.);
#34661=ORIENTED_EDGE('',*,*,#25712,.F.);
#34662=ORIENTED_EDGE('',*,*,#25011,.F.);
#34663=ORIENTED_EDGE('',*,*,#25714,.T.);
#34664=ORIENTED_EDGE('',*,*,#23895,.T.);
#34665=ORIENTED_EDGE('',*,*,#25713,.F.);
#34666=ORIENTED_EDGE('',*,*,#25010,.F.);
#34667=ORIENTED_EDGE('',*,*,#25710,.T.);
#34668=ORIENTED_EDGE('',*,*,#23896,.T.);
#34669=ORIENTED_EDGE('',*,*,#25714,.F.);
#34670=ORIENTED_EDGE('',*,*,#25009,.F.);
#34671=ORIENTED_EDGE('',*,*,#25715,.T.);
#34672=ORIENTED_EDGE('',*,*,#23885,.T.);
#34673=ORIENTED_EDGE('',*,*,#25716,.F.);
#34674=ORIENTED_EDGE('',*,*,#25002,.F.);
#34675=ORIENTED_EDGE('',*,*,#25717,.T.);
#34676=ORIENTED_EDGE('',*,*,#23886,.T.);
#34677=ORIENTED_EDGE('',*,*,#25715,.F.);
#34678=ORIENTED_EDGE('',*,*,#25001,.F.);
#34679=ORIENTED_EDGE('',*,*,#25718,.T.);
#34680=ORIENTED_EDGE('',*,*,#23887,.T.);
#34681=ORIENTED_EDGE('',*,*,#25717,.F.);
#34682=ORIENTED_EDGE('',*,*,#25006,.F.);
#34683=ORIENTED_EDGE('',*,*,#25719,.T.);
#34684=ORIENTED_EDGE('',*,*,#23888,.T.);
#34685=ORIENTED_EDGE('',*,*,#25718,.F.);
#34686=ORIENTED_EDGE('',*,*,#25005,.F.);
#34687=ORIENTED_EDGE('',*,*,#25720,.T.);
#34688=ORIENTED_EDGE('',*,*,#23889,.T.);
#34689=ORIENTED_EDGE('',*,*,#25719,.F.);
#34690=ORIENTED_EDGE('',*,*,#25004,.F.);
#34691=ORIENTED_EDGE('',*,*,#25716,.T.);
#34692=ORIENTED_EDGE('',*,*,#23890,.T.);
#34693=ORIENTED_EDGE('',*,*,#25720,.F.);
#34694=ORIENTED_EDGE('',*,*,#25003,.F.);
#34695=ORIENTED_EDGE('',*,*,#25721,.T.);
#34696=ORIENTED_EDGE('',*,*,#23879,.T.);
#34697=ORIENTED_EDGE('',*,*,#25722,.F.);
#34698=ORIENTED_EDGE('',*,*,#24996,.F.);
#34699=ORIENTED_EDGE('',*,*,#25723,.T.);
#34700=ORIENTED_EDGE('',*,*,#23880,.T.);
#34701=ORIENTED_EDGE('',*,*,#25721,.F.);
#34702=ORIENTED_EDGE('',*,*,#24995,.F.);
#34703=ORIENTED_EDGE('',*,*,#25724,.T.);
#34704=ORIENTED_EDGE('',*,*,#23881,.T.);
#34705=ORIENTED_EDGE('',*,*,#25723,.F.);
#34706=ORIENTED_EDGE('',*,*,#25000,.F.);
#34707=ORIENTED_EDGE('',*,*,#25725,.T.);
#34708=ORIENTED_EDGE('',*,*,#23882,.T.);
#34709=ORIENTED_EDGE('',*,*,#25724,.F.);
#34710=ORIENTED_EDGE('',*,*,#24999,.F.);
#34711=ORIENTED_EDGE('',*,*,#25726,.T.);
#34712=ORIENTED_EDGE('',*,*,#23883,.T.);
#34713=ORIENTED_EDGE('',*,*,#25725,.F.);
#34714=ORIENTED_EDGE('',*,*,#24998,.F.);
#34715=ORIENTED_EDGE('',*,*,#25722,.T.);
#34716=ORIENTED_EDGE('',*,*,#23884,.T.);
#34717=ORIENTED_EDGE('',*,*,#25726,.F.);
#34718=ORIENTED_EDGE('',*,*,#24997,.F.);
#34719=ORIENTED_EDGE('',*,*,#25727,.T.);
#34720=ORIENTED_EDGE('',*,*,#23873,.T.);
#34721=ORIENTED_EDGE('',*,*,#25728,.F.);
#34722=ORIENTED_EDGE('',*,*,#24990,.F.);
#34723=ORIENTED_EDGE('',*,*,#25729,.T.);
#34724=ORIENTED_EDGE('',*,*,#23874,.T.);
#34725=ORIENTED_EDGE('',*,*,#25727,.F.);
#34726=ORIENTED_EDGE('',*,*,#24989,.F.);
#34727=ORIENTED_EDGE('',*,*,#25730,.T.);
#34728=ORIENTED_EDGE('',*,*,#23875,.T.);
#34729=ORIENTED_EDGE('',*,*,#25729,.F.);
#34730=ORIENTED_EDGE('',*,*,#24994,.F.);
#34731=ORIENTED_EDGE('',*,*,#25731,.T.);
#34732=ORIENTED_EDGE('',*,*,#23876,.T.);
#34733=ORIENTED_EDGE('',*,*,#25730,.F.);
#34734=ORIENTED_EDGE('',*,*,#24993,.F.);
#34735=ORIENTED_EDGE('',*,*,#25732,.T.);
#34736=ORIENTED_EDGE('',*,*,#23877,.T.);
#34737=ORIENTED_EDGE('',*,*,#25731,.F.);
#34738=ORIENTED_EDGE('',*,*,#24992,.F.);
#34739=ORIENTED_EDGE('',*,*,#25728,.T.);
#34740=ORIENTED_EDGE('',*,*,#23878,.T.);
#34741=ORIENTED_EDGE('',*,*,#25732,.F.);
#34742=ORIENTED_EDGE('',*,*,#24991,.F.);
#34743=ORIENTED_EDGE('',*,*,#25733,.T.);
#34744=ORIENTED_EDGE('',*,*,#23867,.T.);
#34745=ORIENTED_EDGE('',*,*,#25734,.F.);
#34746=ORIENTED_EDGE('',*,*,#24984,.F.);
#34747=ORIENTED_EDGE('',*,*,#25735,.T.);
#34748=ORIENTED_EDGE('',*,*,#23868,.T.);
#34749=ORIENTED_EDGE('',*,*,#25733,.F.);
#34750=ORIENTED_EDGE('',*,*,#24983,.F.);
#34751=ORIENTED_EDGE('',*,*,#25736,.T.);
#34752=ORIENTED_EDGE('',*,*,#23869,.T.);
#34753=ORIENTED_EDGE('',*,*,#25735,.F.);
#34754=ORIENTED_EDGE('',*,*,#24988,.F.);
#34755=ORIENTED_EDGE('',*,*,#25737,.T.);
#34756=ORIENTED_EDGE('',*,*,#23870,.T.);
#34757=ORIENTED_EDGE('',*,*,#25736,.F.);
#34758=ORIENTED_EDGE('',*,*,#24987,.F.);
#34759=ORIENTED_EDGE('',*,*,#25738,.T.);
#34760=ORIENTED_EDGE('',*,*,#23871,.T.);
#34761=ORIENTED_EDGE('',*,*,#25737,.F.);
#34762=ORIENTED_EDGE('',*,*,#24986,.F.);
#34763=ORIENTED_EDGE('',*,*,#25734,.T.);
#34764=ORIENTED_EDGE('',*,*,#23872,.T.);
#34765=ORIENTED_EDGE('',*,*,#25738,.F.);
#34766=ORIENTED_EDGE('',*,*,#24985,.F.);
#34767=ORIENTED_EDGE('',*,*,#25739,.T.);
#34768=ORIENTED_EDGE('',*,*,#23861,.T.);
#34769=ORIENTED_EDGE('',*,*,#25740,.F.);
#34770=ORIENTED_EDGE('',*,*,#24978,.F.);
#34771=ORIENTED_EDGE('',*,*,#25741,.T.);
#34772=ORIENTED_EDGE('',*,*,#23862,.T.);
#34773=ORIENTED_EDGE('',*,*,#25739,.F.);
#34774=ORIENTED_EDGE('',*,*,#24977,.F.);
#34775=ORIENTED_EDGE('',*,*,#25742,.T.);
#34776=ORIENTED_EDGE('',*,*,#23863,.T.);
#34777=ORIENTED_EDGE('',*,*,#25741,.F.);
#34778=ORIENTED_EDGE('',*,*,#24982,.F.);
#34779=ORIENTED_EDGE('',*,*,#25743,.T.);
#34780=ORIENTED_EDGE('',*,*,#23864,.T.);
#34781=ORIENTED_EDGE('',*,*,#25742,.F.);
#34782=ORIENTED_EDGE('',*,*,#24981,.F.);
#34783=ORIENTED_EDGE('',*,*,#25744,.T.);
#34784=ORIENTED_EDGE('',*,*,#23865,.T.);
#34785=ORIENTED_EDGE('',*,*,#25743,.F.);
#34786=ORIENTED_EDGE('',*,*,#24980,.F.);
#34787=ORIENTED_EDGE('',*,*,#25740,.T.);
#34788=ORIENTED_EDGE('',*,*,#23866,.T.);
#34789=ORIENTED_EDGE('',*,*,#25744,.F.);
#34790=ORIENTED_EDGE('',*,*,#24979,.F.);
#34791=ORIENTED_EDGE('',*,*,#25745,.T.);
#34792=ORIENTED_EDGE('',*,*,#23855,.T.);
#34793=ORIENTED_EDGE('',*,*,#25746,.F.);
#34794=ORIENTED_EDGE('',*,*,#24972,.F.);
#34795=ORIENTED_EDGE('',*,*,#25747,.T.);
#34796=ORIENTED_EDGE('',*,*,#23856,.T.);
#34797=ORIENTED_EDGE('',*,*,#25745,.F.);
#34798=ORIENTED_EDGE('',*,*,#24971,.F.);
#34799=ORIENTED_EDGE('',*,*,#25748,.T.);
#34800=ORIENTED_EDGE('',*,*,#23857,.T.);
#34801=ORIENTED_EDGE('',*,*,#25747,.F.);
#34802=ORIENTED_EDGE('',*,*,#24976,.F.);
#34803=ORIENTED_EDGE('',*,*,#25749,.T.);
#34804=ORIENTED_EDGE('',*,*,#23858,.T.);
#34805=ORIENTED_EDGE('',*,*,#25748,.F.);
#34806=ORIENTED_EDGE('',*,*,#24975,.F.);
#34807=ORIENTED_EDGE('',*,*,#25750,.T.);
#34808=ORIENTED_EDGE('',*,*,#23859,.T.);
#34809=ORIENTED_EDGE('',*,*,#25749,.F.);
#34810=ORIENTED_EDGE('',*,*,#24974,.F.);
#34811=ORIENTED_EDGE('',*,*,#25746,.T.);
#34812=ORIENTED_EDGE('',*,*,#23860,.T.);
#34813=ORIENTED_EDGE('',*,*,#25750,.F.);
#34814=ORIENTED_EDGE('',*,*,#24973,.F.);
#34815=ORIENTED_EDGE('',*,*,#25751,.T.);
#34816=ORIENTED_EDGE('',*,*,#23849,.T.);
#34817=ORIENTED_EDGE('',*,*,#25752,.F.);
#34818=ORIENTED_EDGE('',*,*,#24966,.F.);
#34819=ORIENTED_EDGE('',*,*,#25753,.T.);
#34820=ORIENTED_EDGE('',*,*,#23850,.T.);
#34821=ORIENTED_EDGE('',*,*,#25751,.F.);
#34822=ORIENTED_EDGE('',*,*,#24965,.F.);
#34823=ORIENTED_EDGE('',*,*,#25754,.T.);
#34824=ORIENTED_EDGE('',*,*,#23851,.T.);
#34825=ORIENTED_EDGE('',*,*,#25753,.F.);
#34826=ORIENTED_EDGE('',*,*,#24970,.F.);
#34827=ORIENTED_EDGE('',*,*,#25755,.T.);
#34828=ORIENTED_EDGE('',*,*,#23852,.T.);
#34829=ORIENTED_EDGE('',*,*,#25754,.F.);
#34830=ORIENTED_EDGE('',*,*,#24969,.F.);
#34831=ORIENTED_EDGE('',*,*,#25756,.T.);
#34832=ORIENTED_EDGE('',*,*,#23853,.T.);
#34833=ORIENTED_EDGE('',*,*,#25755,.F.);
#34834=ORIENTED_EDGE('',*,*,#24968,.F.);
#34835=ORIENTED_EDGE('',*,*,#25752,.T.);
#34836=ORIENTED_EDGE('',*,*,#23854,.T.);
#34837=ORIENTED_EDGE('',*,*,#25756,.F.);
#34838=ORIENTED_EDGE('',*,*,#24967,.F.);
#34839=ORIENTED_EDGE('',*,*,#25757,.T.);
#34840=ORIENTED_EDGE('',*,*,#23843,.T.);
#34841=ORIENTED_EDGE('',*,*,#25758,.F.);
#34842=ORIENTED_EDGE('',*,*,#24960,.F.);
#34843=ORIENTED_EDGE('',*,*,#25759,.T.);
#34844=ORIENTED_EDGE('',*,*,#23844,.T.);
#34845=ORIENTED_EDGE('',*,*,#25757,.F.);
#34846=ORIENTED_EDGE('',*,*,#24959,.F.);
#34847=ORIENTED_EDGE('',*,*,#25760,.T.);
#34848=ORIENTED_EDGE('',*,*,#23845,.T.);
#34849=ORIENTED_EDGE('',*,*,#25759,.F.);
#34850=ORIENTED_EDGE('',*,*,#24964,.F.);
#34851=ORIENTED_EDGE('',*,*,#25761,.T.);
#34852=ORIENTED_EDGE('',*,*,#23846,.T.);
#34853=ORIENTED_EDGE('',*,*,#25760,.F.);
#34854=ORIENTED_EDGE('',*,*,#24963,.F.);
#34855=ORIENTED_EDGE('',*,*,#25762,.T.);
#34856=ORIENTED_EDGE('',*,*,#23847,.T.);
#34857=ORIENTED_EDGE('',*,*,#25761,.F.);
#34858=ORIENTED_EDGE('',*,*,#24962,.F.);
#34859=ORIENTED_EDGE('',*,*,#25758,.T.);
#34860=ORIENTED_EDGE('',*,*,#23848,.T.);
#34861=ORIENTED_EDGE('',*,*,#25762,.F.);
#34862=ORIENTED_EDGE('',*,*,#24961,.F.);
#34863=ORIENTED_EDGE('',*,*,#25763,.T.);
#34864=ORIENTED_EDGE('',*,*,#23837,.T.);
#34865=ORIENTED_EDGE('',*,*,#25764,.F.);
#34866=ORIENTED_EDGE('',*,*,#24954,.F.);
#34867=ORIENTED_EDGE('',*,*,#25765,.T.);
#34868=ORIENTED_EDGE('',*,*,#23838,.T.);
#34869=ORIENTED_EDGE('',*,*,#25763,.F.);
#34870=ORIENTED_EDGE('',*,*,#24953,.F.);
#34871=ORIENTED_EDGE('',*,*,#25766,.T.);
#34872=ORIENTED_EDGE('',*,*,#23839,.T.);
#34873=ORIENTED_EDGE('',*,*,#25765,.F.);
#34874=ORIENTED_EDGE('',*,*,#24958,.F.);
#34875=ORIENTED_EDGE('',*,*,#25767,.T.);
#34876=ORIENTED_EDGE('',*,*,#23840,.T.);
#34877=ORIENTED_EDGE('',*,*,#25766,.F.);
#34878=ORIENTED_EDGE('',*,*,#24957,.F.);
#34879=ORIENTED_EDGE('',*,*,#25768,.T.);
#34880=ORIENTED_EDGE('',*,*,#23841,.T.);
#34881=ORIENTED_EDGE('',*,*,#25767,.F.);
#34882=ORIENTED_EDGE('',*,*,#24956,.F.);
#34883=ORIENTED_EDGE('',*,*,#25764,.T.);
#34884=ORIENTED_EDGE('',*,*,#23842,.T.);
#34885=ORIENTED_EDGE('',*,*,#25768,.F.);
#34886=ORIENTED_EDGE('',*,*,#24955,.F.);
#34887=ORIENTED_EDGE('',*,*,#25769,.T.);
#34888=ORIENTED_EDGE('',*,*,#23831,.T.);
#34889=ORIENTED_EDGE('',*,*,#25770,.F.);
#34890=ORIENTED_EDGE('',*,*,#24948,.F.);
#34891=ORIENTED_EDGE('',*,*,#25771,.T.);
#34892=ORIENTED_EDGE('',*,*,#23832,.T.);
#34893=ORIENTED_EDGE('',*,*,#25769,.F.);
#34894=ORIENTED_EDGE('',*,*,#24947,.F.);
#34895=ORIENTED_EDGE('',*,*,#25772,.T.);
#34896=ORIENTED_EDGE('',*,*,#23833,.T.);
#34897=ORIENTED_EDGE('',*,*,#25771,.F.);
#34898=ORIENTED_EDGE('',*,*,#24952,.F.);
#34899=ORIENTED_EDGE('',*,*,#25773,.T.);
#34900=ORIENTED_EDGE('',*,*,#23834,.T.);
#34901=ORIENTED_EDGE('',*,*,#25772,.F.);
#34902=ORIENTED_EDGE('',*,*,#24951,.F.);
#34903=ORIENTED_EDGE('',*,*,#25774,.T.);
#34904=ORIENTED_EDGE('',*,*,#23835,.T.);
#34905=ORIENTED_EDGE('',*,*,#25773,.F.);
#34906=ORIENTED_EDGE('',*,*,#24950,.F.);
#34907=ORIENTED_EDGE('',*,*,#25770,.T.);
#34908=ORIENTED_EDGE('',*,*,#23836,.T.);
#34909=ORIENTED_EDGE('',*,*,#25774,.F.);
#34910=ORIENTED_EDGE('',*,*,#24949,.F.);
#34911=ORIENTED_EDGE('',*,*,#25775,.T.);
#34912=ORIENTED_EDGE('',*,*,#23825,.T.);
#34913=ORIENTED_EDGE('',*,*,#25776,.F.);
#34914=ORIENTED_EDGE('',*,*,#24942,.F.);
#34915=ORIENTED_EDGE('',*,*,#25777,.T.);
#34916=ORIENTED_EDGE('',*,*,#23826,.T.);
#34917=ORIENTED_EDGE('',*,*,#25775,.F.);
#34918=ORIENTED_EDGE('',*,*,#24941,.F.);
#34919=ORIENTED_EDGE('',*,*,#25778,.T.);
#34920=ORIENTED_EDGE('',*,*,#23827,.T.);
#34921=ORIENTED_EDGE('',*,*,#25777,.F.);
#34922=ORIENTED_EDGE('',*,*,#24946,.F.);
#34923=ORIENTED_EDGE('',*,*,#25779,.T.);
#34924=ORIENTED_EDGE('',*,*,#23828,.T.);
#34925=ORIENTED_EDGE('',*,*,#25778,.F.);
#34926=ORIENTED_EDGE('',*,*,#24945,.F.);
#34927=ORIENTED_EDGE('',*,*,#25780,.T.);
#34928=ORIENTED_EDGE('',*,*,#23829,.T.);
#34929=ORIENTED_EDGE('',*,*,#25779,.F.);
#34930=ORIENTED_EDGE('',*,*,#24944,.F.);
#34931=ORIENTED_EDGE('',*,*,#25776,.T.);
#34932=ORIENTED_EDGE('',*,*,#23830,.T.);
#34933=ORIENTED_EDGE('',*,*,#25780,.F.);
#34934=ORIENTED_EDGE('',*,*,#24943,.F.);
#34935=ORIENTED_EDGE('',*,*,#25781,.T.);
#34936=ORIENTED_EDGE('',*,*,#23819,.T.);
#34937=ORIENTED_EDGE('',*,*,#25782,.F.);
#34938=ORIENTED_EDGE('',*,*,#24936,.F.);
#34939=ORIENTED_EDGE('',*,*,#25783,.T.);
#34940=ORIENTED_EDGE('',*,*,#23820,.T.);
#34941=ORIENTED_EDGE('',*,*,#25781,.F.);
#34942=ORIENTED_EDGE('',*,*,#24935,.F.);
#34943=ORIENTED_EDGE('',*,*,#25784,.T.);
#34944=ORIENTED_EDGE('',*,*,#23821,.T.);
#34945=ORIENTED_EDGE('',*,*,#25783,.F.);
#34946=ORIENTED_EDGE('',*,*,#24940,.F.);
#34947=ORIENTED_EDGE('',*,*,#25785,.T.);
#34948=ORIENTED_EDGE('',*,*,#23822,.T.);
#34949=ORIENTED_EDGE('',*,*,#25784,.F.);
#34950=ORIENTED_EDGE('',*,*,#24939,.F.);
#34951=ORIENTED_EDGE('',*,*,#25786,.T.);
#34952=ORIENTED_EDGE('',*,*,#23823,.T.);
#34953=ORIENTED_EDGE('',*,*,#25785,.F.);
#34954=ORIENTED_EDGE('',*,*,#24938,.F.);
#34955=ORIENTED_EDGE('',*,*,#25782,.T.);
#34956=ORIENTED_EDGE('',*,*,#23824,.T.);
#34957=ORIENTED_EDGE('',*,*,#25786,.F.);
#34958=ORIENTED_EDGE('',*,*,#24937,.F.);
#34959=ORIENTED_EDGE('',*,*,#25787,.T.);
#34960=ORIENTED_EDGE('',*,*,#23813,.T.);
#34961=ORIENTED_EDGE('',*,*,#25788,.F.);
#34962=ORIENTED_EDGE('',*,*,#24930,.F.);
#34963=ORIENTED_EDGE('',*,*,#25789,.T.);
#34964=ORIENTED_EDGE('',*,*,#23814,.T.);
#34965=ORIENTED_EDGE('',*,*,#25787,.F.);
#34966=ORIENTED_EDGE('',*,*,#24929,.F.);
#34967=ORIENTED_EDGE('',*,*,#25790,.T.);
#34968=ORIENTED_EDGE('',*,*,#23815,.T.);
#34969=ORIENTED_EDGE('',*,*,#25789,.F.);
#34970=ORIENTED_EDGE('',*,*,#24934,.F.);
#34971=ORIENTED_EDGE('',*,*,#25791,.T.);
#34972=ORIENTED_EDGE('',*,*,#23816,.T.);
#34973=ORIENTED_EDGE('',*,*,#25790,.F.);
#34974=ORIENTED_EDGE('',*,*,#24933,.F.);
#34975=ORIENTED_EDGE('',*,*,#25792,.T.);
#34976=ORIENTED_EDGE('',*,*,#23817,.T.);
#34977=ORIENTED_EDGE('',*,*,#25791,.F.);
#34978=ORIENTED_EDGE('',*,*,#24932,.F.);
#34979=ORIENTED_EDGE('',*,*,#25788,.T.);
#34980=ORIENTED_EDGE('',*,*,#23818,.T.);
#34981=ORIENTED_EDGE('',*,*,#25792,.F.);
#34982=ORIENTED_EDGE('',*,*,#24931,.F.);
#34983=ORIENTED_EDGE('',*,*,#25793,.T.);
#34984=ORIENTED_EDGE('',*,*,#23807,.T.);
#34985=ORIENTED_EDGE('',*,*,#25794,.F.);
#34986=ORIENTED_EDGE('',*,*,#24924,.F.);
#34987=ORIENTED_EDGE('',*,*,#25795,.T.);
#34988=ORIENTED_EDGE('',*,*,#23808,.T.);
#34989=ORIENTED_EDGE('',*,*,#25793,.F.);
#34990=ORIENTED_EDGE('',*,*,#24923,.F.);
#34991=ORIENTED_EDGE('',*,*,#25796,.T.);
#34992=ORIENTED_EDGE('',*,*,#23809,.T.);
#34993=ORIENTED_EDGE('',*,*,#25795,.F.);
#34994=ORIENTED_EDGE('',*,*,#24928,.F.);
#34995=ORIENTED_EDGE('',*,*,#25797,.T.);
#34996=ORIENTED_EDGE('',*,*,#23810,.T.);
#34997=ORIENTED_EDGE('',*,*,#25796,.F.);
#34998=ORIENTED_EDGE('',*,*,#24927,.F.);
#34999=ORIENTED_EDGE('',*,*,#25798,.T.);
#35000=ORIENTED_EDGE('',*,*,#23811,.T.);
#35001=ORIENTED_EDGE('',*,*,#25797,.F.);
#35002=ORIENTED_EDGE('',*,*,#24926,.F.);
#35003=ORIENTED_EDGE('',*,*,#25794,.T.);
#35004=ORIENTED_EDGE('',*,*,#23812,.T.);
#35005=ORIENTED_EDGE('',*,*,#25798,.F.);
#35006=ORIENTED_EDGE('',*,*,#24925,.F.);
#35007=ORIENTED_EDGE('',*,*,#25799,.T.);
#35008=ORIENTED_EDGE('',*,*,#23801,.T.);
#35009=ORIENTED_EDGE('',*,*,#25800,.F.);
#35010=ORIENTED_EDGE('',*,*,#24918,.F.);
#35011=ORIENTED_EDGE('',*,*,#25801,.T.);
#35012=ORIENTED_EDGE('',*,*,#23802,.T.);
#35013=ORIENTED_EDGE('',*,*,#25799,.F.);
#35014=ORIENTED_EDGE('',*,*,#24917,.F.);
#35015=ORIENTED_EDGE('',*,*,#25802,.T.);
#35016=ORIENTED_EDGE('',*,*,#23803,.T.);
#35017=ORIENTED_EDGE('',*,*,#25801,.F.);
#35018=ORIENTED_EDGE('',*,*,#24922,.F.);
#35019=ORIENTED_EDGE('',*,*,#25803,.T.);
#35020=ORIENTED_EDGE('',*,*,#23804,.T.);
#35021=ORIENTED_EDGE('',*,*,#25802,.F.);
#35022=ORIENTED_EDGE('',*,*,#24921,.F.);
#35023=ORIENTED_EDGE('',*,*,#25804,.T.);
#35024=ORIENTED_EDGE('',*,*,#23805,.T.);
#35025=ORIENTED_EDGE('',*,*,#25803,.F.);
#35026=ORIENTED_EDGE('',*,*,#24920,.F.);
#35027=ORIENTED_EDGE('',*,*,#25800,.T.);
#35028=ORIENTED_EDGE('',*,*,#23806,.T.);
#35029=ORIENTED_EDGE('',*,*,#25804,.F.);
#35030=ORIENTED_EDGE('',*,*,#24919,.F.);
#35031=ORIENTED_EDGE('',*,*,#25805,.T.);
#35032=ORIENTED_EDGE('',*,*,#23795,.T.);
#35033=ORIENTED_EDGE('',*,*,#25806,.F.);
#35034=ORIENTED_EDGE('',*,*,#24912,.F.);
#35035=ORIENTED_EDGE('',*,*,#25807,.T.);
#35036=ORIENTED_EDGE('',*,*,#23796,.T.);
#35037=ORIENTED_EDGE('',*,*,#25805,.F.);
#35038=ORIENTED_EDGE('',*,*,#24911,.F.);
#35039=ORIENTED_EDGE('',*,*,#25808,.T.);
#35040=ORIENTED_EDGE('',*,*,#23797,.T.);
#35041=ORIENTED_EDGE('',*,*,#25807,.F.);
#35042=ORIENTED_EDGE('',*,*,#24916,.F.);
#35043=ORIENTED_EDGE('',*,*,#25809,.T.);
#35044=ORIENTED_EDGE('',*,*,#23798,.T.);
#35045=ORIENTED_EDGE('',*,*,#25808,.F.);
#35046=ORIENTED_EDGE('',*,*,#24915,.F.);
#35047=ORIENTED_EDGE('',*,*,#25810,.T.);
#35048=ORIENTED_EDGE('',*,*,#23799,.T.);
#35049=ORIENTED_EDGE('',*,*,#25809,.F.);
#35050=ORIENTED_EDGE('',*,*,#24914,.F.);
#35051=ORIENTED_EDGE('',*,*,#25806,.T.);
#35052=ORIENTED_EDGE('',*,*,#23800,.T.);
#35053=ORIENTED_EDGE('',*,*,#25810,.F.);
#35054=ORIENTED_EDGE('',*,*,#24913,.F.);
#35055=ORIENTED_EDGE('',*,*,#25811,.T.);
#35056=ORIENTED_EDGE('',*,*,#23789,.T.);
#35057=ORIENTED_EDGE('',*,*,#25812,.F.);
#35058=ORIENTED_EDGE('',*,*,#24906,.F.);
#35059=ORIENTED_EDGE('',*,*,#25813,.T.);
#35060=ORIENTED_EDGE('',*,*,#23790,.T.);
#35061=ORIENTED_EDGE('',*,*,#25811,.F.);
#35062=ORIENTED_EDGE('',*,*,#24905,.F.);
#35063=ORIENTED_EDGE('',*,*,#25814,.T.);
#35064=ORIENTED_EDGE('',*,*,#23791,.T.);
#35065=ORIENTED_EDGE('',*,*,#25813,.F.);
#35066=ORIENTED_EDGE('',*,*,#24910,.F.);
#35067=ORIENTED_EDGE('',*,*,#25815,.T.);
#35068=ORIENTED_EDGE('',*,*,#23792,.T.);
#35069=ORIENTED_EDGE('',*,*,#25814,.F.);
#35070=ORIENTED_EDGE('',*,*,#24909,.F.);
#35071=ORIENTED_EDGE('',*,*,#25816,.T.);
#35072=ORIENTED_EDGE('',*,*,#23793,.T.);
#35073=ORIENTED_EDGE('',*,*,#25815,.F.);
#35074=ORIENTED_EDGE('',*,*,#24908,.F.);
#35075=ORIENTED_EDGE('',*,*,#25812,.T.);
#35076=ORIENTED_EDGE('',*,*,#23794,.T.);
#35077=ORIENTED_EDGE('',*,*,#25816,.F.);
#35078=ORIENTED_EDGE('',*,*,#24907,.F.);
#35079=ORIENTED_EDGE('',*,*,#25817,.T.);
#35080=ORIENTED_EDGE('',*,*,#23783,.T.);
#35081=ORIENTED_EDGE('',*,*,#25818,.F.);
#35082=ORIENTED_EDGE('',*,*,#24900,.F.);
#35083=ORIENTED_EDGE('',*,*,#25819,.T.);
#35084=ORIENTED_EDGE('',*,*,#23784,.T.);
#35085=ORIENTED_EDGE('',*,*,#25817,.F.);
#35086=ORIENTED_EDGE('',*,*,#24899,.F.);
#35087=ORIENTED_EDGE('',*,*,#25820,.T.);
#35088=ORIENTED_EDGE('',*,*,#23785,.T.);
#35089=ORIENTED_EDGE('',*,*,#25819,.F.);
#35090=ORIENTED_EDGE('',*,*,#24904,.F.);
#35091=ORIENTED_EDGE('',*,*,#25821,.T.);
#35092=ORIENTED_EDGE('',*,*,#23786,.T.);
#35093=ORIENTED_EDGE('',*,*,#25820,.F.);
#35094=ORIENTED_EDGE('',*,*,#24903,.F.);
#35095=ORIENTED_EDGE('',*,*,#25822,.T.);
#35096=ORIENTED_EDGE('',*,*,#23787,.T.);
#35097=ORIENTED_EDGE('',*,*,#25821,.F.);
#35098=ORIENTED_EDGE('',*,*,#24902,.F.);
#35099=ORIENTED_EDGE('',*,*,#25818,.T.);
#35100=ORIENTED_EDGE('',*,*,#23788,.T.);
#35101=ORIENTED_EDGE('',*,*,#25822,.F.);
#35102=ORIENTED_EDGE('',*,*,#24901,.F.);
#35103=ORIENTED_EDGE('',*,*,#25823,.T.);
#35104=ORIENTED_EDGE('',*,*,#23777,.T.);
#35105=ORIENTED_EDGE('',*,*,#25824,.F.);
#35106=ORIENTED_EDGE('',*,*,#24894,.F.);
#35107=ORIENTED_EDGE('',*,*,#25825,.T.);
#35108=ORIENTED_EDGE('',*,*,#23778,.T.);
#35109=ORIENTED_EDGE('',*,*,#25823,.F.);
#35110=ORIENTED_EDGE('',*,*,#24893,.F.);
#35111=ORIENTED_EDGE('',*,*,#25826,.T.);
#35112=ORIENTED_EDGE('',*,*,#23779,.T.);
#35113=ORIENTED_EDGE('',*,*,#25825,.F.);
#35114=ORIENTED_EDGE('',*,*,#24898,.F.);
#35115=ORIENTED_EDGE('',*,*,#25827,.T.);
#35116=ORIENTED_EDGE('',*,*,#23780,.T.);
#35117=ORIENTED_EDGE('',*,*,#25826,.F.);
#35118=ORIENTED_EDGE('',*,*,#24897,.F.);
#35119=ORIENTED_EDGE('',*,*,#25828,.T.);
#35120=ORIENTED_EDGE('',*,*,#23781,.T.);
#35121=ORIENTED_EDGE('',*,*,#25827,.F.);
#35122=ORIENTED_EDGE('',*,*,#24896,.F.);
#35123=ORIENTED_EDGE('',*,*,#25824,.T.);
#35124=ORIENTED_EDGE('',*,*,#23782,.T.);
#35125=ORIENTED_EDGE('',*,*,#25828,.F.);
#35126=ORIENTED_EDGE('',*,*,#24895,.F.);
#35127=ORIENTED_EDGE('',*,*,#25829,.T.);
#35128=ORIENTED_EDGE('',*,*,#23771,.T.);
#35129=ORIENTED_EDGE('',*,*,#25830,.F.);
#35130=ORIENTED_EDGE('',*,*,#24888,.F.);
#35131=ORIENTED_EDGE('',*,*,#25831,.T.);
#35132=ORIENTED_EDGE('',*,*,#23772,.T.);
#35133=ORIENTED_EDGE('',*,*,#25829,.F.);
#35134=ORIENTED_EDGE('',*,*,#24887,.F.);
#35135=ORIENTED_EDGE('',*,*,#25832,.T.);
#35136=ORIENTED_EDGE('',*,*,#23773,.T.);
#35137=ORIENTED_EDGE('',*,*,#25831,.F.);
#35138=ORIENTED_EDGE('',*,*,#24892,.F.);
#35139=ORIENTED_EDGE('',*,*,#25833,.T.);
#35140=ORIENTED_EDGE('',*,*,#23774,.T.);
#35141=ORIENTED_EDGE('',*,*,#25832,.F.);
#35142=ORIENTED_EDGE('',*,*,#24891,.F.);
#35143=ORIENTED_EDGE('',*,*,#25834,.T.);
#35144=ORIENTED_EDGE('',*,*,#23775,.T.);
#35145=ORIENTED_EDGE('',*,*,#25833,.F.);
#35146=ORIENTED_EDGE('',*,*,#24890,.F.);
#35147=ORIENTED_EDGE('',*,*,#25830,.T.);
#35148=ORIENTED_EDGE('',*,*,#23776,.T.);
#35149=ORIENTED_EDGE('',*,*,#25834,.F.);
#35150=ORIENTED_EDGE('',*,*,#24889,.F.);
#35151=ORIENTED_EDGE('',*,*,#25835,.T.);
#35152=ORIENTED_EDGE('',*,*,#23765,.T.);
#35153=ORIENTED_EDGE('',*,*,#25836,.F.);
#35154=ORIENTED_EDGE('',*,*,#24882,.F.);
#35155=ORIENTED_EDGE('',*,*,#25837,.T.);
#35156=ORIENTED_EDGE('',*,*,#23766,.T.);
#35157=ORIENTED_EDGE('',*,*,#25835,.F.);
#35158=ORIENTED_EDGE('',*,*,#24881,.F.);
#35159=ORIENTED_EDGE('',*,*,#25838,.T.);
#35160=ORIENTED_EDGE('',*,*,#23767,.T.);
#35161=ORIENTED_EDGE('',*,*,#25837,.F.);
#35162=ORIENTED_EDGE('',*,*,#24886,.F.);
#35163=ORIENTED_EDGE('',*,*,#25839,.T.);
#35164=ORIENTED_EDGE('',*,*,#23768,.T.);
#35165=ORIENTED_EDGE('',*,*,#25838,.F.);
#35166=ORIENTED_EDGE('',*,*,#24885,.F.);
#35167=ORIENTED_EDGE('',*,*,#25840,.T.);
#35168=ORIENTED_EDGE('',*,*,#23769,.T.);
#35169=ORIENTED_EDGE('',*,*,#25839,.F.);
#35170=ORIENTED_EDGE('',*,*,#24884,.F.);
#35171=ORIENTED_EDGE('',*,*,#25836,.T.);
#35172=ORIENTED_EDGE('',*,*,#23770,.T.);
#35173=ORIENTED_EDGE('',*,*,#25840,.F.);
#35174=ORIENTED_EDGE('',*,*,#24883,.F.);
#35175=ORIENTED_EDGE('',*,*,#25841,.T.);
#35176=ORIENTED_EDGE('',*,*,#23759,.T.);
#35177=ORIENTED_EDGE('',*,*,#25842,.F.);
#35178=ORIENTED_EDGE('',*,*,#24876,.F.);
#35179=ORIENTED_EDGE('',*,*,#25843,.T.);
#35180=ORIENTED_EDGE('',*,*,#23760,.T.);
#35181=ORIENTED_EDGE('',*,*,#25841,.F.);
#35182=ORIENTED_EDGE('',*,*,#24875,.F.);
#35183=ORIENTED_EDGE('',*,*,#25844,.T.);
#35184=ORIENTED_EDGE('',*,*,#23761,.T.);
#35185=ORIENTED_EDGE('',*,*,#25843,.F.);
#35186=ORIENTED_EDGE('',*,*,#24880,.F.);
#35187=ORIENTED_EDGE('',*,*,#25845,.T.);
#35188=ORIENTED_EDGE('',*,*,#23762,.T.);
#35189=ORIENTED_EDGE('',*,*,#25844,.F.);
#35190=ORIENTED_EDGE('',*,*,#24879,.F.);
#35191=ORIENTED_EDGE('',*,*,#25846,.T.);
#35192=ORIENTED_EDGE('',*,*,#23763,.T.);
#35193=ORIENTED_EDGE('',*,*,#25845,.F.);
#35194=ORIENTED_EDGE('',*,*,#24878,.F.);
#35195=ORIENTED_EDGE('',*,*,#25842,.T.);
#35196=ORIENTED_EDGE('',*,*,#23764,.T.);
#35197=ORIENTED_EDGE('',*,*,#25846,.F.);
#35198=ORIENTED_EDGE('',*,*,#24877,.F.);
#35199=ORIENTED_EDGE('',*,*,#25847,.T.);
#35200=ORIENTED_EDGE('',*,*,#23753,.T.);
#35201=ORIENTED_EDGE('',*,*,#25848,.F.);
#35202=ORIENTED_EDGE('',*,*,#24870,.F.);
#35203=ORIENTED_EDGE('',*,*,#25849,.T.);
#35204=ORIENTED_EDGE('',*,*,#23754,.T.);
#35205=ORIENTED_EDGE('',*,*,#25847,.F.);
#35206=ORIENTED_EDGE('',*,*,#24869,.F.);
#35207=ORIENTED_EDGE('',*,*,#25850,.T.);
#35208=ORIENTED_EDGE('',*,*,#23755,.T.);
#35209=ORIENTED_EDGE('',*,*,#25849,.F.);
#35210=ORIENTED_EDGE('',*,*,#24874,.F.);
#35211=ORIENTED_EDGE('',*,*,#25851,.T.);
#35212=ORIENTED_EDGE('',*,*,#23756,.T.);
#35213=ORIENTED_EDGE('',*,*,#25850,.F.);
#35214=ORIENTED_EDGE('',*,*,#24873,.F.);
#35215=ORIENTED_EDGE('',*,*,#25852,.T.);
#35216=ORIENTED_EDGE('',*,*,#23757,.T.);
#35217=ORIENTED_EDGE('',*,*,#25851,.F.);
#35218=ORIENTED_EDGE('',*,*,#24872,.F.);
#35219=ORIENTED_EDGE('',*,*,#25848,.T.);
#35220=ORIENTED_EDGE('',*,*,#23758,.T.);
#35221=ORIENTED_EDGE('',*,*,#25852,.F.);
#35222=ORIENTED_EDGE('',*,*,#24871,.F.);
#35223=ORIENTED_EDGE('',*,*,#25853,.T.);
#35224=ORIENTED_EDGE('',*,*,#23747,.T.);
#35225=ORIENTED_EDGE('',*,*,#25854,.F.);
#35226=ORIENTED_EDGE('',*,*,#24864,.F.);
#35227=ORIENTED_EDGE('',*,*,#25855,.T.);
#35228=ORIENTED_EDGE('',*,*,#23748,.T.);
#35229=ORIENTED_EDGE('',*,*,#25853,.F.);
#35230=ORIENTED_EDGE('',*,*,#24863,.F.);
#35231=ORIENTED_EDGE('',*,*,#25856,.T.);
#35232=ORIENTED_EDGE('',*,*,#23749,.T.);
#35233=ORIENTED_EDGE('',*,*,#25855,.F.);
#35234=ORIENTED_EDGE('',*,*,#24868,.F.);
#35235=ORIENTED_EDGE('',*,*,#25857,.T.);
#35236=ORIENTED_EDGE('',*,*,#23750,.T.);
#35237=ORIENTED_EDGE('',*,*,#25856,.F.);
#35238=ORIENTED_EDGE('',*,*,#24867,.F.);
#35239=ORIENTED_EDGE('',*,*,#25858,.T.);
#35240=ORIENTED_EDGE('',*,*,#23751,.T.);
#35241=ORIENTED_EDGE('',*,*,#25857,.F.);
#35242=ORIENTED_EDGE('',*,*,#24866,.F.);
#35243=ORIENTED_EDGE('',*,*,#25854,.T.);
#35244=ORIENTED_EDGE('',*,*,#23752,.T.);
#35245=ORIENTED_EDGE('',*,*,#25858,.F.);
#35246=ORIENTED_EDGE('',*,*,#24865,.F.);
#35247=ORIENTED_EDGE('',*,*,#25859,.T.);
#35248=ORIENTED_EDGE('',*,*,#23741,.T.);
#35249=ORIENTED_EDGE('',*,*,#25860,.F.);
#35250=ORIENTED_EDGE('',*,*,#24858,.F.);
#35251=ORIENTED_EDGE('',*,*,#25861,.T.);
#35252=ORIENTED_EDGE('',*,*,#23742,.T.);
#35253=ORIENTED_EDGE('',*,*,#25859,.F.);
#35254=ORIENTED_EDGE('',*,*,#24857,.F.);
#35255=ORIENTED_EDGE('',*,*,#25862,.T.);
#35256=ORIENTED_EDGE('',*,*,#23743,.T.);
#35257=ORIENTED_EDGE('',*,*,#25861,.F.);
#35258=ORIENTED_EDGE('',*,*,#24862,.F.);
#35259=ORIENTED_EDGE('',*,*,#25863,.T.);
#35260=ORIENTED_EDGE('',*,*,#23744,.T.);
#35261=ORIENTED_EDGE('',*,*,#25862,.F.);
#35262=ORIENTED_EDGE('',*,*,#24861,.F.);
#35263=ORIENTED_EDGE('',*,*,#25864,.T.);
#35264=ORIENTED_EDGE('',*,*,#23745,.T.);
#35265=ORIENTED_EDGE('',*,*,#25863,.F.);
#35266=ORIENTED_EDGE('',*,*,#24860,.F.);
#35267=ORIENTED_EDGE('',*,*,#25860,.T.);
#35268=ORIENTED_EDGE('',*,*,#23746,.T.);
#35269=ORIENTED_EDGE('',*,*,#25864,.F.);
#35270=ORIENTED_EDGE('',*,*,#24859,.F.);
#35271=ORIENTED_EDGE('',*,*,#25865,.T.);
#35272=ORIENTED_EDGE('',*,*,#23735,.T.);
#35273=ORIENTED_EDGE('',*,*,#25866,.F.);
#35274=ORIENTED_EDGE('',*,*,#24852,.F.);
#35275=ORIENTED_EDGE('',*,*,#25867,.T.);
#35276=ORIENTED_EDGE('',*,*,#23736,.T.);
#35277=ORIENTED_EDGE('',*,*,#25865,.F.);
#35278=ORIENTED_EDGE('',*,*,#24851,.F.);
#35279=ORIENTED_EDGE('',*,*,#25868,.T.);
#35280=ORIENTED_EDGE('',*,*,#23737,.T.);
#35281=ORIENTED_EDGE('',*,*,#25867,.F.);
#35282=ORIENTED_EDGE('',*,*,#24856,.F.);
#35283=ORIENTED_EDGE('',*,*,#25869,.T.);
#35284=ORIENTED_EDGE('',*,*,#23738,.T.);
#35285=ORIENTED_EDGE('',*,*,#25868,.F.);
#35286=ORIENTED_EDGE('',*,*,#24855,.F.);
#35287=ORIENTED_EDGE('',*,*,#25870,.T.);
#35288=ORIENTED_EDGE('',*,*,#23739,.T.);
#35289=ORIENTED_EDGE('',*,*,#25869,.F.);
#35290=ORIENTED_EDGE('',*,*,#24854,.F.);
#35291=ORIENTED_EDGE('',*,*,#25866,.T.);
#35292=ORIENTED_EDGE('',*,*,#23740,.T.);
#35293=ORIENTED_EDGE('',*,*,#25870,.F.);
#35294=ORIENTED_EDGE('',*,*,#24853,.F.);
#35295=ORIENTED_EDGE('',*,*,#25871,.T.);
#35296=ORIENTED_EDGE('',*,*,#23729,.T.);
#35297=ORIENTED_EDGE('',*,*,#25872,.F.);
#35298=ORIENTED_EDGE('',*,*,#24846,.F.);
#35299=ORIENTED_EDGE('',*,*,#25873,.T.);
#35300=ORIENTED_EDGE('',*,*,#23730,.T.);
#35301=ORIENTED_EDGE('',*,*,#25871,.F.);
#35302=ORIENTED_EDGE('',*,*,#24845,.F.);
#35303=ORIENTED_EDGE('',*,*,#25874,.T.);
#35304=ORIENTED_EDGE('',*,*,#23731,.T.);
#35305=ORIENTED_EDGE('',*,*,#25873,.F.);
#35306=ORIENTED_EDGE('',*,*,#24850,.F.);
#35307=ORIENTED_EDGE('',*,*,#25875,.T.);
#35308=ORIENTED_EDGE('',*,*,#23732,.T.);
#35309=ORIENTED_EDGE('',*,*,#25874,.F.);
#35310=ORIENTED_EDGE('',*,*,#24849,.F.);
#35311=ORIENTED_EDGE('',*,*,#25876,.T.);
#35312=ORIENTED_EDGE('',*,*,#23733,.T.);
#35313=ORIENTED_EDGE('',*,*,#25875,.F.);
#35314=ORIENTED_EDGE('',*,*,#24848,.F.);
#35315=ORIENTED_EDGE('',*,*,#25872,.T.);
#35316=ORIENTED_EDGE('',*,*,#23734,.T.);
#35317=ORIENTED_EDGE('',*,*,#25876,.F.);
#35318=ORIENTED_EDGE('',*,*,#24847,.F.);
#35319=ORIENTED_EDGE('',*,*,#25877,.T.);
#35320=ORIENTED_EDGE('',*,*,#23723,.T.);
#35321=ORIENTED_EDGE('',*,*,#25878,.F.);
#35322=ORIENTED_EDGE('',*,*,#24840,.F.);
#35323=ORIENTED_EDGE('',*,*,#25879,.T.);
#35324=ORIENTED_EDGE('',*,*,#23724,.T.);
#35325=ORIENTED_EDGE('',*,*,#25877,.F.);
#35326=ORIENTED_EDGE('',*,*,#24839,.F.);
#35327=ORIENTED_EDGE('',*,*,#25880,.T.);
#35328=ORIENTED_EDGE('',*,*,#23725,.T.);
#35329=ORIENTED_EDGE('',*,*,#25879,.F.);
#35330=ORIENTED_EDGE('',*,*,#24844,.F.);
#35331=ORIENTED_EDGE('',*,*,#25881,.T.);
#35332=ORIENTED_EDGE('',*,*,#23726,.T.);
#35333=ORIENTED_EDGE('',*,*,#25880,.F.);
#35334=ORIENTED_EDGE('',*,*,#24843,.F.);
#35335=ORIENTED_EDGE('',*,*,#25882,.T.);
#35336=ORIENTED_EDGE('',*,*,#23727,.T.);
#35337=ORIENTED_EDGE('',*,*,#25881,.F.);
#35338=ORIENTED_EDGE('',*,*,#24842,.F.);
#35339=ORIENTED_EDGE('',*,*,#25878,.T.);
#35340=ORIENTED_EDGE('',*,*,#23728,.T.);
#35341=ORIENTED_EDGE('',*,*,#25882,.F.);
#35342=ORIENTED_EDGE('',*,*,#24841,.F.);
#35343=ORIENTED_EDGE('',*,*,#25883,.T.);
#35344=ORIENTED_EDGE('',*,*,#23717,.T.);
#35345=ORIENTED_EDGE('',*,*,#25884,.F.);
#35346=ORIENTED_EDGE('',*,*,#24834,.F.);
#35347=ORIENTED_EDGE('',*,*,#25885,.T.);
#35348=ORIENTED_EDGE('',*,*,#23718,.T.);
#35349=ORIENTED_EDGE('',*,*,#25883,.F.);
#35350=ORIENTED_EDGE('',*,*,#24833,.F.);
#35351=ORIENTED_EDGE('',*,*,#25886,.T.);
#35352=ORIENTED_EDGE('',*,*,#23719,.T.);
#35353=ORIENTED_EDGE('',*,*,#25885,.F.);
#35354=ORIENTED_EDGE('',*,*,#24838,.F.);
#35355=ORIENTED_EDGE('',*,*,#25887,.T.);
#35356=ORIENTED_EDGE('',*,*,#23720,.T.);
#35357=ORIENTED_EDGE('',*,*,#25886,.F.);
#35358=ORIENTED_EDGE('',*,*,#24837,.F.);
#35359=ORIENTED_EDGE('',*,*,#25888,.T.);
#35360=ORIENTED_EDGE('',*,*,#23721,.T.);
#35361=ORIENTED_EDGE('',*,*,#25887,.F.);
#35362=ORIENTED_EDGE('',*,*,#24836,.F.);
#35363=ORIENTED_EDGE('',*,*,#25884,.T.);
#35364=ORIENTED_EDGE('',*,*,#23722,.T.);
#35365=ORIENTED_EDGE('',*,*,#25888,.F.);
#35366=ORIENTED_EDGE('',*,*,#24835,.F.);
#35367=ORIENTED_EDGE('',*,*,#25889,.T.);
#35368=ORIENTED_EDGE('',*,*,#23711,.T.);
#35369=ORIENTED_EDGE('',*,*,#25890,.F.);
#35370=ORIENTED_EDGE('',*,*,#24828,.F.);
#35371=ORIENTED_EDGE('',*,*,#25891,.T.);
#35372=ORIENTED_EDGE('',*,*,#23712,.T.);
#35373=ORIENTED_EDGE('',*,*,#25889,.F.);
#35374=ORIENTED_EDGE('',*,*,#24827,.F.);
#35375=ORIENTED_EDGE('',*,*,#25892,.T.);
#35376=ORIENTED_EDGE('',*,*,#23713,.T.);
#35377=ORIENTED_EDGE('',*,*,#25891,.F.);
#35378=ORIENTED_EDGE('',*,*,#24832,.F.);
#35379=ORIENTED_EDGE('',*,*,#25893,.T.);
#35380=ORIENTED_EDGE('',*,*,#23714,.T.);
#35381=ORIENTED_EDGE('',*,*,#25892,.F.);
#35382=ORIENTED_EDGE('',*,*,#24831,.F.);
#35383=ORIENTED_EDGE('',*,*,#25894,.T.);
#35384=ORIENTED_EDGE('',*,*,#23715,.T.);
#35385=ORIENTED_EDGE('',*,*,#25893,.F.);
#35386=ORIENTED_EDGE('',*,*,#24830,.F.);
#35387=ORIENTED_EDGE('',*,*,#25890,.T.);
#35388=ORIENTED_EDGE('',*,*,#23716,.T.);
#35389=ORIENTED_EDGE('',*,*,#25894,.F.);
#35390=ORIENTED_EDGE('',*,*,#24829,.F.);
#35391=ORIENTED_EDGE('',*,*,#25895,.T.);
#35392=ORIENTED_EDGE('',*,*,#23705,.T.);
#35393=ORIENTED_EDGE('',*,*,#25896,.F.);
#35394=ORIENTED_EDGE('',*,*,#24822,.F.);
#35395=ORIENTED_EDGE('',*,*,#25897,.T.);
#35396=ORIENTED_EDGE('',*,*,#23706,.T.);
#35397=ORIENTED_EDGE('',*,*,#25895,.F.);
#35398=ORIENTED_EDGE('',*,*,#24821,.F.);
#35399=ORIENTED_EDGE('',*,*,#25898,.T.);
#35400=ORIENTED_EDGE('',*,*,#23707,.T.);
#35401=ORIENTED_EDGE('',*,*,#25897,.F.);
#35402=ORIENTED_EDGE('',*,*,#24826,.F.);
#35403=ORIENTED_EDGE('',*,*,#25899,.T.);
#35404=ORIENTED_EDGE('',*,*,#23708,.T.);
#35405=ORIENTED_EDGE('',*,*,#25898,.F.);
#35406=ORIENTED_EDGE('',*,*,#24825,.F.);
#35407=ORIENTED_EDGE('',*,*,#25900,.T.);
#35408=ORIENTED_EDGE('',*,*,#23709,.T.);
#35409=ORIENTED_EDGE('',*,*,#25899,.F.);
#35410=ORIENTED_EDGE('',*,*,#24824,.F.);
#35411=ORIENTED_EDGE('',*,*,#25896,.T.);
#35412=ORIENTED_EDGE('',*,*,#23710,.T.);
#35413=ORIENTED_EDGE('',*,*,#25900,.F.);
#35414=ORIENTED_EDGE('',*,*,#24823,.F.);
#35415=ORIENTED_EDGE('',*,*,#25901,.T.);
#35416=ORIENTED_EDGE('',*,*,#23699,.T.);
#35417=ORIENTED_EDGE('',*,*,#25902,.F.);
#35418=ORIENTED_EDGE('',*,*,#24816,.F.);
#35419=ORIENTED_EDGE('',*,*,#25903,.T.);
#35420=ORIENTED_EDGE('',*,*,#23700,.T.);
#35421=ORIENTED_EDGE('',*,*,#25901,.F.);
#35422=ORIENTED_EDGE('',*,*,#24815,.F.);
#35423=ORIENTED_EDGE('',*,*,#25904,.T.);
#35424=ORIENTED_EDGE('',*,*,#23701,.T.);
#35425=ORIENTED_EDGE('',*,*,#25903,.F.);
#35426=ORIENTED_EDGE('',*,*,#24820,.F.);
#35427=ORIENTED_EDGE('',*,*,#25905,.T.);
#35428=ORIENTED_EDGE('',*,*,#23702,.T.);
#35429=ORIENTED_EDGE('',*,*,#25904,.F.);
#35430=ORIENTED_EDGE('',*,*,#24819,.F.);
#35431=ORIENTED_EDGE('',*,*,#25906,.T.);
#35432=ORIENTED_EDGE('',*,*,#23703,.T.);
#35433=ORIENTED_EDGE('',*,*,#25905,.F.);
#35434=ORIENTED_EDGE('',*,*,#24818,.F.);
#35435=ORIENTED_EDGE('',*,*,#25902,.T.);
#35436=ORIENTED_EDGE('',*,*,#23704,.T.);
#35437=ORIENTED_EDGE('',*,*,#25906,.F.);
#35438=ORIENTED_EDGE('',*,*,#24817,.F.);
#35439=ORIENTED_EDGE('',*,*,#25907,.T.);
#35440=ORIENTED_EDGE('',*,*,#23693,.T.);
#35441=ORIENTED_EDGE('',*,*,#25908,.F.);
#35442=ORIENTED_EDGE('',*,*,#24810,.F.);
#35443=ORIENTED_EDGE('',*,*,#25909,.T.);
#35444=ORIENTED_EDGE('',*,*,#23694,.T.);
#35445=ORIENTED_EDGE('',*,*,#25907,.F.);
#35446=ORIENTED_EDGE('',*,*,#24809,.F.);
#35447=ORIENTED_EDGE('',*,*,#25910,.T.);
#35448=ORIENTED_EDGE('',*,*,#23695,.T.);
#35449=ORIENTED_EDGE('',*,*,#25909,.F.);
#35450=ORIENTED_EDGE('',*,*,#24814,.F.);
#35451=ORIENTED_EDGE('',*,*,#25911,.T.);
#35452=ORIENTED_EDGE('',*,*,#23696,.T.);
#35453=ORIENTED_EDGE('',*,*,#25910,.F.);
#35454=ORIENTED_EDGE('',*,*,#24813,.F.);
#35455=ORIENTED_EDGE('',*,*,#25912,.T.);
#35456=ORIENTED_EDGE('',*,*,#23697,.T.);
#35457=ORIENTED_EDGE('',*,*,#25911,.F.);
#35458=ORIENTED_EDGE('',*,*,#24812,.F.);
#35459=ORIENTED_EDGE('',*,*,#25908,.T.);
#35460=ORIENTED_EDGE('',*,*,#23698,.T.);
#35461=ORIENTED_EDGE('',*,*,#25912,.F.);
#35462=ORIENTED_EDGE('',*,*,#24811,.F.);
#35463=ORIENTED_EDGE('',*,*,#25913,.T.);
#35464=ORIENTED_EDGE('',*,*,#23687,.T.);
#35465=ORIENTED_EDGE('',*,*,#25914,.F.);
#35466=ORIENTED_EDGE('',*,*,#24804,.F.);
#35467=ORIENTED_EDGE('',*,*,#25915,.T.);
#35468=ORIENTED_EDGE('',*,*,#23688,.T.);
#35469=ORIENTED_EDGE('',*,*,#25913,.F.);
#35470=ORIENTED_EDGE('',*,*,#24803,.F.);
#35471=ORIENTED_EDGE('',*,*,#25916,.T.);
#35472=ORIENTED_EDGE('',*,*,#23689,.T.);
#35473=ORIENTED_EDGE('',*,*,#25915,.F.);
#35474=ORIENTED_EDGE('',*,*,#24808,.F.);
#35475=ORIENTED_EDGE('',*,*,#25917,.T.);
#35476=ORIENTED_EDGE('',*,*,#23690,.T.);
#35477=ORIENTED_EDGE('',*,*,#25916,.F.);
#35478=ORIENTED_EDGE('',*,*,#24807,.F.);
#35479=ORIENTED_EDGE('',*,*,#25918,.T.);
#35480=ORIENTED_EDGE('',*,*,#23691,.T.);
#35481=ORIENTED_EDGE('',*,*,#25917,.F.);
#35482=ORIENTED_EDGE('',*,*,#24806,.F.);
#35483=ORIENTED_EDGE('',*,*,#25914,.T.);
#35484=ORIENTED_EDGE('',*,*,#23692,.T.);
#35485=ORIENTED_EDGE('',*,*,#25918,.F.);
#35486=ORIENTED_EDGE('',*,*,#24805,.F.);
#35487=ORIENTED_EDGE('',*,*,#25919,.T.);
#35488=ORIENTED_EDGE('',*,*,#23681,.T.);
#35489=ORIENTED_EDGE('',*,*,#25920,.F.);
#35490=ORIENTED_EDGE('',*,*,#24798,.F.);
#35491=ORIENTED_EDGE('',*,*,#25921,.T.);
#35492=ORIENTED_EDGE('',*,*,#23682,.T.);
#35493=ORIENTED_EDGE('',*,*,#25919,.F.);
#35494=ORIENTED_EDGE('',*,*,#24797,.F.);
#35495=ORIENTED_EDGE('',*,*,#25922,.T.);
#35496=ORIENTED_EDGE('',*,*,#23683,.T.);
#35497=ORIENTED_EDGE('',*,*,#25921,.F.);
#35498=ORIENTED_EDGE('',*,*,#24802,.F.);
#35499=ORIENTED_EDGE('',*,*,#25923,.T.);
#35500=ORIENTED_EDGE('',*,*,#23684,.T.);
#35501=ORIENTED_EDGE('',*,*,#25922,.F.);
#35502=ORIENTED_EDGE('',*,*,#24801,.F.);
#35503=ORIENTED_EDGE('',*,*,#25924,.T.);
#35504=ORIENTED_EDGE('',*,*,#23685,.T.);
#35505=ORIENTED_EDGE('',*,*,#25923,.F.);
#35506=ORIENTED_EDGE('',*,*,#24800,.F.);
#35507=ORIENTED_EDGE('',*,*,#25920,.T.);
#35508=ORIENTED_EDGE('',*,*,#23686,.T.);
#35509=ORIENTED_EDGE('',*,*,#25924,.F.);
#35510=ORIENTED_EDGE('',*,*,#24799,.F.);
#35511=ORIENTED_EDGE('',*,*,#25925,.T.);
#35512=ORIENTED_EDGE('',*,*,#23675,.T.);
#35513=ORIENTED_EDGE('',*,*,#25926,.F.);
#35514=ORIENTED_EDGE('',*,*,#24792,.F.);
#35515=ORIENTED_EDGE('',*,*,#25927,.T.);
#35516=ORIENTED_EDGE('',*,*,#23676,.T.);
#35517=ORIENTED_EDGE('',*,*,#25925,.F.);
#35518=ORIENTED_EDGE('',*,*,#24791,.F.);
#35519=ORIENTED_EDGE('',*,*,#25928,.T.);
#35520=ORIENTED_EDGE('',*,*,#23677,.T.);
#35521=ORIENTED_EDGE('',*,*,#25927,.F.);
#35522=ORIENTED_EDGE('',*,*,#24796,.F.);
#35523=ORIENTED_EDGE('',*,*,#25929,.T.);
#35524=ORIENTED_EDGE('',*,*,#23678,.T.);
#35525=ORIENTED_EDGE('',*,*,#25928,.F.);
#35526=ORIENTED_EDGE('',*,*,#24795,.F.);
#35527=ORIENTED_EDGE('',*,*,#25930,.T.);
#35528=ORIENTED_EDGE('',*,*,#23679,.T.);
#35529=ORIENTED_EDGE('',*,*,#25929,.F.);
#35530=ORIENTED_EDGE('',*,*,#24794,.F.);
#35531=ORIENTED_EDGE('',*,*,#25926,.T.);
#35532=ORIENTED_EDGE('',*,*,#23680,.T.);
#35533=ORIENTED_EDGE('',*,*,#25930,.F.);
#35534=ORIENTED_EDGE('',*,*,#24793,.F.);
#35535=ORIENTED_EDGE('',*,*,#25931,.T.);
#35536=ORIENTED_EDGE('',*,*,#23669,.T.);
#35537=ORIENTED_EDGE('',*,*,#25932,.F.);
#35538=ORIENTED_EDGE('',*,*,#24786,.F.);
#35539=ORIENTED_EDGE('',*,*,#25933,.T.);
#35540=ORIENTED_EDGE('',*,*,#23670,.T.);
#35541=ORIENTED_EDGE('',*,*,#25931,.F.);
#35542=ORIENTED_EDGE('',*,*,#24785,.F.);
#35543=ORIENTED_EDGE('',*,*,#25934,.T.);
#35544=ORIENTED_EDGE('',*,*,#23671,.T.);
#35545=ORIENTED_EDGE('',*,*,#25933,.F.);
#35546=ORIENTED_EDGE('',*,*,#24790,.F.);
#35547=ORIENTED_EDGE('',*,*,#25935,.T.);
#35548=ORIENTED_EDGE('',*,*,#23672,.T.);
#35549=ORIENTED_EDGE('',*,*,#25934,.F.);
#35550=ORIENTED_EDGE('',*,*,#24789,.F.);
#35551=ORIENTED_EDGE('',*,*,#25936,.T.);
#35552=ORIENTED_EDGE('',*,*,#23673,.T.);
#35553=ORIENTED_EDGE('',*,*,#25935,.F.);
#35554=ORIENTED_EDGE('',*,*,#24788,.F.);
#35555=ORIENTED_EDGE('',*,*,#25932,.T.);
#35556=ORIENTED_EDGE('',*,*,#23674,.T.);
#35557=ORIENTED_EDGE('',*,*,#25936,.F.);
#35558=ORIENTED_EDGE('',*,*,#24787,.F.);
#35559=ORIENTED_EDGE('',*,*,#25937,.T.);
#35560=ORIENTED_EDGE('',*,*,#23663,.T.);
#35561=ORIENTED_EDGE('',*,*,#25938,.F.);
#35562=ORIENTED_EDGE('',*,*,#24780,.F.);
#35563=ORIENTED_EDGE('',*,*,#25939,.T.);
#35564=ORIENTED_EDGE('',*,*,#23664,.T.);
#35565=ORIENTED_EDGE('',*,*,#25937,.F.);
#35566=ORIENTED_EDGE('',*,*,#24779,.F.);
#35567=ORIENTED_EDGE('',*,*,#25940,.T.);
#35568=ORIENTED_EDGE('',*,*,#23665,.T.);
#35569=ORIENTED_EDGE('',*,*,#25939,.F.);
#35570=ORIENTED_EDGE('',*,*,#24784,.F.);
#35571=ORIENTED_EDGE('',*,*,#25941,.T.);
#35572=ORIENTED_EDGE('',*,*,#23666,.T.);
#35573=ORIENTED_EDGE('',*,*,#25940,.F.);
#35574=ORIENTED_EDGE('',*,*,#24783,.F.);
#35575=ORIENTED_EDGE('',*,*,#25942,.T.);
#35576=ORIENTED_EDGE('',*,*,#23667,.T.);
#35577=ORIENTED_EDGE('',*,*,#25941,.F.);
#35578=ORIENTED_EDGE('',*,*,#24782,.F.);
#35579=ORIENTED_EDGE('',*,*,#25938,.T.);
#35580=ORIENTED_EDGE('',*,*,#23668,.T.);
#35581=ORIENTED_EDGE('',*,*,#25942,.F.);
#35582=ORIENTED_EDGE('',*,*,#24781,.F.);
#35583=ORIENTED_EDGE('',*,*,#25943,.T.);
#35584=ORIENTED_EDGE('',*,*,#23657,.T.);
#35585=ORIENTED_EDGE('',*,*,#25944,.F.);
#35586=ORIENTED_EDGE('',*,*,#24774,.F.);
#35587=ORIENTED_EDGE('',*,*,#25945,.T.);
#35588=ORIENTED_EDGE('',*,*,#23658,.T.);
#35589=ORIENTED_EDGE('',*,*,#25943,.F.);
#35590=ORIENTED_EDGE('',*,*,#24773,.F.);
#35591=ORIENTED_EDGE('',*,*,#25946,.T.);
#35592=ORIENTED_EDGE('',*,*,#23659,.T.);
#35593=ORIENTED_EDGE('',*,*,#25945,.F.);
#35594=ORIENTED_EDGE('',*,*,#24778,.F.);
#35595=ORIENTED_EDGE('',*,*,#25947,.T.);
#35596=ORIENTED_EDGE('',*,*,#23660,.T.);
#35597=ORIENTED_EDGE('',*,*,#25946,.F.);
#35598=ORIENTED_EDGE('',*,*,#24777,.F.);
#35599=ORIENTED_EDGE('',*,*,#25948,.T.);
#35600=ORIENTED_EDGE('',*,*,#23661,.T.);
#35601=ORIENTED_EDGE('',*,*,#25947,.F.);
#35602=ORIENTED_EDGE('',*,*,#24776,.F.);
#35603=ORIENTED_EDGE('',*,*,#25944,.T.);
#35604=ORIENTED_EDGE('',*,*,#23662,.T.);
#35605=ORIENTED_EDGE('',*,*,#25948,.F.);
#35606=ORIENTED_EDGE('',*,*,#24775,.F.);
#35607=ORIENTED_EDGE('',*,*,#25949,.T.);
#35608=ORIENTED_EDGE('',*,*,#23651,.T.);
#35609=ORIENTED_EDGE('',*,*,#25950,.F.);
#35610=ORIENTED_EDGE('',*,*,#24768,.F.);
#35611=ORIENTED_EDGE('',*,*,#25951,.T.);
#35612=ORIENTED_EDGE('',*,*,#23652,.T.);
#35613=ORIENTED_EDGE('',*,*,#25949,.F.);
#35614=ORIENTED_EDGE('',*,*,#24767,.F.);
#35615=ORIENTED_EDGE('',*,*,#25952,.T.);
#35616=ORIENTED_EDGE('',*,*,#23653,.T.);
#35617=ORIENTED_EDGE('',*,*,#25951,.F.);
#35618=ORIENTED_EDGE('',*,*,#24772,.F.);
#35619=ORIENTED_EDGE('',*,*,#25953,.T.);
#35620=ORIENTED_EDGE('',*,*,#23654,.T.);
#35621=ORIENTED_EDGE('',*,*,#25952,.F.);
#35622=ORIENTED_EDGE('',*,*,#24771,.F.);
#35623=ORIENTED_EDGE('',*,*,#25954,.T.);
#35624=ORIENTED_EDGE('',*,*,#23655,.T.);
#35625=ORIENTED_EDGE('',*,*,#25953,.F.);
#35626=ORIENTED_EDGE('',*,*,#24770,.F.);
#35627=ORIENTED_EDGE('',*,*,#25950,.T.);
#35628=ORIENTED_EDGE('',*,*,#23656,.T.);
#35629=ORIENTED_EDGE('',*,*,#25954,.F.);
#35630=ORIENTED_EDGE('',*,*,#24769,.F.);
#35631=ORIENTED_EDGE('',*,*,#25955,.T.);
#35632=ORIENTED_EDGE('',*,*,#23645,.T.);
#35633=ORIENTED_EDGE('',*,*,#25956,.F.);
#35634=ORIENTED_EDGE('',*,*,#24762,.F.);
#35635=ORIENTED_EDGE('',*,*,#25957,.T.);
#35636=ORIENTED_EDGE('',*,*,#23646,.T.);
#35637=ORIENTED_EDGE('',*,*,#25955,.F.);
#35638=ORIENTED_EDGE('',*,*,#24761,.F.);
#35639=ORIENTED_EDGE('',*,*,#25958,.T.);
#35640=ORIENTED_EDGE('',*,*,#23647,.T.);
#35641=ORIENTED_EDGE('',*,*,#25957,.F.);
#35642=ORIENTED_EDGE('',*,*,#24766,.F.);
#35643=ORIENTED_EDGE('',*,*,#25959,.T.);
#35644=ORIENTED_EDGE('',*,*,#23648,.T.);
#35645=ORIENTED_EDGE('',*,*,#25958,.F.);
#35646=ORIENTED_EDGE('',*,*,#24765,.F.);
#35647=ORIENTED_EDGE('',*,*,#25960,.T.);
#35648=ORIENTED_EDGE('',*,*,#23649,.T.);
#35649=ORIENTED_EDGE('',*,*,#25959,.F.);
#35650=ORIENTED_EDGE('',*,*,#24764,.F.);
#35651=ORIENTED_EDGE('',*,*,#25956,.T.);
#35652=ORIENTED_EDGE('',*,*,#23650,.T.);
#35653=ORIENTED_EDGE('',*,*,#25960,.F.);
#35654=ORIENTED_EDGE('',*,*,#24763,.F.);
#35655=ORIENTED_EDGE('',*,*,#25961,.T.);
#35656=ORIENTED_EDGE('',*,*,#23639,.T.);
#35657=ORIENTED_EDGE('',*,*,#25962,.F.);
#35658=ORIENTED_EDGE('',*,*,#24756,.F.);
#35659=ORIENTED_EDGE('',*,*,#25963,.T.);
#35660=ORIENTED_EDGE('',*,*,#23640,.T.);
#35661=ORIENTED_EDGE('',*,*,#25961,.F.);
#35662=ORIENTED_EDGE('',*,*,#24755,.F.);
#35663=ORIENTED_EDGE('',*,*,#25964,.T.);
#35664=ORIENTED_EDGE('',*,*,#23641,.T.);
#35665=ORIENTED_EDGE('',*,*,#25963,.F.);
#35666=ORIENTED_EDGE('',*,*,#24760,.F.);
#35667=ORIENTED_EDGE('',*,*,#25965,.T.);
#35668=ORIENTED_EDGE('',*,*,#23642,.T.);
#35669=ORIENTED_EDGE('',*,*,#25964,.F.);
#35670=ORIENTED_EDGE('',*,*,#24759,.F.);
#35671=ORIENTED_EDGE('',*,*,#25966,.T.);
#35672=ORIENTED_EDGE('',*,*,#23643,.T.);
#35673=ORIENTED_EDGE('',*,*,#25965,.F.);
#35674=ORIENTED_EDGE('',*,*,#24758,.F.);
#35675=ORIENTED_EDGE('',*,*,#25962,.T.);
#35676=ORIENTED_EDGE('',*,*,#23644,.T.);
#35677=ORIENTED_EDGE('',*,*,#25966,.F.);
#35678=ORIENTED_EDGE('',*,*,#24757,.F.);
#35679=ORIENTED_EDGE('',*,*,#25967,.T.);
#35680=ORIENTED_EDGE('',*,*,#23633,.T.);
#35681=ORIENTED_EDGE('',*,*,#25968,.F.);
#35682=ORIENTED_EDGE('',*,*,#24750,.F.);
#35683=ORIENTED_EDGE('',*,*,#25969,.T.);
#35684=ORIENTED_EDGE('',*,*,#23634,.T.);
#35685=ORIENTED_EDGE('',*,*,#25967,.F.);
#35686=ORIENTED_EDGE('',*,*,#24749,.F.);
#35687=ORIENTED_EDGE('',*,*,#25970,.T.);
#35688=ORIENTED_EDGE('',*,*,#23635,.T.);
#35689=ORIENTED_EDGE('',*,*,#25969,.F.);
#35690=ORIENTED_EDGE('',*,*,#24754,.F.);
#35691=ORIENTED_EDGE('',*,*,#25971,.T.);
#35692=ORIENTED_EDGE('',*,*,#23636,.T.);
#35693=ORIENTED_EDGE('',*,*,#25970,.F.);
#35694=ORIENTED_EDGE('',*,*,#24753,.F.);
#35695=ORIENTED_EDGE('',*,*,#25972,.T.);
#35696=ORIENTED_EDGE('',*,*,#23637,.T.);
#35697=ORIENTED_EDGE('',*,*,#25971,.F.);
#35698=ORIENTED_EDGE('',*,*,#24752,.F.);
#35699=ORIENTED_EDGE('',*,*,#25968,.T.);
#35700=ORIENTED_EDGE('',*,*,#23638,.T.);
#35701=ORIENTED_EDGE('',*,*,#25972,.F.);
#35702=ORIENTED_EDGE('',*,*,#24751,.F.);
#35703=ORIENTED_EDGE('',*,*,#25973,.T.);
#35704=ORIENTED_EDGE('',*,*,#23627,.T.);
#35705=ORIENTED_EDGE('',*,*,#25974,.F.);
#35706=ORIENTED_EDGE('',*,*,#24744,.F.);
#35707=ORIENTED_EDGE('',*,*,#25975,.T.);
#35708=ORIENTED_EDGE('',*,*,#23628,.T.);
#35709=ORIENTED_EDGE('',*,*,#25973,.F.);
#35710=ORIENTED_EDGE('',*,*,#24743,.F.);
#35711=ORIENTED_EDGE('',*,*,#25976,.T.);
#35712=ORIENTED_EDGE('',*,*,#23629,.T.);
#35713=ORIENTED_EDGE('',*,*,#25975,.F.);
#35714=ORIENTED_EDGE('',*,*,#24748,.F.);
#35715=ORIENTED_EDGE('',*,*,#25977,.T.);
#35716=ORIENTED_EDGE('',*,*,#23630,.T.);
#35717=ORIENTED_EDGE('',*,*,#25976,.F.);
#35718=ORIENTED_EDGE('',*,*,#24747,.F.);
#35719=ORIENTED_EDGE('',*,*,#25978,.T.);
#35720=ORIENTED_EDGE('',*,*,#23631,.T.);
#35721=ORIENTED_EDGE('',*,*,#25977,.F.);
#35722=ORIENTED_EDGE('',*,*,#24746,.F.);
#35723=ORIENTED_EDGE('',*,*,#25974,.T.);
#35724=ORIENTED_EDGE('',*,*,#23632,.T.);
#35725=ORIENTED_EDGE('',*,*,#25978,.F.);
#35726=ORIENTED_EDGE('',*,*,#24745,.F.);
#35727=ORIENTED_EDGE('',*,*,#25979,.T.);
#35728=ORIENTED_EDGE('',*,*,#23621,.T.);
#35729=ORIENTED_EDGE('',*,*,#25980,.F.);
#35730=ORIENTED_EDGE('',*,*,#24738,.F.);
#35731=ORIENTED_EDGE('',*,*,#25981,.T.);
#35732=ORIENTED_EDGE('',*,*,#23622,.T.);
#35733=ORIENTED_EDGE('',*,*,#25979,.F.);
#35734=ORIENTED_EDGE('',*,*,#24737,.F.);
#35735=ORIENTED_EDGE('',*,*,#25982,.T.);
#35736=ORIENTED_EDGE('',*,*,#23623,.T.);
#35737=ORIENTED_EDGE('',*,*,#25981,.F.);
#35738=ORIENTED_EDGE('',*,*,#24742,.F.);
#35739=ORIENTED_EDGE('',*,*,#25983,.T.);
#35740=ORIENTED_EDGE('',*,*,#23624,.T.);
#35741=ORIENTED_EDGE('',*,*,#25982,.F.);
#35742=ORIENTED_EDGE('',*,*,#24741,.F.);
#35743=ORIENTED_EDGE('',*,*,#25984,.T.);
#35744=ORIENTED_EDGE('',*,*,#23625,.T.);
#35745=ORIENTED_EDGE('',*,*,#25983,.F.);
#35746=ORIENTED_EDGE('',*,*,#24740,.F.);
#35747=ORIENTED_EDGE('',*,*,#25980,.T.);
#35748=ORIENTED_EDGE('',*,*,#23626,.T.);
#35749=ORIENTED_EDGE('',*,*,#25984,.F.);
#35750=ORIENTED_EDGE('',*,*,#24739,.F.);
#35751=ORIENTED_EDGE('',*,*,#25985,.T.);
#35752=ORIENTED_EDGE('',*,*,#23615,.T.);
#35753=ORIENTED_EDGE('',*,*,#25986,.F.);
#35754=ORIENTED_EDGE('',*,*,#24732,.F.);
#35755=ORIENTED_EDGE('',*,*,#25987,.T.);
#35756=ORIENTED_EDGE('',*,*,#23616,.T.);
#35757=ORIENTED_EDGE('',*,*,#25985,.F.);
#35758=ORIENTED_EDGE('',*,*,#24731,.F.);
#35759=ORIENTED_EDGE('',*,*,#25988,.T.);
#35760=ORIENTED_EDGE('',*,*,#23617,.T.);
#35761=ORIENTED_EDGE('',*,*,#25987,.F.);
#35762=ORIENTED_EDGE('',*,*,#24736,.F.);
#35763=ORIENTED_EDGE('',*,*,#25989,.T.);
#35764=ORIENTED_EDGE('',*,*,#23618,.T.);
#35765=ORIENTED_EDGE('',*,*,#25988,.F.);
#35766=ORIENTED_EDGE('',*,*,#24735,.F.);
#35767=ORIENTED_EDGE('',*,*,#25990,.T.);
#35768=ORIENTED_EDGE('',*,*,#23619,.T.);
#35769=ORIENTED_EDGE('',*,*,#25989,.F.);
#35770=ORIENTED_EDGE('',*,*,#24734,.F.);
#35771=ORIENTED_EDGE('',*,*,#25986,.T.);
#35772=ORIENTED_EDGE('',*,*,#23620,.T.);
#35773=ORIENTED_EDGE('',*,*,#25990,.F.);
#35774=ORIENTED_EDGE('',*,*,#24733,.F.);
#35775=ORIENTED_EDGE('',*,*,#25991,.T.);
#35776=ORIENTED_EDGE('',*,*,#23609,.T.);
#35777=ORIENTED_EDGE('',*,*,#25992,.F.);
#35778=ORIENTED_EDGE('',*,*,#24726,.F.);
#35779=ORIENTED_EDGE('',*,*,#25993,.T.);
#35780=ORIENTED_EDGE('',*,*,#23610,.T.);
#35781=ORIENTED_EDGE('',*,*,#25991,.F.);
#35782=ORIENTED_EDGE('',*,*,#24725,.F.);
#35783=ORIENTED_EDGE('',*,*,#25994,.T.);
#35784=ORIENTED_EDGE('',*,*,#23611,.T.);
#35785=ORIENTED_EDGE('',*,*,#25993,.F.);
#35786=ORIENTED_EDGE('',*,*,#24730,.F.);
#35787=ORIENTED_EDGE('',*,*,#25995,.T.);
#35788=ORIENTED_EDGE('',*,*,#23612,.T.);
#35789=ORIENTED_EDGE('',*,*,#25994,.F.);
#35790=ORIENTED_EDGE('',*,*,#24729,.F.);
#35791=ORIENTED_EDGE('',*,*,#25996,.T.);
#35792=ORIENTED_EDGE('',*,*,#23613,.T.);
#35793=ORIENTED_EDGE('',*,*,#25995,.F.);
#35794=ORIENTED_EDGE('',*,*,#24728,.F.);
#35795=ORIENTED_EDGE('',*,*,#25992,.T.);
#35796=ORIENTED_EDGE('',*,*,#23614,.T.);
#35797=ORIENTED_EDGE('',*,*,#25996,.F.);
#35798=ORIENTED_EDGE('',*,*,#24727,.F.);
#35799=ORIENTED_EDGE('',*,*,#25997,.T.);
#35800=ORIENTED_EDGE('',*,*,#23603,.T.);
#35801=ORIENTED_EDGE('',*,*,#25998,.F.);
#35802=ORIENTED_EDGE('',*,*,#24720,.F.);
#35803=ORIENTED_EDGE('',*,*,#25999,.T.);
#35804=ORIENTED_EDGE('',*,*,#23604,.T.);
#35805=ORIENTED_EDGE('',*,*,#25997,.F.);
#35806=ORIENTED_EDGE('',*,*,#24719,.F.);
#35807=ORIENTED_EDGE('',*,*,#26000,.T.);
#35808=ORIENTED_EDGE('',*,*,#23605,.T.);
#35809=ORIENTED_EDGE('',*,*,#25999,.F.);
#35810=ORIENTED_EDGE('',*,*,#24724,.F.);
#35811=ORIENTED_EDGE('',*,*,#26001,.T.);
#35812=ORIENTED_EDGE('',*,*,#23606,.T.);
#35813=ORIENTED_EDGE('',*,*,#26000,.F.);
#35814=ORIENTED_EDGE('',*,*,#24723,.F.);
#35815=ORIENTED_EDGE('',*,*,#26002,.T.);
#35816=ORIENTED_EDGE('',*,*,#23607,.T.);
#35817=ORIENTED_EDGE('',*,*,#26001,.F.);
#35818=ORIENTED_EDGE('',*,*,#24722,.F.);
#35819=ORIENTED_EDGE('',*,*,#25998,.T.);
#35820=ORIENTED_EDGE('',*,*,#23608,.T.);
#35821=ORIENTED_EDGE('',*,*,#26002,.F.);
#35822=ORIENTED_EDGE('',*,*,#24721,.F.);
#35823=ORIENTED_EDGE('',*,*,#26003,.T.);
#35824=ORIENTED_EDGE('',*,*,#23597,.T.);
#35825=ORIENTED_EDGE('',*,*,#26004,.F.);
#35826=ORIENTED_EDGE('',*,*,#24714,.F.);
#35827=ORIENTED_EDGE('',*,*,#26005,.T.);
#35828=ORIENTED_EDGE('',*,*,#23598,.T.);
#35829=ORIENTED_EDGE('',*,*,#26003,.F.);
#35830=ORIENTED_EDGE('',*,*,#24713,.F.);
#35831=ORIENTED_EDGE('',*,*,#26006,.T.);
#35832=ORIENTED_EDGE('',*,*,#23599,.T.);
#35833=ORIENTED_EDGE('',*,*,#26005,.F.);
#35834=ORIENTED_EDGE('',*,*,#24718,.F.);
#35835=ORIENTED_EDGE('',*,*,#26007,.T.);
#35836=ORIENTED_EDGE('',*,*,#23600,.T.);
#35837=ORIENTED_EDGE('',*,*,#26006,.F.);
#35838=ORIENTED_EDGE('',*,*,#24717,.F.);
#35839=ORIENTED_EDGE('',*,*,#26008,.T.);
#35840=ORIENTED_EDGE('',*,*,#23601,.T.);
#35841=ORIENTED_EDGE('',*,*,#26007,.F.);
#35842=ORIENTED_EDGE('',*,*,#24716,.F.);
#35843=ORIENTED_EDGE('',*,*,#26004,.T.);
#35844=ORIENTED_EDGE('',*,*,#23602,.T.);
#35845=ORIENTED_EDGE('',*,*,#26008,.F.);
#35846=ORIENTED_EDGE('',*,*,#24715,.F.);
#35847=ORIENTED_EDGE('',*,*,#26009,.T.);
#35848=ORIENTED_EDGE('',*,*,#23591,.T.);
#35849=ORIENTED_EDGE('',*,*,#26010,.F.);
#35850=ORIENTED_EDGE('',*,*,#24708,.F.);
#35851=ORIENTED_EDGE('',*,*,#26011,.T.);
#35852=ORIENTED_EDGE('',*,*,#23592,.T.);
#35853=ORIENTED_EDGE('',*,*,#26009,.F.);
#35854=ORIENTED_EDGE('',*,*,#24707,.F.);
#35855=ORIENTED_EDGE('',*,*,#26012,.T.);
#35856=ORIENTED_EDGE('',*,*,#23593,.T.);
#35857=ORIENTED_EDGE('',*,*,#26011,.F.);
#35858=ORIENTED_EDGE('',*,*,#24712,.F.);
#35859=ORIENTED_EDGE('',*,*,#26013,.T.);
#35860=ORIENTED_EDGE('',*,*,#23594,.T.);
#35861=ORIENTED_EDGE('',*,*,#26012,.F.);
#35862=ORIENTED_EDGE('',*,*,#24711,.F.);
#35863=ORIENTED_EDGE('',*,*,#26014,.T.);
#35864=ORIENTED_EDGE('',*,*,#23595,.T.);
#35865=ORIENTED_EDGE('',*,*,#26013,.F.);
#35866=ORIENTED_EDGE('',*,*,#24710,.F.);
#35867=ORIENTED_EDGE('',*,*,#26010,.T.);
#35868=ORIENTED_EDGE('',*,*,#23596,.T.);
#35869=ORIENTED_EDGE('',*,*,#26014,.F.);
#35870=ORIENTED_EDGE('',*,*,#24709,.F.);
#35871=ORIENTED_EDGE('',*,*,#26015,.T.);
#35872=ORIENTED_EDGE('',*,*,#23585,.T.);
#35873=ORIENTED_EDGE('',*,*,#26016,.F.);
#35874=ORIENTED_EDGE('',*,*,#24702,.F.);
#35875=ORIENTED_EDGE('',*,*,#26017,.T.);
#35876=ORIENTED_EDGE('',*,*,#23586,.T.);
#35877=ORIENTED_EDGE('',*,*,#26015,.F.);
#35878=ORIENTED_EDGE('',*,*,#24701,.F.);
#35879=ORIENTED_EDGE('',*,*,#26018,.T.);
#35880=ORIENTED_EDGE('',*,*,#23587,.T.);
#35881=ORIENTED_EDGE('',*,*,#26017,.F.);
#35882=ORIENTED_EDGE('',*,*,#24706,.F.);
#35883=ORIENTED_EDGE('',*,*,#26019,.T.);
#35884=ORIENTED_EDGE('',*,*,#23588,.T.);
#35885=ORIENTED_EDGE('',*,*,#26018,.F.);
#35886=ORIENTED_EDGE('',*,*,#24705,.F.);
#35887=ORIENTED_EDGE('',*,*,#26020,.T.);
#35888=ORIENTED_EDGE('',*,*,#23589,.T.);
#35889=ORIENTED_EDGE('',*,*,#26019,.F.);
#35890=ORIENTED_EDGE('',*,*,#24704,.F.);
#35891=ORIENTED_EDGE('',*,*,#26016,.T.);
#35892=ORIENTED_EDGE('',*,*,#23590,.T.);
#35893=ORIENTED_EDGE('',*,*,#26020,.F.);
#35894=ORIENTED_EDGE('',*,*,#24703,.F.);
#35895=ORIENTED_EDGE('',*,*,#26021,.T.);
#35896=ORIENTED_EDGE('',*,*,#23579,.T.);
#35897=ORIENTED_EDGE('',*,*,#26022,.F.);
#35898=ORIENTED_EDGE('',*,*,#24696,.F.);
#35899=ORIENTED_EDGE('',*,*,#26023,.T.);
#35900=ORIENTED_EDGE('',*,*,#23580,.T.);
#35901=ORIENTED_EDGE('',*,*,#26021,.F.);
#35902=ORIENTED_EDGE('',*,*,#24695,.F.);
#35903=ORIENTED_EDGE('',*,*,#26024,.T.);
#35904=ORIENTED_EDGE('',*,*,#23581,.T.);
#35905=ORIENTED_EDGE('',*,*,#26023,.F.);
#35906=ORIENTED_EDGE('',*,*,#24700,.F.);
#35907=ORIENTED_EDGE('',*,*,#26025,.T.);
#35908=ORIENTED_EDGE('',*,*,#23582,.T.);
#35909=ORIENTED_EDGE('',*,*,#26024,.F.);
#35910=ORIENTED_EDGE('',*,*,#24699,.F.);
#35911=ORIENTED_EDGE('',*,*,#26026,.T.);
#35912=ORIENTED_EDGE('',*,*,#23583,.T.);
#35913=ORIENTED_EDGE('',*,*,#26025,.F.);
#35914=ORIENTED_EDGE('',*,*,#24698,.F.);
#35915=ORIENTED_EDGE('',*,*,#26022,.T.);
#35916=ORIENTED_EDGE('',*,*,#23584,.T.);
#35917=ORIENTED_EDGE('',*,*,#26026,.F.);
#35918=ORIENTED_EDGE('',*,*,#24697,.F.);
#35919=ORIENTED_EDGE('',*,*,#26027,.T.);
#35920=ORIENTED_EDGE('',*,*,#23573,.T.);
#35921=ORIENTED_EDGE('',*,*,#26028,.F.);
#35922=ORIENTED_EDGE('',*,*,#24690,.F.);
#35923=ORIENTED_EDGE('',*,*,#26029,.T.);
#35924=ORIENTED_EDGE('',*,*,#23574,.T.);
#35925=ORIENTED_EDGE('',*,*,#26027,.F.);
#35926=ORIENTED_EDGE('',*,*,#24689,.F.);
#35927=ORIENTED_EDGE('',*,*,#26030,.T.);
#35928=ORIENTED_EDGE('',*,*,#23575,.T.);
#35929=ORIENTED_EDGE('',*,*,#26029,.F.);
#35930=ORIENTED_EDGE('',*,*,#24694,.F.);
#35931=ORIENTED_EDGE('',*,*,#26031,.T.);
#35932=ORIENTED_EDGE('',*,*,#23576,.T.);
#35933=ORIENTED_EDGE('',*,*,#26030,.F.);
#35934=ORIENTED_EDGE('',*,*,#24693,.F.);
#35935=ORIENTED_EDGE('',*,*,#26032,.T.);
#35936=ORIENTED_EDGE('',*,*,#23577,.T.);
#35937=ORIENTED_EDGE('',*,*,#26031,.F.);
#35938=ORIENTED_EDGE('',*,*,#24692,.F.);
#35939=ORIENTED_EDGE('',*,*,#26028,.T.);
#35940=ORIENTED_EDGE('',*,*,#23578,.T.);
#35941=ORIENTED_EDGE('',*,*,#26032,.F.);
#35942=ORIENTED_EDGE('',*,*,#24691,.F.);
#35943=ORIENTED_EDGE('',*,*,#26033,.T.);
#35944=ORIENTED_EDGE('',*,*,#23567,.T.);
#35945=ORIENTED_EDGE('',*,*,#26034,.F.);
#35946=ORIENTED_EDGE('',*,*,#24684,.F.);
#35947=ORIENTED_EDGE('',*,*,#26035,.T.);
#35948=ORIENTED_EDGE('',*,*,#23568,.T.);
#35949=ORIENTED_EDGE('',*,*,#26033,.F.);
#35950=ORIENTED_EDGE('',*,*,#24683,.F.);
#35951=ORIENTED_EDGE('',*,*,#26036,.T.);
#35952=ORIENTED_EDGE('',*,*,#23569,.T.);
#35953=ORIENTED_EDGE('',*,*,#26035,.F.);
#35954=ORIENTED_EDGE('',*,*,#24688,.F.);
#35955=ORIENTED_EDGE('',*,*,#26037,.T.);
#35956=ORIENTED_EDGE('',*,*,#23570,.T.);
#35957=ORIENTED_EDGE('',*,*,#26036,.F.);
#35958=ORIENTED_EDGE('',*,*,#24687,.F.);
#35959=ORIENTED_EDGE('',*,*,#26038,.T.);
#35960=ORIENTED_EDGE('',*,*,#23571,.T.);
#35961=ORIENTED_EDGE('',*,*,#26037,.F.);
#35962=ORIENTED_EDGE('',*,*,#24686,.F.);
#35963=ORIENTED_EDGE('',*,*,#26034,.T.);
#35964=ORIENTED_EDGE('',*,*,#23572,.T.);
#35965=ORIENTED_EDGE('',*,*,#26038,.F.);
#35966=ORIENTED_EDGE('',*,*,#24685,.F.);
#35967=ORIENTED_EDGE('',*,*,#26039,.T.);
#35968=ORIENTED_EDGE('',*,*,#23561,.T.);
#35969=ORIENTED_EDGE('',*,*,#26040,.F.);
#35970=ORIENTED_EDGE('',*,*,#24678,.F.);
#35971=ORIENTED_EDGE('',*,*,#26041,.T.);
#35972=ORIENTED_EDGE('',*,*,#23562,.T.);
#35973=ORIENTED_EDGE('',*,*,#26039,.F.);
#35974=ORIENTED_EDGE('',*,*,#24677,.F.);
#35975=ORIENTED_EDGE('',*,*,#26042,.T.);
#35976=ORIENTED_EDGE('',*,*,#23563,.T.);
#35977=ORIENTED_EDGE('',*,*,#26041,.F.);
#35978=ORIENTED_EDGE('',*,*,#24682,.F.);
#35979=ORIENTED_EDGE('',*,*,#26043,.T.);
#35980=ORIENTED_EDGE('',*,*,#23564,.T.);
#35981=ORIENTED_EDGE('',*,*,#26042,.F.);
#35982=ORIENTED_EDGE('',*,*,#24681,.F.);
#35983=ORIENTED_EDGE('',*,*,#26044,.T.);
#35984=ORIENTED_EDGE('',*,*,#23565,.T.);
#35985=ORIENTED_EDGE('',*,*,#26043,.F.);
#35986=ORIENTED_EDGE('',*,*,#24680,.F.);
#35987=ORIENTED_EDGE('',*,*,#26040,.T.);
#35988=ORIENTED_EDGE('',*,*,#23566,.T.);
#35989=ORIENTED_EDGE('',*,*,#26044,.F.);
#35990=ORIENTED_EDGE('',*,*,#24679,.F.);
#35991=ORIENTED_EDGE('',*,*,#26045,.T.);
#35992=ORIENTED_EDGE('',*,*,#23555,.T.);
#35993=ORIENTED_EDGE('',*,*,#26046,.F.);
#35994=ORIENTED_EDGE('',*,*,#24672,.F.);
#35995=ORIENTED_EDGE('',*,*,#26047,.T.);
#35996=ORIENTED_EDGE('',*,*,#23556,.T.);
#35997=ORIENTED_EDGE('',*,*,#26045,.F.);
#35998=ORIENTED_EDGE('',*,*,#24671,.F.);
#35999=ORIENTED_EDGE('',*,*,#26048,.T.);
#36000=ORIENTED_EDGE('',*,*,#23557,.T.);
#36001=ORIENTED_EDGE('',*,*,#26047,.F.);
#36002=ORIENTED_EDGE('',*,*,#24676,.F.);
#36003=ORIENTED_EDGE('',*,*,#26049,.T.);
#36004=ORIENTED_EDGE('',*,*,#23558,.T.);
#36005=ORIENTED_EDGE('',*,*,#26048,.F.);
#36006=ORIENTED_EDGE('',*,*,#24675,.F.);
#36007=ORIENTED_EDGE('',*,*,#26050,.T.);
#36008=ORIENTED_EDGE('',*,*,#23559,.T.);
#36009=ORIENTED_EDGE('',*,*,#26049,.F.);
#36010=ORIENTED_EDGE('',*,*,#24674,.F.);
#36011=ORIENTED_EDGE('',*,*,#26046,.T.);
#36012=ORIENTED_EDGE('',*,*,#23560,.T.);
#36013=ORIENTED_EDGE('',*,*,#26050,.F.);
#36014=ORIENTED_EDGE('',*,*,#24673,.F.);
#36015=ORIENTED_EDGE('',*,*,#26051,.T.);
#36016=ORIENTED_EDGE('',*,*,#23549,.T.);
#36017=ORIENTED_EDGE('',*,*,#26052,.F.);
#36018=ORIENTED_EDGE('',*,*,#24666,.F.);
#36019=ORIENTED_EDGE('',*,*,#26053,.T.);
#36020=ORIENTED_EDGE('',*,*,#23550,.T.);
#36021=ORIENTED_EDGE('',*,*,#26051,.F.);
#36022=ORIENTED_EDGE('',*,*,#24665,.F.);
#36023=ORIENTED_EDGE('',*,*,#26054,.T.);
#36024=ORIENTED_EDGE('',*,*,#23551,.T.);
#36025=ORIENTED_EDGE('',*,*,#26053,.F.);
#36026=ORIENTED_EDGE('',*,*,#24670,.F.);
#36027=ORIENTED_EDGE('',*,*,#26055,.T.);
#36028=ORIENTED_EDGE('',*,*,#23552,.T.);
#36029=ORIENTED_EDGE('',*,*,#26054,.F.);
#36030=ORIENTED_EDGE('',*,*,#24669,.F.);
#36031=ORIENTED_EDGE('',*,*,#26056,.T.);
#36032=ORIENTED_EDGE('',*,*,#23553,.T.);
#36033=ORIENTED_EDGE('',*,*,#26055,.F.);
#36034=ORIENTED_EDGE('',*,*,#24668,.F.);
#36035=ORIENTED_EDGE('',*,*,#26052,.T.);
#36036=ORIENTED_EDGE('',*,*,#23554,.T.);
#36037=ORIENTED_EDGE('',*,*,#26056,.F.);
#36038=ORIENTED_EDGE('',*,*,#24667,.F.);
#36039=ORIENTED_EDGE('',*,*,#26057,.T.);
#36040=ORIENTED_EDGE('',*,*,#23543,.T.);
#36041=ORIENTED_EDGE('',*,*,#26058,.F.);
#36042=ORIENTED_EDGE('',*,*,#24660,.F.);
#36043=ORIENTED_EDGE('',*,*,#26059,.T.);
#36044=ORIENTED_EDGE('',*,*,#23544,.T.);
#36045=ORIENTED_EDGE('',*,*,#26057,.F.);
#36046=ORIENTED_EDGE('',*,*,#24659,.F.);
#36047=ORIENTED_EDGE('',*,*,#26060,.T.);
#36048=ORIENTED_EDGE('',*,*,#23545,.T.);
#36049=ORIENTED_EDGE('',*,*,#26059,.F.);
#36050=ORIENTED_EDGE('',*,*,#24664,.F.);
#36051=ORIENTED_EDGE('',*,*,#26061,.T.);
#36052=ORIENTED_EDGE('',*,*,#23546,.T.);
#36053=ORIENTED_EDGE('',*,*,#26060,.F.);
#36054=ORIENTED_EDGE('',*,*,#24663,.F.);
#36055=ORIENTED_EDGE('',*,*,#26062,.T.);
#36056=ORIENTED_EDGE('',*,*,#23547,.T.);
#36057=ORIENTED_EDGE('',*,*,#26061,.F.);
#36058=ORIENTED_EDGE('',*,*,#24662,.F.);
#36059=ORIENTED_EDGE('',*,*,#26058,.T.);
#36060=ORIENTED_EDGE('',*,*,#23548,.T.);
#36061=ORIENTED_EDGE('',*,*,#26062,.F.);
#36062=ORIENTED_EDGE('',*,*,#24661,.F.);
#36063=ORIENTED_EDGE('',*,*,#26063,.T.);
#36064=ORIENTED_EDGE('',*,*,#23537,.T.);
#36065=ORIENTED_EDGE('',*,*,#26064,.F.);
#36066=ORIENTED_EDGE('',*,*,#24654,.F.);
#36067=ORIENTED_EDGE('',*,*,#26065,.T.);
#36068=ORIENTED_EDGE('',*,*,#23538,.T.);
#36069=ORIENTED_EDGE('',*,*,#26063,.F.);
#36070=ORIENTED_EDGE('',*,*,#24653,.F.);
#36071=ORIENTED_EDGE('',*,*,#26066,.T.);
#36072=ORIENTED_EDGE('',*,*,#23539,.T.);
#36073=ORIENTED_EDGE('',*,*,#26065,.F.);
#36074=ORIENTED_EDGE('',*,*,#24658,.F.);
#36075=ORIENTED_EDGE('',*,*,#26067,.T.);
#36076=ORIENTED_EDGE('',*,*,#23540,.T.);
#36077=ORIENTED_EDGE('',*,*,#26066,.F.);
#36078=ORIENTED_EDGE('',*,*,#24657,.F.);
#36079=ORIENTED_EDGE('',*,*,#26068,.T.);
#36080=ORIENTED_EDGE('',*,*,#23541,.T.);
#36081=ORIENTED_EDGE('',*,*,#26067,.F.);
#36082=ORIENTED_EDGE('',*,*,#24656,.F.);
#36083=ORIENTED_EDGE('',*,*,#26064,.T.);
#36084=ORIENTED_EDGE('',*,*,#23542,.T.);
#36085=ORIENTED_EDGE('',*,*,#26068,.F.);
#36086=ORIENTED_EDGE('',*,*,#24655,.F.);
#36087=ORIENTED_EDGE('',*,*,#26069,.T.);
#36088=ORIENTED_EDGE('',*,*,#23531,.T.);
#36089=ORIENTED_EDGE('',*,*,#26070,.F.);
#36090=ORIENTED_EDGE('',*,*,#24648,.F.);
#36091=ORIENTED_EDGE('',*,*,#26071,.T.);
#36092=ORIENTED_EDGE('',*,*,#23532,.T.);
#36093=ORIENTED_EDGE('',*,*,#26069,.F.);
#36094=ORIENTED_EDGE('',*,*,#24647,.F.);
#36095=ORIENTED_EDGE('',*,*,#26072,.T.);
#36096=ORIENTED_EDGE('',*,*,#23533,.T.);
#36097=ORIENTED_EDGE('',*,*,#26071,.F.);
#36098=ORIENTED_EDGE('',*,*,#24652,.F.);
#36099=ORIENTED_EDGE('',*,*,#26073,.T.);
#36100=ORIENTED_EDGE('',*,*,#23534,.T.);
#36101=ORIENTED_EDGE('',*,*,#26072,.F.);
#36102=ORIENTED_EDGE('',*,*,#24651,.F.);
#36103=ORIENTED_EDGE('',*,*,#26074,.T.);
#36104=ORIENTED_EDGE('',*,*,#23535,.T.);
#36105=ORIENTED_EDGE('',*,*,#26073,.F.);
#36106=ORIENTED_EDGE('',*,*,#24650,.F.);
#36107=ORIENTED_EDGE('',*,*,#26070,.T.);
#36108=ORIENTED_EDGE('',*,*,#23536,.T.);
#36109=ORIENTED_EDGE('',*,*,#26074,.F.);
#36110=ORIENTED_EDGE('',*,*,#24649,.F.);
#36111=ORIENTED_EDGE('',*,*,#26075,.T.);
#36112=ORIENTED_EDGE('',*,*,#23525,.T.);
#36113=ORIENTED_EDGE('',*,*,#26076,.F.);
#36114=ORIENTED_EDGE('',*,*,#24642,.F.);
#36115=ORIENTED_EDGE('',*,*,#26077,.T.);
#36116=ORIENTED_EDGE('',*,*,#23526,.T.);
#36117=ORIENTED_EDGE('',*,*,#26075,.F.);
#36118=ORIENTED_EDGE('',*,*,#24641,.F.);
#36119=ORIENTED_EDGE('',*,*,#26078,.T.);
#36120=ORIENTED_EDGE('',*,*,#23527,.T.);
#36121=ORIENTED_EDGE('',*,*,#26077,.F.);
#36122=ORIENTED_EDGE('',*,*,#24646,.F.);
#36123=ORIENTED_EDGE('',*,*,#26079,.T.);
#36124=ORIENTED_EDGE('',*,*,#23528,.T.);
#36125=ORIENTED_EDGE('',*,*,#26078,.F.);
#36126=ORIENTED_EDGE('',*,*,#24645,.F.);
#36127=ORIENTED_EDGE('',*,*,#26080,.T.);
#36128=ORIENTED_EDGE('',*,*,#23529,.T.);
#36129=ORIENTED_EDGE('',*,*,#26079,.F.);
#36130=ORIENTED_EDGE('',*,*,#24644,.F.);
#36131=ORIENTED_EDGE('',*,*,#26076,.T.);
#36132=ORIENTED_EDGE('',*,*,#23530,.T.);
#36133=ORIENTED_EDGE('',*,*,#26080,.F.);
#36134=ORIENTED_EDGE('',*,*,#24643,.F.);
#36135=ORIENTED_EDGE('',*,*,#26081,.T.);
#36136=ORIENTED_EDGE('',*,*,#23519,.T.);
#36137=ORIENTED_EDGE('',*,*,#26082,.F.);
#36138=ORIENTED_EDGE('',*,*,#24636,.F.);
#36139=ORIENTED_EDGE('',*,*,#26083,.T.);
#36140=ORIENTED_EDGE('',*,*,#23520,.T.);
#36141=ORIENTED_EDGE('',*,*,#26081,.F.);
#36142=ORIENTED_EDGE('',*,*,#24635,.F.);
#36143=ORIENTED_EDGE('',*,*,#26084,.T.);
#36144=ORIENTED_EDGE('',*,*,#23521,.T.);
#36145=ORIENTED_EDGE('',*,*,#26083,.F.);
#36146=ORIENTED_EDGE('',*,*,#24640,.F.);
#36147=ORIENTED_EDGE('',*,*,#26085,.T.);
#36148=ORIENTED_EDGE('',*,*,#23522,.T.);
#36149=ORIENTED_EDGE('',*,*,#26084,.F.);
#36150=ORIENTED_EDGE('',*,*,#24639,.F.);
#36151=ORIENTED_EDGE('',*,*,#26086,.T.);
#36152=ORIENTED_EDGE('',*,*,#23523,.T.);
#36153=ORIENTED_EDGE('',*,*,#26085,.F.);
#36154=ORIENTED_EDGE('',*,*,#24638,.F.);
#36155=ORIENTED_EDGE('',*,*,#26082,.T.);
#36156=ORIENTED_EDGE('',*,*,#23524,.T.);
#36157=ORIENTED_EDGE('',*,*,#26086,.F.);
#36158=ORIENTED_EDGE('',*,*,#24637,.F.);
#36159=ORIENTED_EDGE('',*,*,#26087,.T.);
#36160=ORIENTED_EDGE('',*,*,#23513,.T.);
#36161=ORIENTED_EDGE('',*,*,#26088,.F.);
#36162=ORIENTED_EDGE('',*,*,#24630,.F.);
#36163=ORIENTED_EDGE('',*,*,#26089,.T.);
#36164=ORIENTED_EDGE('',*,*,#23514,.T.);
#36165=ORIENTED_EDGE('',*,*,#26087,.F.);
#36166=ORIENTED_EDGE('',*,*,#24629,.F.);
#36167=ORIENTED_EDGE('',*,*,#26090,.T.);
#36168=ORIENTED_EDGE('',*,*,#23515,.T.);
#36169=ORIENTED_EDGE('',*,*,#26089,.F.);
#36170=ORIENTED_EDGE('',*,*,#24634,.F.);
#36171=ORIENTED_EDGE('',*,*,#26091,.T.);
#36172=ORIENTED_EDGE('',*,*,#23516,.T.);
#36173=ORIENTED_EDGE('',*,*,#26090,.F.);
#36174=ORIENTED_EDGE('',*,*,#24633,.F.);
#36175=ORIENTED_EDGE('',*,*,#26092,.T.);
#36176=ORIENTED_EDGE('',*,*,#23517,.T.);
#36177=ORIENTED_EDGE('',*,*,#26091,.F.);
#36178=ORIENTED_EDGE('',*,*,#24632,.F.);
#36179=ORIENTED_EDGE('',*,*,#26088,.T.);
#36180=ORIENTED_EDGE('',*,*,#23518,.T.);
#36181=ORIENTED_EDGE('',*,*,#26092,.F.);
#36182=ORIENTED_EDGE('',*,*,#24631,.F.);
#36183=ORIENTED_EDGE('',*,*,#26093,.T.);
#36184=ORIENTED_EDGE('',*,*,#23507,.T.);
#36185=ORIENTED_EDGE('',*,*,#26094,.F.);
#36186=ORIENTED_EDGE('',*,*,#24624,.F.);
#36187=ORIENTED_EDGE('',*,*,#26095,.T.);
#36188=ORIENTED_EDGE('',*,*,#23508,.T.);
#36189=ORIENTED_EDGE('',*,*,#26093,.F.);
#36190=ORIENTED_EDGE('',*,*,#24623,.F.);
#36191=ORIENTED_EDGE('',*,*,#26096,.T.);
#36192=ORIENTED_EDGE('',*,*,#23509,.T.);
#36193=ORIENTED_EDGE('',*,*,#26095,.F.);
#36194=ORIENTED_EDGE('',*,*,#24628,.F.);
#36195=ORIENTED_EDGE('',*,*,#26097,.T.);
#36196=ORIENTED_EDGE('',*,*,#23510,.T.);
#36197=ORIENTED_EDGE('',*,*,#26096,.F.);
#36198=ORIENTED_EDGE('',*,*,#24627,.F.);
#36199=ORIENTED_EDGE('',*,*,#26098,.T.);
#36200=ORIENTED_EDGE('',*,*,#23511,.T.);
#36201=ORIENTED_EDGE('',*,*,#26097,.F.);
#36202=ORIENTED_EDGE('',*,*,#24626,.F.);
#36203=ORIENTED_EDGE('',*,*,#26094,.T.);
#36204=ORIENTED_EDGE('',*,*,#23512,.T.);
#36205=ORIENTED_EDGE('',*,*,#26098,.F.);
#36206=ORIENTED_EDGE('',*,*,#24625,.F.);
#36207=ORIENTED_EDGE('',*,*,#26099,.T.);
#36208=ORIENTED_EDGE('',*,*,#23501,.T.);
#36209=ORIENTED_EDGE('',*,*,#26100,.F.);
#36210=ORIENTED_EDGE('',*,*,#24618,.F.);
#36211=ORIENTED_EDGE('',*,*,#26101,.T.);
#36212=ORIENTED_EDGE('',*,*,#23502,.T.);
#36213=ORIENTED_EDGE('',*,*,#26099,.F.);
#36214=ORIENTED_EDGE('',*,*,#24617,.F.);
#36215=ORIENTED_EDGE('',*,*,#26102,.T.);
#36216=ORIENTED_EDGE('',*,*,#23503,.T.);
#36217=ORIENTED_EDGE('',*,*,#26101,.F.);
#36218=ORIENTED_EDGE('',*,*,#24622,.F.);
#36219=ORIENTED_EDGE('',*,*,#26103,.T.);
#36220=ORIENTED_EDGE('',*,*,#23504,.T.);
#36221=ORIENTED_EDGE('',*,*,#26102,.F.);
#36222=ORIENTED_EDGE('',*,*,#24621,.F.);
#36223=ORIENTED_EDGE('',*,*,#26104,.T.);
#36224=ORIENTED_EDGE('',*,*,#23505,.T.);
#36225=ORIENTED_EDGE('',*,*,#26103,.F.);
#36226=ORIENTED_EDGE('',*,*,#24620,.F.);
#36227=ORIENTED_EDGE('',*,*,#26100,.T.);
#36228=ORIENTED_EDGE('',*,*,#23506,.T.);
#36229=ORIENTED_EDGE('',*,*,#26104,.F.);
#36230=ORIENTED_EDGE('',*,*,#24619,.F.);
#36231=ORIENTED_EDGE('',*,*,#26105,.T.);
#36232=ORIENTED_EDGE('',*,*,#23495,.T.);
#36233=ORIENTED_EDGE('',*,*,#26106,.F.);
#36234=ORIENTED_EDGE('',*,*,#24612,.F.);
#36235=ORIENTED_EDGE('',*,*,#26107,.T.);
#36236=ORIENTED_EDGE('',*,*,#23496,.T.);
#36237=ORIENTED_EDGE('',*,*,#26105,.F.);
#36238=ORIENTED_EDGE('',*,*,#24611,.F.);
#36239=ORIENTED_EDGE('',*,*,#26108,.T.);
#36240=ORIENTED_EDGE('',*,*,#23497,.T.);
#36241=ORIENTED_EDGE('',*,*,#26107,.F.);
#36242=ORIENTED_EDGE('',*,*,#24616,.F.);
#36243=ORIENTED_EDGE('',*,*,#26109,.T.);
#36244=ORIENTED_EDGE('',*,*,#23498,.T.);
#36245=ORIENTED_EDGE('',*,*,#26108,.F.);
#36246=ORIENTED_EDGE('',*,*,#24615,.F.);
#36247=ORIENTED_EDGE('',*,*,#26110,.T.);
#36248=ORIENTED_EDGE('',*,*,#23499,.T.);
#36249=ORIENTED_EDGE('',*,*,#26109,.F.);
#36250=ORIENTED_EDGE('',*,*,#24614,.F.);
#36251=ORIENTED_EDGE('',*,*,#26106,.T.);
#36252=ORIENTED_EDGE('',*,*,#23500,.T.);
#36253=ORIENTED_EDGE('',*,*,#26110,.F.);
#36254=ORIENTED_EDGE('',*,*,#24613,.F.);
#36255=ORIENTED_EDGE('',*,*,#26111,.T.);
#36256=ORIENTED_EDGE('',*,*,#23489,.T.);
#36257=ORIENTED_EDGE('',*,*,#26112,.F.);
#36258=ORIENTED_EDGE('',*,*,#24606,.F.);
#36259=ORIENTED_EDGE('',*,*,#26113,.T.);
#36260=ORIENTED_EDGE('',*,*,#23490,.T.);
#36261=ORIENTED_EDGE('',*,*,#26111,.F.);
#36262=ORIENTED_EDGE('',*,*,#24605,.F.);
#36263=ORIENTED_EDGE('',*,*,#26114,.T.);
#36264=ORIENTED_EDGE('',*,*,#23491,.T.);
#36265=ORIENTED_EDGE('',*,*,#26113,.F.);
#36266=ORIENTED_EDGE('',*,*,#24610,.F.);
#36267=ORIENTED_EDGE('',*,*,#26115,.T.);
#36268=ORIENTED_EDGE('',*,*,#23492,.T.);
#36269=ORIENTED_EDGE('',*,*,#26114,.F.);
#36270=ORIENTED_EDGE('',*,*,#24609,.F.);
#36271=ORIENTED_EDGE('',*,*,#26116,.T.);
#36272=ORIENTED_EDGE('',*,*,#23493,.T.);
#36273=ORIENTED_EDGE('',*,*,#26115,.F.);
#36274=ORIENTED_EDGE('',*,*,#24608,.F.);
#36275=ORIENTED_EDGE('',*,*,#26112,.T.);
#36276=ORIENTED_EDGE('',*,*,#23494,.T.);
#36277=ORIENTED_EDGE('',*,*,#26116,.F.);
#36278=ORIENTED_EDGE('',*,*,#24607,.F.);
#36279=ORIENTED_EDGE('',*,*,#26117,.T.);
#36280=ORIENTED_EDGE('',*,*,#23483,.T.);
#36281=ORIENTED_EDGE('',*,*,#26118,.F.);
#36282=ORIENTED_EDGE('',*,*,#24600,.F.);
#36283=ORIENTED_EDGE('',*,*,#26119,.T.);
#36284=ORIENTED_EDGE('',*,*,#23484,.T.);
#36285=ORIENTED_EDGE('',*,*,#26117,.F.);
#36286=ORIENTED_EDGE('',*,*,#24599,.F.);
#36287=ORIENTED_EDGE('',*,*,#26120,.T.);
#36288=ORIENTED_EDGE('',*,*,#23485,.T.);
#36289=ORIENTED_EDGE('',*,*,#26119,.F.);
#36290=ORIENTED_EDGE('',*,*,#24604,.F.);
#36291=ORIENTED_EDGE('',*,*,#26121,.T.);
#36292=ORIENTED_EDGE('',*,*,#23486,.T.);
#36293=ORIENTED_EDGE('',*,*,#26120,.F.);
#36294=ORIENTED_EDGE('',*,*,#24603,.F.);
#36295=ORIENTED_EDGE('',*,*,#26122,.T.);
#36296=ORIENTED_EDGE('',*,*,#23487,.T.);
#36297=ORIENTED_EDGE('',*,*,#26121,.F.);
#36298=ORIENTED_EDGE('',*,*,#24602,.F.);
#36299=ORIENTED_EDGE('',*,*,#26118,.T.);
#36300=ORIENTED_EDGE('',*,*,#23488,.T.);
#36301=ORIENTED_EDGE('',*,*,#26122,.F.);
#36302=ORIENTED_EDGE('',*,*,#24601,.F.);
#36303=ORIENTED_EDGE('',*,*,#26123,.T.);
#36304=ORIENTED_EDGE('',*,*,#23477,.T.);
#36305=ORIENTED_EDGE('',*,*,#26124,.F.);
#36306=ORIENTED_EDGE('',*,*,#24594,.F.);
#36307=ORIENTED_EDGE('',*,*,#26125,.T.);
#36308=ORIENTED_EDGE('',*,*,#23478,.T.);
#36309=ORIENTED_EDGE('',*,*,#26123,.F.);
#36310=ORIENTED_EDGE('',*,*,#24593,.F.);
#36311=ORIENTED_EDGE('',*,*,#26126,.T.);
#36312=ORIENTED_EDGE('',*,*,#23479,.T.);
#36313=ORIENTED_EDGE('',*,*,#26125,.F.);
#36314=ORIENTED_EDGE('',*,*,#24598,.F.);
#36315=ORIENTED_EDGE('',*,*,#26127,.T.);
#36316=ORIENTED_EDGE('',*,*,#23480,.T.);
#36317=ORIENTED_EDGE('',*,*,#26126,.F.);
#36318=ORIENTED_EDGE('',*,*,#24597,.F.);
#36319=ORIENTED_EDGE('',*,*,#26128,.T.);
#36320=ORIENTED_EDGE('',*,*,#23481,.T.);
#36321=ORIENTED_EDGE('',*,*,#26127,.F.);
#36322=ORIENTED_EDGE('',*,*,#24596,.F.);
#36323=ORIENTED_EDGE('',*,*,#26124,.T.);
#36324=ORIENTED_EDGE('',*,*,#23482,.T.);
#36325=ORIENTED_EDGE('',*,*,#26128,.F.);
#36326=ORIENTED_EDGE('',*,*,#24595,.F.);
#36327=ORIENTED_EDGE('',*,*,#26129,.T.);
#36328=ORIENTED_EDGE('',*,*,#23471,.T.);
#36329=ORIENTED_EDGE('',*,*,#26130,.F.);
#36330=ORIENTED_EDGE('',*,*,#24588,.F.);
#36331=ORIENTED_EDGE('',*,*,#26131,.T.);
#36332=ORIENTED_EDGE('',*,*,#23472,.T.);
#36333=ORIENTED_EDGE('',*,*,#26129,.F.);
#36334=ORIENTED_EDGE('',*,*,#24587,.F.);
#36335=ORIENTED_EDGE('',*,*,#26132,.T.);
#36336=ORIENTED_EDGE('',*,*,#23473,.T.);
#36337=ORIENTED_EDGE('',*,*,#26131,.F.);
#36338=ORIENTED_EDGE('',*,*,#24592,.F.);
#36339=ORIENTED_EDGE('',*,*,#26133,.T.);
#36340=ORIENTED_EDGE('',*,*,#23474,.T.);
#36341=ORIENTED_EDGE('',*,*,#26132,.F.);
#36342=ORIENTED_EDGE('',*,*,#24591,.F.);
#36343=ORIENTED_EDGE('',*,*,#26134,.T.);
#36344=ORIENTED_EDGE('',*,*,#23475,.T.);
#36345=ORIENTED_EDGE('',*,*,#26133,.F.);
#36346=ORIENTED_EDGE('',*,*,#24590,.F.);
#36347=ORIENTED_EDGE('',*,*,#26130,.T.);
#36348=ORIENTED_EDGE('',*,*,#23476,.T.);
#36349=ORIENTED_EDGE('',*,*,#26134,.F.);
#36350=ORIENTED_EDGE('',*,*,#24589,.F.);
#36351=ORIENTED_EDGE('',*,*,#26135,.T.);
#36352=ORIENTED_EDGE('',*,*,#23465,.T.);
#36353=ORIENTED_EDGE('',*,*,#26136,.F.);
#36354=ORIENTED_EDGE('',*,*,#24582,.F.);
#36355=ORIENTED_EDGE('',*,*,#26137,.T.);
#36356=ORIENTED_EDGE('',*,*,#23466,.T.);
#36357=ORIENTED_EDGE('',*,*,#26135,.F.);
#36358=ORIENTED_EDGE('',*,*,#24581,.F.);
#36359=ORIENTED_EDGE('',*,*,#26138,.T.);
#36360=ORIENTED_EDGE('',*,*,#23467,.T.);
#36361=ORIENTED_EDGE('',*,*,#26137,.F.);
#36362=ORIENTED_EDGE('',*,*,#24586,.F.);
#36363=ORIENTED_EDGE('',*,*,#26139,.T.);
#36364=ORIENTED_EDGE('',*,*,#23468,.T.);
#36365=ORIENTED_EDGE('',*,*,#26138,.F.);
#36366=ORIENTED_EDGE('',*,*,#24585,.F.);
#36367=ORIENTED_EDGE('',*,*,#26140,.T.);
#36368=ORIENTED_EDGE('',*,*,#23469,.T.);
#36369=ORIENTED_EDGE('',*,*,#26139,.F.);
#36370=ORIENTED_EDGE('',*,*,#24584,.F.);
#36371=ORIENTED_EDGE('',*,*,#26136,.T.);
#36372=ORIENTED_EDGE('',*,*,#23470,.T.);
#36373=ORIENTED_EDGE('',*,*,#26140,.F.);
#36374=ORIENTED_EDGE('',*,*,#24583,.F.);
#36375=ORIENTED_EDGE('',*,*,#26141,.T.);
#36376=ORIENTED_EDGE('',*,*,#23459,.T.);
#36377=ORIENTED_EDGE('',*,*,#26142,.F.);
#36378=ORIENTED_EDGE('',*,*,#24576,.F.);
#36379=ORIENTED_EDGE('',*,*,#26143,.T.);
#36380=ORIENTED_EDGE('',*,*,#23460,.T.);
#36381=ORIENTED_EDGE('',*,*,#26141,.F.);
#36382=ORIENTED_EDGE('',*,*,#24575,.F.);
#36383=ORIENTED_EDGE('',*,*,#26144,.T.);
#36384=ORIENTED_EDGE('',*,*,#23461,.T.);
#36385=ORIENTED_EDGE('',*,*,#26143,.F.);
#36386=ORIENTED_EDGE('',*,*,#24580,.F.);
#36387=ORIENTED_EDGE('',*,*,#26145,.T.);
#36388=ORIENTED_EDGE('',*,*,#23462,.T.);
#36389=ORIENTED_EDGE('',*,*,#26144,.F.);
#36390=ORIENTED_EDGE('',*,*,#24579,.F.);
#36391=ORIENTED_EDGE('',*,*,#26146,.T.);
#36392=ORIENTED_EDGE('',*,*,#23463,.T.);
#36393=ORIENTED_EDGE('',*,*,#26145,.F.);
#36394=ORIENTED_EDGE('',*,*,#24578,.F.);
#36395=ORIENTED_EDGE('',*,*,#26142,.T.);
#36396=ORIENTED_EDGE('',*,*,#23464,.T.);
#36397=ORIENTED_EDGE('',*,*,#26146,.F.);
#36398=ORIENTED_EDGE('',*,*,#24577,.F.);
#36399=ORIENTED_EDGE('',*,*,#26147,.T.);
#36400=ORIENTED_EDGE('',*,*,#23453,.T.);
#36401=ORIENTED_EDGE('',*,*,#26148,.F.);
#36402=ORIENTED_EDGE('',*,*,#24570,.F.);
#36403=ORIENTED_EDGE('',*,*,#26149,.T.);
#36404=ORIENTED_EDGE('',*,*,#23454,.T.);
#36405=ORIENTED_EDGE('',*,*,#26147,.F.);
#36406=ORIENTED_EDGE('',*,*,#24569,.F.);
#36407=ORIENTED_EDGE('',*,*,#26150,.T.);
#36408=ORIENTED_EDGE('',*,*,#23455,.T.);
#36409=ORIENTED_EDGE('',*,*,#26149,.F.);
#36410=ORIENTED_EDGE('',*,*,#24574,.F.);
#36411=ORIENTED_EDGE('',*,*,#26151,.T.);
#36412=ORIENTED_EDGE('',*,*,#23456,.T.);
#36413=ORIENTED_EDGE('',*,*,#26150,.F.);
#36414=ORIENTED_EDGE('',*,*,#24573,.F.);
#36415=ORIENTED_EDGE('',*,*,#26152,.T.);
#36416=ORIENTED_EDGE('',*,*,#23457,.T.);
#36417=ORIENTED_EDGE('',*,*,#26151,.F.);
#36418=ORIENTED_EDGE('',*,*,#24572,.F.);
#36419=ORIENTED_EDGE('',*,*,#26148,.T.);
#36420=ORIENTED_EDGE('',*,*,#23458,.T.);
#36421=ORIENTED_EDGE('',*,*,#26152,.F.);
#36422=ORIENTED_EDGE('',*,*,#24571,.F.);
#36423=ORIENTED_EDGE('',*,*,#26153,.T.);
#36424=ORIENTED_EDGE('',*,*,#23447,.T.);
#36425=ORIENTED_EDGE('',*,*,#26154,.F.);
#36426=ORIENTED_EDGE('',*,*,#24564,.F.);
#36427=ORIENTED_EDGE('',*,*,#26155,.T.);
#36428=ORIENTED_EDGE('',*,*,#23448,.T.);
#36429=ORIENTED_EDGE('',*,*,#26153,.F.);
#36430=ORIENTED_EDGE('',*,*,#24563,.F.);
#36431=ORIENTED_EDGE('',*,*,#26156,.T.);
#36432=ORIENTED_EDGE('',*,*,#23449,.T.);
#36433=ORIENTED_EDGE('',*,*,#26155,.F.);
#36434=ORIENTED_EDGE('',*,*,#24568,.F.);
#36435=ORIENTED_EDGE('',*,*,#26157,.T.);
#36436=ORIENTED_EDGE('',*,*,#23450,.T.);
#36437=ORIENTED_EDGE('',*,*,#26156,.F.);
#36438=ORIENTED_EDGE('',*,*,#24567,.F.);
#36439=ORIENTED_EDGE('',*,*,#26158,.T.);
#36440=ORIENTED_EDGE('',*,*,#23451,.T.);
#36441=ORIENTED_EDGE('',*,*,#26157,.F.);
#36442=ORIENTED_EDGE('',*,*,#24566,.F.);
#36443=ORIENTED_EDGE('',*,*,#26154,.T.);
#36444=ORIENTED_EDGE('',*,*,#23452,.T.);
#36445=ORIENTED_EDGE('',*,*,#26158,.F.);
#36446=ORIENTED_EDGE('',*,*,#24565,.F.);
#36447=ORIENTED_EDGE('',*,*,#26159,.T.);
#36448=ORIENTED_EDGE('',*,*,#23441,.T.);
#36449=ORIENTED_EDGE('',*,*,#26160,.F.);
#36450=ORIENTED_EDGE('',*,*,#24558,.F.);
#36451=ORIENTED_EDGE('',*,*,#26161,.T.);
#36452=ORIENTED_EDGE('',*,*,#23442,.T.);
#36453=ORIENTED_EDGE('',*,*,#26159,.F.);
#36454=ORIENTED_EDGE('',*,*,#24557,.F.);
#36455=ORIENTED_EDGE('',*,*,#26162,.T.);
#36456=ORIENTED_EDGE('',*,*,#23443,.T.);
#36457=ORIENTED_EDGE('',*,*,#26161,.F.);
#36458=ORIENTED_EDGE('',*,*,#24562,.F.);
#36459=ORIENTED_EDGE('',*,*,#26163,.T.);
#36460=ORIENTED_EDGE('',*,*,#23444,.T.);
#36461=ORIENTED_EDGE('',*,*,#26162,.F.);
#36462=ORIENTED_EDGE('',*,*,#24561,.F.);
#36463=ORIENTED_EDGE('',*,*,#26164,.T.);
#36464=ORIENTED_EDGE('',*,*,#23445,.T.);
#36465=ORIENTED_EDGE('',*,*,#26163,.F.);
#36466=ORIENTED_EDGE('',*,*,#24560,.F.);
#36467=ORIENTED_EDGE('',*,*,#26160,.T.);
#36468=ORIENTED_EDGE('',*,*,#23446,.T.);
#36469=ORIENTED_EDGE('',*,*,#26164,.F.);
#36470=ORIENTED_EDGE('',*,*,#24559,.F.);
#36471=ORIENTED_EDGE('',*,*,#26165,.T.);
#36472=ORIENTED_EDGE('',*,*,#23435,.T.);
#36473=ORIENTED_EDGE('',*,*,#26166,.F.);
#36474=ORIENTED_EDGE('',*,*,#24552,.F.);
#36475=ORIENTED_EDGE('',*,*,#26167,.T.);
#36476=ORIENTED_EDGE('',*,*,#23436,.T.);
#36477=ORIENTED_EDGE('',*,*,#26165,.F.);
#36478=ORIENTED_EDGE('',*,*,#24551,.F.);
#36479=ORIENTED_EDGE('',*,*,#26168,.T.);
#36480=ORIENTED_EDGE('',*,*,#23437,.T.);
#36481=ORIENTED_EDGE('',*,*,#26167,.F.);
#36482=ORIENTED_EDGE('',*,*,#24556,.F.);
#36483=ORIENTED_EDGE('',*,*,#26169,.T.);
#36484=ORIENTED_EDGE('',*,*,#23438,.T.);
#36485=ORIENTED_EDGE('',*,*,#26168,.F.);
#36486=ORIENTED_EDGE('',*,*,#24555,.F.);
#36487=ORIENTED_EDGE('',*,*,#26170,.T.);
#36488=ORIENTED_EDGE('',*,*,#23439,.T.);
#36489=ORIENTED_EDGE('',*,*,#26169,.F.);
#36490=ORIENTED_EDGE('',*,*,#24554,.F.);
#36491=ORIENTED_EDGE('',*,*,#26166,.T.);
#36492=ORIENTED_EDGE('',*,*,#23440,.T.);
#36493=ORIENTED_EDGE('',*,*,#26170,.F.);
#36494=ORIENTED_EDGE('',*,*,#24553,.F.);
#36495=ORIENTED_EDGE('',*,*,#26171,.T.);
#36496=ORIENTED_EDGE('',*,*,#23429,.T.);
#36497=ORIENTED_EDGE('',*,*,#26172,.F.);
#36498=ORIENTED_EDGE('',*,*,#24546,.F.);
#36499=ORIENTED_EDGE('',*,*,#26173,.T.);
#36500=ORIENTED_EDGE('',*,*,#23430,.T.);
#36501=ORIENTED_EDGE('',*,*,#26171,.F.);
#36502=ORIENTED_EDGE('',*,*,#24545,.F.);
#36503=ORIENTED_EDGE('',*,*,#26174,.T.);
#36504=ORIENTED_EDGE('',*,*,#23431,.T.);
#36505=ORIENTED_EDGE('',*,*,#26173,.F.);
#36506=ORIENTED_EDGE('',*,*,#24550,.F.);
#36507=ORIENTED_EDGE('',*,*,#26175,.T.);
#36508=ORIENTED_EDGE('',*,*,#23432,.T.);
#36509=ORIENTED_EDGE('',*,*,#26174,.F.);
#36510=ORIENTED_EDGE('',*,*,#24549,.F.);
#36511=ORIENTED_EDGE('',*,*,#26176,.T.);
#36512=ORIENTED_EDGE('',*,*,#23433,.T.);
#36513=ORIENTED_EDGE('',*,*,#26175,.F.);
#36514=ORIENTED_EDGE('',*,*,#24548,.F.);
#36515=ORIENTED_EDGE('',*,*,#26172,.T.);
#36516=ORIENTED_EDGE('',*,*,#23434,.T.);
#36517=ORIENTED_EDGE('',*,*,#26176,.F.);
#36518=ORIENTED_EDGE('',*,*,#24547,.F.);
#36519=ORIENTED_EDGE('',*,*,#26177,.T.);
#36520=ORIENTED_EDGE('',*,*,#23423,.T.);
#36521=ORIENTED_EDGE('',*,*,#26178,.F.);
#36522=ORIENTED_EDGE('',*,*,#24540,.F.);
#36523=ORIENTED_EDGE('',*,*,#26179,.T.);
#36524=ORIENTED_EDGE('',*,*,#23424,.T.);
#36525=ORIENTED_EDGE('',*,*,#26177,.F.);
#36526=ORIENTED_EDGE('',*,*,#24539,.F.);
#36527=ORIENTED_EDGE('',*,*,#26180,.T.);
#36528=ORIENTED_EDGE('',*,*,#23425,.T.);
#36529=ORIENTED_EDGE('',*,*,#26179,.F.);
#36530=ORIENTED_EDGE('',*,*,#24544,.F.);
#36531=ORIENTED_EDGE('',*,*,#26181,.T.);
#36532=ORIENTED_EDGE('',*,*,#23426,.T.);
#36533=ORIENTED_EDGE('',*,*,#26180,.F.);
#36534=ORIENTED_EDGE('',*,*,#24543,.F.);
#36535=ORIENTED_EDGE('',*,*,#26182,.T.);
#36536=ORIENTED_EDGE('',*,*,#23427,.T.);
#36537=ORIENTED_EDGE('',*,*,#26181,.F.);
#36538=ORIENTED_EDGE('',*,*,#24542,.F.);
#36539=ORIENTED_EDGE('',*,*,#26178,.T.);
#36540=ORIENTED_EDGE('',*,*,#23428,.T.);
#36541=ORIENTED_EDGE('',*,*,#26182,.F.);
#36542=ORIENTED_EDGE('',*,*,#24541,.F.);
#36543=ORIENTED_EDGE('',*,*,#26183,.T.);
#36544=ORIENTED_EDGE('',*,*,#23417,.T.);
#36545=ORIENTED_EDGE('',*,*,#26184,.F.);
#36546=ORIENTED_EDGE('',*,*,#24534,.F.);
#36547=ORIENTED_EDGE('',*,*,#26185,.T.);
#36548=ORIENTED_EDGE('',*,*,#23418,.T.);
#36549=ORIENTED_EDGE('',*,*,#26183,.F.);
#36550=ORIENTED_EDGE('',*,*,#24533,.F.);
#36551=ORIENTED_EDGE('',*,*,#26186,.T.);
#36552=ORIENTED_EDGE('',*,*,#23419,.T.);
#36553=ORIENTED_EDGE('',*,*,#26185,.F.);
#36554=ORIENTED_EDGE('',*,*,#24538,.F.);
#36555=ORIENTED_EDGE('',*,*,#26187,.T.);
#36556=ORIENTED_EDGE('',*,*,#23420,.T.);
#36557=ORIENTED_EDGE('',*,*,#26186,.F.);
#36558=ORIENTED_EDGE('',*,*,#24537,.F.);
#36559=ORIENTED_EDGE('',*,*,#26188,.T.);
#36560=ORIENTED_EDGE('',*,*,#23421,.T.);
#36561=ORIENTED_EDGE('',*,*,#26187,.F.);
#36562=ORIENTED_EDGE('',*,*,#24536,.F.);
#36563=ORIENTED_EDGE('',*,*,#26184,.T.);
#36564=ORIENTED_EDGE('',*,*,#23422,.T.);
#36565=ORIENTED_EDGE('',*,*,#26188,.F.);
#36566=ORIENTED_EDGE('',*,*,#24535,.F.);
#36567=ORIENTED_EDGE('',*,*,#26189,.T.);
#36568=ORIENTED_EDGE('',*,*,#23411,.T.);
#36569=ORIENTED_EDGE('',*,*,#26190,.F.);
#36570=ORIENTED_EDGE('',*,*,#24528,.F.);
#36571=ORIENTED_EDGE('',*,*,#26191,.T.);
#36572=ORIENTED_EDGE('',*,*,#23412,.T.);
#36573=ORIENTED_EDGE('',*,*,#26189,.F.);
#36574=ORIENTED_EDGE('',*,*,#24527,.F.);
#36575=ORIENTED_EDGE('',*,*,#26192,.T.);
#36576=ORIENTED_EDGE('',*,*,#23413,.T.);
#36577=ORIENTED_EDGE('',*,*,#26191,.F.);
#36578=ORIENTED_EDGE('',*,*,#24532,.F.);
#36579=ORIENTED_EDGE('',*,*,#26193,.T.);
#36580=ORIENTED_EDGE('',*,*,#23414,.T.);
#36581=ORIENTED_EDGE('',*,*,#26192,.F.);
#36582=ORIENTED_EDGE('',*,*,#24531,.F.);
#36583=ORIENTED_EDGE('',*,*,#26194,.T.);
#36584=ORIENTED_EDGE('',*,*,#23415,.T.);
#36585=ORIENTED_EDGE('',*,*,#26193,.F.);
#36586=ORIENTED_EDGE('',*,*,#24530,.F.);
#36587=ORIENTED_EDGE('',*,*,#26190,.T.);
#36588=ORIENTED_EDGE('',*,*,#23416,.T.);
#36589=ORIENTED_EDGE('',*,*,#26194,.F.);
#36590=ORIENTED_EDGE('',*,*,#24529,.F.);
#36591=ORIENTED_EDGE('',*,*,#26195,.T.);
#36592=ORIENTED_EDGE('',*,*,#23405,.T.);
#36593=ORIENTED_EDGE('',*,*,#26196,.F.);
#36594=ORIENTED_EDGE('',*,*,#24522,.F.);
#36595=ORIENTED_EDGE('',*,*,#26197,.T.);
#36596=ORIENTED_EDGE('',*,*,#23406,.T.);
#36597=ORIENTED_EDGE('',*,*,#26195,.F.);
#36598=ORIENTED_EDGE('',*,*,#24521,.F.);
#36599=ORIENTED_EDGE('',*,*,#26198,.T.);
#36600=ORIENTED_EDGE('',*,*,#23407,.T.);
#36601=ORIENTED_EDGE('',*,*,#26197,.F.);
#36602=ORIENTED_EDGE('',*,*,#24526,.F.);
#36603=ORIENTED_EDGE('',*,*,#26199,.T.);
#36604=ORIENTED_EDGE('',*,*,#23408,.T.);
#36605=ORIENTED_EDGE('',*,*,#26198,.F.);
#36606=ORIENTED_EDGE('',*,*,#24525,.F.);
#36607=ORIENTED_EDGE('',*,*,#26200,.T.);
#36608=ORIENTED_EDGE('',*,*,#23409,.T.);
#36609=ORIENTED_EDGE('',*,*,#26199,.F.);
#36610=ORIENTED_EDGE('',*,*,#24524,.F.);
#36611=ORIENTED_EDGE('',*,*,#26196,.T.);
#36612=ORIENTED_EDGE('',*,*,#23410,.T.);
#36613=ORIENTED_EDGE('',*,*,#26200,.F.);
#36614=ORIENTED_EDGE('',*,*,#24523,.F.);
#36615=ORIENTED_EDGE('',*,*,#26201,.T.);
#36616=ORIENTED_EDGE('',*,*,#23399,.T.);
#36617=ORIENTED_EDGE('',*,*,#26202,.F.);
#36618=ORIENTED_EDGE('',*,*,#24516,.F.);
#36619=ORIENTED_EDGE('',*,*,#26203,.T.);
#36620=ORIENTED_EDGE('',*,*,#23400,.T.);
#36621=ORIENTED_EDGE('',*,*,#26201,.F.);
#36622=ORIENTED_EDGE('',*,*,#24515,.F.);
#36623=ORIENTED_EDGE('',*,*,#26204,.T.);
#36624=ORIENTED_EDGE('',*,*,#23401,.T.);
#36625=ORIENTED_EDGE('',*,*,#26203,.F.);
#36626=ORIENTED_EDGE('',*,*,#24520,.F.);
#36627=ORIENTED_EDGE('',*,*,#26205,.T.);
#36628=ORIENTED_EDGE('',*,*,#23402,.T.);
#36629=ORIENTED_EDGE('',*,*,#26204,.F.);
#36630=ORIENTED_EDGE('',*,*,#24519,.F.);
#36631=ORIENTED_EDGE('',*,*,#26206,.T.);
#36632=ORIENTED_EDGE('',*,*,#23403,.T.);
#36633=ORIENTED_EDGE('',*,*,#26205,.F.);
#36634=ORIENTED_EDGE('',*,*,#24518,.F.);
#36635=ORIENTED_EDGE('',*,*,#26202,.T.);
#36636=ORIENTED_EDGE('',*,*,#23404,.T.);
#36637=ORIENTED_EDGE('',*,*,#26206,.F.);
#36638=ORIENTED_EDGE('',*,*,#24517,.F.);
#36639=ORIENTED_EDGE('',*,*,#26207,.T.);
#36640=ORIENTED_EDGE('',*,*,#23393,.T.);
#36641=ORIENTED_EDGE('',*,*,#26208,.F.);
#36642=ORIENTED_EDGE('',*,*,#24510,.F.);
#36643=ORIENTED_EDGE('',*,*,#26209,.T.);
#36644=ORIENTED_EDGE('',*,*,#23394,.T.);
#36645=ORIENTED_EDGE('',*,*,#26207,.F.);
#36646=ORIENTED_EDGE('',*,*,#24509,.F.);
#36647=ORIENTED_EDGE('',*,*,#26210,.T.);
#36648=ORIENTED_EDGE('',*,*,#23395,.T.);
#36649=ORIENTED_EDGE('',*,*,#26209,.F.);
#36650=ORIENTED_EDGE('',*,*,#24514,.F.);
#36651=ORIENTED_EDGE('',*,*,#26211,.T.);
#36652=ORIENTED_EDGE('',*,*,#23396,.T.);
#36653=ORIENTED_EDGE('',*,*,#26210,.F.);
#36654=ORIENTED_EDGE('',*,*,#24513,.F.);
#36655=ORIENTED_EDGE('',*,*,#26212,.T.);
#36656=ORIENTED_EDGE('',*,*,#23397,.T.);
#36657=ORIENTED_EDGE('',*,*,#26211,.F.);
#36658=ORIENTED_EDGE('',*,*,#24512,.F.);
#36659=ORIENTED_EDGE('',*,*,#26208,.T.);
#36660=ORIENTED_EDGE('',*,*,#23398,.T.);
#36661=ORIENTED_EDGE('',*,*,#26212,.F.);
#36662=ORIENTED_EDGE('',*,*,#24511,.F.);
#36663=ORIENTED_EDGE('',*,*,#26213,.T.);
#36664=ORIENTED_EDGE('',*,*,#23387,.T.);
#36665=ORIENTED_EDGE('',*,*,#26214,.F.);
#36666=ORIENTED_EDGE('',*,*,#24504,.F.);
#36667=ORIENTED_EDGE('',*,*,#26215,.T.);
#36668=ORIENTED_EDGE('',*,*,#23388,.T.);
#36669=ORIENTED_EDGE('',*,*,#26213,.F.);
#36670=ORIENTED_EDGE('',*,*,#24503,.F.);
#36671=ORIENTED_EDGE('',*,*,#26216,.T.);
#36672=ORIENTED_EDGE('',*,*,#23389,.T.);
#36673=ORIENTED_EDGE('',*,*,#26215,.F.);
#36674=ORIENTED_EDGE('',*,*,#24508,.F.);
#36675=ORIENTED_EDGE('',*,*,#26217,.T.);
#36676=ORIENTED_EDGE('',*,*,#23390,.T.);
#36677=ORIENTED_EDGE('',*,*,#26216,.F.);
#36678=ORIENTED_EDGE('',*,*,#24507,.F.);
#36679=ORIENTED_EDGE('',*,*,#26218,.T.);
#36680=ORIENTED_EDGE('',*,*,#23391,.T.);
#36681=ORIENTED_EDGE('',*,*,#26217,.F.);
#36682=ORIENTED_EDGE('',*,*,#24506,.F.);
#36683=ORIENTED_EDGE('',*,*,#26214,.T.);
#36684=ORIENTED_EDGE('',*,*,#23392,.T.);
#36685=ORIENTED_EDGE('',*,*,#26218,.F.);
#36686=ORIENTED_EDGE('',*,*,#24505,.F.);
#36687=ORIENTED_EDGE('',*,*,#26219,.T.);
#36688=ORIENTED_EDGE('',*,*,#23381,.T.);
#36689=ORIENTED_EDGE('',*,*,#26220,.F.);
#36690=ORIENTED_EDGE('',*,*,#24498,.F.);
#36691=ORIENTED_EDGE('',*,*,#26221,.T.);
#36692=ORIENTED_EDGE('',*,*,#23382,.T.);
#36693=ORIENTED_EDGE('',*,*,#26219,.F.);
#36694=ORIENTED_EDGE('',*,*,#24497,.F.);
#36695=ORIENTED_EDGE('',*,*,#26222,.T.);
#36696=ORIENTED_EDGE('',*,*,#23383,.T.);
#36697=ORIENTED_EDGE('',*,*,#26221,.F.);
#36698=ORIENTED_EDGE('',*,*,#24502,.F.);
#36699=ORIENTED_EDGE('',*,*,#26223,.T.);
#36700=ORIENTED_EDGE('',*,*,#23384,.T.);
#36701=ORIENTED_EDGE('',*,*,#26222,.F.);
#36702=ORIENTED_EDGE('',*,*,#24501,.F.);
#36703=ORIENTED_EDGE('',*,*,#26224,.T.);
#36704=ORIENTED_EDGE('',*,*,#23385,.T.);
#36705=ORIENTED_EDGE('',*,*,#26223,.F.);
#36706=ORIENTED_EDGE('',*,*,#24500,.F.);
#36707=ORIENTED_EDGE('',*,*,#26220,.T.);
#36708=ORIENTED_EDGE('',*,*,#23386,.T.);
#36709=ORIENTED_EDGE('',*,*,#26224,.F.);
#36710=ORIENTED_EDGE('',*,*,#24499,.F.);
#36711=ORIENTED_EDGE('',*,*,#26225,.T.);
#36712=ORIENTED_EDGE('',*,*,#23375,.T.);
#36713=ORIENTED_EDGE('',*,*,#26226,.F.);
#36714=ORIENTED_EDGE('',*,*,#24492,.F.);
#36715=ORIENTED_EDGE('',*,*,#26227,.T.);
#36716=ORIENTED_EDGE('',*,*,#23376,.T.);
#36717=ORIENTED_EDGE('',*,*,#26225,.F.);
#36718=ORIENTED_EDGE('',*,*,#24491,.F.);
#36719=ORIENTED_EDGE('',*,*,#26228,.T.);
#36720=ORIENTED_EDGE('',*,*,#23377,.T.);
#36721=ORIENTED_EDGE('',*,*,#26227,.F.);
#36722=ORIENTED_EDGE('',*,*,#24496,.F.);
#36723=ORIENTED_EDGE('',*,*,#26229,.T.);
#36724=ORIENTED_EDGE('',*,*,#23378,.T.);
#36725=ORIENTED_EDGE('',*,*,#26228,.F.);
#36726=ORIENTED_EDGE('',*,*,#24495,.F.);
#36727=ORIENTED_EDGE('',*,*,#26230,.T.);
#36728=ORIENTED_EDGE('',*,*,#23379,.T.);
#36729=ORIENTED_EDGE('',*,*,#26229,.F.);
#36730=ORIENTED_EDGE('',*,*,#24494,.F.);
#36731=ORIENTED_EDGE('',*,*,#26226,.T.);
#36732=ORIENTED_EDGE('',*,*,#23380,.T.);
#36733=ORIENTED_EDGE('',*,*,#26230,.F.);
#36734=ORIENTED_EDGE('',*,*,#24493,.F.);
#36735=ORIENTED_EDGE('',*,*,#26231,.T.);
#36736=ORIENTED_EDGE('',*,*,#23369,.T.);
#36737=ORIENTED_EDGE('',*,*,#26232,.F.);
#36738=ORIENTED_EDGE('',*,*,#24486,.F.);
#36739=ORIENTED_EDGE('',*,*,#26233,.T.);
#36740=ORIENTED_EDGE('',*,*,#23370,.T.);
#36741=ORIENTED_EDGE('',*,*,#26231,.F.);
#36742=ORIENTED_EDGE('',*,*,#24485,.F.);
#36743=ORIENTED_EDGE('',*,*,#26234,.T.);
#36744=ORIENTED_EDGE('',*,*,#23371,.T.);
#36745=ORIENTED_EDGE('',*,*,#26233,.F.);
#36746=ORIENTED_EDGE('',*,*,#24490,.F.);
#36747=ORIENTED_EDGE('',*,*,#26235,.T.);
#36748=ORIENTED_EDGE('',*,*,#23372,.T.);
#36749=ORIENTED_EDGE('',*,*,#26234,.F.);
#36750=ORIENTED_EDGE('',*,*,#24489,.F.);
#36751=ORIENTED_EDGE('',*,*,#26236,.T.);
#36752=ORIENTED_EDGE('',*,*,#23373,.T.);
#36753=ORIENTED_EDGE('',*,*,#26235,.F.);
#36754=ORIENTED_EDGE('',*,*,#24488,.F.);
#36755=ORIENTED_EDGE('',*,*,#26232,.T.);
#36756=ORIENTED_EDGE('',*,*,#23374,.T.);
#36757=ORIENTED_EDGE('',*,*,#26236,.F.);
#36758=ORIENTED_EDGE('',*,*,#24487,.F.);
#36759=ORIENTED_EDGE('',*,*,#26237,.T.);
#36760=ORIENTED_EDGE('',*,*,#23363,.T.);
#36761=ORIENTED_EDGE('',*,*,#26238,.F.);
#36762=ORIENTED_EDGE('',*,*,#24480,.F.);
#36763=ORIENTED_EDGE('',*,*,#26239,.T.);
#36764=ORIENTED_EDGE('',*,*,#23364,.T.);
#36765=ORIENTED_EDGE('',*,*,#26237,.F.);
#36766=ORIENTED_EDGE('',*,*,#24479,.F.);
#36767=ORIENTED_EDGE('',*,*,#26240,.T.);
#36768=ORIENTED_EDGE('',*,*,#23365,.T.);
#36769=ORIENTED_EDGE('',*,*,#26239,.F.);
#36770=ORIENTED_EDGE('',*,*,#24484,.F.);
#36771=ORIENTED_EDGE('',*,*,#26241,.T.);
#36772=ORIENTED_EDGE('',*,*,#23366,.T.);
#36773=ORIENTED_EDGE('',*,*,#26240,.F.);
#36774=ORIENTED_EDGE('',*,*,#24483,.F.);
#36775=ORIENTED_EDGE('',*,*,#26242,.T.);
#36776=ORIENTED_EDGE('',*,*,#23367,.T.);
#36777=ORIENTED_EDGE('',*,*,#26241,.F.);
#36778=ORIENTED_EDGE('',*,*,#24482,.F.);
#36779=ORIENTED_EDGE('',*,*,#26238,.T.);
#36780=ORIENTED_EDGE('',*,*,#23368,.T.);
#36781=ORIENTED_EDGE('',*,*,#26242,.F.);
#36782=ORIENTED_EDGE('',*,*,#24481,.F.);
#36783=ORIENTED_EDGE('',*,*,#26243,.T.);
#36784=ORIENTED_EDGE('',*,*,#23357,.T.);
#36785=ORIENTED_EDGE('',*,*,#26244,.F.);
#36786=ORIENTED_EDGE('',*,*,#24474,.F.);
#36787=ORIENTED_EDGE('',*,*,#26245,.T.);
#36788=ORIENTED_EDGE('',*,*,#23358,.T.);
#36789=ORIENTED_EDGE('',*,*,#26243,.F.);
#36790=ORIENTED_EDGE('',*,*,#24473,.F.);
#36791=ORIENTED_EDGE('',*,*,#26246,.T.);
#36792=ORIENTED_EDGE('',*,*,#23359,.T.);
#36793=ORIENTED_EDGE('',*,*,#26245,.F.);
#36794=ORIENTED_EDGE('',*,*,#24478,.F.);
#36795=ORIENTED_EDGE('',*,*,#26247,.T.);
#36796=ORIENTED_EDGE('',*,*,#23360,.T.);
#36797=ORIENTED_EDGE('',*,*,#26246,.F.);
#36798=ORIENTED_EDGE('',*,*,#24477,.F.);
#36799=ORIENTED_EDGE('',*,*,#26248,.T.);
#36800=ORIENTED_EDGE('',*,*,#23361,.T.);
#36801=ORIENTED_EDGE('',*,*,#26247,.F.);
#36802=ORIENTED_EDGE('',*,*,#24476,.F.);
#36803=ORIENTED_EDGE('',*,*,#26244,.T.);
#36804=ORIENTED_EDGE('',*,*,#23362,.T.);
#36805=ORIENTED_EDGE('',*,*,#26248,.F.);
#36806=ORIENTED_EDGE('',*,*,#24475,.F.);
#36807=ORIENTED_EDGE('',*,*,#26249,.T.);
#36808=ORIENTED_EDGE('',*,*,#23351,.T.);
#36809=ORIENTED_EDGE('',*,*,#26250,.F.);
#36810=ORIENTED_EDGE('',*,*,#24468,.F.);
#36811=ORIENTED_EDGE('',*,*,#26251,.T.);
#36812=ORIENTED_EDGE('',*,*,#23352,.T.);
#36813=ORIENTED_EDGE('',*,*,#26249,.F.);
#36814=ORIENTED_EDGE('',*,*,#24467,.F.);
#36815=ORIENTED_EDGE('',*,*,#26252,.T.);
#36816=ORIENTED_EDGE('',*,*,#23353,.T.);
#36817=ORIENTED_EDGE('',*,*,#26251,.F.);
#36818=ORIENTED_EDGE('',*,*,#24472,.F.);
#36819=ORIENTED_EDGE('',*,*,#26253,.T.);
#36820=ORIENTED_EDGE('',*,*,#23354,.T.);
#36821=ORIENTED_EDGE('',*,*,#26252,.F.);
#36822=ORIENTED_EDGE('',*,*,#24471,.F.);
#36823=ORIENTED_EDGE('',*,*,#26254,.T.);
#36824=ORIENTED_EDGE('',*,*,#23355,.T.);
#36825=ORIENTED_EDGE('',*,*,#26253,.F.);
#36826=ORIENTED_EDGE('',*,*,#24470,.F.);
#36827=ORIENTED_EDGE('',*,*,#26250,.T.);
#36828=ORIENTED_EDGE('',*,*,#23356,.T.);
#36829=ORIENTED_EDGE('',*,*,#26254,.F.);
#36830=ORIENTED_EDGE('',*,*,#24469,.F.);
#36831=ORIENTED_EDGE('',*,*,#26255,.T.);
#36832=ORIENTED_EDGE('',*,*,#23345,.T.);
#36833=ORIENTED_EDGE('',*,*,#26256,.F.);
#36834=ORIENTED_EDGE('',*,*,#24462,.F.);
#36835=ORIENTED_EDGE('',*,*,#26257,.T.);
#36836=ORIENTED_EDGE('',*,*,#23346,.T.);
#36837=ORIENTED_EDGE('',*,*,#26255,.F.);
#36838=ORIENTED_EDGE('',*,*,#24461,.F.);
#36839=ORIENTED_EDGE('',*,*,#26258,.T.);
#36840=ORIENTED_EDGE('',*,*,#23347,.T.);
#36841=ORIENTED_EDGE('',*,*,#26257,.F.);
#36842=ORIENTED_EDGE('',*,*,#24466,.F.);
#36843=ORIENTED_EDGE('',*,*,#26259,.T.);
#36844=ORIENTED_EDGE('',*,*,#23348,.T.);
#36845=ORIENTED_EDGE('',*,*,#26258,.F.);
#36846=ORIENTED_EDGE('',*,*,#24465,.F.);
#36847=ORIENTED_EDGE('',*,*,#26260,.T.);
#36848=ORIENTED_EDGE('',*,*,#23349,.T.);
#36849=ORIENTED_EDGE('',*,*,#26259,.F.);
#36850=ORIENTED_EDGE('',*,*,#24464,.F.);
#36851=ORIENTED_EDGE('',*,*,#26256,.T.);
#36852=ORIENTED_EDGE('',*,*,#23350,.T.);
#36853=ORIENTED_EDGE('',*,*,#26260,.F.);
#36854=ORIENTED_EDGE('',*,*,#24463,.F.);
#36855=ORIENTED_EDGE('',*,*,#26261,.T.);
#36856=ORIENTED_EDGE('',*,*,#23339,.T.);
#36857=ORIENTED_EDGE('',*,*,#26262,.F.);
#36858=ORIENTED_EDGE('',*,*,#24456,.F.);
#36859=ORIENTED_EDGE('',*,*,#26263,.T.);
#36860=ORIENTED_EDGE('',*,*,#23340,.T.);
#36861=ORIENTED_EDGE('',*,*,#26261,.F.);
#36862=ORIENTED_EDGE('',*,*,#24455,.F.);
#36863=ORIENTED_EDGE('',*,*,#26264,.T.);
#36864=ORIENTED_EDGE('',*,*,#23341,.T.);
#36865=ORIENTED_EDGE('',*,*,#26263,.F.);
#36866=ORIENTED_EDGE('',*,*,#24460,.F.);
#36867=ORIENTED_EDGE('',*,*,#26265,.T.);
#36868=ORIENTED_EDGE('',*,*,#23342,.T.);
#36869=ORIENTED_EDGE('',*,*,#26264,.F.);
#36870=ORIENTED_EDGE('',*,*,#24459,.F.);
#36871=ORIENTED_EDGE('',*,*,#26266,.T.);
#36872=ORIENTED_EDGE('',*,*,#23343,.T.);
#36873=ORIENTED_EDGE('',*,*,#26265,.F.);
#36874=ORIENTED_EDGE('',*,*,#24458,.F.);
#36875=ORIENTED_EDGE('',*,*,#26262,.T.);
#36876=ORIENTED_EDGE('',*,*,#23344,.T.);
#36877=ORIENTED_EDGE('',*,*,#26266,.F.);
#36878=ORIENTED_EDGE('',*,*,#24457,.F.);
#36879=ORIENTED_EDGE('',*,*,#26267,.T.);
#36880=ORIENTED_EDGE('',*,*,#23333,.T.);
#36881=ORIENTED_EDGE('',*,*,#26268,.F.);
#36882=ORIENTED_EDGE('',*,*,#24450,.F.);
#36883=ORIENTED_EDGE('',*,*,#26269,.T.);
#36884=ORIENTED_EDGE('',*,*,#23334,.T.);
#36885=ORIENTED_EDGE('',*,*,#26267,.F.);
#36886=ORIENTED_EDGE('',*,*,#24449,.F.);
#36887=ORIENTED_EDGE('',*,*,#26270,.T.);
#36888=ORIENTED_EDGE('',*,*,#23335,.T.);
#36889=ORIENTED_EDGE('',*,*,#26269,.F.);
#36890=ORIENTED_EDGE('',*,*,#24454,.F.);
#36891=ORIENTED_EDGE('',*,*,#26271,.T.);
#36892=ORIENTED_EDGE('',*,*,#23336,.T.);
#36893=ORIENTED_EDGE('',*,*,#26270,.F.);
#36894=ORIENTED_EDGE('',*,*,#24453,.F.);
#36895=ORIENTED_EDGE('',*,*,#26272,.T.);
#36896=ORIENTED_EDGE('',*,*,#23337,.T.);
#36897=ORIENTED_EDGE('',*,*,#26271,.F.);
#36898=ORIENTED_EDGE('',*,*,#24452,.F.);
#36899=ORIENTED_EDGE('',*,*,#26268,.T.);
#36900=ORIENTED_EDGE('',*,*,#23338,.T.);
#36901=ORIENTED_EDGE('',*,*,#26272,.F.);
#36902=ORIENTED_EDGE('',*,*,#24451,.F.);
#36903=ORIENTED_EDGE('',*,*,#26273,.T.);
#36904=ORIENTED_EDGE('',*,*,#23327,.T.);
#36905=ORIENTED_EDGE('',*,*,#26274,.F.);
#36906=ORIENTED_EDGE('',*,*,#24444,.F.);
#36907=ORIENTED_EDGE('',*,*,#26275,.T.);
#36908=ORIENTED_EDGE('',*,*,#23328,.T.);
#36909=ORIENTED_EDGE('',*,*,#26273,.F.);
#36910=ORIENTED_EDGE('',*,*,#24443,.F.);
#36911=ORIENTED_EDGE('',*,*,#26276,.T.);
#36912=ORIENTED_EDGE('',*,*,#23329,.T.);
#36913=ORIENTED_EDGE('',*,*,#26275,.F.);
#36914=ORIENTED_EDGE('',*,*,#24448,.F.);
#36915=ORIENTED_EDGE('',*,*,#26277,.T.);
#36916=ORIENTED_EDGE('',*,*,#23330,.T.);
#36917=ORIENTED_EDGE('',*,*,#26276,.F.);
#36918=ORIENTED_EDGE('',*,*,#24447,.F.);
#36919=ORIENTED_EDGE('',*,*,#26278,.T.);
#36920=ORIENTED_EDGE('',*,*,#23331,.T.);
#36921=ORIENTED_EDGE('',*,*,#26277,.F.);
#36922=ORIENTED_EDGE('',*,*,#24446,.F.);
#36923=ORIENTED_EDGE('',*,*,#26274,.T.);
#36924=ORIENTED_EDGE('',*,*,#23332,.T.);
#36925=ORIENTED_EDGE('',*,*,#26278,.F.);
#36926=ORIENTED_EDGE('',*,*,#24445,.F.);
#36927=ORIENTED_EDGE('',*,*,#26279,.T.);
#36928=ORIENTED_EDGE('',*,*,#23321,.T.);
#36929=ORIENTED_EDGE('',*,*,#26280,.F.);
#36930=ORIENTED_EDGE('',*,*,#24438,.F.);
#36931=ORIENTED_EDGE('',*,*,#26281,.T.);
#36932=ORIENTED_EDGE('',*,*,#23322,.T.);
#36933=ORIENTED_EDGE('',*,*,#26279,.F.);
#36934=ORIENTED_EDGE('',*,*,#24437,.F.);
#36935=ORIENTED_EDGE('',*,*,#26282,.T.);
#36936=ORIENTED_EDGE('',*,*,#23323,.T.);
#36937=ORIENTED_EDGE('',*,*,#26281,.F.);
#36938=ORIENTED_EDGE('',*,*,#24442,.F.);
#36939=ORIENTED_EDGE('',*,*,#26283,.T.);
#36940=ORIENTED_EDGE('',*,*,#23324,.T.);
#36941=ORIENTED_EDGE('',*,*,#26282,.F.);
#36942=ORIENTED_EDGE('',*,*,#24441,.F.);
#36943=ORIENTED_EDGE('',*,*,#26284,.T.);
#36944=ORIENTED_EDGE('',*,*,#23325,.T.);
#36945=ORIENTED_EDGE('',*,*,#26283,.F.);
#36946=ORIENTED_EDGE('',*,*,#24440,.F.);
#36947=ORIENTED_EDGE('',*,*,#26280,.T.);
#36948=ORIENTED_EDGE('',*,*,#23326,.T.);
#36949=ORIENTED_EDGE('',*,*,#26284,.F.);
#36950=ORIENTED_EDGE('',*,*,#24439,.F.);
#36951=ORIENTED_EDGE('',*,*,#26285,.T.);
#36952=ORIENTED_EDGE('',*,*,#23315,.T.);
#36953=ORIENTED_EDGE('',*,*,#26286,.F.);
#36954=ORIENTED_EDGE('',*,*,#24432,.F.);
#36955=ORIENTED_EDGE('',*,*,#26287,.T.);
#36956=ORIENTED_EDGE('',*,*,#23316,.T.);
#36957=ORIENTED_EDGE('',*,*,#26285,.F.);
#36958=ORIENTED_EDGE('',*,*,#24431,.F.);
#36959=ORIENTED_EDGE('',*,*,#26288,.T.);
#36960=ORIENTED_EDGE('',*,*,#23317,.T.);
#36961=ORIENTED_EDGE('',*,*,#26287,.F.);
#36962=ORIENTED_EDGE('',*,*,#24436,.F.);
#36963=ORIENTED_EDGE('',*,*,#26289,.T.);
#36964=ORIENTED_EDGE('',*,*,#23318,.T.);
#36965=ORIENTED_EDGE('',*,*,#26288,.F.);
#36966=ORIENTED_EDGE('',*,*,#24435,.F.);
#36967=ORIENTED_EDGE('',*,*,#26290,.T.);
#36968=ORIENTED_EDGE('',*,*,#23319,.T.);
#36969=ORIENTED_EDGE('',*,*,#26289,.F.);
#36970=ORIENTED_EDGE('',*,*,#24434,.F.);
#36971=ORIENTED_EDGE('',*,*,#26286,.T.);
#36972=ORIENTED_EDGE('',*,*,#23320,.T.);
#36973=ORIENTED_EDGE('',*,*,#26290,.F.);
#36974=ORIENTED_EDGE('',*,*,#24433,.F.);
#36975=ORIENTED_EDGE('',*,*,#26291,.T.);
#36976=ORIENTED_EDGE('',*,*,#23309,.T.);
#36977=ORIENTED_EDGE('',*,*,#26292,.F.);
#36978=ORIENTED_EDGE('',*,*,#24426,.F.);
#36979=ORIENTED_EDGE('',*,*,#26293,.T.);
#36980=ORIENTED_EDGE('',*,*,#23310,.T.);
#36981=ORIENTED_EDGE('',*,*,#26291,.F.);
#36982=ORIENTED_EDGE('',*,*,#24425,.F.);
#36983=ORIENTED_EDGE('',*,*,#26294,.T.);
#36984=ORIENTED_EDGE('',*,*,#23311,.T.);
#36985=ORIENTED_EDGE('',*,*,#26293,.F.);
#36986=ORIENTED_EDGE('',*,*,#24430,.F.);
#36987=ORIENTED_EDGE('',*,*,#26295,.T.);
#36988=ORIENTED_EDGE('',*,*,#23312,.T.);
#36989=ORIENTED_EDGE('',*,*,#26294,.F.);
#36990=ORIENTED_EDGE('',*,*,#24429,.F.);
#36991=ORIENTED_EDGE('',*,*,#26296,.T.);
#36992=ORIENTED_EDGE('',*,*,#23313,.T.);
#36993=ORIENTED_EDGE('',*,*,#26295,.F.);
#36994=ORIENTED_EDGE('',*,*,#24428,.F.);
#36995=ORIENTED_EDGE('',*,*,#26292,.T.);
#36996=ORIENTED_EDGE('',*,*,#23314,.T.);
#36997=ORIENTED_EDGE('',*,*,#26296,.F.);
#36998=ORIENTED_EDGE('',*,*,#24427,.F.);
#36999=ORIENTED_EDGE('',*,*,#26297,.T.);
#37000=ORIENTED_EDGE('',*,*,#23303,.T.);
#37001=ORIENTED_EDGE('',*,*,#26298,.F.);
#37002=ORIENTED_EDGE('',*,*,#24420,.F.);
#37003=ORIENTED_EDGE('',*,*,#26299,.T.);
#37004=ORIENTED_EDGE('',*,*,#23304,.T.);
#37005=ORIENTED_EDGE('',*,*,#26297,.F.);
#37006=ORIENTED_EDGE('',*,*,#24419,.F.);
#37007=ORIENTED_EDGE('',*,*,#26300,.T.);
#37008=ORIENTED_EDGE('',*,*,#23305,.T.);
#37009=ORIENTED_EDGE('',*,*,#26299,.F.);
#37010=ORIENTED_EDGE('',*,*,#24424,.F.);
#37011=ORIENTED_EDGE('',*,*,#26301,.T.);
#37012=ORIENTED_EDGE('',*,*,#23306,.T.);
#37013=ORIENTED_EDGE('',*,*,#26300,.F.);
#37014=ORIENTED_EDGE('',*,*,#24423,.F.);
#37015=ORIENTED_EDGE('',*,*,#26302,.T.);
#37016=ORIENTED_EDGE('',*,*,#23307,.T.);
#37017=ORIENTED_EDGE('',*,*,#26301,.F.);
#37018=ORIENTED_EDGE('',*,*,#24422,.F.);
#37019=ORIENTED_EDGE('',*,*,#26298,.T.);
#37020=ORIENTED_EDGE('',*,*,#23308,.T.);
#37021=ORIENTED_EDGE('',*,*,#26302,.F.);
#37022=ORIENTED_EDGE('',*,*,#24421,.F.);
#37023=ORIENTED_EDGE('',*,*,#26303,.T.);
#37024=ORIENTED_EDGE('',*,*,#23297,.T.);
#37025=ORIENTED_EDGE('',*,*,#26304,.F.);
#37026=ORIENTED_EDGE('',*,*,#24414,.F.);
#37027=ORIENTED_EDGE('',*,*,#26305,.T.);
#37028=ORIENTED_EDGE('',*,*,#23298,.T.);
#37029=ORIENTED_EDGE('',*,*,#26303,.F.);
#37030=ORIENTED_EDGE('',*,*,#24413,.F.);
#37031=ORIENTED_EDGE('',*,*,#26306,.T.);
#37032=ORIENTED_EDGE('',*,*,#23299,.T.);
#37033=ORIENTED_EDGE('',*,*,#26305,.F.);
#37034=ORIENTED_EDGE('',*,*,#24418,.F.);
#37035=ORIENTED_EDGE('',*,*,#26307,.T.);
#37036=ORIENTED_EDGE('',*,*,#23300,.T.);
#37037=ORIENTED_EDGE('',*,*,#26306,.F.);
#37038=ORIENTED_EDGE('',*,*,#24417,.F.);
#37039=ORIENTED_EDGE('',*,*,#26308,.T.);
#37040=ORIENTED_EDGE('',*,*,#23301,.T.);
#37041=ORIENTED_EDGE('',*,*,#26307,.F.);
#37042=ORIENTED_EDGE('',*,*,#24416,.F.);
#37043=ORIENTED_EDGE('',*,*,#26304,.T.);
#37044=ORIENTED_EDGE('',*,*,#23302,.T.);
#37045=ORIENTED_EDGE('',*,*,#26308,.F.);
#37046=ORIENTED_EDGE('',*,*,#24415,.F.);
#37047=ORIENTED_EDGE('',*,*,#26309,.T.);
#37048=ORIENTED_EDGE('',*,*,#23291,.T.);
#37049=ORIENTED_EDGE('',*,*,#26310,.F.);
#37050=ORIENTED_EDGE('',*,*,#24408,.F.);
#37051=ORIENTED_EDGE('',*,*,#26311,.T.);
#37052=ORIENTED_EDGE('',*,*,#23292,.T.);
#37053=ORIENTED_EDGE('',*,*,#26309,.F.);
#37054=ORIENTED_EDGE('',*,*,#24407,.F.);
#37055=ORIENTED_EDGE('',*,*,#26312,.T.);
#37056=ORIENTED_EDGE('',*,*,#23293,.T.);
#37057=ORIENTED_EDGE('',*,*,#26311,.F.);
#37058=ORIENTED_EDGE('',*,*,#24412,.F.);
#37059=ORIENTED_EDGE('',*,*,#26313,.T.);
#37060=ORIENTED_EDGE('',*,*,#23294,.T.);
#37061=ORIENTED_EDGE('',*,*,#26312,.F.);
#37062=ORIENTED_EDGE('',*,*,#24411,.F.);
#37063=ORIENTED_EDGE('',*,*,#26314,.T.);
#37064=ORIENTED_EDGE('',*,*,#23295,.T.);
#37065=ORIENTED_EDGE('',*,*,#26313,.F.);
#37066=ORIENTED_EDGE('',*,*,#24410,.F.);
#37067=ORIENTED_EDGE('',*,*,#26310,.T.);
#37068=ORIENTED_EDGE('',*,*,#23296,.T.);
#37069=ORIENTED_EDGE('',*,*,#26314,.F.);
#37070=ORIENTED_EDGE('',*,*,#24409,.F.);
#37071=ORIENTED_EDGE('',*,*,#26315,.T.);
#37072=ORIENTED_EDGE('',*,*,#23285,.T.);
#37073=ORIENTED_EDGE('',*,*,#26316,.F.);
#37074=ORIENTED_EDGE('',*,*,#24402,.F.);
#37075=ORIENTED_EDGE('',*,*,#26317,.T.);
#37076=ORIENTED_EDGE('',*,*,#23286,.T.);
#37077=ORIENTED_EDGE('',*,*,#26315,.F.);
#37078=ORIENTED_EDGE('',*,*,#24401,.F.);
#37079=ORIENTED_EDGE('',*,*,#26318,.T.);
#37080=ORIENTED_EDGE('',*,*,#23287,.T.);
#37081=ORIENTED_EDGE('',*,*,#26317,.F.);
#37082=ORIENTED_EDGE('',*,*,#24406,.F.);
#37083=ORIENTED_EDGE('',*,*,#26319,.T.);
#37084=ORIENTED_EDGE('',*,*,#23288,.T.);
#37085=ORIENTED_EDGE('',*,*,#26318,.F.);
#37086=ORIENTED_EDGE('',*,*,#24405,.F.);
#37087=ORIENTED_EDGE('',*,*,#26320,.T.);
#37088=ORIENTED_EDGE('',*,*,#23289,.T.);
#37089=ORIENTED_EDGE('',*,*,#26319,.F.);
#37090=ORIENTED_EDGE('',*,*,#24404,.F.);
#37091=ORIENTED_EDGE('',*,*,#26316,.T.);
#37092=ORIENTED_EDGE('',*,*,#23290,.T.);
#37093=ORIENTED_EDGE('',*,*,#26320,.F.);
#37094=ORIENTED_EDGE('',*,*,#24403,.F.);
#37095=ORIENTED_EDGE('',*,*,#26321,.T.);
#37096=ORIENTED_EDGE('',*,*,#23279,.T.);
#37097=ORIENTED_EDGE('',*,*,#26322,.F.);
#37098=ORIENTED_EDGE('',*,*,#24396,.F.);
#37099=ORIENTED_EDGE('',*,*,#26323,.T.);
#37100=ORIENTED_EDGE('',*,*,#23280,.T.);
#37101=ORIENTED_EDGE('',*,*,#26321,.F.);
#37102=ORIENTED_EDGE('',*,*,#24395,.F.);
#37103=ORIENTED_EDGE('',*,*,#26324,.T.);
#37104=ORIENTED_EDGE('',*,*,#23281,.T.);
#37105=ORIENTED_EDGE('',*,*,#26323,.F.);
#37106=ORIENTED_EDGE('',*,*,#24400,.F.);
#37107=ORIENTED_EDGE('',*,*,#26325,.T.);
#37108=ORIENTED_EDGE('',*,*,#23282,.T.);
#37109=ORIENTED_EDGE('',*,*,#26324,.F.);
#37110=ORIENTED_EDGE('',*,*,#24399,.F.);
#37111=ORIENTED_EDGE('',*,*,#26326,.T.);
#37112=ORIENTED_EDGE('',*,*,#23283,.T.);
#37113=ORIENTED_EDGE('',*,*,#26325,.F.);
#37114=ORIENTED_EDGE('',*,*,#24398,.F.);
#37115=ORIENTED_EDGE('',*,*,#26322,.T.);
#37116=ORIENTED_EDGE('',*,*,#23284,.T.);
#37117=ORIENTED_EDGE('',*,*,#26326,.F.);
#37118=ORIENTED_EDGE('',*,*,#24397,.F.);
#37119=ORIENTED_EDGE('',*,*,#26327,.T.);
#37120=ORIENTED_EDGE('',*,*,#23273,.T.);
#37121=ORIENTED_EDGE('',*,*,#26328,.F.);
#37122=ORIENTED_EDGE('',*,*,#24390,.F.);
#37123=ORIENTED_EDGE('',*,*,#26329,.T.);
#37124=ORIENTED_EDGE('',*,*,#23274,.T.);
#37125=ORIENTED_EDGE('',*,*,#26327,.F.);
#37126=ORIENTED_EDGE('',*,*,#24389,.F.);
#37127=ORIENTED_EDGE('',*,*,#26330,.T.);
#37128=ORIENTED_EDGE('',*,*,#23275,.T.);
#37129=ORIENTED_EDGE('',*,*,#26329,.F.);
#37130=ORIENTED_EDGE('',*,*,#24394,.F.);
#37131=ORIENTED_EDGE('',*,*,#26331,.T.);
#37132=ORIENTED_EDGE('',*,*,#23276,.T.);
#37133=ORIENTED_EDGE('',*,*,#26330,.F.);
#37134=ORIENTED_EDGE('',*,*,#24393,.F.);
#37135=ORIENTED_EDGE('',*,*,#26332,.T.);
#37136=ORIENTED_EDGE('',*,*,#23277,.T.);
#37137=ORIENTED_EDGE('',*,*,#26331,.F.);
#37138=ORIENTED_EDGE('',*,*,#24392,.F.);
#37139=ORIENTED_EDGE('',*,*,#26328,.T.);
#37140=ORIENTED_EDGE('',*,*,#23278,.T.);
#37141=ORIENTED_EDGE('',*,*,#26332,.F.);
#37142=ORIENTED_EDGE('',*,*,#24391,.F.);
#37143=ORIENTED_EDGE('',*,*,#26333,.T.);
#37144=ORIENTED_EDGE('',*,*,#23267,.T.);
#37145=ORIENTED_EDGE('',*,*,#26334,.F.);
#37146=ORIENTED_EDGE('',*,*,#24384,.F.);
#37147=ORIENTED_EDGE('',*,*,#26335,.T.);
#37148=ORIENTED_EDGE('',*,*,#23268,.T.);
#37149=ORIENTED_EDGE('',*,*,#26333,.F.);
#37150=ORIENTED_EDGE('',*,*,#24383,.F.);
#37151=ORIENTED_EDGE('',*,*,#26336,.T.);
#37152=ORIENTED_EDGE('',*,*,#23269,.T.);
#37153=ORIENTED_EDGE('',*,*,#26335,.F.);
#37154=ORIENTED_EDGE('',*,*,#24388,.F.);
#37155=ORIENTED_EDGE('',*,*,#26337,.T.);
#37156=ORIENTED_EDGE('',*,*,#23270,.T.);
#37157=ORIENTED_EDGE('',*,*,#26336,.F.);
#37158=ORIENTED_EDGE('',*,*,#24387,.F.);
#37159=ORIENTED_EDGE('',*,*,#26338,.T.);
#37160=ORIENTED_EDGE('',*,*,#23271,.T.);
#37161=ORIENTED_EDGE('',*,*,#26337,.F.);
#37162=ORIENTED_EDGE('',*,*,#24386,.F.);
#37163=ORIENTED_EDGE('',*,*,#26334,.T.);
#37164=ORIENTED_EDGE('',*,*,#23272,.T.);
#37165=ORIENTED_EDGE('',*,*,#26338,.F.);
#37166=ORIENTED_EDGE('',*,*,#24385,.F.);
#37167=ORIENTED_EDGE('',*,*,#26339,.T.);
#37168=ORIENTED_EDGE('',*,*,#23261,.T.);
#37169=ORIENTED_EDGE('',*,*,#26340,.F.);
#37170=ORIENTED_EDGE('',*,*,#24378,.F.);
#37171=ORIENTED_EDGE('',*,*,#26341,.T.);
#37172=ORIENTED_EDGE('',*,*,#23262,.T.);
#37173=ORIENTED_EDGE('',*,*,#26339,.F.);
#37174=ORIENTED_EDGE('',*,*,#24377,.F.);
#37175=ORIENTED_EDGE('',*,*,#26342,.T.);
#37176=ORIENTED_EDGE('',*,*,#23263,.T.);
#37177=ORIENTED_EDGE('',*,*,#26341,.F.);
#37178=ORIENTED_EDGE('',*,*,#24382,.F.);
#37179=ORIENTED_EDGE('',*,*,#26343,.T.);
#37180=ORIENTED_EDGE('',*,*,#23264,.T.);
#37181=ORIENTED_EDGE('',*,*,#26342,.F.);
#37182=ORIENTED_EDGE('',*,*,#24381,.F.);
#37183=ORIENTED_EDGE('',*,*,#26344,.T.);
#37184=ORIENTED_EDGE('',*,*,#23265,.T.);
#37185=ORIENTED_EDGE('',*,*,#26343,.F.);
#37186=ORIENTED_EDGE('',*,*,#24380,.F.);
#37187=ORIENTED_EDGE('',*,*,#26340,.T.);
#37188=ORIENTED_EDGE('',*,*,#23266,.T.);
#37189=ORIENTED_EDGE('',*,*,#26344,.F.);
#37190=ORIENTED_EDGE('',*,*,#24379,.F.);
#37191=ORIENTED_EDGE('',*,*,#26345,.T.);
#37192=ORIENTED_EDGE('',*,*,#23255,.T.);
#37193=ORIENTED_EDGE('',*,*,#26346,.F.);
#37194=ORIENTED_EDGE('',*,*,#24372,.F.);
#37195=ORIENTED_EDGE('',*,*,#26347,.T.);
#37196=ORIENTED_EDGE('',*,*,#23256,.T.);
#37197=ORIENTED_EDGE('',*,*,#26345,.F.);
#37198=ORIENTED_EDGE('',*,*,#24371,.F.);
#37199=ORIENTED_EDGE('',*,*,#26348,.T.);
#37200=ORIENTED_EDGE('',*,*,#23257,.T.);
#37201=ORIENTED_EDGE('',*,*,#26347,.F.);
#37202=ORIENTED_EDGE('',*,*,#24376,.F.);
#37203=ORIENTED_EDGE('',*,*,#26349,.T.);
#37204=ORIENTED_EDGE('',*,*,#23258,.T.);
#37205=ORIENTED_EDGE('',*,*,#26348,.F.);
#37206=ORIENTED_EDGE('',*,*,#24375,.F.);
#37207=ORIENTED_EDGE('',*,*,#26350,.T.);
#37208=ORIENTED_EDGE('',*,*,#23259,.T.);
#37209=ORIENTED_EDGE('',*,*,#26349,.F.);
#37210=ORIENTED_EDGE('',*,*,#24374,.F.);
#37211=ORIENTED_EDGE('',*,*,#26346,.T.);
#37212=ORIENTED_EDGE('',*,*,#23260,.T.);
#37213=ORIENTED_EDGE('',*,*,#26350,.F.);
#37214=ORIENTED_EDGE('',*,*,#24373,.F.);
#37215=ORIENTED_EDGE('',*,*,#26351,.T.);
#37216=ORIENTED_EDGE('',*,*,#23249,.T.);
#37217=ORIENTED_EDGE('',*,*,#26352,.F.);
#37218=ORIENTED_EDGE('',*,*,#24366,.F.);
#37219=ORIENTED_EDGE('',*,*,#26353,.T.);
#37220=ORIENTED_EDGE('',*,*,#23250,.T.);
#37221=ORIENTED_EDGE('',*,*,#26351,.F.);
#37222=ORIENTED_EDGE('',*,*,#24365,.F.);
#37223=ORIENTED_EDGE('',*,*,#26354,.T.);
#37224=ORIENTED_EDGE('',*,*,#23251,.T.);
#37225=ORIENTED_EDGE('',*,*,#26353,.F.);
#37226=ORIENTED_EDGE('',*,*,#24370,.F.);
#37227=ORIENTED_EDGE('',*,*,#26355,.T.);
#37228=ORIENTED_EDGE('',*,*,#23252,.T.);
#37229=ORIENTED_EDGE('',*,*,#26354,.F.);
#37230=ORIENTED_EDGE('',*,*,#24369,.F.);
#37231=ORIENTED_EDGE('',*,*,#26356,.T.);
#37232=ORIENTED_EDGE('',*,*,#23253,.T.);
#37233=ORIENTED_EDGE('',*,*,#26355,.F.);
#37234=ORIENTED_EDGE('',*,*,#24368,.F.);
#37235=ORIENTED_EDGE('',*,*,#26352,.T.);
#37236=ORIENTED_EDGE('',*,*,#23254,.T.);
#37237=ORIENTED_EDGE('',*,*,#26356,.F.);
#37238=ORIENTED_EDGE('',*,*,#24367,.F.);
#37239=ORIENTED_EDGE('',*,*,#26357,.T.);
#37240=ORIENTED_EDGE('',*,*,#23243,.T.);
#37241=ORIENTED_EDGE('',*,*,#26358,.F.);
#37242=ORIENTED_EDGE('',*,*,#24360,.F.);
#37243=ORIENTED_EDGE('',*,*,#26359,.T.);
#37244=ORIENTED_EDGE('',*,*,#23244,.T.);
#37245=ORIENTED_EDGE('',*,*,#26357,.F.);
#37246=ORIENTED_EDGE('',*,*,#24359,.F.);
#37247=ORIENTED_EDGE('',*,*,#26360,.T.);
#37248=ORIENTED_EDGE('',*,*,#23245,.T.);
#37249=ORIENTED_EDGE('',*,*,#26359,.F.);
#37250=ORIENTED_EDGE('',*,*,#24364,.F.);
#37251=ORIENTED_EDGE('',*,*,#26361,.T.);
#37252=ORIENTED_EDGE('',*,*,#23246,.T.);
#37253=ORIENTED_EDGE('',*,*,#26360,.F.);
#37254=ORIENTED_EDGE('',*,*,#24363,.F.);
#37255=ORIENTED_EDGE('',*,*,#26362,.T.);
#37256=ORIENTED_EDGE('',*,*,#23247,.T.);
#37257=ORIENTED_EDGE('',*,*,#26361,.F.);
#37258=ORIENTED_EDGE('',*,*,#24362,.F.);
#37259=ORIENTED_EDGE('',*,*,#26358,.T.);
#37260=ORIENTED_EDGE('',*,*,#23248,.T.);
#37261=ORIENTED_EDGE('',*,*,#26362,.F.);
#37262=ORIENTED_EDGE('',*,*,#24361,.F.);
#37263=ORIENTED_EDGE('',*,*,#26363,.T.);
#37264=ORIENTED_EDGE('',*,*,#23237,.T.);
#37265=ORIENTED_EDGE('',*,*,#26364,.F.);
#37266=ORIENTED_EDGE('',*,*,#24354,.F.);
#37267=ORIENTED_EDGE('',*,*,#26365,.T.);
#37268=ORIENTED_EDGE('',*,*,#23238,.T.);
#37269=ORIENTED_EDGE('',*,*,#26363,.F.);
#37270=ORIENTED_EDGE('',*,*,#24353,.F.);
#37271=ORIENTED_EDGE('',*,*,#26366,.T.);
#37272=ORIENTED_EDGE('',*,*,#23239,.T.);
#37273=ORIENTED_EDGE('',*,*,#26365,.F.);
#37274=ORIENTED_EDGE('',*,*,#24358,.F.);
#37275=ORIENTED_EDGE('',*,*,#26367,.T.);
#37276=ORIENTED_EDGE('',*,*,#23240,.T.);
#37277=ORIENTED_EDGE('',*,*,#26366,.F.);
#37278=ORIENTED_EDGE('',*,*,#24357,.F.);
#37279=ORIENTED_EDGE('',*,*,#26368,.T.);
#37280=ORIENTED_EDGE('',*,*,#23241,.T.);
#37281=ORIENTED_EDGE('',*,*,#26367,.F.);
#37282=ORIENTED_EDGE('',*,*,#24356,.F.);
#37283=ORIENTED_EDGE('',*,*,#26364,.T.);
#37284=ORIENTED_EDGE('',*,*,#23242,.T.);
#37285=ORIENTED_EDGE('',*,*,#26368,.F.);
#37286=ORIENTED_EDGE('',*,*,#24355,.F.);
#37287=ORIENTED_EDGE('',*,*,#26369,.T.);
#37288=ORIENTED_EDGE('',*,*,#23231,.T.);
#37289=ORIENTED_EDGE('',*,*,#26370,.F.);
#37290=ORIENTED_EDGE('',*,*,#24348,.F.);
#37291=ORIENTED_EDGE('',*,*,#26371,.T.);
#37292=ORIENTED_EDGE('',*,*,#23232,.T.);
#37293=ORIENTED_EDGE('',*,*,#26369,.F.);
#37294=ORIENTED_EDGE('',*,*,#24347,.F.);
#37295=ORIENTED_EDGE('',*,*,#26372,.T.);
#37296=ORIENTED_EDGE('',*,*,#23233,.T.);
#37297=ORIENTED_EDGE('',*,*,#26371,.F.);
#37298=ORIENTED_EDGE('',*,*,#24352,.F.);
#37299=ORIENTED_EDGE('',*,*,#26373,.T.);
#37300=ORIENTED_EDGE('',*,*,#23234,.T.);
#37301=ORIENTED_EDGE('',*,*,#26372,.F.);
#37302=ORIENTED_EDGE('',*,*,#24351,.F.);
#37303=ORIENTED_EDGE('',*,*,#26374,.T.);
#37304=ORIENTED_EDGE('',*,*,#23235,.T.);
#37305=ORIENTED_EDGE('',*,*,#26373,.F.);
#37306=ORIENTED_EDGE('',*,*,#24350,.F.);
#37307=ORIENTED_EDGE('',*,*,#26370,.T.);
#37308=ORIENTED_EDGE('',*,*,#23236,.T.);
#37309=ORIENTED_EDGE('',*,*,#26374,.F.);
#37310=ORIENTED_EDGE('',*,*,#24349,.F.);
#37311=ORIENTED_EDGE('',*,*,#26375,.T.);
#37312=ORIENTED_EDGE('',*,*,#23225,.T.);
#37313=ORIENTED_EDGE('',*,*,#26376,.F.);
#37314=ORIENTED_EDGE('',*,*,#24342,.F.);
#37315=ORIENTED_EDGE('',*,*,#26377,.T.);
#37316=ORIENTED_EDGE('',*,*,#23226,.T.);
#37317=ORIENTED_EDGE('',*,*,#26375,.F.);
#37318=ORIENTED_EDGE('',*,*,#24341,.F.);
#37319=ORIENTED_EDGE('',*,*,#26378,.T.);
#37320=ORIENTED_EDGE('',*,*,#23227,.T.);
#37321=ORIENTED_EDGE('',*,*,#26377,.F.);
#37322=ORIENTED_EDGE('',*,*,#24346,.F.);
#37323=ORIENTED_EDGE('',*,*,#26379,.T.);
#37324=ORIENTED_EDGE('',*,*,#23228,.T.);
#37325=ORIENTED_EDGE('',*,*,#26378,.F.);
#37326=ORIENTED_EDGE('',*,*,#24345,.F.);
#37327=ORIENTED_EDGE('',*,*,#26380,.T.);
#37328=ORIENTED_EDGE('',*,*,#23229,.T.);
#37329=ORIENTED_EDGE('',*,*,#26379,.F.);
#37330=ORIENTED_EDGE('',*,*,#24344,.F.);
#37331=ORIENTED_EDGE('',*,*,#26376,.T.);
#37332=ORIENTED_EDGE('',*,*,#23230,.T.);
#37333=ORIENTED_EDGE('',*,*,#26380,.F.);
#37334=ORIENTED_EDGE('',*,*,#24343,.F.);
#37335=ORIENTED_EDGE('',*,*,#26381,.T.);
#37336=ORIENTED_EDGE('',*,*,#23219,.T.);
#37337=ORIENTED_EDGE('',*,*,#26382,.F.);
#37338=ORIENTED_EDGE('',*,*,#24336,.F.);
#37339=ORIENTED_EDGE('',*,*,#26383,.T.);
#37340=ORIENTED_EDGE('',*,*,#23220,.T.);
#37341=ORIENTED_EDGE('',*,*,#26381,.F.);
#37342=ORIENTED_EDGE('',*,*,#24335,.F.);
#37343=ORIENTED_EDGE('',*,*,#26384,.T.);
#37344=ORIENTED_EDGE('',*,*,#23221,.T.);
#37345=ORIENTED_EDGE('',*,*,#26383,.F.);
#37346=ORIENTED_EDGE('',*,*,#24340,.F.);
#37347=ORIENTED_EDGE('',*,*,#26385,.T.);
#37348=ORIENTED_EDGE('',*,*,#23222,.T.);
#37349=ORIENTED_EDGE('',*,*,#26384,.F.);
#37350=ORIENTED_EDGE('',*,*,#24339,.F.);
#37351=ORIENTED_EDGE('',*,*,#26386,.T.);
#37352=ORIENTED_EDGE('',*,*,#23223,.T.);
#37353=ORIENTED_EDGE('',*,*,#26385,.F.);
#37354=ORIENTED_EDGE('',*,*,#24338,.F.);
#37355=ORIENTED_EDGE('',*,*,#26382,.T.);
#37356=ORIENTED_EDGE('',*,*,#23224,.T.);
#37357=ORIENTED_EDGE('',*,*,#26386,.F.);
#37358=ORIENTED_EDGE('',*,*,#24337,.F.);
#37359=ORIENTED_EDGE('',*,*,#26387,.T.);
#37360=ORIENTED_EDGE('',*,*,#23213,.T.);
#37361=ORIENTED_EDGE('',*,*,#26388,.F.);
#37362=ORIENTED_EDGE('',*,*,#24330,.F.);
#37363=ORIENTED_EDGE('',*,*,#26389,.T.);
#37364=ORIENTED_EDGE('',*,*,#23214,.T.);
#37365=ORIENTED_EDGE('',*,*,#26387,.F.);
#37366=ORIENTED_EDGE('',*,*,#24329,.F.);
#37367=ORIENTED_EDGE('',*,*,#26390,.T.);
#37368=ORIENTED_EDGE('',*,*,#23215,.T.);
#37369=ORIENTED_EDGE('',*,*,#26389,.F.);
#37370=ORIENTED_EDGE('',*,*,#24334,.F.);
#37371=ORIENTED_EDGE('',*,*,#26391,.T.);
#37372=ORIENTED_EDGE('',*,*,#23216,.T.);
#37373=ORIENTED_EDGE('',*,*,#26390,.F.);
#37374=ORIENTED_EDGE('',*,*,#24333,.F.);
#37375=ORIENTED_EDGE('',*,*,#26392,.T.);
#37376=ORIENTED_EDGE('',*,*,#23217,.T.);
#37377=ORIENTED_EDGE('',*,*,#26391,.F.);
#37378=ORIENTED_EDGE('',*,*,#24332,.F.);
#37379=ORIENTED_EDGE('',*,*,#26388,.T.);
#37380=ORIENTED_EDGE('',*,*,#23218,.T.);
#37381=ORIENTED_EDGE('',*,*,#26392,.F.);
#37382=ORIENTED_EDGE('',*,*,#24331,.F.);
#37383=ORIENTED_EDGE('',*,*,#26393,.T.);
#37384=ORIENTED_EDGE('',*,*,#23207,.T.);
#37385=ORIENTED_EDGE('',*,*,#26394,.F.);
#37386=ORIENTED_EDGE('',*,*,#24324,.F.);
#37387=ORIENTED_EDGE('',*,*,#26395,.T.);
#37388=ORIENTED_EDGE('',*,*,#23208,.T.);
#37389=ORIENTED_EDGE('',*,*,#26393,.F.);
#37390=ORIENTED_EDGE('',*,*,#24323,.F.);
#37391=ORIENTED_EDGE('',*,*,#26396,.T.);
#37392=ORIENTED_EDGE('',*,*,#23209,.T.);
#37393=ORIENTED_EDGE('',*,*,#26395,.F.);
#37394=ORIENTED_EDGE('',*,*,#24328,.F.);
#37395=ORIENTED_EDGE('',*,*,#26397,.T.);
#37396=ORIENTED_EDGE('',*,*,#23210,.T.);
#37397=ORIENTED_EDGE('',*,*,#26396,.F.);
#37398=ORIENTED_EDGE('',*,*,#24327,.F.);
#37399=ORIENTED_EDGE('',*,*,#26398,.T.);
#37400=ORIENTED_EDGE('',*,*,#23211,.T.);
#37401=ORIENTED_EDGE('',*,*,#26397,.F.);
#37402=ORIENTED_EDGE('',*,*,#24326,.F.);
#37403=ORIENTED_EDGE('',*,*,#26394,.T.);
#37404=ORIENTED_EDGE('',*,*,#23212,.T.);
#37405=ORIENTED_EDGE('',*,*,#26398,.F.);
#37406=ORIENTED_EDGE('',*,*,#24325,.F.);
#37407=ORIENTED_EDGE('',*,*,#26399,.T.);
#37408=ORIENTED_EDGE('',*,*,#23201,.T.);
#37409=ORIENTED_EDGE('',*,*,#26400,.F.);
#37410=ORIENTED_EDGE('',*,*,#24318,.F.);
#37411=ORIENTED_EDGE('',*,*,#26401,.T.);
#37412=ORIENTED_EDGE('',*,*,#23202,.T.);
#37413=ORIENTED_EDGE('',*,*,#26399,.F.);
#37414=ORIENTED_EDGE('',*,*,#24317,.F.);
#37415=ORIENTED_EDGE('',*,*,#26402,.T.);
#37416=ORIENTED_EDGE('',*,*,#23203,.T.);
#37417=ORIENTED_EDGE('',*,*,#26401,.F.);
#37418=ORIENTED_EDGE('',*,*,#24322,.F.);
#37419=ORIENTED_EDGE('',*,*,#26403,.T.);
#37420=ORIENTED_EDGE('',*,*,#23204,.T.);
#37421=ORIENTED_EDGE('',*,*,#26402,.F.);
#37422=ORIENTED_EDGE('',*,*,#24321,.F.);
#37423=ORIENTED_EDGE('',*,*,#26404,.T.);
#37424=ORIENTED_EDGE('',*,*,#23205,.T.);
#37425=ORIENTED_EDGE('',*,*,#26403,.F.);
#37426=ORIENTED_EDGE('',*,*,#24320,.F.);
#37427=ORIENTED_EDGE('',*,*,#26400,.T.);
#37428=ORIENTED_EDGE('',*,*,#23206,.T.);
#37429=ORIENTED_EDGE('',*,*,#26404,.F.);
#37430=ORIENTED_EDGE('',*,*,#24319,.F.);
#37431=ORIENTED_EDGE('',*,*,#26405,.T.);
#37432=ORIENTED_EDGE('',*,*,#23195,.T.);
#37433=ORIENTED_EDGE('',*,*,#26406,.F.);
#37434=ORIENTED_EDGE('',*,*,#24312,.F.);
#37435=ORIENTED_EDGE('',*,*,#26407,.T.);
#37436=ORIENTED_EDGE('',*,*,#23196,.T.);
#37437=ORIENTED_EDGE('',*,*,#26405,.F.);
#37438=ORIENTED_EDGE('',*,*,#24311,.F.);
#37439=ORIENTED_EDGE('',*,*,#26408,.T.);
#37440=ORIENTED_EDGE('',*,*,#23197,.T.);
#37441=ORIENTED_EDGE('',*,*,#26407,.F.);
#37442=ORIENTED_EDGE('',*,*,#24316,.F.);
#37443=ORIENTED_EDGE('',*,*,#26409,.T.);
#37444=ORIENTED_EDGE('',*,*,#23198,.T.);
#37445=ORIENTED_EDGE('',*,*,#26408,.F.);
#37446=ORIENTED_EDGE('',*,*,#24315,.F.);
#37447=ORIENTED_EDGE('',*,*,#26410,.T.);
#37448=ORIENTED_EDGE('',*,*,#23199,.T.);
#37449=ORIENTED_EDGE('',*,*,#26409,.F.);
#37450=ORIENTED_EDGE('',*,*,#24314,.F.);
#37451=ORIENTED_EDGE('',*,*,#26406,.T.);
#37452=ORIENTED_EDGE('',*,*,#23200,.T.);
#37453=ORIENTED_EDGE('',*,*,#26410,.F.);
#37454=ORIENTED_EDGE('',*,*,#24313,.F.);
#37455=ORIENTED_EDGE('',*,*,#26411,.T.);
#37456=ORIENTED_EDGE('',*,*,#23189,.T.);
#37457=ORIENTED_EDGE('',*,*,#26412,.F.);
#37458=ORIENTED_EDGE('',*,*,#24306,.F.);
#37459=ORIENTED_EDGE('',*,*,#26413,.T.);
#37460=ORIENTED_EDGE('',*,*,#23190,.T.);
#37461=ORIENTED_EDGE('',*,*,#26411,.F.);
#37462=ORIENTED_EDGE('',*,*,#24305,.F.);
#37463=ORIENTED_EDGE('',*,*,#26414,.T.);
#37464=ORIENTED_EDGE('',*,*,#23191,.T.);
#37465=ORIENTED_EDGE('',*,*,#26413,.F.);
#37466=ORIENTED_EDGE('',*,*,#24310,.F.);
#37467=ORIENTED_EDGE('',*,*,#26415,.T.);
#37468=ORIENTED_EDGE('',*,*,#23192,.T.);
#37469=ORIENTED_EDGE('',*,*,#26414,.F.);
#37470=ORIENTED_EDGE('',*,*,#24309,.F.);
#37471=ORIENTED_EDGE('',*,*,#26416,.T.);
#37472=ORIENTED_EDGE('',*,*,#23193,.T.);
#37473=ORIENTED_EDGE('',*,*,#26415,.F.);
#37474=ORIENTED_EDGE('',*,*,#24308,.F.);
#37475=ORIENTED_EDGE('',*,*,#26412,.T.);
#37476=ORIENTED_EDGE('',*,*,#23194,.T.);
#37477=ORIENTED_EDGE('',*,*,#26416,.F.);
#37478=ORIENTED_EDGE('',*,*,#24307,.F.);
#37479=ORIENTED_EDGE('',*,*,#26417,.T.);
#37480=ORIENTED_EDGE('',*,*,#23183,.T.);
#37481=ORIENTED_EDGE('',*,*,#26418,.F.);
#37482=ORIENTED_EDGE('',*,*,#24300,.F.);
#37483=ORIENTED_EDGE('',*,*,#26419,.T.);
#37484=ORIENTED_EDGE('',*,*,#23184,.T.);
#37485=ORIENTED_EDGE('',*,*,#26417,.F.);
#37486=ORIENTED_EDGE('',*,*,#24299,.F.);
#37487=ORIENTED_EDGE('',*,*,#26420,.T.);
#37488=ORIENTED_EDGE('',*,*,#23185,.T.);
#37489=ORIENTED_EDGE('',*,*,#26419,.F.);
#37490=ORIENTED_EDGE('',*,*,#24304,.F.);
#37491=ORIENTED_EDGE('',*,*,#26421,.T.);
#37492=ORIENTED_EDGE('',*,*,#23186,.T.);
#37493=ORIENTED_EDGE('',*,*,#26420,.F.);
#37494=ORIENTED_EDGE('',*,*,#24303,.F.);
#37495=ORIENTED_EDGE('',*,*,#26422,.T.);
#37496=ORIENTED_EDGE('',*,*,#23187,.T.);
#37497=ORIENTED_EDGE('',*,*,#26421,.F.);
#37498=ORIENTED_EDGE('',*,*,#24302,.F.);
#37499=ORIENTED_EDGE('',*,*,#26418,.T.);
#37500=ORIENTED_EDGE('',*,*,#23188,.T.);
#37501=ORIENTED_EDGE('',*,*,#26422,.F.);
#37502=ORIENTED_EDGE('',*,*,#24301,.F.);
#37503=ORIENTED_EDGE('',*,*,#26423,.T.);
#37504=ORIENTED_EDGE('',*,*,#23177,.T.);
#37505=ORIENTED_EDGE('',*,*,#26424,.F.);
#37506=ORIENTED_EDGE('',*,*,#24294,.F.);
#37507=ORIENTED_EDGE('',*,*,#26425,.T.);
#37508=ORIENTED_EDGE('',*,*,#23178,.T.);
#37509=ORIENTED_EDGE('',*,*,#26423,.F.);
#37510=ORIENTED_EDGE('',*,*,#24293,.F.);
#37511=ORIENTED_EDGE('',*,*,#26426,.T.);
#37512=ORIENTED_EDGE('',*,*,#23179,.T.);
#37513=ORIENTED_EDGE('',*,*,#26425,.F.);
#37514=ORIENTED_EDGE('',*,*,#24298,.F.);
#37515=ORIENTED_EDGE('',*,*,#26427,.T.);
#37516=ORIENTED_EDGE('',*,*,#23180,.T.);
#37517=ORIENTED_EDGE('',*,*,#26426,.F.);
#37518=ORIENTED_EDGE('',*,*,#24297,.F.);
#37519=ORIENTED_EDGE('',*,*,#26428,.T.);
#37520=ORIENTED_EDGE('',*,*,#23181,.T.);
#37521=ORIENTED_EDGE('',*,*,#26427,.F.);
#37522=ORIENTED_EDGE('',*,*,#24296,.F.);
#37523=ORIENTED_EDGE('',*,*,#26424,.T.);
#37524=ORIENTED_EDGE('',*,*,#23182,.T.);
#37525=ORIENTED_EDGE('',*,*,#26428,.F.);
#37526=ORIENTED_EDGE('',*,*,#24295,.F.);
#37527=ORIENTED_EDGE('',*,*,#26429,.T.);
#37528=ORIENTED_EDGE('',*,*,#23171,.T.);
#37529=ORIENTED_EDGE('',*,*,#26430,.F.);
#37530=ORIENTED_EDGE('',*,*,#24288,.F.);
#37531=ORIENTED_EDGE('',*,*,#26431,.T.);
#37532=ORIENTED_EDGE('',*,*,#23172,.T.);
#37533=ORIENTED_EDGE('',*,*,#26429,.F.);
#37534=ORIENTED_EDGE('',*,*,#24287,.F.);
#37535=ORIENTED_EDGE('',*,*,#26432,.T.);
#37536=ORIENTED_EDGE('',*,*,#23173,.T.);
#37537=ORIENTED_EDGE('',*,*,#26431,.F.);
#37538=ORIENTED_EDGE('',*,*,#24292,.F.);
#37539=ORIENTED_EDGE('',*,*,#26433,.T.);
#37540=ORIENTED_EDGE('',*,*,#23174,.T.);
#37541=ORIENTED_EDGE('',*,*,#26432,.F.);
#37542=ORIENTED_EDGE('',*,*,#24291,.F.);
#37543=ORIENTED_EDGE('',*,*,#26434,.T.);
#37544=ORIENTED_EDGE('',*,*,#23175,.T.);
#37545=ORIENTED_EDGE('',*,*,#26433,.F.);
#37546=ORIENTED_EDGE('',*,*,#24290,.F.);
#37547=ORIENTED_EDGE('',*,*,#26430,.T.);
#37548=ORIENTED_EDGE('',*,*,#23176,.T.);
#37549=ORIENTED_EDGE('',*,*,#26434,.F.);
#37550=ORIENTED_EDGE('',*,*,#24289,.F.);
#37551=ORIENTED_EDGE('',*,*,#26435,.T.);
#37552=ORIENTED_EDGE('',*,*,#23165,.T.);
#37553=ORIENTED_EDGE('',*,*,#26436,.F.);
#37554=ORIENTED_EDGE('',*,*,#24282,.F.);
#37555=ORIENTED_EDGE('',*,*,#26437,.T.);
#37556=ORIENTED_EDGE('',*,*,#23166,.T.);
#37557=ORIENTED_EDGE('',*,*,#26435,.F.);
#37558=ORIENTED_EDGE('',*,*,#24281,.F.);
#37559=ORIENTED_EDGE('',*,*,#26438,.T.);
#37560=ORIENTED_EDGE('',*,*,#23167,.T.);
#37561=ORIENTED_EDGE('',*,*,#26437,.F.);
#37562=ORIENTED_EDGE('',*,*,#24286,.F.);
#37563=ORIENTED_EDGE('',*,*,#26439,.T.);
#37564=ORIENTED_EDGE('',*,*,#23168,.T.);
#37565=ORIENTED_EDGE('',*,*,#26438,.F.);
#37566=ORIENTED_EDGE('',*,*,#24285,.F.);
#37567=ORIENTED_EDGE('',*,*,#26440,.T.);
#37568=ORIENTED_EDGE('',*,*,#23169,.T.);
#37569=ORIENTED_EDGE('',*,*,#26439,.F.);
#37570=ORIENTED_EDGE('',*,*,#24284,.F.);
#37571=ORIENTED_EDGE('',*,*,#26436,.T.);
#37572=ORIENTED_EDGE('',*,*,#23170,.T.);
#37573=ORIENTED_EDGE('',*,*,#26440,.F.);
#37574=ORIENTED_EDGE('',*,*,#24283,.F.);
#37575=ORIENTED_EDGE('',*,*,#26441,.T.);
#37576=ORIENTED_EDGE('',*,*,#23159,.T.);
#37577=ORIENTED_EDGE('',*,*,#26442,.F.);
#37578=ORIENTED_EDGE('',*,*,#24276,.F.);
#37579=ORIENTED_EDGE('',*,*,#26443,.T.);
#37580=ORIENTED_EDGE('',*,*,#23160,.T.);
#37581=ORIENTED_EDGE('',*,*,#26441,.F.);
#37582=ORIENTED_EDGE('',*,*,#24275,.F.);
#37583=ORIENTED_EDGE('',*,*,#26444,.T.);
#37584=ORIENTED_EDGE('',*,*,#23161,.T.);
#37585=ORIENTED_EDGE('',*,*,#26443,.F.);
#37586=ORIENTED_EDGE('',*,*,#24280,.F.);
#37587=ORIENTED_EDGE('',*,*,#26445,.T.);
#37588=ORIENTED_EDGE('',*,*,#23162,.T.);
#37589=ORIENTED_EDGE('',*,*,#26444,.F.);
#37590=ORIENTED_EDGE('',*,*,#24279,.F.);
#37591=ORIENTED_EDGE('',*,*,#26446,.T.);
#37592=ORIENTED_EDGE('',*,*,#23163,.T.);
#37593=ORIENTED_EDGE('',*,*,#26445,.F.);
#37594=ORIENTED_EDGE('',*,*,#24278,.F.);
#37595=ORIENTED_EDGE('',*,*,#26442,.T.);
#37596=ORIENTED_EDGE('',*,*,#23164,.T.);
#37597=ORIENTED_EDGE('',*,*,#26446,.F.);
#37598=ORIENTED_EDGE('',*,*,#24277,.F.);
#37599=ORIENTED_EDGE('',*,*,#26447,.T.);
#37600=ORIENTED_EDGE('',*,*,#23153,.T.);
#37601=ORIENTED_EDGE('',*,*,#26448,.F.);
#37602=ORIENTED_EDGE('',*,*,#24270,.F.);
#37603=ORIENTED_EDGE('',*,*,#26449,.T.);
#37604=ORIENTED_EDGE('',*,*,#23154,.T.);
#37605=ORIENTED_EDGE('',*,*,#26447,.F.);
#37606=ORIENTED_EDGE('',*,*,#24269,.F.);
#37607=ORIENTED_EDGE('',*,*,#26450,.T.);
#37608=ORIENTED_EDGE('',*,*,#23155,.T.);
#37609=ORIENTED_EDGE('',*,*,#26449,.F.);
#37610=ORIENTED_EDGE('',*,*,#24274,.F.);
#37611=ORIENTED_EDGE('',*,*,#26451,.T.);
#37612=ORIENTED_EDGE('',*,*,#23156,.T.);
#37613=ORIENTED_EDGE('',*,*,#26450,.F.);
#37614=ORIENTED_EDGE('',*,*,#24273,.F.);
#37615=ORIENTED_EDGE('',*,*,#26452,.T.);
#37616=ORIENTED_EDGE('',*,*,#23157,.T.);
#37617=ORIENTED_EDGE('',*,*,#26451,.F.);
#37618=ORIENTED_EDGE('',*,*,#24272,.F.);
#37619=ORIENTED_EDGE('',*,*,#26448,.T.);
#37620=ORIENTED_EDGE('',*,*,#23158,.T.);
#37621=ORIENTED_EDGE('',*,*,#26452,.F.);
#37622=ORIENTED_EDGE('',*,*,#24271,.F.);
#37623=ORIENTED_EDGE('',*,*,#26453,.T.);
#37624=ORIENTED_EDGE('',*,*,#23147,.T.);
#37625=ORIENTED_EDGE('',*,*,#26454,.F.);
#37626=ORIENTED_EDGE('',*,*,#24264,.F.);
#37627=ORIENTED_EDGE('',*,*,#26455,.T.);
#37628=ORIENTED_EDGE('',*,*,#23148,.T.);
#37629=ORIENTED_EDGE('',*,*,#26453,.F.);
#37630=ORIENTED_EDGE('',*,*,#24263,.F.);
#37631=ORIENTED_EDGE('',*,*,#26456,.T.);
#37632=ORIENTED_EDGE('',*,*,#23149,.T.);
#37633=ORIENTED_EDGE('',*,*,#26455,.F.);
#37634=ORIENTED_EDGE('',*,*,#24268,.F.);
#37635=ORIENTED_EDGE('',*,*,#26457,.T.);
#37636=ORIENTED_EDGE('',*,*,#23150,.T.);
#37637=ORIENTED_EDGE('',*,*,#26456,.F.);
#37638=ORIENTED_EDGE('',*,*,#24267,.F.);
#37639=ORIENTED_EDGE('',*,*,#26458,.T.);
#37640=ORIENTED_EDGE('',*,*,#23151,.T.);
#37641=ORIENTED_EDGE('',*,*,#26457,.F.);
#37642=ORIENTED_EDGE('',*,*,#24266,.F.);
#37643=ORIENTED_EDGE('',*,*,#26454,.T.);
#37644=ORIENTED_EDGE('',*,*,#23152,.T.);
#37645=ORIENTED_EDGE('',*,*,#26458,.F.);
#37646=ORIENTED_EDGE('',*,*,#24265,.F.);
#37647=ORIENTED_EDGE('',*,*,#26459,.T.);
#37648=ORIENTED_EDGE('',*,*,#23141,.T.);
#37649=ORIENTED_EDGE('',*,*,#26460,.F.);
#37650=ORIENTED_EDGE('',*,*,#24258,.F.);
#37651=ORIENTED_EDGE('',*,*,#26461,.T.);
#37652=ORIENTED_EDGE('',*,*,#23142,.T.);
#37653=ORIENTED_EDGE('',*,*,#26459,.F.);
#37654=ORIENTED_EDGE('',*,*,#24257,.F.);
#37655=ORIENTED_EDGE('',*,*,#26462,.T.);
#37656=ORIENTED_EDGE('',*,*,#23143,.T.);
#37657=ORIENTED_EDGE('',*,*,#26461,.F.);
#37658=ORIENTED_EDGE('',*,*,#24262,.F.);
#37659=ORIENTED_EDGE('',*,*,#26463,.T.);
#37660=ORIENTED_EDGE('',*,*,#23144,.T.);
#37661=ORIENTED_EDGE('',*,*,#26462,.F.);
#37662=ORIENTED_EDGE('',*,*,#24261,.F.);
#37663=ORIENTED_EDGE('',*,*,#26464,.T.);
#37664=ORIENTED_EDGE('',*,*,#23145,.T.);
#37665=ORIENTED_EDGE('',*,*,#26463,.F.);
#37666=ORIENTED_EDGE('',*,*,#24260,.F.);
#37667=ORIENTED_EDGE('',*,*,#26460,.T.);
#37668=ORIENTED_EDGE('',*,*,#23146,.T.);
#37669=ORIENTED_EDGE('',*,*,#26464,.F.);
#37670=ORIENTED_EDGE('',*,*,#24259,.F.);
#37671=ORIENTED_EDGE('',*,*,#26465,.T.);
#37672=ORIENTED_EDGE('',*,*,#23135,.T.);
#37673=ORIENTED_EDGE('',*,*,#26466,.F.);
#37674=ORIENTED_EDGE('',*,*,#24252,.F.);
#37675=ORIENTED_EDGE('',*,*,#26467,.T.);
#37676=ORIENTED_EDGE('',*,*,#23136,.T.);
#37677=ORIENTED_EDGE('',*,*,#26465,.F.);
#37678=ORIENTED_EDGE('',*,*,#24251,.F.);
#37679=ORIENTED_EDGE('',*,*,#26468,.T.);
#37680=ORIENTED_EDGE('',*,*,#23137,.T.);
#37681=ORIENTED_EDGE('',*,*,#26467,.F.);
#37682=ORIENTED_EDGE('',*,*,#24256,.F.);
#37683=ORIENTED_EDGE('',*,*,#26469,.T.);
#37684=ORIENTED_EDGE('',*,*,#23138,.T.);
#37685=ORIENTED_EDGE('',*,*,#26468,.F.);
#37686=ORIENTED_EDGE('',*,*,#24255,.F.);
#37687=ORIENTED_EDGE('',*,*,#26470,.T.);
#37688=ORIENTED_EDGE('',*,*,#23139,.T.);
#37689=ORIENTED_EDGE('',*,*,#26469,.F.);
#37690=ORIENTED_EDGE('',*,*,#24254,.F.);
#37691=ORIENTED_EDGE('',*,*,#26466,.T.);
#37692=ORIENTED_EDGE('',*,*,#23140,.T.);
#37693=ORIENTED_EDGE('',*,*,#26470,.F.);
#37694=ORIENTED_EDGE('',*,*,#24253,.F.);
#37695=ORIENTED_EDGE('',*,*,#26471,.T.);
#37696=ORIENTED_EDGE('',*,*,#23129,.T.);
#37697=ORIENTED_EDGE('',*,*,#26472,.F.);
#37698=ORIENTED_EDGE('',*,*,#24246,.F.);
#37699=ORIENTED_EDGE('',*,*,#26473,.T.);
#37700=ORIENTED_EDGE('',*,*,#23130,.T.);
#37701=ORIENTED_EDGE('',*,*,#26471,.F.);
#37702=ORIENTED_EDGE('',*,*,#24245,.F.);
#37703=ORIENTED_EDGE('',*,*,#26474,.T.);
#37704=ORIENTED_EDGE('',*,*,#23131,.T.);
#37705=ORIENTED_EDGE('',*,*,#26473,.F.);
#37706=ORIENTED_EDGE('',*,*,#24250,.F.);
#37707=ORIENTED_EDGE('',*,*,#26475,.T.);
#37708=ORIENTED_EDGE('',*,*,#23132,.T.);
#37709=ORIENTED_EDGE('',*,*,#26474,.F.);
#37710=ORIENTED_EDGE('',*,*,#24249,.F.);
#37711=ORIENTED_EDGE('',*,*,#26476,.T.);
#37712=ORIENTED_EDGE('',*,*,#23133,.T.);
#37713=ORIENTED_EDGE('',*,*,#26475,.F.);
#37714=ORIENTED_EDGE('',*,*,#24248,.F.);
#37715=ORIENTED_EDGE('',*,*,#26472,.T.);
#37716=ORIENTED_EDGE('',*,*,#23134,.T.);
#37717=ORIENTED_EDGE('',*,*,#26476,.F.);
#37718=ORIENTED_EDGE('',*,*,#24247,.F.);
#38007=CYLINDRICAL_SURFACE('',#41338,1.6);
#38008=CYLINDRICAL_SURFACE('',#41339,0.799999999999995);
#38009=CYLINDRICAL_SURFACE('',#41346,1.6);
#38010=CYLINDRICAL_SURFACE('',#41347,0.799999999999995);
#38011=CYLINDRICAL_SURFACE('',#41348,5.);
#38012=CYLINDRICAL_SURFACE('',#41352,5.);
#38013=CYLINDRICAL_SURFACE('',#41368,1.6);
#38014=CYLINDRICAL_SURFACE('',#41369,0.799999999999995);
#38015=CYLINDRICAL_SURFACE('',#41376,1.6);
#38016=CYLINDRICAL_SURFACE('',#41377,0.799999999999995);
#38017=CYLINDRICAL_SURFACE('',#41378,5.);
#38018=CYLINDRICAL_SURFACE('',#41382,5.);
#38765=ADVANCED_FACE('',(#3077),#2189,.F.);
#38766=ADVANCED_FACE('',(#3078),#2190,.F.);
#38767=ADVANCED_FACE('',(#3079),#2191,.T.);
#38768=ADVANCED_FACE('',(#3080),#2192,.T.);
#38769=ADVANCED_FACE('',(#3081,#255),#1029,.T.);
#38770=ADVANCED_FACE('',(#3082,#256),#1030,.F.);
#38771=ADVANCED_FACE('',(#3083),#1031,.T.);
#38772=ADVANCED_FACE('',(#3084),#1032,.T.);
#38773=ADVANCED_FACE('',(#3085),#1033,.F.);
#38774=ADVANCED_FACE('',(#3086),#1034,.T.);
#38775=ADVANCED_FACE('',(#3087),#1035,.F.);
#38776=ADVANCED_FACE('',(#3088),#1036,.T.);
#38777=ADVANCED_FACE('',(#3089),#1037,.T.);
#38778=ADVANCED_FACE('',(#3090),#1038,.F.);
#38779=ADVANCED_FACE('',(#3091),#1039,.T.);
#38780=ADVANCED_FACE('',(#3092),#1040,.T.);
#38781=ADVANCED_FACE('',(#3093),#38007,.T.);
#38782=ADVANCED_FACE('',(#3094),#38008,.F.);
#38783=ADVANCED_FACE('',(#3095),#1041,.T.);
#38784=ADVANCED_FACE('',(#3096),#1042,.T.);
#38785=ADVANCED_FACE('',(#3097),#38009,.T.);
#38786=ADVANCED_FACE('',(#3098),#38010,.F.);
#38787=ADVANCED_FACE('',(#3099),#38011,.T.);
#38788=ADVANCED_FACE('',(#3100),#1043,.F.);
#38789=ADVANCED_FACE('',(#3101),#38012,.T.);
#38790=ADVANCED_FACE('',(#3102),#1044,.F.);
#38791=ADVANCED_FACE('',(#3103),#1045,.F.);
#38792=ADVANCED_FACE('',(#3104),#1046,.F.);
#38793=ADVANCED_FACE('',(#3105),#1047,.T.);
#38794=ADVANCED_FACE('',(#3106),#1048,.T.);
#38795=ADVANCED_FACE('',(#3107),#1049,.T.);
#38796=ADVANCED_FACE('',(#3108),#1050,.T.);
#38797=ADVANCED_FACE('',(#3109),#1051,.T.);
#38798=ADVANCED_FACE('',(#3110),#1052,.T.);
#38799=ADVANCED_FACE('',(#3111),#38013,.T.);
#38800=ADVANCED_FACE('',(#3112),#38014,.F.);
#38801=ADVANCED_FACE('',(#3113),#1053,.T.);
#38802=ADVANCED_FACE('',(#3114),#1054,.T.);
#38803=ADVANCED_FACE('',(#3115),#38015,.T.);
#38804=ADVANCED_FACE('',(#3116),#38016,.F.);
#38805=ADVANCED_FACE('',(#3117),#38017,.T.);
#38806=ADVANCED_FACE('',(#3118),#1055,.T.);
#38807=ADVANCED_FACE('',(#3119),#38018,.T.);
#38808=ADVANCED_FACE('',(#3120),#1056,.F.);
#38809=ADVANCED_FACE('',(#3121),#1057,.F.);
#38810=ADVANCED_FACE('',(#3122),#1058,.F.);
#38811=ADVANCED_FACE('',(#3123),#1059,.T.);
#38812=ADVANCED_FACE('',(#3124),#1060,.T.);
#38813=ADVANCED_FACE('',(#3125),#1061,.F.);
#38814=ADVANCED_FACE('',(#3126),#1062,.T.);
#38815=ADVANCED_FACE('',(#3127,#257,#258,#259,#260,#261,#262,#263,#264,
#265,#266,#267,#268,#269,#270,#271,#272,#273,#274,#275,#276,#277,#278,#279,
#280,#281,#282,#283,#284,#285,#286,#287,#288,#289,#290,#291,#292,#293,#294,
#295,#296,#297,#298,#299,#300,#301,#302,#303,#304,#305,#306,#307,#308,#309,
#310,#311,#312,#313,#314,#315,#316,#317,#318,#319,#320,#321,#322,#323,#324,
#325,#326,#327,#328,#329,#330,#331,#332,#333,#334,#335,#336,#337,#338,#339,
#340,#341,#342,#343,#344,#345,#346,#347,#348,#349,#350,#351,#352,#353,#354,
#355,#356,#357,#358,#359,#360,#361,#362,#363,#364,#365,#366,#367,#368,#369,
#370,#371,#372,#373,#374,#375,#376,#377,#378,#379,#380,#381,#382,#383,#384,
#385,#386,#387,#388,#389,#390,#391,#392,#393,#394,#395,#396,#397,#398,#399,
#400,#401,#402,#403,#404,#405,#406,#407,#408,#409,#410,#411,#412,#413,#414,
#415,#416,#417,#418,#419,#420,#421,#422,#423,#424,#425,#426,#427,#428,#429,
#430,#431,#432,#433,#434,#435,#436,#437,#438,#439,#440,#441,#442),#1063,
 .T.);
#38816=ADVANCED_FACE('',(#3128,#443,#444,#445,#446,#447,#448,#449,#450,
#451,#452,#453,#454,#455,#456,#457,#458,#459,#460,#461,#462,#463,#464,#465,
#466,#467,#468,#469,#470,#471,#472,#473,#474,#475,#476,#477,#478,#479,#480,
#481,#482,#483,#484,#485,#486,#487,#488,#489,#490,#491,#492,#493,#494,#495,
#496,#497,#498,#499,#500,#501,#502,#503,#504,#505,#506,#507,#508,#509,#510,
#511,#512,#513,#514,#515,#516,#517,#518,#519,#520,#521,#522,#523,#524,#525,
#526,#527,#528,#529,#530,#531,#532,#533,#534,#535,#536,#537,#538,#539,#540,
#541,#542,#543,#544,#545,#546,#547,#548,#549,#550,#551,#552,#553,#554,#555,
#556,#557,#558,#559,#560,#561,#562,#563,#564,#565,#566,#567,#568,#569,#570,
#571,#572,#573,#574,#575,#576,#577,#578,#579,#580,#581,#582,#583,#584,#585,
#586,#587,#588,#589,#590,#591,#592,#593,#594,#595,#596,#597,#598,#599,#600,
#601,#602,#603,#604,#605,#606,#607,#608,#609,#610,#611,#612,#613,#614,#615,
#616,#617,#618,#619,#620,#621,#622,#623,#624,#625,#626,#627,#628),#1064,
 .F.);
#38817=ADVANCED_FACE('',(#3129),#1065,.F.);
#38818=ADVANCED_FACE('',(#3130),#1066,.F.);
#38819=ADVANCED_FACE('',(#3131),#1067,.F.);
#38820=ADVANCED_FACE('',(#3132),#1068,.F.);
#38821=ADVANCED_FACE('',(#3133),#1069,.F.);
#38822=ADVANCED_FACE('',(#3134),#1070,.F.);
#38823=ADVANCED_FACE('',(#3135),#1071,.F.);
#38824=ADVANCED_FACE('',(#3136),#1072,.F.);
#38825=ADVANCED_FACE('',(#3137),#1073,.F.);
#38826=ADVANCED_FACE('',(#3138),#1074,.F.);
#38827=ADVANCED_FACE('',(#3139),#1075,.F.);
#38828=ADVANCED_FACE('',(#3140),#1076,.F.);
#38829=ADVANCED_FACE('',(#3141),#1077,.F.);
#38830=ADVANCED_FACE('',(#3142),#1078,.F.);
#38831=ADVANCED_FACE('',(#3143),#1079,.F.);
#38832=ADVANCED_FACE('',(#3144),#1080,.F.);
#38833=ADVANCED_FACE('',(#3145),#1081,.F.);
#38834=ADVANCED_FACE('',(#3146),#1082,.F.);
#38835=ADVANCED_FACE('',(#3147),#1083,.F.);
#38836=ADVANCED_FACE('',(#3148),#1084,.F.);
#38837=ADVANCED_FACE('',(#3149),#1085,.F.);
#38838=ADVANCED_FACE('',(#3150),#1086,.F.);
#38839=ADVANCED_FACE('',(#3151),#1087,.F.);
#38840=ADVANCED_FACE('',(#3152),#1088,.F.);
#38841=ADVANCED_FACE('',(#3153),#1089,.F.);
#38842=ADVANCED_FACE('',(#3154),#1090,.F.);
#38843=ADVANCED_FACE('',(#3155),#1091,.F.);
#38844=ADVANCED_FACE('',(#3156),#1092,.F.);
#38845=ADVANCED_FACE('',(#3157),#1093,.F.);
#38846=ADVANCED_FACE('',(#3158),#1094,.F.);
#38847=ADVANCED_FACE('',(#3159),#1095,.F.);
#38848=ADVANCED_FACE('',(#3160),#1096,.F.);
#38849=ADVANCED_FACE('',(#3161),#1097,.F.);
#38850=ADVANCED_FACE('',(#3162),#1098,.F.);
#38851=ADVANCED_FACE('',(#3163),#1099,.F.);
#38852=ADVANCED_FACE('',(#3164),#1100,.F.);
#38853=ADVANCED_FACE('',(#3165),#1101,.F.);
#38854=ADVANCED_FACE('',(#3166),#1102,.F.);
#38855=ADVANCED_FACE('',(#3167),#1103,.F.);
#38856=ADVANCED_FACE('',(#3168),#1104,.F.);
#38857=ADVANCED_FACE('',(#3169),#1105,.F.);
#38858=ADVANCED_FACE('',(#3170),#1106,.F.);
#38859=ADVANCED_FACE('',(#3171),#1107,.F.);
#38860=ADVANCED_FACE('',(#3172),#1108,.F.);
#38861=ADVANCED_FACE('',(#3173),#1109,.F.);
#38862=ADVANCED_FACE('',(#3174),#1110,.F.);
#38863=ADVANCED_FACE('',(#3175),#1111,.F.);
#38864=ADVANCED_FACE('',(#3176),#1112,.F.);
#38865=ADVANCED_FACE('',(#3177),#1113,.F.);
#38866=ADVANCED_FACE('',(#3178),#1114,.F.);
#38867=ADVANCED_FACE('',(#3179),#1115,.F.);
#38868=ADVANCED_FACE('',(#3180),#1116,.F.);
#38869=ADVANCED_FACE('',(#3181),#1117,.F.);
#38870=ADVANCED_FACE('',(#3182),#1118,.F.);
#38871=ADVANCED_FACE('',(#3183),#1119,.F.);
#38872=ADVANCED_FACE('',(#3184),#1120,.F.);
#38873=ADVANCED_FACE('',(#3185),#1121,.F.);
#38874=ADVANCED_FACE('',(#3186),#1122,.F.);
#38875=ADVANCED_FACE('',(#3187),#1123,.F.);
#38876=ADVANCED_FACE('',(#3188),#1124,.F.);
#38877=ADVANCED_FACE('',(#3189),#1125,.F.);
#38878=ADVANCED_FACE('',(#3190),#1126,.F.);
#38879=ADVANCED_FACE('',(#3191),#1127,.F.);
#38880=ADVANCED_FACE('',(#3192),#1128,.F.);
#38881=ADVANCED_FACE('',(#3193),#1129,.F.);
#38882=ADVANCED_FACE('',(#3194),#1130,.F.);
#38883=ADVANCED_FACE('',(#3195),#1131,.F.);
#38884=ADVANCED_FACE('',(#3196),#1132,.F.);
#38885=ADVANCED_FACE('',(#3197),#1133,.F.);
#38886=ADVANCED_FACE('',(#3198),#1134,.F.);
#38887=ADVANCED_FACE('',(#3199),#1135,.F.);
#38888=ADVANCED_FACE('',(#3200),#1136,.F.);
#38889=ADVANCED_FACE('',(#3201),#1137,.F.);
#38890=ADVANCED_FACE('',(#3202),#1138,.F.);
#38891=ADVANCED_FACE('',(#3203),#1139,.F.);
#38892=ADVANCED_FACE('',(#3204),#1140,.F.);
#38893=ADVANCED_FACE('',(#3205),#1141,.F.);
#38894=ADVANCED_FACE('',(#3206),#1142,.F.);
#38895=ADVANCED_FACE('',(#3207),#1143,.F.);
#38896=ADVANCED_FACE('',(#3208),#1144,.F.);
#38897=ADVANCED_FACE('',(#3209),#1145,.F.);
#38898=ADVANCED_FACE('',(#3210),#1146,.F.);
#38899=ADVANCED_FACE('',(#3211),#1147,.F.);
#38900=ADVANCED_FACE('',(#3212),#1148,.F.);
#38901=ADVANCED_FACE('',(#3213),#1149,.F.);
#38902=ADVANCED_FACE('',(#3214),#1150,.F.);
#38903=ADVANCED_FACE('',(#3215),#1151,.F.);
#38904=ADVANCED_FACE('',(#3216),#1152,.F.);
#38905=ADVANCED_FACE('',(#3217),#1153,.F.);
#38906=ADVANCED_FACE('',(#3218),#1154,.F.);
#38907=ADVANCED_FACE('',(#3219),#1155,.F.);
#38908=ADVANCED_FACE('',(#3220),#1156,.F.);
#38909=ADVANCED_FACE('',(#3221),#1157,.F.);
#38910=ADVANCED_FACE('',(#3222),#1158,.F.);
#38911=ADVANCED_FACE('',(#3223),#1159,.F.);
#38912=ADVANCED_FACE('',(#3224),#1160,.F.);
#38913=ADVANCED_FACE('',(#3225),#1161,.F.);
#38914=ADVANCED_FACE('',(#3226),#1162,.F.);
#38915=ADVANCED_FACE('',(#3227),#1163,.F.);
#38916=ADVANCED_FACE('',(#3228),#1164,.F.);
#38917=ADVANCED_FACE('',(#3229),#1165,.F.);
#38918=ADVANCED_FACE('',(#3230),#1166,.F.);
#38919=ADVANCED_FACE('',(#3231),#1167,.F.);
#38920=ADVANCED_FACE('',(#3232),#1168,.F.);
#38921=ADVANCED_FACE('',(#3233),#1169,.F.);
#38922=ADVANCED_FACE('',(#3234),#1170,.F.);
#38923=ADVANCED_FACE('',(#3235),#1171,.F.);
#38924=ADVANCED_FACE('',(#3236),#1172,.F.);
#38925=ADVANCED_FACE('',(#3237),#1173,.F.);
#38926=ADVANCED_FACE('',(#3238),#1174,.F.);
#38927=ADVANCED_FACE('',(#3239),#1175,.F.);
#38928=ADVANCED_FACE('',(#3240),#1176,.F.);
#38929=ADVANCED_FACE('',(#3241),#1177,.F.);
#38930=ADVANCED_FACE('',(#3242),#1178,.F.);
#38931=ADVANCED_FACE('',(#3243),#1179,.F.);
#38932=ADVANCED_FACE('',(#3244),#1180,.F.);
#38933=ADVANCED_FACE('',(#3245),#1181,.F.);
#38934=ADVANCED_FACE('',(#3246),#1182,.F.);
#38935=ADVANCED_FACE('',(#3247),#1183,.F.);
#38936=ADVANCED_FACE('',(#3248),#1184,.F.);
#38937=ADVANCED_FACE('',(#3249),#1185,.F.);
#38938=ADVANCED_FACE('',(#3250),#1186,.F.);
#38939=ADVANCED_FACE('',(#3251),#1187,.F.);
#38940=ADVANCED_FACE('',(#3252),#1188,.F.);
#38941=ADVANCED_FACE('',(#3253),#1189,.F.);
#38942=ADVANCED_FACE('',(#3254),#1190,.F.);
#38943=ADVANCED_FACE('',(#3255),#1191,.F.);
#38944=ADVANCED_FACE('',(#3256),#1192,.F.);
#38945=ADVANCED_FACE('',(#3257),#1193,.F.);
#38946=ADVANCED_FACE('',(#3258),#1194,.F.);
#38947=ADVANCED_FACE('',(#3259),#1195,.F.);
#38948=ADVANCED_FACE('',(#3260),#1196,.F.);
#38949=ADVANCED_FACE('',(#3261),#1197,.F.);
#38950=ADVANCED_FACE('',(#3262),#1198,.F.);
#38951=ADVANCED_FACE('',(#3263),#1199,.F.);
#38952=ADVANCED_FACE('',(#3264),#1200,.F.);
#38953=ADVANCED_FACE('',(#3265),#1201,.F.);
#38954=ADVANCED_FACE('',(#3266),#1202,.F.);
#38955=ADVANCED_FACE('',(#3267),#1203,.F.);
#38956=ADVANCED_FACE('',(#3268),#1204,.F.);
#38957=ADVANCED_FACE('',(#3269),#1205,.F.);
#38958=ADVANCED_FACE('',(#3270),#1206,.F.);
#38959=ADVANCED_FACE('',(#3271),#1207,.F.);
#38960=ADVANCED_FACE('',(#3272),#1208,.F.);
#38961=ADVANCED_FACE('',(#3273),#1209,.F.);
#38962=ADVANCED_FACE('',(#3274),#1210,.F.);
#38963=ADVANCED_FACE('',(#3275),#1211,.F.);
#38964=ADVANCED_FACE('',(#3276),#1212,.F.);
#38965=ADVANCED_FACE('',(#3277),#1213,.F.);
#38966=ADVANCED_FACE('',(#3278),#1214,.F.);
#38967=ADVANCED_FACE('',(#3279),#1215,.F.);
#38968=ADVANCED_FACE('',(#3280),#1216,.F.);
#38969=ADVANCED_FACE('',(#3281),#1217,.F.);
#38970=ADVANCED_FACE('',(#3282),#1218,.F.);
#38971=ADVANCED_FACE('',(#3283),#1219,.F.);
#38972=ADVANCED_FACE('',(#3284),#1220,.F.);
#38973=ADVANCED_FACE('',(#3285),#1221,.F.);
#38974=ADVANCED_FACE('',(#3286),#1222,.F.);
#38975=ADVANCED_FACE('',(#3287),#1223,.F.);
#38976=ADVANCED_FACE('',(#3288),#1224,.F.);
#38977=ADVANCED_FACE('',(#3289),#1225,.F.);
#38978=ADVANCED_FACE('',(#3290),#1226,.F.);
#38979=ADVANCED_FACE('',(#3291),#1227,.F.);
#38980=ADVANCED_FACE('',(#3292),#1228,.F.);
#38981=ADVANCED_FACE('',(#3293),#1229,.F.);
#38982=ADVANCED_FACE('',(#3294),#1230,.F.);
#38983=ADVANCED_FACE('',(#3295),#1231,.F.);
#38984=ADVANCED_FACE('',(#3296),#1232,.F.);
#38985=ADVANCED_FACE('',(#3297),#1233,.F.);
#38986=ADVANCED_FACE('',(#3298),#1234,.F.);
#38987=ADVANCED_FACE('',(#3299),#1235,.F.);
#38988=ADVANCED_FACE('',(#3300),#1236,.F.);
#38989=ADVANCED_FACE('',(#3301),#1237,.F.);
#38990=ADVANCED_FACE('',(#3302),#1238,.F.);
#38991=ADVANCED_FACE('',(#3303),#1239,.F.);
#38992=ADVANCED_FACE('',(#3304),#1240,.F.);
#38993=ADVANCED_FACE('',(#3305),#1241,.F.);
#38994=ADVANCED_FACE('',(#3306),#1242,.F.);
#38995=ADVANCED_FACE('',(#3307),#1243,.F.);
#38996=ADVANCED_FACE('',(#3308),#1244,.F.);
#38997=ADVANCED_FACE('',(#3309),#1245,.F.);
#38998=ADVANCED_FACE('',(#3310),#1246,.F.);
#38999=ADVANCED_FACE('',(#3311),#1247,.F.);
#39000=ADVANCED_FACE('',(#3312),#1248,.F.);
#39001=ADVANCED_FACE('',(#3313),#1249,.F.);
#39002=ADVANCED_FACE('',(#3314),#1250,.F.);
#39003=ADVANCED_FACE('',(#3315),#1251,.F.);
#39004=ADVANCED_FACE('',(#3316),#1252,.F.);
#39005=ADVANCED_FACE('',(#3317),#1253,.F.);
#39006=ADVANCED_FACE('',(#3318),#1254,.F.);
#39007=ADVANCED_FACE('',(#3319),#1255,.F.);
#39008=ADVANCED_FACE('',(#3320),#1256,.F.);
#39009=ADVANCED_FACE('',(#3321),#1257,.F.);
#39010=ADVANCED_FACE('',(#3322),#1258,.F.);
#39011=ADVANCED_FACE('',(#3323),#1259,.F.);
#39012=ADVANCED_FACE('',(#3324),#1260,.F.);
#39013=ADVANCED_FACE('',(#3325),#1261,.F.);
#39014=ADVANCED_FACE('',(#3326),#1262,.F.);
#39015=ADVANCED_FACE('',(#3327),#1263,.F.);
#39016=ADVANCED_FACE('',(#3328),#1264,.F.);
#39017=ADVANCED_FACE('',(#3329),#1265,.F.);
#39018=ADVANCED_FACE('',(#3330),#1266,.F.);
#39019=ADVANCED_FACE('',(#3331),#1267,.F.);
#39020=ADVANCED_FACE('',(#3332),#1268,.F.);
#39021=ADVANCED_FACE('',(#3333),#1269,.F.);
#39022=ADVANCED_FACE('',(#3334),#1270,.F.);
#39023=ADVANCED_FACE('',(#3335),#1271,.F.);
#39024=ADVANCED_FACE('',(#3336),#1272,.F.);
#39025=ADVANCED_FACE('',(#3337),#1273,.F.);
#39026=ADVANCED_FACE('',(#3338),#1274,.F.);
#39027=ADVANCED_FACE('',(#3339),#1275,.F.);
#39028=ADVANCED_FACE('',(#3340),#1276,.F.);
#39029=ADVANCED_FACE('',(#3341),#1277,.F.);
#39030=ADVANCED_FACE('',(#3342),#1278,.F.);
#39031=ADVANCED_FACE('',(#3343),#1279,.F.);
#39032=ADVANCED_FACE('',(#3344),#1280,.F.);
#39033=ADVANCED_FACE('',(#3345),#1281,.F.);
#39034=ADVANCED_FACE('',(#3346),#1282,.F.);
#39035=ADVANCED_FACE('',(#3347),#1283,.F.);
#39036=ADVANCED_FACE('',(#3348),#1284,.F.);
#39037=ADVANCED_FACE('',(#3349),#1285,.F.);
#39038=ADVANCED_FACE('',(#3350),#1286,.F.);
#39039=ADVANCED_FACE('',(#3351),#1287,.F.);
#39040=ADVANCED_FACE('',(#3352),#1288,.F.);
#39041=ADVANCED_FACE('',(#3353),#1289,.F.);
#39042=ADVANCED_FACE('',(#3354),#1290,.F.);
#39043=ADVANCED_FACE('',(#3355),#1291,.F.);
#39044=ADVANCED_FACE('',(#3356),#1292,.F.);
#39045=ADVANCED_FACE('',(#3357),#1293,.F.);
#39046=ADVANCED_FACE('',(#3358),#1294,.F.);
#39047=ADVANCED_FACE('',(#3359),#1295,.F.);
#39048=ADVANCED_FACE('',(#3360),#1296,.F.);
#39049=ADVANCED_FACE('',(#3361),#1297,.F.);
#39050=ADVANCED_FACE('',(#3362),#1298,.F.);
#39051=ADVANCED_FACE('',(#3363),#1299,.F.);
#39052=ADVANCED_FACE('',(#3364),#1300,.F.);
#39053=ADVANCED_FACE('',(#3365),#1301,.F.);
#39054=ADVANCED_FACE('',(#3366),#1302,.F.);
#39055=ADVANCED_FACE('',(#3367),#1303,.F.);
#39056=ADVANCED_FACE('',(#3368),#1304,.F.);
#39057=ADVANCED_FACE('',(#3369),#1305,.F.);
#39058=ADVANCED_FACE('',(#3370),#1306,.F.);
#39059=ADVANCED_FACE('',(#3371),#1307,.F.);
#39060=ADVANCED_FACE('',(#3372),#1308,.F.);
#39061=ADVANCED_FACE('',(#3373),#1309,.F.);
#39062=ADVANCED_FACE('',(#3374),#1310,.F.);
#39063=ADVANCED_FACE('',(#3375),#1311,.F.);
#39064=ADVANCED_FACE('',(#3376),#1312,.F.);
#39065=ADVANCED_FACE('',(#3377),#1313,.F.);
#39066=ADVANCED_FACE('',(#3378),#1314,.F.);
#39067=ADVANCED_FACE('',(#3379),#1315,.F.);
#39068=ADVANCED_FACE('',(#3380),#1316,.F.);
#39069=ADVANCED_FACE('',(#3381),#1317,.F.);
#39070=ADVANCED_FACE('',(#3382),#1318,.F.);
#39071=ADVANCED_FACE('',(#3383),#1319,.F.);
#39072=ADVANCED_FACE('',(#3384),#1320,.F.);
#39073=ADVANCED_FACE('',(#3385),#1321,.F.);
#39074=ADVANCED_FACE('',(#3386),#1322,.F.);
#39075=ADVANCED_FACE('',(#3387),#1323,.F.);
#39076=ADVANCED_FACE('',(#3388),#1324,.F.);
#39077=ADVANCED_FACE('',(#3389),#1325,.F.);
#39078=ADVANCED_FACE('',(#3390),#1326,.F.);
#39079=ADVANCED_FACE('',(#3391),#1327,.F.);
#39080=ADVANCED_FACE('',(#3392),#1328,.F.);
#39081=ADVANCED_FACE('',(#3393),#1329,.F.);
#39082=ADVANCED_FACE('',(#3394),#1330,.F.);
#39083=ADVANCED_FACE('',(#3395),#1331,.F.);
#39084=ADVANCED_FACE('',(#3396),#1332,.F.);
#39085=ADVANCED_FACE('',(#3397),#1333,.F.);
#39086=ADVANCED_FACE('',(#3398),#1334,.F.);
#39087=ADVANCED_FACE('',(#3399),#1335,.F.);
#39088=ADVANCED_FACE('',(#3400),#1336,.F.);
#39089=ADVANCED_FACE('',(#3401),#1337,.F.);
#39090=ADVANCED_FACE('',(#3402),#1338,.F.);
#39091=ADVANCED_FACE('',(#3403),#1339,.F.);
#39092=ADVANCED_FACE('',(#3404),#1340,.F.);
#39093=ADVANCED_FACE('',(#3405),#1341,.F.);
#39094=ADVANCED_FACE('',(#3406),#1342,.F.);
#39095=ADVANCED_FACE('',(#3407),#1343,.F.);
#39096=ADVANCED_FACE('',(#3408),#1344,.F.);
#39097=ADVANCED_FACE('',(#3409),#1345,.F.);
#39098=ADVANCED_FACE('',(#3410),#1346,.F.);
#39099=ADVANCED_FACE('',(#3411),#1347,.F.);
#39100=ADVANCED_FACE('',(#3412),#1348,.F.);
#39101=ADVANCED_FACE('',(#3413),#1349,.F.);
#39102=ADVANCED_FACE('',(#3414),#1350,.F.);
#39103=ADVANCED_FACE('',(#3415),#1351,.F.);
#39104=ADVANCED_FACE('',(#3416),#1352,.F.);
#39105=ADVANCED_FACE('',(#3417),#1353,.F.);
#39106=ADVANCED_FACE('',(#3418),#1354,.F.);
#39107=ADVANCED_FACE('',(#3419),#1355,.F.);
#39108=ADVANCED_FACE('',(#3420),#1356,.F.);
#39109=ADVANCED_FACE('',(#3421),#1357,.F.);
#39110=ADVANCED_FACE('',(#3422),#1358,.F.);
#39111=ADVANCED_FACE('',(#3423),#1359,.F.);
#39112=ADVANCED_FACE('',(#3424),#1360,.F.);
#39113=ADVANCED_FACE('',(#3425),#1361,.F.);
#39114=ADVANCED_FACE('',(#3426),#1362,.F.);
#39115=ADVANCED_FACE('',(#3427),#1363,.F.);
#39116=ADVANCED_FACE('',(#3428),#1364,.F.);
#39117=ADVANCED_FACE('',(#3429),#1365,.F.);
#39118=ADVANCED_FACE('',(#3430),#1366,.F.);
#39119=ADVANCED_FACE('',(#3431),#1367,.F.);
#39120=ADVANCED_FACE('',(#3432),#1368,.F.);
#39121=ADVANCED_FACE('',(#3433),#1369,.F.);
#39122=ADVANCED_FACE('',(#3434),#1370,.F.);
#39123=ADVANCED_FACE('',(#3435),#1371,.F.);
#39124=ADVANCED_FACE('',(#3436),#1372,.F.);
#39125=ADVANCED_FACE('',(#3437),#1373,.F.);
#39126=ADVANCED_FACE('',(#3438),#1374,.F.);
#39127=ADVANCED_FACE('',(#3439),#1375,.F.);
#39128=ADVANCED_FACE('',(#3440),#1376,.F.);
#39129=ADVANCED_FACE('',(#3441),#1377,.F.);
#39130=ADVANCED_FACE('',(#3442),#1378,.F.);
#39131=ADVANCED_FACE('',(#3443),#1379,.F.);
#39132=ADVANCED_FACE('',(#3444),#1380,.F.);
#39133=ADVANCED_FACE('',(#3445),#1381,.F.);
#39134=ADVANCED_FACE('',(#3446),#1382,.F.);
#39135=ADVANCED_FACE('',(#3447),#1383,.F.);
#39136=ADVANCED_FACE('',(#3448),#1384,.F.);
#39137=ADVANCED_FACE('',(#3449),#1385,.F.);
#39138=ADVANCED_FACE('',(#3450),#1386,.F.);
#39139=ADVANCED_FACE('',(#3451),#1387,.F.);
#39140=ADVANCED_FACE('',(#3452),#1388,.F.);
#39141=ADVANCED_FACE('',(#3453),#1389,.F.);
#39142=ADVANCED_FACE('',(#3454),#1390,.F.);
#39143=ADVANCED_FACE('',(#3455),#1391,.F.);
#39144=ADVANCED_FACE('',(#3456),#1392,.F.);
#39145=ADVANCED_FACE('',(#3457),#1393,.F.);
#39146=ADVANCED_FACE('',(#3458),#1394,.F.);
#39147=ADVANCED_FACE('',(#3459),#1395,.F.);
#39148=ADVANCED_FACE('',(#3460),#1396,.F.);
#39149=ADVANCED_FACE('',(#3461),#1397,.F.);
#39150=ADVANCED_FACE('',(#3462),#1398,.F.);
#39151=ADVANCED_FACE('',(#3463),#1399,.F.);
#39152=ADVANCED_FACE('',(#3464),#1400,.F.);
#39153=ADVANCED_FACE('',(#3465),#1401,.F.);
#39154=ADVANCED_FACE('',(#3466),#1402,.F.);
#39155=ADVANCED_FACE('',(#3467),#1403,.F.);
#39156=ADVANCED_FACE('',(#3468),#1404,.F.);
#39157=ADVANCED_FACE('',(#3469),#1405,.F.);
#39158=ADVANCED_FACE('',(#3470),#1406,.F.);
#39159=ADVANCED_FACE('',(#3471),#1407,.F.);
#39160=ADVANCED_FACE('',(#3472),#1408,.F.);
#39161=ADVANCED_FACE('',(#3473),#1409,.F.);
#39162=ADVANCED_FACE('',(#3474),#1410,.F.);
#39163=ADVANCED_FACE('',(#3475),#1411,.F.);
#39164=ADVANCED_FACE('',(#3476),#1412,.F.);
#39165=ADVANCED_FACE('',(#3477),#1413,.F.);
#39166=ADVANCED_FACE('',(#3478),#1414,.F.);
#39167=ADVANCED_FACE('',(#3479),#1415,.F.);
#39168=ADVANCED_FACE('',(#3480),#1416,.F.);
#39169=ADVANCED_FACE('',(#3481),#1417,.F.);
#39170=ADVANCED_FACE('',(#3482),#1418,.F.);
#39171=ADVANCED_FACE('',(#3483),#1419,.F.);
#39172=ADVANCED_FACE('',(#3484),#1420,.F.);
#39173=ADVANCED_FACE('',(#3485),#1421,.F.);
#39174=ADVANCED_FACE('',(#3486),#1422,.F.);
#39175=ADVANCED_FACE('',(#3487),#1423,.F.);
#39176=ADVANCED_FACE('',(#3488),#1424,.F.);
#39177=ADVANCED_FACE('',(#3489),#1425,.F.);
#39178=ADVANCED_FACE('',(#3490),#1426,.F.);
#39179=ADVANCED_FACE('',(#3491),#1427,.F.);
#39180=ADVANCED_FACE('',(#3492),#1428,.F.);
#39181=ADVANCED_FACE('',(#3493),#1429,.F.);
#39182=ADVANCED_FACE('',(#3494),#1430,.F.);
#39183=ADVANCED_FACE('',(#3495),#1431,.F.);
#39184=ADVANCED_FACE('',(#3496),#1432,.F.);
#39185=ADVANCED_FACE('',(#3497),#1433,.F.);
#39186=ADVANCED_FACE('',(#3498),#1434,.F.);
#39187=ADVANCED_FACE('',(#3499),#1435,.F.);
#39188=ADVANCED_FACE('',(#3500),#1436,.F.);
#39189=ADVANCED_FACE('',(#3501),#1437,.F.);
#39190=ADVANCED_FACE('',(#3502),#1438,.F.);
#39191=ADVANCED_FACE('',(#3503),#1439,.F.);
#39192=ADVANCED_FACE('',(#3504),#1440,.F.);
#39193=ADVANCED_FACE('',(#3505),#1441,.F.);
#39194=ADVANCED_FACE('',(#3506),#1442,.F.);
#39195=ADVANCED_FACE('',(#3507),#1443,.F.);
#39196=ADVANCED_FACE('',(#3508),#1444,.F.);
#39197=ADVANCED_FACE('',(#3509),#1445,.F.);
#39198=ADVANCED_FACE('',(#3510),#1446,.F.);
#39199=ADVANCED_FACE('',(#3511),#1447,.F.);
#39200=ADVANCED_FACE('',(#3512),#1448,.F.);
#39201=ADVANCED_FACE('',(#3513),#1449,.F.);
#39202=ADVANCED_FACE('',(#3514),#1450,.F.);
#39203=ADVANCED_FACE('',(#3515),#1451,.F.);
#39204=ADVANCED_FACE('',(#3516),#1452,.F.);
#39205=ADVANCED_FACE('',(#3517),#1453,.F.);
#39206=ADVANCED_FACE('',(#3518),#1454,.F.);
#39207=ADVANCED_FACE('',(#3519),#1455,.F.);
#39208=ADVANCED_FACE('',(#3520),#1456,.F.);
#39209=ADVANCED_FACE('',(#3521),#1457,.F.);
#39210=ADVANCED_FACE('',(#3522),#1458,.F.);
#39211=ADVANCED_FACE('',(#3523),#1459,.F.);
#39212=ADVANCED_FACE('',(#3524),#1460,.F.);
#39213=ADVANCED_FACE('',(#3525),#1461,.F.);
#39214=ADVANCED_FACE('',(#3526),#1462,.F.);
#39215=ADVANCED_FACE('',(#3527),#1463,.F.);
#39216=ADVANCED_FACE('',(#3528),#1464,.F.);
#39217=ADVANCED_FACE('',(#3529),#1465,.F.);
#39218=ADVANCED_FACE('',(#3530),#1466,.F.);
#39219=ADVANCED_FACE('',(#3531),#1467,.F.);
#39220=ADVANCED_FACE('',(#3532),#1468,.F.);
#39221=ADVANCED_FACE('',(#3533),#1469,.F.);
#39222=ADVANCED_FACE('',(#3534),#1470,.F.);
#39223=ADVANCED_FACE('',(#3535),#1471,.F.);
#39224=ADVANCED_FACE('',(#3536),#1472,.F.);
#39225=ADVANCED_FACE('',(#3537),#1473,.F.);
#39226=ADVANCED_FACE('',(#3538),#1474,.F.);
#39227=ADVANCED_FACE('',(#3539),#1475,.F.);
#39228=ADVANCED_FACE('',(#3540),#1476,.F.);
#39229=ADVANCED_FACE('',(#3541),#1477,.F.);
#39230=ADVANCED_FACE('',(#3542),#1478,.F.);
#39231=ADVANCED_FACE('',(#3543),#1479,.F.);
#39232=ADVANCED_FACE('',(#3544),#1480,.F.);
#39233=ADVANCED_FACE('',(#3545),#1481,.F.);
#39234=ADVANCED_FACE('',(#3546),#1482,.F.);
#39235=ADVANCED_FACE('',(#3547),#1483,.F.);
#39236=ADVANCED_FACE('',(#3548),#1484,.F.);
#39237=ADVANCED_FACE('',(#3549),#1485,.F.);
#39238=ADVANCED_FACE('',(#3550),#1486,.F.);
#39239=ADVANCED_FACE('',(#3551),#1487,.F.);
#39240=ADVANCED_FACE('',(#3552),#1488,.F.);
#39241=ADVANCED_FACE('',(#3553),#1489,.F.);
#39242=ADVANCED_FACE('',(#3554),#1490,.F.);
#39243=ADVANCED_FACE('',(#3555),#1491,.F.);
#39244=ADVANCED_FACE('',(#3556),#1492,.F.);
#39245=ADVANCED_FACE('',(#3557),#1493,.F.);
#39246=ADVANCED_FACE('',(#3558),#1494,.F.);
#39247=ADVANCED_FACE('',(#3559),#1495,.F.);
#39248=ADVANCED_FACE('',(#3560),#1496,.F.);
#39249=ADVANCED_FACE('',(#3561),#1497,.F.);
#39250=ADVANCED_FACE('',(#3562),#1498,.F.);
#39251=ADVANCED_FACE('',(#3563),#1499,.F.);
#39252=ADVANCED_FACE('',(#3564),#1500,.F.);
#39253=ADVANCED_FACE('',(#3565),#1501,.F.);
#39254=ADVANCED_FACE('',(#3566),#1502,.F.);
#39255=ADVANCED_FACE('',(#3567),#1503,.F.);
#39256=ADVANCED_FACE('',(#3568),#1504,.F.);
#39257=ADVANCED_FACE('',(#3569),#1505,.F.);
#39258=ADVANCED_FACE('',(#3570),#1506,.F.);
#39259=ADVANCED_FACE('',(#3571),#1507,.F.);
#39260=ADVANCED_FACE('',(#3572),#1508,.F.);
#39261=ADVANCED_FACE('',(#3573),#1509,.F.);
#39262=ADVANCED_FACE('',(#3574),#1510,.F.);
#39263=ADVANCED_FACE('',(#3575),#1511,.F.);
#39264=ADVANCED_FACE('',(#3576),#1512,.F.);
#39265=ADVANCED_FACE('',(#3577),#1513,.F.);
#39266=ADVANCED_FACE('',(#3578),#1514,.F.);
#39267=ADVANCED_FACE('',(#3579),#1515,.F.);
#39268=ADVANCED_FACE('',(#3580),#1516,.F.);
#39269=ADVANCED_FACE('',(#3581),#1517,.F.);
#39270=ADVANCED_FACE('',(#3582),#1518,.F.);
#39271=ADVANCED_FACE('',(#3583),#1519,.F.);
#39272=ADVANCED_FACE('',(#3584),#1520,.F.);
#39273=ADVANCED_FACE('',(#3585),#1521,.F.);
#39274=ADVANCED_FACE('',(#3586),#1522,.F.);
#39275=ADVANCED_FACE('',(#3587),#1523,.F.);
#39276=ADVANCED_FACE('',(#3588),#1524,.F.);
#39277=ADVANCED_FACE('',(#3589),#1525,.F.);
#39278=ADVANCED_FACE('',(#3590),#1526,.F.);
#39279=ADVANCED_FACE('',(#3591),#1527,.F.);
#39280=ADVANCED_FACE('',(#3592),#1528,.F.);
#39281=ADVANCED_FACE('',(#3593),#1529,.F.);
#39282=ADVANCED_FACE('',(#3594),#1530,.F.);
#39283=ADVANCED_FACE('',(#3595),#1531,.F.);
#39284=ADVANCED_FACE('',(#3596),#1532,.F.);
#39285=ADVANCED_FACE('',(#3597),#1533,.F.);
#39286=ADVANCED_FACE('',(#3598),#1534,.F.);
#39287=ADVANCED_FACE('',(#3599),#1535,.F.);
#39288=ADVANCED_FACE('',(#3600),#1536,.F.);
#39289=ADVANCED_FACE('',(#3601),#1537,.F.);
#39290=ADVANCED_FACE('',(#3602),#1538,.F.);
#39291=ADVANCED_FACE('',(#3603),#1539,.F.);
#39292=ADVANCED_FACE('',(#3604),#1540,.F.);
#39293=ADVANCED_FACE('',(#3605),#1541,.F.);
#39294=ADVANCED_FACE('',(#3606),#1542,.F.);
#39295=ADVANCED_FACE('',(#3607),#1543,.F.);
#39296=ADVANCED_FACE('',(#3608),#1544,.F.);
#39297=ADVANCED_FACE('',(#3609),#1545,.F.);
#39298=ADVANCED_FACE('',(#3610),#1546,.F.);
#39299=ADVANCED_FACE('',(#3611),#1547,.F.);
#39300=ADVANCED_FACE('',(#3612),#1548,.F.);
#39301=ADVANCED_FACE('',(#3613),#1549,.F.);
#39302=ADVANCED_FACE('',(#3614),#1550,.F.);
#39303=ADVANCED_FACE('',(#3615),#1551,.F.);
#39304=ADVANCED_FACE('',(#3616),#1552,.F.);
#39305=ADVANCED_FACE('',(#3617),#1553,.F.);
#39306=ADVANCED_FACE('',(#3618),#1554,.F.);
#39307=ADVANCED_FACE('',(#3619),#1555,.F.);
#39308=ADVANCED_FACE('',(#3620),#1556,.F.);
#39309=ADVANCED_FACE('',(#3621),#1557,.F.);
#39310=ADVANCED_FACE('',(#3622),#1558,.F.);
#39311=ADVANCED_FACE('',(#3623),#1559,.F.);
#39312=ADVANCED_FACE('',(#3624),#1560,.F.);
#39313=ADVANCED_FACE('',(#3625),#1561,.F.);
#39314=ADVANCED_FACE('',(#3626),#1562,.F.);
#39315=ADVANCED_FACE('',(#3627),#1563,.F.);
#39316=ADVANCED_FACE('',(#3628),#1564,.F.);
#39317=ADVANCED_FACE('',(#3629),#1565,.F.);
#39318=ADVANCED_FACE('',(#3630),#1566,.F.);
#39319=ADVANCED_FACE('',(#3631),#1567,.F.);
#39320=ADVANCED_FACE('',(#3632),#1568,.F.);
#39321=ADVANCED_FACE('',(#3633),#1569,.F.);
#39322=ADVANCED_FACE('',(#3634),#1570,.F.);
#39323=ADVANCED_FACE('',(#3635),#1571,.F.);
#39324=ADVANCED_FACE('',(#3636),#1572,.F.);
#39325=ADVANCED_FACE('',(#3637),#1573,.F.);
#39326=ADVANCED_FACE('',(#3638),#1574,.F.);
#39327=ADVANCED_FACE('',(#3639),#1575,.F.);
#39328=ADVANCED_FACE('',(#3640),#1576,.F.);
#39329=ADVANCED_FACE('',(#3641),#1577,.F.);
#39330=ADVANCED_FACE('',(#3642),#1578,.F.);
#39331=ADVANCED_FACE('',(#3643),#1579,.F.);
#39332=ADVANCED_FACE('',(#3644),#1580,.F.);
#39333=ADVANCED_FACE('',(#3645),#1581,.F.);
#39334=ADVANCED_FACE('',(#3646),#1582,.F.);
#39335=ADVANCED_FACE('',(#3647),#1583,.F.);
#39336=ADVANCED_FACE('',(#3648),#1584,.F.);
#39337=ADVANCED_FACE('',(#3649),#1585,.F.);
#39338=ADVANCED_FACE('',(#3650),#1586,.F.);
#39339=ADVANCED_FACE('',(#3651),#1587,.F.);
#39340=ADVANCED_FACE('',(#3652),#1588,.F.);
#39341=ADVANCED_FACE('',(#3653),#1589,.F.);
#39342=ADVANCED_FACE('',(#3654),#1590,.F.);
#39343=ADVANCED_FACE('',(#3655),#1591,.F.);
#39344=ADVANCED_FACE('',(#3656),#1592,.F.);
#39345=ADVANCED_FACE('',(#3657),#1593,.F.);
#39346=ADVANCED_FACE('',(#3658),#1594,.F.);
#39347=ADVANCED_FACE('',(#3659),#1595,.F.);
#39348=ADVANCED_FACE('',(#3660),#1596,.F.);
#39349=ADVANCED_FACE('',(#3661),#1597,.F.);
#39350=ADVANCED_FACE('',(#3662),#1598,.F.);
#39351=ADVANCED_FACE('',(#3663),#1599,.F.);
#39352=ADVANCED_FACE('',(#3664),#1600,.F.);
#39353=ADVANCED_FACE('',(#3665),#1601,.F.);
#39354=ADVANCED_FACE('',(#3666),#1602,.F.);
#39355=ADVANCED_FACE('',(#3667),#1603,.F.);
#39356=ADVANCED_FACE('',(#3668),#1604,.F.);
#39357=ADVANCED_FACE('',(#3669),#1605,.F.);
#39358=ADVANCED_FACE('',(#3670),#1606,.F.);
#39359=ADVANCED_FACE('',(#3671),#1607,.F.);
#39360=ADVANCED_FACE('',(#3672),#1608,.F.);
#39361=ADVANCED_FACE('',(#3673),#1609,.F.);
#39362=ADVANCED_FACE('',(#3674),#1610,.F.);
#39363=ADVANCED_FACE('',(#3675),#1611,.F.);
#39364=ADVANCED_FACE('',(#3676),#1612,.F.);
#39365=ADVANCED_FACE('',(#3677),#1613,.F.);
#39366=ADVANCED_FACE('',(#3678),#1614,.F.);
#39367=ADVANCED_FACE('',(#3679),#1615,.F.);
#39368=ADVANCED_FACE('',(#3680),#1616,.F.);
#39369=ADVANCED_FACE('',(#3681),#1617,.F.);
#39370=ADVANCED_FACE('',(#3682),#1618,.F.);
#39371=ADVANCED_FACE('',(#3683),#1619,.F.);
#39372=ADVANCED_FACE('',(#3684),#1620,.F.);
#39373=ADVANCED_FACE('',(#3685),#1621,.F.);
#39374=ADVANCED_FACE('',(#3686),#1622,.F.);
#39375=ADVANCED_FACE('',(#3687),#1623,.F.);
#39376=ADVANCED_FACE('',(#3688),#1624,.F.);
#39377=ADVANCED_FACE('',(#3689),#1625,.F.);
#39378=ADVANCED_FACE('',(#3690),#1626,.F.);
#39379=ADVANCED_FACE('',(#3691),#1627,.F.);
#39380=ADVANCED_FACE('',(#3692),#1628,.F.);
#39381=ADVANCED_FACE('',(#3693),#1629,.F.);
#39382=ADVANCED_FACE('',(#3694),#1630,.F.);
#39383=ADVANCED_FACE('',(#3695),#1631,.F.);
#39384=ADVANCED_FACE('',(#3696),#1632,.F.);
#39385=ADVANCED_FACE('',(#3697),#1633,.F.);
#39386=ADVANCED_FACE('',(#3698),#1634,.F.);
#39387=ADVANCED_FACE('',(#3699),#1635,.F.);
#39388=ADVANCED_FACE('',(#3700),#1636,.F.);
#39389=ADVANCED_FACE('',(#3701),#1637,.F.);
#39390=ADVANCED_FACE('',(#3702),#1638,.F.);
#39391=ADVANCED_FACE('',(#3703),#1639,.F.);
#39392=ADVANCED_FACE('',(#3704),#1640,.F.);
#39393=ADVANCED_FACE('',(#3705),#1641,.F.);
#39394=ADVANCED_FACE('',(#3706),#1642,.F.);
#39395=ADVANCED_FACE('',(#3707),#1643,.F.);
#39396=ADVANCED_FACE('',(#3708),#1644,.F.);
#39397=ADVANCED_FACE('',(#3709),#1645,.F.);
#39398=ADVANCED_FACE('',(#3710),#1646,.F.);
#39399=ADVANCED_FACE('',(#3711),#1647,.F.);
#39400=ADVANCED_FACE('',(#3712),#1648,.F.);
#39401=ADVANCED_FACE('',(#3713),#1649,.F.);
#39402=ADVANCED_FACE('',(#3714),#1650,.F.);
#39403=ADVANCED_FACE('',(#3715),#1651,.F.);
#39404=ADVANCED_FACE('',(#3716),#1652,.F.);
#39405=ADVANCED_FACE('',(#3717),#1653,.F.);
#39406=ADVANCED_FACE('',(#3718),#1654,.F.);
#39407=ADVANCED_FACE('',(#3719),#1655,.F.);
#39408=ADVANCED_FACE('',(#3720),#1656,.F.);
#39409=ADVANCED_FACE('',(#3721),#1657,.F.);
#39410=ADVANCED_FACE('',(#3722),#1658,.F.);
#39411=ADVANCED_FACE('',(#3723),#1659,.F.);
#39412=ADVANCED_FACE('',(#3724),#1660,.F.);
#39413=ADVANCED_FACE('',(#3725),#1661,.F.);
#39414=ADVANCED_FACE('',(#3726),#1662,.F.);
#39415=ADVANCED_FACE('',(#3727),#1663,.F.);
#39416=ADVANCED_FACE('',(#3728),#1664,.F.);
#39417=ADVANCED_FACE('',(#3729),#1665,.F.);
#39418=ADVANCED_FACE('',(#3730),#1666,.F.);
#39419=ADVANCED_FACE('',(#3731),#1667,.F.);
#39420=ADVANCED_FACE('',(#3732),#1668,.F.);
#39421=ADVANCED_FACE('',(#3733),#1669,.F.);
#39422=ADVANCED_FACE('',(#3734),#1670,.F.);
#39423=ADVANCED_FACE('',(#3735),#1671,.F.);
#39424=ADVANCED_FACE('',(#3736),#1672,.F.);
#39425=ADVANCED_FACE('',(#3737),#1673,.F.);
#39426=ADVANCED_FACE('',(#3738),#1674,.F.);
#39427=ADVANCED_FACE('',(#3739),#1675,.F.);
#39428=ADVANCED_FACE('',(#3740),#1676,.F.);
#39429=ADVANCED_FACE('',(#3741),#1677,.F.);
#39430=ADVANCED_FACE('',(#3742),#1678,.F.);
#39431=ADVANCED_FACE('',(#3743),#1679,.F.);
#39432=ADVANCED_FACE('',(#3744),#1680,.F.);
#39433=ADVANCED_FACE('',(#3745),#1681,.F.);
#39434=ADVANCED_FACE('',(#3746),#1682,.F.);
#39435=ADVANCED_FACE('',(#3747),#1683,.F.);
#39436=ADVANCED_FACE('',(#3748),#1684,.F.);
#39437=ADVANCED_FACE('',(#3749),#1685,.F.);
#39438=ADVANCED_FACE('',(#3750),#1686,.F.);
#39439=ADVANCED_FACE('',(#3751),#1687,.F.);
#39440=ADVANCED_FACE('',(#3752),#1688,.F.);
#39441=ADVANCED_FACE('',(#3753),#1689,.F.);
#39442=ADVANCED_FACE('',(#3754),#1690,.F.);
#39443=ADVANCED_FACE('',(#3755),#1691,.F.);
#39444=ADVANCED_FACE('',(#3756),#1692,.F.);
#39445=ADVANCED_FACE('',(#3757),#1693,.F.);
#39446=ADVANCED_FACE('',(#3758),#1694,.F.);
#39447=ADVANCED_FACE('',(#3759),#1695,.F.);
#39448=ADVANCED_FACE('',(#3760),#1696,.F.);
#39449=ADVANCED_FACE('',(#3761),#1697,.F.);
#39450=ADVANCED_FACE('',(#3762),#1698,.F.);
#39451=ADVANCED_FACE('',(#3763),#1699,.F.);
#39452=ADVANCED_FACE('',(#3764),#1700,.F.);
#39453=ADVANCED_FACE('',(#3765),#1701,.F.);
#39454=ADVANCED_FACE('',(#3766),#1702,.F.);
#39455=ADVANCED_FACE('',(#3767),#1703,.F.);
#39456=ADVANCED_FACE('',(#3768),#1704,.F.);
#39457=ADVANCED_FACE('',(#3769),#1705,.F.);
#39458=ADVANCED_FACE('',(#3770),#1706,.F.);
#39459=ADVANCED_FACE('',(#3771),#1707,.F.);
#39460=ADVANCED_FACE('',(#3772),#1708,.F.);
#39461=ADVANCED_FACE('',(#3773),#1709,.F.);
#39462=ADVANCED_FACE('',(#3774),#1710,.F.);
#39463=ADVANCED_FACE('',(#3775),#1711,.F.);
#39464=ADVANCED_FACE('',(#3776),#1712,.F.);
#39465=ADVANCED_FACE('',(#3777),#1713,.F.);
#39466=ADVANCED_FACE('',(#3778),#1714,.F.);
#39467=ADVANCED_FACE('',(#3779),#1715,.F.);
#39468=ADVANCED_FACE('',(#3780),#1716,.F.);
#39469=ADVANCED_FACE('',(#3781),#1717,.F.);
#39470=ADVANCED_FACE('',(#3782),#1718,.F.);
#39471=ADVANCED_FACE('',(#3783),#1719,.F.);
#39472=ADVANCED_FACE('',(#3784),#1720,.F.);
#39473=ADVANCED_FACE('',(#3785),#1721,.F.);
#39474=ADVANCED_FACE('',(#3786),#1722,.F.);
#39475=ADVANCED_FACE('',(#3787),#1723,.F.);
#39476=ADVANCED_FACE('',(#3788),#1724,.F.);
#39477=ADVANCED_FACE('',(#3789),#1725,.F.);
#39478=ADVANCED_FACE('',(#3790),#1726,.F.);
#39479=ADVANCED_FACE('',(#3791),#1727,.F.);
#39480=ADVANCED_FACE('',(#3792),#1728,.F.);
#39481=ADVANCED_FACE('',(#3793),#1729,.F.);
#39482=ADVANCED_FACE('',(#3794),#1730,.F.);
#39483=ADVANCED_FACE('',(#3795),#1731,.F.);
#39484=ADVANCED_FACE('',(#3796),#1732,.F.);
#39485=ADVANCED_FACE('',(#3797),#1733,.F.);
#39486=ADVANCED_FACE('',(#3798),#1734,.F.);
#39487=ADVANCED_FACE('',(#3799),#1735,.F.);
#39488=ADVANCED_FACE('',(#3800),#1736,.F.);
#39489=ADVANCED_FACE('',(#3801),#1737,.F.);
#39490=ADVANCED_FACE('',(#3802),#1738,.F.);
#39491=ADVANCED_FACE('',(#3803),#1739,.F.);
#39492=ADVANCED_FACE('',(#3804),#1740,.F.);
#39493=ADVANCED_FACE('',(#3805),#1741,.F.);
#39494=ADVANCED_FACE('',(#3806),#1742,.F.);
#39495=ADVANCED_FACE('',(#3807),#1743,.F.);
#39496=ADVANCED_FACE('',(#3808),#1744,.F.);
#39497=ADVANCED_FACE('',(#3809),#1745,.F.);
#39498=ADVANCED_FACE('',(#3810),#1746,.F.);
#39499=ADVANCED_FACE('',(#3811),#1747,.F.);
#39500=ADVANCED_FACE('',(#3812),#1748,.F.);
#39501=ADVANCED_FACE('',(#3813),#1749,.F.);
#39502=ADVANCED_FACE('',(#3814),#1750,.F.);
#39503=ADVANCED_FACE('',(#3815),#1751,.F.);
#39504=ADVANCED_FACE('',(#3816),#1752,.F.);
#39505=ADVANCED_FACE('',(#3817),#1753,.F.);
#39506=ADVANCED_FACE('',(#3818),#1754,.F.);
#39507=ADVANCED_FACE('',(#3819),#1755,.F.);
#39508=ADVANCED_FACE('',(#3820),#1756,.F.);
#39509=ADVANCED_FACE('',(#3821),#1757,.F.);
#39510=ADVANCED_FACE('',(#3822),#1758,.F.);
#39511=ADVANCED_FACE('',(#3823),#1759,.F.);
#39512=ADVANCED_FACE('',(#3824),#1760,.F.);
#39513=ADVANCED_FACE('',(#3825),#1761,.F.);
#39514=ADVANCED_FACE('',(#3826),#1762,.F.);
#39515=ADVANCED_FACE('',(#3827),#1763,.F.);
#39516=ADVANCED_FACE('',(#3828),#1764,.F.);
#39517=ADVANCED_FACE('',(#3829),#1765,.F.);
#39518=ADVANCED_FACE('',(#3830),#1766,.F.);
#39519=ADVANCED_FACE('',(#3831),#1767,.F.);
#39520=ADVANCED_FACE('',(#3832),#1768,.F.);
#39521=ADVANCED_FACE('',(#3833),#1769,.F.);
#39522=ADVANCED_FACE('',(#3834),#1770,.F.);
#39523=ADVANCED_FACE('',(#3835),#1771,.F.);
#39524=ADVANCED_FACE('',(#3836),#1772,.F.);
#39525=ADVANCED_FACE('',(#3837),#1773,.F.);
#39526=ADVANCED_FACE('',(#3838),#1774,.F.);
#39527=ADVANCED_FACE('',(#3839),#1775,.F.);
#39528=ADVANCED_FACE('',(#3840),#1776,.F.);
#39529=ADVANCED_FACE('',(#3841),#1777,.F.);
#39530=ADVANCED_FACE('',(#3842),#1778,.F.);
#39531=ADVANCED_FACE('',(#3843),#1779,.F.);
#39532=ADVANCED_FACE('',(#3844),#1780,.F.);
#39533=ADVANCED_FACE('',(#3845),#1781,.F.);
#39534=ADVANCED_FACE('',(#3846),#1782,.F.);
#39535=ADVANCED_FACE('',(#3847),#1783,.F.);
#39536=ADVANCED_FACE('',(#3848),#1784,.F.);
#39537=ADVANCED_FACE('',(#3849),#1785,.F.);
#39538=ADVANCED_FACE('',(#3850),#1786,.F.);
#39539=ADVANCED_FACE('',(#3851),#1787,.F.);
#39540=ADVANCED_FACE('',(#3852),#1788,.F.);
#39541=ADVANCED_FACE('',(#3853),#1789,.F.);
#39542=ADVANCED_FACE('',(#3854),#1790,.F.);
#39543=ADVANCED_FACE('',(#3855),#1791,.F.);
#39544=ADVANCED_FACE('',(#3856),#1792,.F.);
#39545=ADVANCED_FACE('',(#3857),#1793,.F.);
#39546=ADVANCED_FACE('',(#3858),#1794,.F.);
#39547=ADVANCED_FACE('',(#3859),#1795,.F.);
#39548=ADVANCED_FACE('',(#3860),#1796,.F.);
#39549=ADVANCED_FACE('',(#3861),#1797,.F.);
#39550=ADVANCED_FACE('',(#3862),#1798,.F.);
#39551=ADVANCED_FACE('',(#3863),#1799,.F.);
#39552=ADVANCED_FACE('',(#3864),#1800,.F.);
#39553=ADVANCED_FACE('',(#3865),#1801,.F.);
#39554=ADVANCED_FACE('',(#3866),#1802,.F.);
#39555=ADVANCED_FACE('',(#3867),#1803,.F.);
#39556=ADVANCED_FACE('',(#3868),#1804,.F.);
#39557=ADVANCED_FACE('',(#3869),#1805,.F.);
#39558=ADVANCED_FACE('',(#3870),#1806,.F.);
#39559=ADVANCED_FACE('',(#3871),#1807,.F.);
#39560=ADVANCED_FACE('',(#3872),#1808,.F.);
#39561=ADVANCED_FACE('',(#3873),#1809,.F.);
#39562=ADVANCED_FACE('',(#3874),#1810,.F.);
#39563=ADVANCED_FACE('',(#3875),#1811,.F.);
#39564=ADVANCED_FACE('',(#3876),#1812,.F.);
#39565=ADVANCED_FACE('',(#3877),#1813,.F.);
#39566=ADVANCED_FACE('',(#3878),#1814,.F.);
#39567=ADVANCED_FACE('',(#3879),#1815,.F.);
#39568=ADVANCED_FACE('',(#3880),#1816,.F.);
#39569=ADVANCED_FACE('',(#3881),#1817,.F.);
#39570=ADVANCED_FACE('',(#3882),#1818,.F.);
#39571=ADVANCED_FACE('',(#3883),#1819,.F.);
#39572=ADVANCED_FACE('',(#3884),#1820,.F.);
#39573=ADVANCED_FACE('',(#3885),#1821,.F.);
#39574=ADVANCED_FACE('',(#3886),#1822,.F.);
#39575=ADVANCED_FACE('',(#3887),#1823,.F.);
#39576=ADVANCED_FACE('',(#3888),#1824,.F.);
#39577=ADVANCED_FACE('',(#3889),#1825,.F.);
#39578=ADVANCED_FACE('',(#3890),#1826,.F.);
#39579=ADVANCED_FACE('',(#3891),#1827,.F.);
#39580=ADVANCED_FACE('',(#3892),#1828,.F.);
#39581=ADVANCED_FACE('',(#3893),#1829,.F.);
#39582=ADVANCED_FACE('',(#3894),#1830,.F.);
#39583=ADVANCED_FACE('',(#3895),#1831,.F.);
#39584=ADVANCED_FACE('',(#3896),#1832,.F.);
#39585=ADVANCED_FACE('',(#3897),#1833,.F.);
#39586=ADVANCED_FACE('',(#3898),#1834,.F.);
#39587=ADVANCED_FACE('',(#3899),#1835,.F.);
#39588=ADVANCED_FACE('',(#3900),#1836,.F.);
#39589=ADVANCED_FACE('',(#3901),#1837,.F.);
#39590=ADVANCED_FACE('',(#3902),#1838,.F.);
#39591=ADVANCED_FACE('',(#3903),#1839,.F.);
#39592=ADVANCED_FACE('',(#3904),#1840,.F.);
#39593=ADVANCED_FACE('',(#3905),#1841,.F.);
#39594=ADVANCED_FACE('',(#3906),#1842,.F.);
#39595=ADVANCED_FACE('',(#3907),#1843,.F.);
#39596=ADVANCED_FACE('',(#3908),#1844,.F.);
#39597=ADVANCED_FACE('',(#3909),#1845,.F.);
#39598=ADVANCED_FACE('',(#3910),#1846,.F.);
#39599=ADVANCED_FACE('',(#3911),#1847,.F.);
#39600=ADVANCED_FACE('',(#3912),#1848,.F.);
#39601=ADVANCED_FACE('',(#3913),#1849,.F.);
#39602=ADVANCED_FACE('',(#3914),#1850,.F.);
#39603=ADVANCED_FACE('',(#3915),#1851,.F.);
#39604=ADVANCED_FACE('',(#3916),#1852,.F.);
#39605=ADVANCED_FACE('',(#3917),#1853,.F.);
#39606=ADVANCED_FACE('',(#3918),#1854,.F.);
#39607=ADVANCED_FACE('',(#3919),#1855,.F.);
#39608=ADVANCED_FACE('',(#3920),#1856,.F.);
#39609=ADVANCED_FACE('',(#3921),#1857,.F.);
#39610=ADVANCED_FACE('',(#3922),#1858,.F.);
#39611=ADVANCED_FACE('',(#3923),#1859,.F.);
#39612=ADVANCED_FACE('',(#3924),#1860,.F.);
#39613=ADVANCED_FACE('',(#3925),#1861,.F.);
#39614=ADVANCED_FACE('',(#3926),#1862,.F.);
#39615=ADVANCED_FACE('',(#3927),#1863,.F.);
#39616=ADVANCED_FACE('',(#3928),#1864,.F.);
#39617=ADVANCED_FACE('',(#3929),#1865,.F.);
#39618=ADVANCED_FACE('',(#3930),#1866,.F.);
#39619=ADVANCED_FACE('',(#3931),#1867,.F.);
#39620=ADVANCED_FACE('',(#3932),#1868,.F.);
#39621=ADVANCED_FACE('',(#3933),#1869,.F.);
#39622=ADVANCED_FACE('',(#3934),#1870,.F.);
#39623=ADVANCED_FACE('',(#3935),#1871,.F.);
#39624=ADVANCED_FACE('',(#3936),#1872,.F.);
#39625=ADVANCED_FACE('',(#3937),#1873,.F.);
#39626=ADVANCED_FACE('',(#3938),#1874,.F.);
#39627=ADVANCED_FACE('',(#3939),#1875,.F.);
#39628=ADVANCED_FACE('',(#3940),#1876,.F.);
#39629=ADVANCED_FACE('',(#3941),#1877,.F.);
#39630=ADVANCED_FACE('',(#3942),#1878,.F.);
#39631=ADVANCED_FACE('',(#3943),#1879,.F.);
#39632=ADVANCED_FACE('',(#3944),#1880,.F.);
#39633=ADVANCED_FACE('',(#3945),#1881,.F.);
#39634=ADVANCED_FACE('',(#3946),#1882,.F.);
#39635=ADVANCED_FACE('',(#3947),#1883,.F.);
#39636=ADVANCED_FACE('',(#3948),#1884,.F.);
#39637=ADVANCED_FACE('',(#3949),#1885,.F.);
#39638=ADVANCED_FACE('',(#3950),#1886,.F.);
#39639=ADVANCED_FACE('',(#3951),#1887,.F.);
#39640=ADVANCED_FACE('',(#3952),#1888,.F.);
#39641=ADVANCED_FACE('',(#3953),#1889,.F.);
#39642=ADVANCED_FACE('',(#3954),#1890,.F.);
#39643=ADVANCED_FACE('',(#3955),#1891,.F.);
#39644=ADVANCED_FACE('',(#3956),#1892,.F.);
#39645=ADVANCED_FACE('',(#3957),#1893,.F.);
#39646=ADVANCED_FACE('',(#3958),#1894,.F.);
#39647=ADVANCED_FACE('',(#3959),#1895,.F.);
#39648=ADVANCED_FACE('',(#3960),#1896,.F.);
#39649=ADVANCED_FACE('',(#3961),#1897,.F.);
#39650=ADVANCED_FACE('',(#3962),#1898,.F.);
#39651=ADVANCED_FACE('',(#3963),#1899,.F.);
#39652=ADVANCED_FACE('',(#3964),#1900,.F.);
#39653=ADVANCED_FACE('',(#3965),#1901,.F.);
#39654=ADVANCED_FACE('',(#3966),#1902,.F.);
#39655=ADVANCED_FACE('',(#3967),#1903,.F.);
#39656=ADVANCED_FACE('',(#3968),#1904,.F.);
#39657=ADVANCED_FACE('',(#3969),#1905,.F.);
#39658=ADVANCED_FACE('',(#3970),#1906,.F.);
#39659=ADVANCED_FACE('',(#3971),#1907,.F.);
#39660=ADVANCED_FACE('',(#3972),#1908,.F.);
#39661=ADVANCED_FACE('',(#3973),#1909,.F.);
#39662=ADVANCED_FACE('',(#3974),#1910,.F.);
#39663=ADVANCED_FACE('',(#3975),#1911,.F.);
#39664=ADVANCED_FACE('',(#3976),#1912,.F.);
#39665=ADVANCED_FACE('',(#3977),#1913,.F.);
#39666=ADVANCED_FACE('',(#3978),#1914,.F.);
#39667=ADVANCED_FACE('',(#3979),#1915,.F.);
#39668=ADVANCED_FACE('',(#3980),#1916,.F.);
#39669=ADVANCED_FACE('',(#3981),#1917,.F.);
#39670=ADVANCED_FACE('',(#3982),#1918,.F.);
#39671=ADVANCED_FACE('',(#3983),#1919,.F.);
#39672=ADVANCED_FACE('',(#3984),#1920,.F.);
#39673=ADVANCED_FACE('',(#3985),#1921,.F.);
#39674=ADVANCED_FACE('',(#3986),#1922,.F.);
#39675=ADVANCED_FACE('',(#3987),#1923,.F.);
#39676=ADVANCED_FACE('',(#3988),#1924,.F.);
#39677=ADVANCED_FACE('',(#3989),#1925,.F.);
#39678=ADVANCED_FACE('',(#3990),#1926,.F.);
#39679=ADVANCED_FACE('',(#3991),#1927,.F.);
#39680=ADVANCED_FACE('',(#3992),#1928,.F.);
#39681=ADVANCED_FACE('',(#3993),#1929,.F.);
#39682=ADVANCED_FACE('',(#3994),#1930,.F.);
#39683=ADVANCED_FACE('',(#3995),#1931,.F.);
#39684=ADVANCED_FACE('',(#3996),#1932,.F.);
#39685=ADVANCED_FACE('',(#3997),#1933,.F.);
#39686=ADVANCED_FACE('',(#3998),#1934,.F.);
#39687=ADVANCED_FACE('',(#3999),#1935,.F.);
#39688=ADVANCED_FACE('',(#4000),#1936,.F.);
#39689=ADVANCED_FACE('',(#4001),#1937,.F.);
#39690=ADVANCED_FACE('',(#4002),#1938,.F.);
#39691=ADVANCED_FACE('',(#4003),#1939,.F.);
#39692=ADVANCED_FACE('',(#4004),#1940,.F.);
#39693=ADVANCED_FACE('',(#4005),#1941,.F.);
#39694=ADVANCED_FACE('',(#4006),#1942,.F.);
#39695=ADVANCED_FACE('',(#4007),#1943,.F.);
#39696=ADVANCED_FACE('',(#4008),#1944,.F.);
#39697=ADVANCED_FACE('',(#4009),#1945,.F.);
#39698=ADVANCED_FACE('',(#4010),#1946,.F.);
#39699=ADVANCED_FACE('',(#4011),#1947,.F.);
#39700=ADVANCED_FACE('',(#4012),#1948,.F.);
#39701=ADVANCED_FACE('',(#4013),#1949,.F.);
#39702=ADVANCED_FACE('',(#4014),#1950,.F.);
#39703=ADVANCED_FACE('',(#4015),#1951,.F.);
#39704=ADVANCED_FACE('',(#4016),#1952,.F.);
#39705=ADVANCED_FACE('',(#4017),#1953,.F.);
#39706=ADVANCED_FACE('',(#4018),#1954,.F.);
#39707=ADVANCED_FACE('',(#4019),#1955,.F.);
#39708=ADVANCED_FACE('',(#4020),#1956,.F.);
#39709=ADVANCED_FACE('',(#4021),#1957,.F.);
#39710=ADVANCED_FACE('',(#4022),#1958,.F.);
#39711=ADVANCED_FACE('',(#4023),#1959,.F.);
#39712=ADVANCED_FACE('',(#4024),#1960,.F.);
#39713=ADVANCED_FACE('',(#4025),#1961,.F.);
#39714=ADVANCED_FACE('',(#4026),#1962,.F.);
#39715=ADVANCED_FACE('',(#4027),#1963,.F.);
#39716=ADVANCED_FACE('',(#4028),#1964,.F.);
#39717=ADVANCED_FACE('',(#4029),#1965,.F.);
#39718=ADVANCED_FACE('',(#4030),#1966,.F.);
#39719=ADVANCED_FACE('',(#4031),#1967,.F.);
#39720=ADVANCED_FACE('',(#4032),#1968,.F.);
#39721=ADVANCED_FACE('',(#4033),#1969,.F.);
#39722=ADVANCED_FACE('',(#4034),#1970,.F.);
#39723=ADVANCED_FACE('',(#4035),#1971,.F.);
#39724=ADVANCED_FACE('',(#4036),#1972,.F.);
#39725=ADVANCED_FACE('',(#4037),#1973,.F.);
#39726=ADVANCED_FACE('',(#4038),#1974,.F.);
#39727=ADVANCED_FACE('',(#4039),#1975,.F.);
#39728=ADVANCED_FACE('',(#4040),#1976,.F.);
#39729=ADVANCED_FACE('',(#4041),#1977,.F.);
#39730=ADVANCED_FACE('',(#4042),#1978,.F.);
#39731=ADVANCED_FACE('',(#4043),#1979,.F.);
#39732=ADVANCED_FACE('',(#4044),#1980,.F.);
#39733=ADVANCED_FACE('',(#4045),#1981,.F.);
#39734=ADVANCED_FACE('',(#4046),#1982,.F.);
#39735=ADVANCED_FACE('',(#4047),#1983,.F.);
#39736=ADVANCED_FACE('',(#4048),#1984,.F.);
#39737=ADVANCED_FACE('',(#4049),#1985,.F.);
#39738=ADVANCED_FACE('',(#4050),#1986,.F.);
#39739=ADVANCED_FACE('',(#4051),#1987,.F.);
#39740=ADVANCED_FACE('',(#4052),#1988,.F.);
#39741=ADVANCED_FACE('',(#4053),#1989,.F.);
#39742=ADVANCED_FACE('',(#4054),#1990,.F.);
#39743=ADVANCED_FACE('',(#4055),#1991,.F.);
#39744=ADVANCED_FACE('',(#4056),#1992,.F.);
#39745=ADVANCED_FACE('',(#4057),#1993,.F.);
#39746=ADVANCED_FACE('',(#4058),#1994,.F.);
#39747=ADVANCED_FACE('',(#4059),#1995,.F.);
#39748=ADVANCED_FACE('',(#4060),#1996,.F.);
#39749=ADVANCED_FACE('',(#4061),#1997,.F.);
#39750=ADVANCED_FACE('',(#4062),#1998,.F.);
#39751=ADVANCED_FACE('',(#4063),#1999,.F.);
#39752=ADVANCED_FACE('',(#4064),#2000,.F.);
#39753=ADVANCED_FACE('',(#4065),#2001,.F.);
#39754=ADVANCED_FACE('',(#4066),#2002,.F.);
#39755=ADVANCED_FACE('',(#4067),#2003,.F.);
#39756=ADVANCED_FACE('',(#4068),#2004,.F.);
#39757=ADVANCED_FACE('',(#4069),#2005,.F.);
#39758=ADVANCED_FACE('',(#4070),#2006,.F.);
#39759=ADVANCED_FACE('',(#4071),#2007,.F.);
#39760=ADVANCED_FACE('',(#4072),#2008,.F.);
#39761=ADVANCED_FACE('',(#4073),#2009,.F.);
#39762=ADVANCED_FACE('',(#4074),#2010,.F.);
#39763=ADVANCED_FACE('',(#4075),#2011,.F.);
#39764=ADVANCED_FACE('',(#4076),#2012,.F.);
#39765=ADVANCED_FACE('',(#4077),#2013,.F.);
#39766=ADVANCED_FACE('',(#4078),#2014,.F.);
#39767=ADVANCED_FACE('',(#4079),#2015,.F.);
#39768=ADVANCED_FACE('',(#4080),#2016,.F.);
#39769=ADVANCED_FACE('',(#4081),#2017,.F.);
#39770=ADVANCED_FACE('',(#4082),#2018,.F.);
#39771=ADVANCED_FACE('',(#4083),#2019,.F.);
#39772=ADVANCED_FACE('',(#4084),#2020,.F.);
#39773=ADVANCED_FACE('',(#4085),#2021,.F.);
#39774=ADVANCED_FACE('',(#4086),#2022,.F.);
#39775=ADVANCED_FACE('',(#4087),#2023,.F.);
#39776=ADVANCED_FACE('',(#4088),#2024,.F.);
#39777=ADVANCED_FACE('',(#4089),#2025,.F.);
#39778=ADVANCED_FACE('',(#4090),#2026,.F.);
#39779=ADVANCED_FACE('',(#4091),#2027,.F.);
#39780=ADVANCED_FACE('',(#4092),#2028,.F.);
#39781=ADVANCED_FACE('',(#4093),#2029,.F.);
#39782=ADVANCED_FACE('',(#4094),#2030,.F.);
#39783=ADVANCED_FACE('',(#4095),#2031,.F.);
#39784=ADVANCED_FACE('',(#4096),#2032,.F.);
#39785=ADVANCED_FACE('',(#4097),#2033,.F.);
#39786=ADVANCED_FACE('',(#4098),#2034,.F.);
#39787=ADVANCED_FACE('',(#4099),#2035,.F.);
#39788=ADVANCED_FACE('',(#4100),#2036,.F.);
#39789=ADVANCED_FACE('',(#4101),#2037,.F.);
#39790=ADVANCED_FACE('',(#4102),#2038,.F.);
#39791=ADVANCED_FACE('',(#4103),#2039,.F.);
#39792=ADVANCED_FACE('',(#4104),#2040,.F.);
#39793=ADVANCED_FACE('',(#4105),#2041,.F.);
#39794=ADVANCED_FACE('',(#4106),#2042,.F.);
#39795=ADVANCED_FACE('',(#4107),#2043,.F.);
#39796=ADVANCED_FACE('',(#4108),#2044,.F.);
#39797=ADVANCED_FACE('',(#4109),#2045,.F.);
#39798=ADVANCED_FACE('',(#4110),#2046,.F.);
#39799=ADVANCED_FACE('',(#4111),#2047,.F.);
#39800=ADVANCED_FACE('',(#4112),#2048,.F.);
#39801=ADVANCED_FACE('',(#4113),#2049,.F.);
#39802=ADVANCED_FACE('',(#4114),#2050,.F.);
#39803=ADVANCED_FACE('',(#4115),#2051,.F.);
#39804=ADVANCED_FACE('',(#4116),#2052,.F.);
#39805=ADVANCED_FACE('',(#4117),#2053,.F.);
#39806=ADVANCED_FACE('',(#4118),#2054,.F.);
#39807=ADVANCED_FACE('',(#4119),#2055,.F.);
#39808=ADVANCED_FACE('',(#4120),#2056,.F.);
#39809=ADVANCED_FACE('',(#4121),#2057,.F.);
#39810=ADVANCED_FACE('',(#4122),#2058,.F.);
#39811=ADVANCED_FACE('',(#4123),#2059,.F.);
#39812=ADVANCED_FACE('',(#4124),#2060,.F.);
#39813=ADVANCED_FACE('',(#4125),#2061,.F.);
#39814=ADVANCED_FACE('',(#4126),#2062,.F.);
#39815=ADVANCED_FACE('',(#4127),#2063,.F.);
#39816=ADVANCED_FACE('',(#4128),#2064,.F.);
#39817=ADVANCED_FACE('',(#4129),#2065,.F.);
#39818=ADVANCED_FACE('',(#4130),#2066,.F.);
#39819=ADVANCED_FACE('',(#4131),#2067,.F.);
#39820=ADVANCED_FACE('',(#4132),#2068,.F.);
#39821=ADVANCED_FACE('',(#4133),#2069,.F.);
#39822=ADVANCED_FACE('',(#4134),#2070,.F.);
#39823=ADVANCED_FACE('',(#4135),#2071,.F.);
#39824=ADVANCED_FACE('',(#4136),#2072,.F.);
#39825=ADVANCED_FACE('',(#4137),#2073,.F.);
#39826=ADVANCED_FACE('',(#4138),#2074,.F.);
#39827=ADVANCED_FACE('',(#4139),#2075,.F.);
#39828=ADVANCED_FACE('',(#4140),#2076,.F.);
#39829=ADVANCED_FACE('',(#4141),#2077,.F.);
#39830=ADVANCED_FACE('',(#4142),#2078,.F.);
#39831=ADVANCED_FACE('',(#4143),#2079,.F.);
#39832=ADVANCED_FACE('',(#4144),#2080,.F.);
#39833=ADVANCED_FACE('',(#4145),#2081,.F.);
#39834=ADVANCED_FACE('',(#4146),#2082,.F.);
#39835=ADVANCED_FACE('',(#4147),#2083,.F.);
#39836=ADVANCED_FACE('',(#4148),#2084,.F.);
#39837=ADVANCED_FACE('',(#4149),#2085,.F.);
#39838=ADVANCED_FACE('',(#4150),#2086,.F.);
#39839=ADVANCED_FACE('',(#4151),#2087,.F.);
#39840=ADVANCED_FACE('',(#4152),#2088,.F.);
#39841=ADVANCED_FACE('',(#4153),#2089,.F.);
#39842=ADVANCED_FACE('',(#4154),#2090,.F.);
#39843=ADVANCED_FACE('',(#4155),#2091,.F.);
#39844=ADVANCED_FACE('',(#4156),#2092,.F.);
#39845=ADVANCED_FACE('',(#4157),#2093,.F.);
#39846=ADVANCED_FACE('',(#4158),#2094,.F.);
#39847=ADVANCED_FACE('',(#4159),#2095,.F.);
#39848=ADVANCED_FACE('',(#4160),#2096,.F.);
#39849=ADVANCED_FACE('',(#4161),#2097,.F.);
#39850=ADVANCED_FACE('',(#4162),#2098,.F.);
#39851=ADVANCED_FACE('',(#4163),#2099,.F.);
#39852=ADVANCED_FACE('',(#4164),#2100,.F.);
#39853=ADVANCED_FACE('',(#4165),#2101,.F.);
#39854=ADVANCED_FACE('',(#4166),#2102,.F.);
#39855=ADVANCED_FACE('',(#4167),#2103,.F.);
#39856=ADVANCED_FACE('',(#4168),#2104,.F.);
#39857=ADVANCED_FACE('',(#4169),#2105,.F.);
#39858=ADVANCED_FACE('',(#4170),#2106,.F.);
#39859=ADVANCED_FACE('',(#4171),#2107,.F.);
#39860=ADVANCED_FACE('',(#4172),#2108,.F.);
#39861=ADVANCED_FACE('',(#4173),#2109,.F.);
#39862=ADVANCED_FACE('',(#4174),#2110,.F.);
#39863=ADVANCED_FACE('',(#4175),#2111,.F.);
#39864=ADVANCED_FACE('',(#4176),#2112,.F.);
#39865=ADVANCED_FACE('',(#4177),#2113,.F.);
#39866=ADVANCED_FACE('',(#4178),#2114,.F.);
#39867=ADVANCED_FACE('',(#4179),#2115,.F.);
#39868=ADVANCED_FACE('',(#4180),#2116,.F.);
#39869=ADVANCED_FACE('',(#4181),#2117,.F.);
#39870=ADVANCED_FACE('',(#4182),#2118,.F.);
#39871=ADVANCED_FACE('',(#4183),#2119,.F.);
#39872=ADVANCED_FACE('',(#4184),#2120,.F.);
#39873=ADVANCED_FACE('',(#4185),#2121,.F.);
#39874=ADVANCED_FACE('',(#4186),#2122,.F.);
#39875=ADVANCED_FACE('',(#4187),#2123,.F.);
#39876=ADVANCED_FACE('',(#4188),#2124,.F.);
#39877=ADVANCED_FACE('',(#4189),#2125,.F.);
#39878=ADVANCED_FACE('',(#4190),#2126,.F.);
#39879=ADVANCED_FACE('',(#4191),#2127,.F.);
#39880=ADVANCED_FACE('',(#4192),#2128,.F.);
#39881=ADVANCED_FACE('',(#4193),#2129,.F.);
#39882=ADVANCED_FACE('',(#4194),#2130,.F.);
#39883=ADVANCED_FACE('',(#4195),#2131,.F.);
#39884=ADVANCED_FACE('',(#4196),#2132,.F.);
#39885=ADVANCED_FACE('',(#4197),#2133,.F.);
#39886=ADVANCED_FACE('',(#4198),#2134,.F.);
#39887=ADVANCED_FACE('',(#4199),#2135,.F.);
#39888=ADVANCED_FACE('',(#4200),#2136,.F.);
#39889=ADVANCED_FACE('',(#4201),#2137,.F.);
#39890=ADVANCED_FACE('',(#4202),#2138,.F.);
#39891=ADVANCED_FACE('',(#4203),#2139,.F.);
#39892=ADVANCED_FACE('',(#4204),#2140,.F.);
#39893=ADVANCED_FACE('',(#4205),#2141,.F.);
#39894=ADVANCED_FACE('',(#4206),#2142,.F.);
#39895=ADVANCED_FACE('',(#4207),#2143,.F.);
#39896=ADVANCED_FACE('',(#4208),#2144,.F.);
#39897=ADVANCED_FACE('',(#4209),#2145,.F.);
#39898=ADVANCED_FACE('',(#4210),#2146,.F.);
#39899=ADVANCED_FACE('',(#4211),#2147,.F.);
#39900=ADVANCED_FACE('',(#4212),#2148,.F.);
#39901=ADVANCED_FACE('',(#4213),#2149,.F.);
#39902=ADVANCED_FACE('',(#4214),#2150,.F.);
#39903=ADVANCED_FACE('',(#4215),#2151,.F.);
#39904=ADVANCED_FACE('',(#4216),#2152,.F.);
#39905=ADVANCED_FACE('',(#4217),#2153,.F.);
#39906=ADVANCED_FACE('',(#4218),#2154,.F.);
#39907=ADVANCED_FACE('',(#4219),#2155,.F.);
#39908=ADVANCED_FACE('',(#4220),#2156,.F.);
#39909=ADVANCED_FACE('',(#4221),#2157,.F.);
#39910=ADVANCED_FACE('',(#4222),#2158,.F.);
#39911=ADVANCED_FACE('',(#4223),#2159,.F.);
#39912=ADVANCED_FACE('',(#4224),#2160,.F.);
#39913=ADVANCED_FACE('',(#4225),#2161,.F.);
#39914=ADVANCED_FACE('',(#4226),#2162,.F.);
#39915=ADVANCED_FACE('',(#4227),#2163,.F.);
#39916=ADVANCED_FACE('',(#4228),#2164,.F.);
#39917=ADVANCED_FACE('',(#4229),#2165,.F.);
#39918=ADVANCED_FACE('',(#4230),#2166,.F.);
#39919=ADVANCED_FACE('',(#4231),#2167,.F.);
#39920=ADVANCED_FACE('',(#4232),#2168,.F.);
#39921=ADVANCED_FACE('',(#4233),#2169,.F.);
#39922=ADVANCED_FACE('',(#4234),#2170,.F.);
#39923=ADVANCED_FACE('',(#4235),#2171,.F.);
#39924=ADVANCED_FACE('',(#4236),#2172,.F.);
#39925=ADVANCED_FACE('',(#4237),#2173,.F.);
#39926=ADVANCED_FACE('',(#4238),#2174,.F.);
#39927=ADVANCED_FACE('',(#4239),#2175,.F.);
#39928=ADVANCED_FACE('',(#4240),#2176,.F.);
#39929=ADVANCED_FACE('',(#4241),#2177,.F.);
#39930=ADVANCED_FACE('',(#4242),#2178,.F.);
#39931=ADVANCED_FACE('',(#4243),#2179,.F.);
#39932=ADVANCED_FACE('',(#4244),#2180,.F.);
#39937=CLOSED_SHELL('',(#38765,#38766,#38767,#38768,#38769,#38770,#38771,
#38772,#38773,#38774,#38775,#38776,#38777,#38778,#38779,#38780,#38781,#38782,
#38783,#38784,#38785,#38786,#38787,#38788,#38789,#38790,#38791,#38792,#38793,
#38794,#38795,#38796,#38797,#38798,#38799,#38800,#38801,#38802,#38803,#38804,
#38805,#38806,#38807,#38808,#38809,#38810,#38811,#38812,#38813,#38814,#38815,
#38816,#38817,#38818,#38819,#38820,#38821,#38822,#38823,#38824,#38825,#38826,
#38827,#38828,#38829,#38830,#38831,#38832,#38833,#38834,#38835,#38836,#38837,
#38838,#38839,#38840,#38841,#38842,#38843,#38844,#38845,#38846,#38847,#38848,
#38849,#38850,#38851,#38852,#38853,#38854,#38855,#38856,#38857,#38858,#38859,
#38860,#38861,#38862,#38863,#38864,#38865,#38866,#38867,#38868,#38869,#38870,
#38871,#38872,#38873,#38874,#38875,#38876,#38877,#38878,#38879,#38880,#38881,
#38882,#38883,#38884,#38885,#38886,#38887,#38888,#38889,#38890,#38891,#38892,
#38893,#38894,#38895,#38896,#38897,#38898,#38899,#38900,#38901,#38902,#38903,
#38904,#38905,#38906,#38907,#38908,#38909,#38910,#38911,#38912,#38913,#38914,
#38915,#38916,#38917,#38918,#38919,#38920,#38921,#38922,#38923,#38924,#38925,
#38926,#38927,#38928,#38929,#38930,#38931,#38932,#38933,#38934,#38935,#38936,
#38937,#38938,#38939,#38940,#38941,#38942,#38943,#38944,#38945,#38946,#38947,
#38948,#38949,#38950,#38951,#38952,#38953,#38954,#38955,#38956,#38957,#38958,
#38959,#38960,#38961,#38962,#38963,#38964,#38965,#38966,#38967,#38968,#38969,
#38970,#38971,#38972,#38973,#38974,#38975,#38976,#38977,#38978,#38979,#38980,
#38981,#38982,#38983,#38984,#38985,#38986,#38987,#38988,#38989,#38990,#38991,
#38992,#38993,#38994,#38995,#38996,#38997,#38998,#38999,#39000,#39001,#39002,
#39003,#39004,#39005,#39006,#39007,#39008,#39009,#39010,#39011,#39012,#39013,
#39014,#39015,#39016,#39017,#39018,#39019,#39020,#39021,#39022,#39023,#39024,
#39025,#39026,#39027,#39028,#39029,#39030,#39031,#39032,#39033,#39034,#39035,
#39036,#39037,#39038,#39039,#39040,#39041,#39042,#39043,#39044,#39045,#39046,
#39047,#39048,#39049,#39050,#39051,#39052,#39053,#39054,#39055,#39056,#39057,
#39058,#39059,#39060,#39061,#39062,#39063,#39064,#39065,#39066,#39067,#39068,
#39069,#39070,#39071,#39072,#39073,#39074,#39075,#39076,#39077,#39078,#39079,
#39080,#39081,#39082,#39083,#39084,#39085,#39086,#39087,#39088,#39089,#39090,
#39091,#39092,#39093,#39094,#39095,#39096,#39097,#39098,#39099,#39100,#39101,
#39102,#39103,#39104,#39105,#39106,#39107,#39108,#39109,#39110,#39111,#39112,
#39113,#39114,#39115,#39116,#39117,#39118,#39119,#39120,#39121,#39122,#39123,
#39124,#39125,#39126,#39127,#39128,#39129,#39130,#39131,#39132,#39133,#39134,
#39135,#39136,#39137,#39138,#39139,#39140,#39141,#39142,#39143,#39144,#39145,
#39146,#39147,#39148,#39149,#39150,#39151,#39152,#39153,#39154,#39155,#39156,
#39157,#39158,#39159,#39160,#39161,#39162,#39163,#39164,#39165,#39166,#39167,
#39168,#39169,#39170,#39171,#39172,#39173,#39174,#39175,#39176,#39177,#39178,
#39179,#39180,#39181,#39182,#39183,#39184,#39185,#39186,#39187,#39188,#39189,
#39190,#39191,#39192,#39193,#39194,#39195,#39196,#39197,#39198,#39199,#39200,
#39201,#39202,#39203,#39204,#39205,#39206,#39207,#39208,#39209,#39210,#39211,
#39212,#39213,#39214,#39215,#39216,#39217,#39218,#39219,#39220,#39221,#39222,
#39223,#39224,#39225,#39226,#39227,#39228,#39229,#39230,#39231,#39232,#39233,
#39234,#39235,#39236,#39237,#39238,#39239,#39240,#39241,#39242,#39243,#39244,
#39245,#39246,#39247,#39248,#39249,#39250,#39251,#39252,#39253,#39254,#39255,
#39256,#39257,#39258,#39259,#39260,#39261,#39262,#39263,#39264,#39265,#39266,
#39267,#39268,#39269,#39270,#39271,#39272,#39273,#39274,#39275,#39276,#39277,
#39278,#39279,#39280,#39281,#39282,#39283,#39284,#39285,#39286,#39287,#39288,
#39289,#39290,#39291,#39292,#39293,#39294,#39295,#39296,#39297,#39298,#39299,
#39300,#39301,#39302,#39303,#39304,#39305,#39306,#39307,#39308,#39309,#39310,
#39311,#39312,#39313,#39314,#39315,#39316,#39317,#39318,#39319,#39320,#39321,
#39322,#39323,#39324,#39325,#39326,#39327,#39328,#39329,#39330,#39331,#39332,
#39333,#39334,#39335,#39336,#39337,#39338,#39339,#39340,#39341,#39342,#39343,
#39344,#39345,#39346,#39347,#39348,#39349,#39350,#39351,#39352,#39353,#39354,
#39355,#39356,#39357,#39358,#39359,#39360,#39361,#39362,#39363,#39364,#39365,
#39366,#39367,#39368,#39369,#39370,#39371,#39372,#39373,#39374,#39375,#39376,
#39377,#39378,#39379,#39380,#39381,#39382,#39383,#39384,#39385,#39386,#39387,
#39388,#39389,#39390,#39391,#39392,#39393,#39394,#39395,#39396,#39397,#39398,
#39399,#39400,#39401,#39402,#39403,#39404,#39405,#39406,#39407,#39408,#39409,
#39410,#39411,#39412,#39413,#39414,#39415,#39416,#39417,#39418,#39419,#39420,
#39421,#39422,#39423,#39424,#39425,#39426,#39427,#39428,#39429,#39430,#39431,
#39432,#39433,#39434,#39435,#39436,#39437,#39438,#39439,#39440,#39441,#39442,
#39443,#39444,#39445,#39446,#39447,#39448,#39449,#39450,#39451,#39452,#39453,
#39454,#39455,#39456,#39457,#39458,#39459,#39460,#39461,#39462,#39463,#39464,
#39465,#39466,#39467,#39468,#39469,#39470,#39471,#39472,#39473,#39474,#39475,
#39476,#39477,#39478,#39479,#39480,#39481,#39482,#39483,#39484,#39485,#39486,
#39487,#39488,#39489,#39490,#39491,#39492,#39493,#39494,#39495,#39496,#39497,
#39498,#39499,#39500,#39501,#39502,#39503,#39504,#39505,#39506,#39507,#39508,
#39509,#39510,#39511,#39512,#39513,#39514,#39515,#39516,#39517,#39518,#39519,
#39520,#39521,#39522,#39523,#39524,#39525,#39526,#39527,#39528,#39529,#39530,
#39531,#39532,#39533,#39534,#39535,#39536,#39537,#39538,#39539,#39540,#39541,
#39542,#39543,#39544,#39545,#39546,#39547,#39548,#39549,#39550,#39551,#39552,
#39553,#39554,#39555,#39556,#39557,#39558,#39559,#39560,#39561,#39562,#39563,
#39564,#39565,#39566,#39567,#39568,#39569,#39570,#39571,#39572,#39573,#39574,
#39575,#39576,#39577,#39578,#39579,#39580,#39581,#39582,#39583,#39584,#39585,
#39586,#39587,#39588,#39589,#39590,#39591,#39592,#39593,#39594,#39595,#39596,
#39597,#39598,#39599,#39600,#39601,#39602,#39603,#39604,#39605,#39606,#39607,
#39608,#39609,#39610,#39611,#39612,#39613,#39614,#39615,#39616,#39617,#39618,
#39619,#39620,#39621,#39622,#39623,#39624,#39625,#39626,#39627,#39628,#39629,
#39630,#39631,#39632,#39633,#39634,#39635,#39636,#39637,#39638,#39639,#39640,
#39641,#39642,#39643,#39644,#39645,#39646,#39647,#39648,#39649,#39650,#39651,
#39652,#39653,#39654,#39655,#39656,#39657,#39658,#39659,#39660,#39661,#39662,
#39663,#39664,#39665,#39666,#39667,#39668,#39669,#39670,#39671,#39672,#39673,
#39674,#39675,#39676,#39677,#39678,#39679,#39680,#39681,#39682,#39683,#39684,
#39685,#39686,#39687,#39688,#39689,#39690,#39691,#39692,#39693,#39694,#39695,
#39696,#39697,#39698,#39699,#39700,#39701,#39702,#39703,#39704,#39705,#39706,
#39707,#39708,#39709,#39710,#39711,#39712,#39713,#39714,#39715,#39716,#39717,
#39718,#39719,#39720,#39721,#39722,#39723,#39724,#39725,#39726,#39727,#39728,
#39729,#39730,#39731,#39732,#39733,#39734,#39735,#39736,#39737,#39738,#39739,
#39740,#39741,#39742,#39743,#39744,#39745,#39746,#39747,#39748,#39749,#39750,
#39751,#39752,#39753,#39754,#39755,#39756,#39757,#39758,#39759,#39760,#39761,
#39762,#39763,#39764,#39765,#39766,#39767,#39768,#39769,#39770,#39771,#39772,
#39773,#39774,#39775,#39776,#39777,#39778,#39779,#39780,#39781,#39782,#39783,
#39784,#39785,#39786,#39787,#39788,#39789,#39790,#39791,#39792,#39793,#39794,
#39795,#39796,#39797,#39798,#39799,#39800,#39801,#39802,#39803,#39804,#39805,
#39806,#39807,#39808,#39809,#39810,#39811,#39812,#39813,#39814,#39815,#39816,
#39817,#39818,#39819,#39820,#39821,#39822,#39823,#39824,#39825,#39826,#39827,
#39828,#39829,#39830,#39831,#39832,#39833,#39834,#39835,#39836,#39837,#39838,
#39839,#39840,#39841,#39842,#39843,#39844,#39845,#39846,#39847,#39848,#39849,
#39850,#39851,#39852,#39853,#39854,#39855,#39856,#39857,#39858,#39859,#39860,
#39861,#39862,#39863,#39864,#39865,#39866,#39867,#39868,#39869,#39870,#39871,
#39872,#39873,#39874,#39875,#39876,#39877,#39878,#39879,#39880,#39881,#39882,
#39883,#39884,#39885,#39886,#39887,#39888,#39889,#39890,#39891,#39892,#39893,
#39894,#39895,#39896,#39897,#39898,#39899,#39900,#39901,#39902,#39903,#39904,
#39905,#39906,#39907,#39908,#39909,#39910,#39911,#39912,#39913,#39914,#39915,
#39916,#39917,#39918,#39919,#39920,#39921,#39922,#39923,#39924,#39925,#39926,
#39927,#39928,#39929,#39930,#39931,#39932));
#41307=AXIS2_PLACEMENT_3D('',#58348,#46601,#46602);
#41308=AXIS2_PLACEMENT_3D('',#58349,#46603,#46604);
#41309=AXIS2_PLACEMENT_3D('',#58351,#46605,#46606);
#41310=AXIS2_PLACEMENT_3D('',#58353,#46607,#46608);
#41311=AXIS2_PLACEMENT_3D('',#58354,#46609,#46610);
#41312=AXIS2_PLACEMENT_3D('',#58355,#46611,#46612);
#41313=AXIS2_PLACEMENT_3D('',#58357,#46613,#46614);
#41314=AXIS2_PLACEMENT_3D('',#58359,#46615,#46616);
#41315=AXIS2_PLACEMENT_3D('',#58360,#46617,#46618);
#41316=AXIS2_PLACEMENT_3D('',#58361,#46619,#46620);
#41317=AXIS2_PLACEMENT_3D('',#58363,#46621,#46622);
#41318=AXIS2_PLACEMENT_3D('',#58364,#46623,#46624);
#41319=AXIS2_PLACEMENT_3D('',#58365,#46625,#46626);
#41320=AXIS2_PLACEMENT_3D('',#58367,#46627,#46628);
#41321=AXIS2_PLACEMENT_3D('',#58368,#46629,#46630);
#41322=AXIS2_PLACEMENT_3D('',#58369,#46631,#46632);
#41323=AXIS2_PLACEMENT_3D('',#58394,#46645,#46646);
#41324=AXIS2_PLACEMENT_3D('',#58419,#46659,#46660);
#41325=AXIS2_PLACEMENT_3D('',#58422,#46663,#46664);
#41326=AXIS2_PLACEMENT_3D('',#58425,#46667,#46668);
#41327=AXIS2_PLACEMENT_3D('',#58428,#46671,#46672);
#41328=AXIS2_PLACEMENT_3D('',#58431,#46675,#46676);
#41329=AXIS2_PLACEMENT_3D('',#58432,#46677,#46678);
#41330=AXIS2_PLACEMENT_3D('',#58435,#46681,#46682);
#41331=AXIS2_PLACEMENT_3D('',#58437,#46684,#46685);
#41332=AXIS2_PLACEMENT_3D('',#58439,#46687,#46688);
#41333=AXIS2_PLACEMENT_3D('',#58443,#46690,#46691);
#41334=AXIS2_PLACEMENT_3D('',#58444,#46692,#46693);
#41335=AXIS2_PLACEMENT_3D('',#58445,#46694,#46695);
#41336=AXIS2_PLACEMENT_3D('',#58447,#46696,#46697);
#41337=AXIS2_PLACEMENT_3D('',#58450,#46699,#46700);
#41338=AXIS2_PLACEMENT_3D('',#58451,#46701,#46702);
#41339=AXIS2_PLACEMENT_3D('',#58453,#46704,#46705);
#41340=AXIS2_PLACEMENT_3D('',#58455,#46707,#46708);
#41341=AXIS2_PLACEMENT_3D('',#58457,#46709,#46710);
#41342=AXIS2_PLACEMENT_3D('',#58460,#46712,#46713);
#41343=AXIS2_PLACEMENT_3D('',#58461,#46714,#46715);
#41344=AXIS2_PLACEMENT_3D('',#58465,#46717,#46718);
#41345=AXIS2_PLACEMENT_3D('',#58466,#46719,#46720);
#41346=AXIS2_PLACEMENT_3D('',#58467,#46721,#46722);
#41347=AXIS2_PLACEMENT_3D('',#58469,#46724,#46725);
#41348=AXIS2_PLACEMENT_3D('',#58471,#46727,#46728);
#41349=AXIS2_PLACEMENT_3D('',#58474,#46729,#46730);
#41350=AXIS2_PLACEMENT_3D('',#58478,#46732,#46733);
#41351=AXIS2_PLACEMENT_3D('',#58480,#46735,#46736);
#41352=AXIS2_PLACEMENT_3D('',#58489,#46741,#46742);
#41353=AXIS2_PLACEMENT_3D('',#58492,#46743,#46744);
#41354=AXIS2_PLACEMENT_3D('',#58496,#46746,#46747);
#41355=AXIS2_PLACEMENT_3D('',#58498,#46749,#46750);
#41356=AXIS2_PLACEMENT_3D('',#58501,#46753,#46754);
#41357=AXIS2_PLACEMENT_3D('',#58506,#46759,#46760);
#41358=AXIS2_PLACEMENT_3D('',#58508,#46762,#46763);
#41359=AXIS2_PLACEMENT_3D('',#58512,#46767,#46768);
#41360=AXIS2_PLACEMENT_3D('',#58513,#46769,#46770);
#41361=AXIS2_PLACEMENT_3D('',#58514,#46771,#46772);
#41362=AXIS2_PLACEMENT_3D('',#58515,#46773,#46774);
#41363=AXIS2_PLACEMENT_3D('',#58519,#46776,#46777);
#41364=AXIS2_PLACEMENT_3D('',#58520,#46778,#46779);
#41365=AXIS2_PLACEMENT_3D('',#58521,#46780,#46781);
#41366=AXIS2_PLACEMENT_3D('',#58523,#46782,#46783);
#41367=AXIS2_PLACEMENT_3D('',#58526,#46785,#46786);
#41368=AXIS2_PLACEMENT_3D('',#58527,#46787,#46788);
#41369=AXIS2_PLACEMENT_3D('',#58529,#46790,#46791);
#41370=AXIS2_PLACEMENT_3D('',#58531,#46793,#46794);
#41371=AXIS2_PLACEMENT_3D('',#58533,#46795,#46796);
#41372=AXIS2_PLACEMENT_3D('',#58536,#46798,#46799);
#41373=AXIS2_PLACEMENT_3D('',#58537,#46800,#46801);
#41374=AXIS2_PLACEMENT_3D('',#58541,#46803,#46804);
#41375=AXIS2_PLACEMENT_3D('',#58542,#46805,#46806);
#41376=AXIS2_PLACEMENT_3D('',#58543,#46807,#46808);
#41377=AXIS2_PLACEMENT_3D('',#58545,#46810,#46811);
#41378=AXIS2_PLACEMENT_3D('',#58547,#46813,#46814);
#41379=AXIS2_PLACEMENT_3D('',#58550,#46815,#46816);
#41380=AXIS2_PLACEMENT_3D('',#58554,#46818,#46819);
#41381=AXIS2_PLACEMENT_3D('',#58556,#46821,#46822);
#41382=AXIS2_PLACEMENT_3D('',#58565,#46827,#46828);
#41383=AXIS2_PLACEMENT_3D('',#58568,#46829,#46830);
#41384=AXIS2_PLACEMENT_3D('',#58572,#46832,#46833);
#41385=AXIS2_PLACEMENT_3D('',#58574,#46835,#46836);
#41386=AXIS2_PLACEMENT_3D('',#58577,#46839,#46840);
#41387=AXIS2_PLACEMENT_3D('',#58582,#46845,#46846);
#41388=AXIS2_PLACEMENT_3D('',#58584,#46848,#46849);
#41389=AXIS2_PLACEMENT_3D('',#58588,#46853,#46854);
#41390=AXIS2_PLACEMENT_3D('',#58589,#46855,#46856);
#41391=AXIS2_PLACEMENT_3D('',#58590,#46857,#46858);
#41392=AXIS2_PLACEMENT_3D('',#58591,#46859,#46860);
#41393=AXIS2_PLACEMENT_3D('',#60824,#47977,#47978);
#41394=AXIS2_PLACEMENT_3D('',#63057,#49095,#49096);
#41395=AXIS2_PLACEMENT_3D('',#63060,#49099,#49100);
#41396=AXIS2_PLACEMENT_3D('',#63062,#49102,#49103);
#41397=AXIS2_PLACEMENT_3D('',#63064,#49105,#49106);
#41398=AXIS2_PLACEMENT_3D('',#63066,#49108,#49109);
#41399=AXIS2_PLACEMENT_3D('',#63068,#49111,#49112);
#41400=AXIS2_PLACEMENT_3D('',#63069,#49113,#49114);
#41401=AXIS2_PLACEMENT_3D('',#63072,#49117,#49118);
#41402=AXIS2_PLACEMENT_3D('',#63074,#49120,#49121);
#41403=AXIS2_PLACEMENT_3D('',#63076,#49123,#49124);
#41404=AXIS2_PLACEMENT_3D('',#63078,#49126,#49127);
#41405=AXIS2_PLACEMENT_3D('',#63080,#49129,#49130);
#41406=AXIS2_PLACEMENT_3D('',#63081,#49131,#49132);
#41407=AXIS2_PLACEMENT_3D('',#63084,#49135,#49136);
#41408=AXIS2_PLACEMENT_3D('',#63086,#49138,#49139);
#41409=AXIS2_PLACEMENT_3D('',#63088,#49141,#49142);
#41410=AXIS2_PLACEMENT_3D('',#63090,#49144,#49145);
#41411=AXIS2_PLACEMENT_3D('',#63092,#49147,#49148);
#41412=AXIS2_PLACEMENT_3D('',#63093,#49149,#49150);
#41413=AXIS2_PLACEMENT_3D('',#63096,#49153,#49154);
#41414=AXIS2_PLACEMENT_3D('',#63098,#49156,#49157);
#41415=AXIS2_PLACEMENT_3D('',#63100,#49159,#49160);
#41416=AXIS2_PLACEMENT_3D('',#63102,#49162,#49163);
#41417=AXIS2_PLACEMENT_3D('',#63104,#49165,#49166);
#41418=AXIS2_PLACEMENT_3D('',#63105,#49167,#49168);
#41419=AXIS2_PLACEMENT_3D('',#63108,#49171,#49172);
#41420=AXIS2_PLACEMENT_3D('',#63110,#49174,#49175);
#41421=AXIS2_PLACEMENT_3D('',#63112,#49177,#49178);
#41422=AXIS2_PLACEMENT_3D('',#63114,#49180,#49181);
#41423=AXIS2_PLACEMENT_3D('',#63116,#49183,#49184);
#41424=AXIS2_PLACEMENT_3D('',#63117,#49185,#49186);
#41425=AXIS2_PLACEMENT_3D('',#63120,#49189,#49190);
#41426=AXIS2_PLACEMENT_3D('',#63122,#49192,#49193);
#41427=AXIS2_PLACEMENT_3D('',#63124,#49195,#49196);
#41428=AXIS2_PLACEMENT_3D('',#63126,#49198,#49199);
#41429=AXIS2_PLACEMENT_3D('',#63128,#49201,#49202);
#41430=AXIS2_PLACEMENT_3D('',#63129,#49203,#49204);
#41431=AXIS2_PLACEMENT_3D('',#63132,#49207,#49208);
#41432=AXIS2_PLACEMENT_3D('',#63134,#49210,#49211);
#41433=AXIS2_PLACEMENT_3D('',#63136,#49213,#49214);
#41434=AXIS2_PLACEMENT_3D('',#63138,#49216,#49217);
#41435=AXIS2_PLACEMENT_3D('',#63140,#49219,#49220);
#41436=AXIS2_PLACEMENT_3D('',#63141,#49221,#49222);
#41437=AXIS2_PLACEMENT_3D('',#63144,#49225,#49226);
#41438=AXIS2_PLACEMENT_3D('',#63146,#49228,#49229);
#41439=AXIS2_PLACEMENT_3D('',#63148,#49231,#49232);
#41440=AXIS2_PLACEMENT_3D('',#63150,#49234,#49235);
#41441=AXIS2_PLACEMENT_3D('',#63152,#49237,#49238);
#41442=AXIS2_PLACEMENT_3D('',#63153,#49239,#49240);
#41443=AXIS2_PLACEMENT_3D('',#63156,#49243,#49244);
#41444=AXIS2_PLACEMENT_3D('',#63158,#49246,#49247);
#41445=AXIS2_PLACEMENT_3D('',#63160,#49249,#49250);
#41446=AXIS2_PLACEMENT_3D('',#63162,#49252,#49253);
#41447=AXIS2_PLACEMENT_3D('',#63164,#49255,#49256);
#41448=AXIS2_PLACEMENT_3D('',#63165,#49257,#49258);
#41449=AXIS2_PLACEMENT_3D('',#63168,#49261,#49262);
#41450=AXIS2_PLACEMENT_3D('',#63170,#49264,#49265);
#41451=AXIS2_PLACEMENT_3D('',#63172,#49267,#49268);
#41452=AXIS2_PLACEMENT_3D('',#63174,#49270,#49271);
#41453=AXIS2_PLACEMENT_3D('',#63176,#49273,#49274);
#41454=AXIS2_PLACEMENT_3D('',#63177,#49275,#49276);
#41455=AXIS2_PLACEMENT_3D('',#63180,#49279,#49280);
#41456=AXIS2_PLACEMENT_3D('',#63182,#49282,#49283);
#41457=AXIS2_PLACEMENT_3D('',#63184,#49285,#49286);
#41458=AXIS2_PLACEMENT_3D('',#63186,#49288,#49289);
#41459=AXIS2_PLACEMENT_3D('',#63188,#49291,#49292);
#41460=AXIS2_PLACEMENT_3D('',#63189,#49293,#49294);
#41461=AXIS2_PLACEMENT_3D('',#63192,#49297,#49298);
#41462=AXIS2_PLACEMENT_3D('',#63194,#49300,#49301);
#41463=AXIS2_PLACEMENT_3D('',#63196,#49303,#49304);
#41464=AXIS2_PLACEMENT_3D('',#63198,#49306,#49307);
#41465=AXIS2_PLACEMENT_3D('',#63200,#49309,#49310);
#41466=AXIS2_PLACEMENT_3D('',#63201,#49311,#49312);
#41467=AXIS2_PLACEMENT_3D('',#63204,#49315,#49316);
#41468=AXIS2_PLACEMENT_3D('',#63206,#49318,#49319);
#41469=AXIS2_PLACEMENT_3D('',#63208,#49321,#49322);
#41470=AXIS2_PLACEMENT_3D('',#63210,#49324,#49325);
#41471=AXIS2_PLACEMENT_3D('',#63212,#49327,#49328);
#41472=AXIS2_PLACEMENT_3D('',#63213,#49329,#49330);
#41473=AXIS2_PLACEMENT_3D('',#63216,#49333,#49334);
#41474=AXIS2_PLACEMENT_3D('',#63218,#49336,#49337);
#41475=AXIS2_PLACEMENT_3D('',#63220,#49339,#49340);
#41476=AXIS2_PLACEMENT_3D('',#63222,#49342,#49343);
#41477=AXIS2_PLACEMENT_3D('',#63224,#49345,#49346);
#41478=AXIS2_PLACEMENT_3D('',#63225,#49347,#49348);
#41479=AXIS2_PLACEMENT_3D('',#63228,#49351,#49352);
#41480=AXIS2_PLACEMENT_3D('',#63230,#49354,#49355);
#41481=AXIS2_PLACEMENT_3D('',#63232,#49357,#49358);
#41482=AXIS2_PLACEMENT_3D('',#63234,#49360,#49361);
#41483=AXIS2_PLACEMENT_3D('',#63236,#49363,#49364);
#41484=AXIS2_PLACEMENT_3D('',#63237,#49365,#49366);
#41485=AXIS2_PLACEMENT_3D('',#63240,#49369,#49370);
#41486=AXIS2_PLACEMENT_3D('',#63242,#49372,#49373);
#41487=AXIS2_PLACEMENT_3D('',#63244,#49375,#49376);
#41488=AXIS2_PLACEMENT_3D('',#63246,#49378,#49379);
#41489=AXIS2_PLACEMENT_3D('',#63248,#49381,#49382);
#41490=AXIS2_PLACEMENT_3D('',#63249,#49383,#49384);
#41491=AXIS2_PLACEMENT_3D('',#63252,#49387,#49388);
#41492=AXIS2_PLACEMENT_3D('',#63254,#49390,#49391);
#41493=AXIS2_PLACEMENT_3D('',#63256,#49393,#49394);
#41494=AXIS2_PLACEMENT_3D('',#63258,#49396,#49397);
#41495=AXIS2_PLACEMENT_3D('',#63260,#49399,#49400);
#41496=AXIS2_PLACEMENT_3D('',#63261,#49401,#49402);
#41497=AXIS2_PLACEMENT_3D('',#63264,#49405,#49406);
#41498=AXIS2_PLACEMENT_3D('',#63266,#49408,#49409);
#41499=AXIS2_PLACEMENT_3D('',#63268,#49411,#49412);
#41500=AXIS2_PLACEMENT_3D('',#63270,#49414,#49415);
#41501=AXIS2_PLACEMENT_3D('',#63272,#49417,#49418);
#41502=AXIS2_PLACEMENT_3D('',#63273,#49419,#49420);
#41503=AXIS2_PLACEMENT_3D('',#63276,#49423,#49424);
#41504=AXIS2_PLACEMENT_3D('',#63278,#49426,#49427);
#41505=AXIS2_PLACEMENT_3D('',#63280,#49429,#49430);
#41506=AXIS2_PLACEMENT_3D('',#63282,#49432,#49433);
#41507=AXIS2_PLACEMENT_3D('',#63284,#49435,#49436);
#41508=AXIS2_PLACEMENT_3D('',#63285,#49437,#49438);
#41509=AXIS2_PLACEMENT_3D('',#63288,#49441,#49442);
#41510=AXIS2_PLACEMENT_3D('',#63290,#49444,#49445);
#41511=AXIS2_PLACEMENT_3D('',#63292,#49447,#49448);
#41512=AXIS2_PLACEMENT_3D('',#63294,#49450,#49451);
#41513=AXIS2_PLACEMENT_3D('',#63296,#49453,#49454);
#41514=AXIS2_PLACEMENT_3D('',#63297,#49455,#49456);
#41515=AXIS2_PLACEMENT_3D('',#63300,#49459,#49460);
#41516=AXIS2_PLACEMENT_3D('',#63302,#49462,#49463);
#41517=AXIS2_PLACEMENT_3D('',#63304,#49465,#49466);
#41518=AXIS2_PLACEMENT_3D('',#63306,#49468,#49469);
#41519=AXIS2_PLACEMENT_3D('',#63308,#49471,#49472);
#41520=AXIS2_PLACEMENT_3D('',#63309,#49473,#49474);
#41521=AXIS2_PLACEMENT_3D('',#63312,#49477,#49478);
#41522=AXIS2_PLACEMENT_3D('',#63314,#49480,#49481);
#41523=AXIS2_PLACEMENT_3D('',#63316,#49483,#49484);
#41524=AXIS2_PLACEMENT_3D('',#63318,#49486,#49487);
#41525=AXIS2_PLACEMENT_3D('',#63320,#49489,#49490);
#41526=AXIS2_PLACEMENT_3D('',#63321,#49491,#49492);
#41527=AXIS2_PLACEMENT_3D('',#63324,#49495,#49496);
#41528=AXIS2_PLACEMENT_3D('',#63326,#49498,#49499);
#41529=AXIS2_PLACEMENT_3D('',#63328,#49501,#49502);
#41530=AXIS2_PLACEMENT_3D('',#63330,#49504,#49505);
#41531=AXIS2_PLACEMENT_3D('',#63332,#49507,#49508);
#41532=AXIS2_PLACEMENT_3D('',#63333,#49509,#49510);
#41533=AXIS2_PLACEMENT_3D('',#63336,#49513,#49514);
#41534=AXIS2_PLACEMENT_3D('',#63338,#49516,#49517);
#41535=AXIS2_PLACEMENT_3D('',#63340,#49519,#49520);
#41536=AXIS2_PLACEMENT_3D('',#63342,#49522,#49523);
#41537=AXIS2_PLACEMENT_3D('',#63344,#49525,#49526);
#41538=AXIS2_PLACEMENT_3D('',#63345,#49527,#49528);
#41539=AXIS2_PLACEMENT_3D('',#63348,#49531,#49532);
#41540=AXIS2_PLACEMENT_3D('',#63350,#49534,#49535);
#41541=AXIS2_PLACEMENT_3D('',#63352,#49537,#49538);
#41542=AXIS2_PLACEMENT_3D('',#63354,#49540,#49541);
#41543=AXIS2_PLACEMENT_3D('',#63356,#49543,#49544);
#41544=AXIS2_PLACEMENT_3D('',#63357,#49545,#49546);
#41545=AXIS2_PLACEMENT_3D('',#63360,#49549,#49550);
#41546=AXIS2_PLACEMENT_3D('',#63362,#49552,#49553);
#41547=AXIS2_PLACEMENT_3D('',#63364,#49555,#49556);
#41548=AXIS2_PLACEMENT_3D('',#63366,#49558,#49559);
#41549=AXIS2_PLACEMENT_3D('',#63368,#49561,#49562);
#41550=AXIS2_PLACEMENT_3D('',#63369,#49563,#49564);
#41551=AXIS2_PLACEMENT_3D('',#63372,#49567,#49568);
#41552=AXIS2_PLACEMENT_3D('',#63374,#49570,#49571);
#41553=AXIS2_PLACEMENT_3D('',#63376,#49573,#49574);
#41554=AXIS2_PLACEMENT_3D('',#63378,#49576,#49577);
#41555=AXIS2_PLACEMENT_3D('',#63380,#49579,#49580);
#41556=AXIS2_PLACEMENT_3D('',#63381,#49581,#49582);
#41557=AXIS2_PLACEMENT_3D('',#63384,#49585,#49586);
#41558=AXIS2_PLACEMENT_3D('',#63386,#49588,#49589);
#41559=AXIS2_PLACEMENT_3D('',#63388,#49591,#49592);
#41560=AXIS2_PLACEMENT_3D('',#63390,#49594,#49595);
#41561=AXIS2_PLACEMENT_3D('',#63392,#49597,#49598);
#41562=AXIS2_PLACEMENT_3D('',#63393,#49599,#49600);
#41563=AXIS2_PLACEMENT_3D('',#63396,#49603,#49604);
#41564=AXIS2_PLACEMENT_3D('',#63398,#49606,#49607);
#41565=AXIS2_PLACEMENT_3D('',#63400,#49609,#49610);
#41566=AXIS2_PLACEMENT_3D('',#63402,#49612,#49613);
#41567=AXIS2_PLACEMENT_3D('',#63404,#49615,#49616);
#41568=AXIS2_PLACEMENT_3D('',#63405,#49617,#49618);
#41569=AXIS2_PLACEMENT_3D('',#63408,#49621,#49622);
#41570=AXIS2_PLACEMENT_3D('',#63410,#49624,#49625);
#41571=AXIS2_PLACEMENT_3D('',#63412,#49627,#49628);
#41572=AXIS2_PLACEMENT_3D('',#63414,#49630,#49631);
#41573=AXIS2_PLACEMENT_3D('',#63416,#49633,#49634);
#41574=AXIS2_PLACEMENT_3D('',#63417,#49635,#49636);
#41575=AXIS2_PLACEMENT_3D('',#63420,#49639,#49640);
#41576=AXIS2_PLACEMENT_3D('',#63422,#49642,#49643);
#41577=AXIS2_PLACEMENT_3D('',#63424,#49645,#49646);
#41578=AXIS2_PLACEMENT_3D('',#63426,#49648,#49649);
#41579=AXIS2_PLACEMENT_3D('',#63428,#49651,#49652);
#41580=AXIS2_PLACEMENT_3D('',#63429,#49653,#49654);
#41581=AXIS2_PLACEMENT_3D('',#63432,#49657,#49658);
#41582=AXIS2_PLACEMENT_3D('',#63434,#49660,#49661);
#41583=AXIS2_PLACEMENT_3D('',#63436,#49663,#49664);
#41584=AXIS2_PLACEMENT_3D('',#63438,#49666,#49667);
#41585=AXIS2_PLACEMENT_3D('',#63440,#49669,#49670);
#41586=AXIS2_PLACEMENT_3D('',#63441,#49671,#49672);
#41587=AXIS2_PLACEMENT_3D('',#63444,#49675,#49676);
#41588=AXIS2_PLACEMENT_3D('',#63446,#49678,#49679);
#41589=AXIS2_PLACEMENT_3D('',#63448,#49681,#49682);
#41590=AXIS2_PLACEMENT_3D('',#63450,#49684,#49685);
#41591=AXIS2_PLACEMENT_3D('',#63452,#49687,#49688);
#41592=AXIS2_PLACEMENT_3D('',#63453,#49689,#49690);
#41593=AXIS2_PLACEMENT_3D('',#63456,#49693,#49694);
#41594=AXIS2_PLACEMENT_3D('',#63458,#49696,#49697);
#41595=AXIS2_PLACEMENT_3D('',#63460,#49699,#49700);
#41596=AXIS2_PLACEMENT_3D('',#63462,#49702,#49703);
#41597=AXIS2_PLACEMENT_3D('',#63464,#49705,#49706);
#41598=AXIS2_PLACEMENT_3D('',#63465,#49707,#49708);
#41599=AXIS2_PLACEMENT_3D('',#63468,#49711,#49712);
#41600=AXIS2_PLACEMENT_3D('',#63470,#49714,#49715);
#41601=AXIS2_PLACEMENT_3D('',#63472,#49717,#49718);
#41602=AXIS2_PLACEMENT_3D('',#63474,#49720,#49721);
#41603=AXIS2_PLACEMENT_3D('',#63476,#49723,#49724);
#41604=AXIS2_PLACEMENT_3D('',#63477,#49725,#49726);
#41605=AXIS2_PLACEMENT_3D('',#63480,#49729,#49730);
#41606=AXIS2_PLACEMENT_3D('',#63482,#49732,#49733);
#41607=AXIS2_PLACEMENT_3D('',#63484,#49735,#49736);
#41608=AXIS2_PLACEMENT_3D('',#63486,#49738,#49739);
#41609=AXIS2_PLACEMENT_3D('',#63488,#49741,#49742);
#41610=AXIS2_PLACEMENT_3D('',#63489,#49743,#49744);
#41611=AXIS2_PLACEMENT_3D('',#63492,#49747,#49748);
#41612=AXIS2_PLACEMENT_3D('',#63494,#49750,#49751);
#41613=AXIS2_PLACEMENT_3D('',#63496,#49753,#49754);
#41614=AXIS2_PLACEMENT_3D('',#63498,#49756,#49757);
#41615=AXIS2_PLACEMENT_3D('',#63500,#49759,#49760);
#41616=AXIS2_PLACEMENT_3D('',#63501,#49761,#49762);
#41617=AXIS2_PLACEMENT_3D('',#63504,#49765,#49766);
#41618=AXIS2_PLACEMENT_3D('',#63506,#49768,#49769);
#41619=AXIS2_PLACEMENT_3D('',#63508,#49771,#49772);
#41620=AXIS2_PLACEMENT_3D('',#63510,#49774,#49775);
#41621=AXIS2_PLACEMENT_3D('',#63512,#49777,#49778);
#41622=AXIS2_PLACEMENT_3D('',#63513,#49779,#49780);
#41623=AXIS2_PLACEMENT_3D('',#63516,#49783,#49784);
#41624=AXIS2_PLACEMENT_3D('',#63518,#49786,#49787);
#41625=AXIS2_PLACEMENT_3D('',#63520,#49789,#49790);
#41626=AXIS2_PLACEMENT_3D('',#63522,#49792,#49793);
#41627=AXIS2_PLACEMENT_3D('',#63524,#49795,#49796);
#41628=AXIS2_PLACEMENT_3D('',#63525,#49797,#49798);
#41629=AXIS2_PLACEMENT_3D('',#63528,#49801,#49802);
#41630=AXIS2_PLACEMENT_3D('',#63530,#49804,#49805);
#41631=AXIS2_PLACEMENT_3D('',#63532,#49807,#49808);
#41632=AXIS2_PLACEMENT_3D('',#63534,#49810,#49811);
#41633=AXIS2_PLACEMENT_3D('',#63536,#49813,#49814);
#41634=AXIS2_PLACEMENT_3D('',#63537,#49815,#49816);
#41635=AXIS2_PLACEMENT_3D('',#63540,#49819,#49820);
#41636=AXIS2_PLACEMENT_3D('',#63542,#49822,#49823);
#41637=AXIS2_PLACEMENT_3D('',#63544,#49825,#49826);
#41638=AXIS2_PLACEMENT_3D('',#63546,#49828,#49829);
#41639=AXIS2_PLACEMENT_3D('',#63548,#49831,#49832);
#41640=AXIS2_PLACEMENT_3D('',#63549,#49833,#49834);
#41641=AXIS2_PLACEMENT_3D('',#63552,#49837,#49838);
#41642=AXIS2_PLACEMENT_3D('',#63554,#49840,#49841);
#41643=AXIS2_PLACEMENT_3D('',#63556,#49843,#49844);
#41644=AXIS2_PLACEMENT_3D('',#63558,#49846,#49847);
#41645=AXIS2_PLACEMENT_3D('',#63560,#49849,#49850);
#41646=AXIS2_PLACEMENT_3D('',#63561,#49851,#49852);
#41647=AXIS2_PLACEMENT_3D('',#63564,#49855,#49856);
#41648=AXIS2_PLACEMENT_3D('',#63566,#49858,#49859);
#41649=AXIS2_PLACEMENT_3D('',#63568,#49861,#49862);
#41650=AXIS2_PLACEMENT_3D('',#63570,#49864,#49865);
#41651=AXIS2_PLACEMENT_3D('',#63572,#49867,#49868);
#41652=AXIS2_PLACEMENT_3D('',#63573,#49869,#49870);
#41653=AXIS2_PLACEMENT_3D('',#63576,#49873,#49874);
#41654=AXIS2_PLACEMENT_3D('',#63578,#49876,#49877);
#41655=AXIS2_PLACEMENT_3D('',#63580,#49879,#49880);
#41656=AXIS2_PLACEMENT_3D('',#63582,#49882,#49883);
#41657=AXIS2_PLACEMENT_3D('',#63584,#49885,#49886);
#41658=AXIS2_PLACEMENT_3D('',#63585,#49887,#49888);
#41659=AXIS2_PLACEMENT_3D('',#63588,#49891,#49892);
#41660=AXIS2_PLACEMENT_3D('',#63590,#49894,#49895);
#41661=AXIS2_PLACEMENT_3D('',#63592,#49897,#49898);
#41662=AXIS2_PLACEMENT_3D('',#63594,#49900,#49901);
#41663=AXIS2_PLACEMENT_3D('',#63596,#49903,#49904);
#41664=AXIS2_PLACEMENT_3D('',#63597,#49905,#49906);
#41665=AXIS2_PLACEMENT_3D('',#63600,#49909,#49910);
#41666=AXIS2_PLACEMENT_3D('',#63602,#49912,#49913);
#41667=AXIS2_PLACEMENT_3D('',#63604,#49915,#49916);
#41668=AXIS2_PLACEMENT_3D('',#63606,#49918,#49919);
#41669=AXIS2_PLACEMENT_3D('',#63608,#49921,#49922);
#41670=AXIS2_PLACEMENT_3D('',#63609,#49923,#49924);
#41671=AXIS2_PLACEMENT_3D('',#63612,#49927,#49928);
#41672=AXIS2_PLACEMENT_3D('',#63614,#49930,#49931);
#41673=AXIS2_PLACEMENT_3D('',#63616,#49933,#49934);
#41674=AXIS2_PLACEMENT_3D('',#63618,#49936,#49937);
#41675=AXIS2_PLACEMENT_3D('',#63620,#49939,#49940);
#41676=AXIS2_PLACEMENT_3D('',#63621,#49941,#49942);
#41677=AXIS2_PLACEMENT_3D('',#63624,#49945,#49946);
#41678=AXIS2_PLACEMENT_3D('',#63626,#49948,#49949);
#41679=AXIS2_PLACEMENT_3D('',#63628,#49951,#49952);
#41680=AXIS2_PLACEMENT_3D('',#63630,#49954,#49955);
#41681=AXIS2_PLACEMENT_3D('',#63632,#49957,#49958);
#41682=AXIS2_PLACEMENT_3D('',#63633,#49959,#49960);
#41683=AXIS2_PLACEMENT_3D('',#63636,#49963,#49964);
#41684=AXIS2_PLACEMENT_3D('',#63638,#49966,#49967);
#41685=AXIS2_PLACEMENT_3D('',#63640,#49969,#49970);
#41686=AXIS2_PLACEMENT_3D('',#63642,#49972,#49973);
#41687=AXIS2_PLACEMENT_3D('',#63644,#49975,#49976);
#41688=AXIS2_PLACEMENT_3D('',#63645,#49977,#49978);
#41689=AXIS2_PLACEMENT_3D('',#63648,#49981,#49982);
#41690=AXIS2_PLACEMENT_3D('',#63650,#49984,#49985);
#41691=AXIS2_PLACEMENT_3D('',#63652,#49987,#49988);
#41692=AXIS2_PLACEMENT_3D('',#63654,#49990,#49991);
#41693=AXIS2_PLACEMENT_3D('',#63656,#49993,#49994);
#41694=AXIS2_PLACEMENT_3D('',#63657,#49995,#49996);
#41695=AXIS2_PLACEMENT_3D('',#63660,#49999,#50000);
#41696=AXIS2_PLACEMENT_3D('',#63662,#50002,#50003);
#41697=AXIS2_PLACEMENT_3D('',#63664,#50005,#50006);
#41698=AXIS2_PLACEMENT_3D('',#63666,#50008,#50009);
#41699=AXIS2_PLACEMENT_3D('',#63668,#50011,#50012);
#41700=AXIS2_PLACEMENT_3D('',#63669,#50013,#50014);
#41701=AXIS2_PLACEMENT_3D('',#63672,#50017,#50018);
#41702=AXIS2_PLACEMENT_3D('',#63674,#50020,#50021);
#41703=AXIS2_PLACEMENT_3D('',#63676,#50023,#50024);
#41704=AXIS2_PLACEMENT_3D('',#63678,#50026,#50027);
#41705=AXIS2_PLACEMENT_3D('',#63680,#50029,#50030);
#41706=AXIS2_PLACEMENT_3D('',#63681,#50031,#50032);
#41707=AXIS2_PLACEMENT_3D('',#63684,#50035,#50036);
#41708=AXIS2_PLACEMENT_3D('',#63686,#50038,#50039);
#41709=AXIS2_PLACEMENT_3D('',#63688,#50041,#50042);
#41710=AXIS2_PLACEMENT_3D('',#63690,#50044,#50045);
#41711=AXIS2_PLACEMENT_3D('',#63692,#50047,#50048);
#41712=AXIS2_PLACEMENT_3D('',#63693,#50049,#50050);
#41713=AXIS2_PLACEMENT_3D('',#63696,#50053,#50054);
#41714=AXIS2_PLACEMENT_3D('',#63698,#50056,#50057);
#41715=AXIS2_PLACEMENT_3D('',#63700,#50059,#50060);
#41716=AXIS2_PLACEMENT_3D('',#63702,#50062,#50063);
#41717=AXIS2_PLACEMENT_3D('',#63704,#50065,#50066);
#41718=AXIS2_PLACEMENT_3D('',#63705,#50067,#50068);
#41719=AXIS2_PLACEMENT_3D('',#63708,#50071,#50072);
#41720=AXIS2_PLACEMENT_3D('',#63710,#50074,#50075);
#41721=AXIS2_PLACEMENT_3D('',#63712,#50077,#50078);
#41722=AXIS2_PLACEMENT_3D('',#63714,#50080,#50081);
#41723=AXIS2_PLACEMENT_3D('',#63716,#50083,#50084);
#41724=AXIS2_PLACEMENT_3D('',#63717,#50085,#50086);
#41725=AXIS2_PLACEMENT_3D('',#63720,#50089,#50090);
#41726=AXIS2_PLACEMENT_3D('',#63722,#50092,#50093);
#41727=AXIS2_PLACEMENT_3D('',#63724,#50095,#50096);
#41728=AXIS2_PLACEMENT_3D('',#63726,#50098,#50099);
#41729=AXIS2_PLACEMENT_3D('',#63728,#50101,#50102);
#41730=AXIS2_PLACEMENT_3D('',#63729,#50103,#50104);
#41731=AXIS2_PLACEMENT_3D('',#63732,#50107,#50108);
#41732=AXIS2_PLACEMENT_3D('',#63734,#50110,#50111);
#41733=AXIS2_PLACEMENT_3D('',#63736,#50113,#50114);
#41734=AXIS2_PLACEMENT_3D('',#63738,#50116,#50117);
#41735=AXIS2_PLACEMENT_3D('',#63740,#50119,#50120);
#41736=AXIS2_PLACEMENT_3D('',#63741,#50121,#50122);
#41737=AXIS2_PLACEMENT_3D('',#63744,#50125,#50126);
#41738=AXIS2_PLACEMENT_3D('',#63746,#50128,#50129);
#41739=AXIS2_PLACEMENT_3D('',#63748,#50131,#50132);
#41740=AXIS2_PLACEMENT_3D('',#63750,#50134,#50135);
#41741=AXIS2_PLACEMENT_3D('',#63752,#50137,#50138);
#41742=AXIS2_PLACEMENT_3D('',#63753,#50139,#50140);
#41743=AXIS2_PLACEMENT_3D('',#63756,#50143,#50144);
#41744=AXIS2_PLACEMENT_3D('',#63758,#50146,#50147);
#41745=AXIS2_PLACEMENT_3D('',#63760,#50149,#50150);
#41746=AXIS2_PLACEMENT_3D('',#63762,#50152,#50153);
#41747=AXIS2_PLACEMENT_3D('',#63764,#50155,#50156);
#41748=AXIS2_PLACEMENT_3D('',#63765,#50157,#50158);
#41749=AXIS2_PLACEMENT_3D('',#63768,#50161,#50162);
#41750=AXIS2_PLACEMENT_3D('',#63770,#50164,#50165);
#41751=AXIS2_PLACEMENT_3D('',#63772,#50167,#50168);
#41752=AXIS2_PLACEMENT_3D('',#63774,#50170,#50171);
#41753=AXIS2_PLACEMENT_3D('',#63776,#50173,#50174);
#41754=AXIS2_PLACEMENT_3D('',#63777,#50175,#50176);
#41755=AXIS2_PLACEMENT_3D('',#63780,#50179,#50180);
#41756=AXIS2_PLACEMENT_3D('',#63782,#50182,#50183);
#41757=AXIS2_PLACEMENT_3D('',#63784,#50185,#50186);
#41758=AXIS2_PLACEMENT_3D('',#63786,#50188,#50189);
#41759=AXIS2_PLACEMENT_3D('',#63788,#50191,#50192);
#41760=AXIS2_PLACEMENT_3D('',#63789,#50193,#50194);
#41761=AXIS2_PLACEMENT_3D('',#63792,#50197,#50198);
#41762=AXIS2_PLACEMENT_3D('',#63794,#50200,#50201);
#41763=AXIS2_PLACEMENT_3D('',#63796,#50203,#50204);
#41764=AXIS2_PLACEMENT_3D('',#63798,#50206,#50207);
#41765=AXIS2_PLACEMENT_3D('',#63800,#50209,#50210);
#41766=AXIS2_PLACEMENT_3D('',#63801,#50211,#50212);
#41767=AXIS2_PLACEMENT_3D('',#63804,#50215,#50216);
#41768=AXIS2_PLACEMENT_3D('',#63806,#50218,#50219);
#41769=AXIS2_PLACEMENT_3D('',#63808,#50221,#50222);
#41770=AXIS2_PLACEMENT_3D('',#63810,#50224,#50225);
#41771=AXIS2_PLACEMENT_3D('',#63812,#50227,#50228);
#41772=AXIS2_PLACEMENT_3D('',#63813,#50229,#50230);
#41773=AXIS2_PLACEMENT_3D('',#63816,#50233,#50234);
#41774=AXIS2_PLACEMENT_3D('',#63818,#50236,#50237);
#41775=AXIS2_PLACEMENT_3D('',#63820,#50239,#50240);
#41776=AXIS2_PLACEMENT_3D('',#63822,#50242,#50243);
#41777=AXIS2_PLACEMENT_3D('',#63824,#50245,#50246);
#41778=AXIS2_PLACEMENT_3D('',#63825,#50247,#50248);
#41779=AXIS2_PLACEMENT_3D('',#63828,#50251,#50252);
#41780=AXIS2_PLACEMENT_3D('',#63830,#50254,#50255);
#41781=AXIS2_PLACEMENT_3D('',#63832,#50257,#50258);
#41782=AXIS2_PLACEMENT_3D('',#63834,#50260,#50261);
#41783=AXIS2_PLACEMENT_3D('',#63836,#50263,#50264);
#41784=AXIS2_PLACEMENT_3D('',#63837,#50265,#50266);
#41785=AXIS2_PLACEMENT_3D('',#63840,#50269,#50270);
#41786=AXIS2_PLACEMENT_3D('',#63842,#50272,#50273);
#41787=AXIS2_PLACEMENT_3D('',#63844,#50275,#50276);
#41788=AXIS2_PLACEMENT_3D('',#63846,#50278,#50279);
#41789=AXIS2_PLACEMENT_3D('',#63848,#50281,#50282);
#41790=AXIS2_PLACEMENT_3D('',#63849,#50283,#50284);
#41791=AXIS2_PLACEMENT_3D('',#63852,#50287,#50288);
#41792=AXIS2_PLACEMENT_3D('',#63854,#50290,#50291);
#41793=AXIS2_PLACEMENT_3D('',#63856,#50293,#50294);
#41794=AXIS2_PLACEMENT_3D('',#63858,#50296,#50297);
#41795=AXIS2_PLACEMENT_3D('',#63860,#50299,#50300);
#41796=AXIS2_PLACEMENT_3D('',#63861,#50301,#50302);
#41797=AXIS2_PLACEMENT_3D('',#63864,#50305,#50306);
#41798=AXIS2_PLACEMENT_3D('',#63866,#50308,#50309);
#41799=AXIS2_PLACEMENT_3D('',#63868,#50311,#50312);
#41800=AXIS2_PLACEMENT_3D('',#63870,#50314,#50315);
#41801=AXIS2_PLACEMENT_3D('',#63872,#50317,#50318);
#41802=AXIS2_PLACEMENT_3D('',#63873,#50319,#50320);
#41803=AXIS2_PLACEMENT_3D('',#63876,#50323,#50324);
#41804=AXIS2_PLACEMENT_3D('',#63878,#50326,#50327);
#41805=AXIS2_PLACEMENT_3D('',#63880,#50329,#50330);
#41806=AXIS2_PLACEMENT_3D('',#63882,#50332,#50333);
#41807=AXIS2_PLACEMENT_3D('',#63884,#50335,#50336);
#41808=AXIS2_PLACEMENT_3D('',#63885,#50337,#50338);
#41809=AXIS2_PLACEMENT_3D('',#63888,#50341,#50342);
#41810=AXIS2_PLACEMENT_3D('',#63890,#50344,#50345);
#41811=AXIS2_PLACEMENT_3D('',#63892,#50347,#50348);
#41812=AXIS2_PLACEMENT_3D('',#63894,#50350,#50351);
#41813=AXIS2_PLACEMENT_3D('',#63896,#50353,#50354);
#41814=AXIS2_PLACEMENT_3D('',#63897,#50355,#50356);
#41815=AXIS2_PLACEMENT_3D('',#63900,#50359,#50360);
#41816=AXIS2_PLACEMENT_3D('',#63902,#50362,#50363);
#41817=AXIS2_PLACEMENT_3D('',#63904,#50365,#50366);
#41818=AXIS2_PLACEMENT_3D('',#63906,#50368,#50369);
#41819=AXIS2_PLACEMENT_3D('',#63908,#50371,#50372);
#41820=AXIS2_PLACEMENT_3D('',#63909,#50373,#50374);
#41821=AXIS2_PLACEMENT_3D('',#63912,#50377,#50378);
#41822=AXIS2_PLACEMENT_3D('',#63914,#50380,#50381);
#41823=AXIS2_PLACEMENT_3D('',#63916,#50383,#50384);
#41824=AXIS2_PLACEMENT_3D('',#63918,#50386,#50387);
#41825=AXIS2_PLACEMENT_3D('',#63920,#50389,#50390);
#41826=AXIS2_PLACEMENT_3D('',#63921,#50391,#50392);
#41827=AXIS2_PLACEMENT_3D('',#63924,#50395,#50396);
#41828=AXIS2_PLACEMENT_3D('',#63926,#50398,#50399);
#41829=AXIS2_PLACEMENT_3D('',#63928,#50401,#50402);
#41830=AXIS2_PLACEMENT_3D('',#63930,#50404,#50405);
#41831=AXIS2_PLACEMENT_3D('',#63932,#50407,#50408);
#41832=AXIS2_PLACEMENT_3D('',#63933,#50409,#50410);
#41833=AXIS2_PLACEMENT_3D('',#63936,#50413,#50414);
#41834=AXIS2_PLACEMENT_3D('',#63938,#50416,#50417);
#41835=AXIS2_PLACEMENT_3D('',#63940,#50419,#50420);
#41836=AXIS2_PLACEMENT_3D('',#63942,#50422,#50423);
#41837=AXIS2_PLACEMENT_3D('',#63944,#50425,#50426);
#41838=AXIS2_PLACEMENT_3D('',#63945,#50427,#50428);
#41839=AXIS2_PLACEMENT_3D('',#63948,#50431,#50432);
#41840=AXIS2_PLACEMENT_3D('',#63950,#50434,#50435);
#41841=AXIS2_PLACEMENT_3D('',#63952,#50437,#50438);
#41842=AXIS2_PLACEMENT_3D('',#63954,#50440,#50441);
#41843=AXIS2_PLACEMENT_3D('',#63956,#50443,#50444);
#41844=AXIS2_PLACEMENT_3D('',#63957,#50445,#50446);
#41845=AXIS2_PLACEMENT_3D('',#63960,#50449,#50450);
#41846=AXIS2_PLACEMENT_3D('',#63962,#50452,#50453);
#41847=AXIS2_PLACEMENT_3D('',#63964,#50455,#50456);
#41848=AXIS2_PLACEMENT_3D('',#63966,#50458,#50459);
#41849=AXIS2_PLACEMENT_3D('',#63968,#50461,#50462);
#41850=AXIS2_PLACEMENT_3D('',#63969,#50463,#50464);
#41851=AXIS2_PLACEMENT_3D('',#63972,#50467,#50468);
#41852=AXIS2_PLACEMENT_3D('',#63974,#50470,#50471);
#41853=AXIS2_PLACEMENT_3D('',#63976,#50473,#50474);
#41854=AXIS2_PLACEMENT_3D('',#63978,#50476,#50477);
#41855=AXIS2_PLACEMENT_3D('',#63980,#50479,#50480);
#41856=AXIS2_PLACEMENT_3D('',#63981,#50481,#50482);
#41857=AXIS2_PLACEMENT_3D('',#63984,#50485,#50486);
#41858=AXIS2_PLACEMENT_3D('',#63986,#50488,#50489);
#41859=AXIS2_PLACEMENT_3D('',#63988,#50491,#50492);
#41860=AXIS2_PLACEMENT_3D('',#63990,#50494,#50495);
#41861=AXIS2_PLACEMENT_3D('',#63992,#50497,#50498);
#41862=AXIS2_PLACEMENT_3D('',#63993,#50499,#50500);
#41863=AXIS2_PLACEMENT_3D('',#63996,#50503,#50504);
#41864=AXIS2_PLACEMENT_3D('',#63998,#50506,#50507);
#41865=AXIS2_PLACEMENT_3D('',#64000,#50509,#50510);
#41866=AXIS2_PLACEMENT_3D('',#64002,#50512,#50513);
#41867=AXIS2_PLACEMENT_3D('',#64004,#50515,#50516);
#41868=AXIS2_PLACEMENT_3D('',#64005,#50517,#50518);
#41869=AXIS2_PLACEMENT_3D('',#64008,#50521,#50522);
#41870=AXIS2_PLACEMENT_3D('',#64010,#50524,#50525);
#41871=AXIS2_PLACEMENT_3D('',#64012,#50527,#50528);
#41872=AXIS2_PLACEMENT_3D('',#64014,#50530,#50531);
#41873=AXIS2_PLACEMENT_3D('',#64016,#50533,#50534);
#41874=AXIS2_PLACEMENT_3D('',#64017,#50535,#50536);
#41875=AXIS2_PLACEMENT_3D('',#64020,#50539,#50540);
#41876=AXIS2_PLACEMENT_3D('',#64022,#50542,#50543);
#41877=AXIS2_PLACEMENT_3D('',#64024,#50545,#50546);
#41878=AXIS2_PLACEMENT_3D('',#64026,#50548,#50549);
#41879=AXIS2_PLACEMENT_3D('',#64028,#50551,#50552);
#41880=AXIS2_PLACEMENT_3D('',#64029,#50553,#50554);
#41881=AXIS2_PLACEMENT_3D('',#64032,#50557,#50558);
#41882=AXIS2_PLACEMENT_3D('',#64034,#50560,#50561);
#41883=AXIS2_PLACEMENT_3D('',#64036,#50563,#50564);
#41884=AXIS2_PLACEMENT_3D('',#64038,#50566,#50567);
#41885=AXIS2_PLACEMENT_3D('',#64040,#50569,#50570);
#41886=AXIS2_PLACEMENT_3D('',#64041,#50571,#50572);
#41887=AXIS2_PLACEMENT_3D('',#64044,#50575,#50576);
#41888=AXIS2_PLACEMENT_3D('',#64046,#50578,#50579);
#41889=AXIS2_PLACEMENT_3D('',#64048,#50581,#50582);
#41890=AXIS2_PLACEMENT_3D('',#64050,#50584,#50585);
#41891=AXIS2_PLACEMENT_3D('',#64052,#50587,#50588);
#41892=AXIS2_PLACEMENT_3D('',#64053,#50589,#50590);
#41893=AXIS2_PLACEMENT_3D('',#64056,#50593,#50594);
#41894=AXIS2_PLACEMENT_3D('',#64058,#50596,#50597);
#41895=AXIS2_PLACEMENT_3D('',#64060,#50599,#50600);
#41896=AXIS2_PLACEMENT_3D('',#64062,#50602,#50603);
#41897=AXIS2_PLACEMENT_3D('',#64064,#50605,#50606);
#41898=AXIS2_PLACEMENT_3D('',#64065,#50607,#50608);
#41899=AXIS2_PLACEMENT_3D('',#64068,#50611,#50612);
#41900=AXIS2_PLACEMENT_3D('',#64070,#50614,#50615);
#41901=AXIS2_PLACEMENT_3D('',#64072,#50617,#50618);
#41902=AXIS2_PLACEMENT_3D('',#64074,#50620,#50621);
#41903=AXIS2_PLACEMENT_3D('',#64076,#50623,#50624);
#41904=AXIS2_PLACEMENT_3D('',#64077,#50625,#50626);
#41905=AXIS2_PLACEMENT_3D('',#64080,#50629,#50630);
#41906=AXIS2_PLACEMENT_3D('',#64082,#50632,#50633);
#41907=AXIS2_PLACEMENT_3D('',#64084,#50635,#50636);
#41908=AXIS2_PLACEMENT_3D('',#64086,#50638,#50639);
#41909=AXIS2_PLACEMENT_3D('',#64088,#50641,#50642);
#41910=AXIS2_PLACEMENT_3D('',#64089,#50643,#50644);
#41911=AXIS2_PLACEMENT_3D('',#64092,#50647,#50648);
#41912=AXIS2_PLACEMENT_3D('',#64094,#50650,#50651);
#41913=AXIS2_PLACEMENT_3D('',#64096,#50653,#50654);
#41914=AXIS2_PLACEMENT_3D('',#64098,#50656,#50657);
#41915=AXIS2_PLACEMENT_3D('',#64100,#50659,#50660);
#41916=AXIS2_PLACEMENT_3D('',#64101,#50661,#50662);
#41917=AXIS2_PLACEMENT_3D('',#64104,#50665,#50666);
#41918=AXIS2_PLACEMENT_3D('',#64106,#50668,#50669);
#41919=AXIS2_PLACEMENT_3D('',#64108,#50671,#50672);
#41920=AXIS2_PLACEMENT_3D('',#64110,#50674,#50675);
#41921=AXIS2_PLACEMENT_3D('',#64112,#50677,#50678);
#41922=AXIS2_PLACEMENT_3D('',#64113,#50679,#50680);
#41923=AXIS2_PLACEMENT_3D('',#64116,#50683,#50684);
#41924=AXIS2_PLACEMENT_3D('',#64118,#50686,#50687);
#41925=AXIS2_PLACEMENT_3D('',#64120,#50689,#50690);
#41926=AXIS2_PLACEMENT_3D('',#64122,#50692,#50693);
#41927=AXIS2_PLACEMENT_3D('',#64124,#50695,#50696);
#41928=AXIS2_PLACEMENT_3D('',#64125,#50697,#50698);
#41929=AXIS2_PLACEMENT_3D('',#64128,#50701,#50702);
#41930=AXIS2_PLACEMENT_3D('',#64130,#50704,#50705);
#41931=AXIS2_PLACEMENT_3D('',#64132,#50707,#50708);
#41932=AXIS2_PLACEMENT_3D('',#64134,#50710,#50711);
#41933=AXIS2_PLACEMENT_3D('',#64136,#50713,#50714);
#41934=AXIS2_PLACEMENT_3D('',#64137,#50715,#50716);
#41935=AXIS2_PLACEMENT_3D('',#64140,#50719,#50720);
#41936=AXIS2_PLACEMENT_3D('',#64142,#50722,#50723);
#41937=AXIS2_PLACEMENT_3D('',#64144,#50725,#50726);
#41938=AXIS2_PLACEMENT_3D('',#64146,#50728,#50729);
#41939=AXIS2_PLACEMENT_3D('',#64148,#50731,#50732);
#41940=AXIS2_PLACEMENT_3D('',#64149,#50733,#50734);
#41941=AXIS2_PLACEMENT_3D('',#64152,#50737,#50738);
#41942=AXIS2_PLACEMENT_3D('',#64154,#50740,#50741);
#41943=AXIS2_PLACEMENT_3D('',#64156,#50743,#50744);
#41944=AXIS2_PLACEMENT_3D('',#64158,#50746,#50747);
#41945=AXIS2_PLACEMENT_3D('',#64160,#50749,#50750);
#41946=AXIS2_PLACEMENT_3D('',#64161,#50751,#50752);
#41947=AXIS2_PLACEMENT_3D('',#64164,#50755,#50756);
#41948=AXIS2_PLACEMENT_3D('',#64166,#50758,#50759);
#41949=AXIS2_PLACEMENT_3D('',#64168,#50761,#50762);
#41950=AXIS2_PLACEMENT_3D('',#64170,#50764,#50765);
#41951=AXIS2_PLACEMENT_3D('',#64172,#50767,#50768);
#41952=AXIS2_PLACEMENT_3D('',#64173,#50769,#50770);
#41953=AXIS2_PLACEMENT_3D('',#64176,#50773,#50774);
#41954=AXIS2_PLACEMENT_3D('',#64178,#50776,#50777);
#41955=AXIS2_PLACEMENT_3D('',#64180,#50779,#50780);
#41956=AXIS2_PLACEMENT_3D('',#64182,#50782,#50783);
#41957=AXIS2_PLACEMENT_3D('',#64184,#50785,#50786);
#41958=AXIS2_PLACEMENT_3D('',#64185,#50787,#50788);
#41959=AXIS2_PLACEMENT_3D('',#64188,#50791,#50792);
#41960=AXIS2_PLACEMENT_3D('',#64190,#50794,#50795);
#41961=AXIS2_PLACEMENT_3D('',#64192,#50797,#50798);
#41962=AXIS2_PLACEMENT_3D('',#64194,#50800,#50801);
#41963=AXIS2_PLACEMENT_3D('',#64196,#50803,#50804);
#41964=AXIS2_PLACEMENT_3D('',#64197,#50805,#50806);
#41965=AXIS2_PLACEMENT_3D('',#64200,#50809,#50810);
#41966=AXIS2_PLACEMENT_3D('',#64202,#50812,#50813);
#41967=AXIS2_PLACEMENT_3D('',#64204,#50815,#50816);
#41968=AXIS2_PLACEMENT_3D('',#64206,#50818,#50819);
#41969=AXIS2_PLACEMENT_3D('',#64208,#50821,#50822);
#41970=AXIS2_PLACEMENT_3D('',#64209,#50823,#50824);
#41971=AXIS2_PLACEMENT_3D('',#64212,#50827,#50828);
#41972=AXIS2_PLACEMENT_3D('',#64214,#50830,#50831);
#41973=AXIS2_PLACEMENT_3D('',#64216,#50833,#50834);
#41974=AXIS2_PLACEMENT_3D('',#64218,#50836,#50837);
#41975=AXIS2_PLACEMENT_3D('',#64220,#50839,#50840);
#41976=AXIS2_PLACEMENT_3D('',#64221,#50841,#50842);
#41977=AXIS2_PLACEMENT_3D('',#64224,#50845,#50846);
#41978=AXIS2_PLACEMENT_3D('',#64226,#50848,#50849);
#41979=AXIS2_PLACEMENT_3D('',#64228,#50851,#50852);
#41980=AXIS2_PLACEMENT_3D('',#64230,#50854,#50855);
#41981=AXIS2_PLACEMENT_3D('',#64232,#50857,#50858);
#41982=AXIS2_PLACEMENT_3D('',#64233,#50859,#50860);
#41983=AXIS2_PLACEMENT_3D('',#64236,#50863,#50864);
#41984=AXIS2_PLACEMENT_3D('',#64238,#50866,#50867);
#41985=AXIS2_PLACEMENT_3D('',#64240,#50869,#50870);
#41986=AXIS2_PLACEMENT_3D('',#64242,#50872,#50873);
#41987=AXIS2_PLACEMENT_3D('',#64244,#50875,#50876);
#41988=AXIS2_PLACEMENT_3D('',#64245,#50877,#50878);
#41989=AXIS2_PLACEMENT_3D('',#64248,#50881,#50882);
#41990=AXIS2_PLACEMENT_3D('',#64250,#50884,#50885);
#41991=AXIS2_PLACEMENT_3D('',#64252,#50887,#50888);
#41992=AXIS2_PLACEMENT_3D('',#64254,#50890,#50891);
#41993=AXIS2_PLACEMENT_3D('',#64256,#50893,#50894);
#41994=AXIS2_PLACEMENT_3D('',#64257,#50895,#50896);
#41995=AXIS2_PLACEMENT_3D('',#64260,#50899,#50900);
#41996=AXIS2_PLACEMENT_3D('',#64262,#50902,#50903);
#41997=AXIS2_PLACEMENT_3D('',#64264,#50905,#50906);
#41998=AXIS2_PLACEMENT_3D('',#64266,#50908,#50909);
#41999=AXIS2_PLACEMENT_3D('',#64268,#50911,#50912);
#42000=AXIS2_PLACEMENT_3D('',#64269,#50913,#50914);
#42001=AXIS2_PLACEMENT_3D('',#64272,#50917,#50918);
#42002=AXIS2_PLACEMENT_3D('',#64274,#50920,#50921);
#42003=AXIS2_PLACEMENT_3D('',#64276,#50923,#50924);
#42004=AXIS2_PLACEMENT_3D('',#64278,#50926,#50927);
#42005=AXIS2_PLACEMENT_3D('',#64280,#50929,#50930);
#42006=AXIS2_PLACEMENT_3D('',#64281,#50931,#50932);
#42007=AXIS2_PLACEMENT_3D('',#64284,#50935,#50936);
#42008=AXIS2_PLACEMENT_3D('',#64286,#50938,#50939);
#42009=AXIS2_PLACEMENT_3D('',#64288,#50941,#50942);
#42010=AXIS2_PLACEMENT_3D('',#64290,#50944,#50945);
#42011=AXIS2_PLACEMENT_3D('',#64292,#50947,#50948);
#42012=AXIS2_PLACEMENT_3D('',#64293,#50949,#50950);
#42013=AXIS2_PLACEMENT_3D('',#64296,#50953,#50954);
#42014=AXIS2_PLACEMENT_3D('',#64298,#50956,#50957);
#42015=AXIS2_PLACEMENT_3D('',#64300,#50959,#50960);
#42016=AXIS2_PLACEMENT_3D('',#64302,#50962,#50963);
#42017=AXIS2_PLACEMENT_3D('',#64304,#50965,#50966);
#42018=AXIS2_PLACEMENT_3D('',#64305,#50967,#50968);
#42019=AXIS2_PLACEMENT_3D('',#64308,#50971,#50972);
#42020=AXIS2_PLACEMENT_3D('',#64310,#50974,#50975);
#42021=AXIS2_PLACEMENT_3D('',#64312,#50977,#50978);
#42022=AXIS2_PLACEMENT_3D('',#64314,#50980,#50981);
#42023=AXIS2_PLACEMENT_3D('',#64316,#50983,#50984);
#42024=AXIS2_PLACEMENT_3D('',#64317,#50985,#50986);
#42025=AXIS2_PLACEMENT_3D('',#64320,#50989,#50990);
#42026=AXIS2_PLACEMENT_3D('',#64322,#50992,#50993);
#42027=AXIS2_PLACEMENT_3D('',#64324,#50995,#50996);
#42028=AXIS2_PLACEMENT_3D('',#64326,#50998,#50999);
#42029=AXIS2_PLACEMENT_3D('',#64328,#51001,#51002);
#42030=AXIS2_PLACEMENT_3D('',#64329,#51003,#51004);
#42031=AXIS2_PLACEMENT_3D('',#64332,#51007,#51008);
#42032=AXIS2_PLACEMENT_3D('',#64334,#51010,#51011);
#42033=AXIS2_PLACEMENT_3D('',#64336,#51013,#51014);
#42034=AXIS2_PLACEMENT_3D('',#64338,#51016,#51017);
#42035=AXIS2_PLACEMENT_3D('',#64340,#51019,#51020);
#42036=AXIS2_PLACEMENT_3D('',#64341,#51021,#51022);
#42037=AXIS2_PLACEMENT_3D('',#64344,#51025,#51026);
#42038=AXIS2_PLACEMENT_3D('',#64346,#51028,#51029);
#42039=AXIS2_PLACEMENT_3D('',#64348,#51031,#51032);
#42040=AXIS2_PLACEMENT_3D('',#64350,#51034,#51035);
#42041=AXIS2_PLACEMENT_3D('',#64352,#51037,#51038);
#42042=AXIS2_PLACEMENT_3D('',#64353,#51039,#51040);
#42043=AXIS2_PLACEMENT_3D('',#64356,#51043,#51044);
#42044=AXIS2_PLACEMENT_3D('',#64358,#51046,#51047);
#42045=AXIS2_PLACEMENT_3D('',#64360,#51049,#51050);
#42046=AXIS2_PLACEMENT_3D('',#64362,#51052,#51053);
#42047=AXIS2_PLACEMENT_3D('',#64364,#51055,#51056);
#42048=AXIS2_PLACEMENT_3D('',#64365,#51057,#51058);
#42049=AXIS2_PLACEMENT_3D('',#64368,#51061,#51062);
#42050=AXIS2_PLACEMENT_3D('',#64370,#51064,#51065);
#42051=AXIS2_PLACEMENT_3D('',#64372,#51067,#51068);
#42052=AXIS2_PLACEMENT_3D('',#64374,#51070,#51071);
#42053=AXIS2_PLACEMENT_3D('',#64376,#51073,#51074);
#42054=AXIS2_PLACEMENT_3D('',#64377,#51075,#51076);
#42055=AXIS2_PLACEMENT_3D('',#64380,#51079,#51080);
#42056=AXIS2_PLACEMENT_3D('',#64382,#51082,#51083);
#42057=AXIS2_PLACEMENT_3D('',#64384,#51085,#51086);
#42058=AXIS2_PLACEMENT_3D('',#64386,#51088,#51089);
#42059=AXIS2_PLACEMENT_3D('',#64388,#51091,#51092);
#42060=AXIS2_PLACEMENT_3D('',#64389,#51093,#51094);
#42061=AXIS2_PLACEMENT_3D('',#64392,#51097,#51098);
#42062=AXIS2_PLACEMENT_3D('',#64394,#51100,#51101);
#42063=AXIS2_PLACEMENT_3D('',#64396,#51103,#51104);
#42064=AXIS2_PLACEMENT_3D('',#64398,#51106,#51107);
#42065=AXIS2_PLACEMENT_3D('',#64400,#51109,#51110);
#42066=AXIS2_PLACEMENT_3D('',#64401,#51111,#51112);
#42067=AXIS2_PLACEMENT_3D('',#64404,#51115,#51116);
#42068=AXIS2_PLACEMENT_3D('',#64406,#51118,#51119);
#42069=AXIS2_PLACEMENT_3D('',#64408,#51121,#51122);
#42070=AXIS2_PLACEMENT_3D('',#64410,#51124,#51125);
#42071=AXIS2_PLACEMENT_3D('',#64412,#51127,#51128);
#42072=AXIS2_PLACEMENT_3D('',#64413,#51129,#51130);
#42073=AXIS2_PLACEMENT_3D('',#64416,#51133,#51134);
#42074=AXIS2_PLACEMENT_3D('',#64418,#51136,#51137);
#42075=AXIS2_PLACEMENT_3D('',#64420,#51139,#51140);
#42076=AXIS2_PLACEMENT_3D('',#64422,#51142,#51143);
#42077=AXIS2_PLACEMENT_3D('',#64424,#51145,#51146);
#42078=AXIS2_PLACEMENT_3D('',#64425,#51147,#51148);
#42079=AXIS2_PLACEMENT_3D('',#64428,#51151,#51152);
#42080=AXIS2_PLACEMENT_3D('',#64430,#51154,#51155);
#42081=AXIS2_PLACEMENT_3D('',#64432,#51157,#51158);
#42082=AXIS2_PLACEMENT_3D('',#64434,#51160,#51161);
#42083=AXIS2_PLACEMENT_3D('',#64436,#51163,#51164);
#42084=AXIS2_PLACEMENT_3D('',#64437,#51165,#51166);
#42085=AXIS2_PLACEMENT_3D('',#64440,#51169,#51170);
#42086=AXIS2_PLACEMENT_3D('',#64442,#51172,#51173);
#42087=AXIS2_PLACEMENT_3D('',#64444,#51175,#51176);
#42088=AXIS2_PLACEMENT_3D('',#64446,#51178,#51179);
#42089=AXIS2_PLACEMENT_3D('',#64448,#51181,#51182);
#42090=AXIS2_PLACEMENT_3D('',#64449,#51183,#51184);
#42091=AXIS2_PLACEMENT_3D('',#64452,#51187,#51188);
#42092=AXIS2_PLACEMENT_3D('',#64454,#51190,#51191);
#42093=AXIS2_PLACEMENT_3D('',#64456,#51193,#51194);
#42094=AXIS2_PLACEMENT_3D('',#64458,#51196,#51197);
#42095=AXIS2_PLACEMENT_3D('',#64460,#51199,#51200);
#42096=AXIS2_PLACEMENT_3D('',#64461,#51201,#51202);
#42097=AXIS2_PLACEMENT_3D('',#64464,#51205,#51206);
#42098=AXIS2_PLACEMENT_3D('',#64466,#51208,#51209);
#42099=AXIS2_PLACEMENT_3D('',#64468,#51211,#51212);
#42100=AXIS2_PLACEMENT_3D('',#64470,#51214,#51215);
#42101=AXIS2_PLACEMENT_3D('',#64472,#51217,#51218);
#42102=AXIS2_PLACEMENT_3D('',#64473,#51219,#51220);
#42103=AXIS2_PLACEMENT_3D('',#64476,#51223,#51224);
#42104=AXIS2_PLACEMENT_3D('',#64478,#51226,#51227);
#42105=AXIS2_PLACEMENT_3D('',#64480,#51229,#51230);
#42106=AXIS2_PLACEMENT_3D('',#64482,#51232,#51233);
#42107=AXIS2_PLACEMENT_3D('',#64484,#51235,#51236);
#42108=AXIS2_PLACEMENT_3D('',#64485,#51237,#51238);
#42109=AXIS2_PLACEMENT_3D('',#64488,#51241,#51242);
#42110=AXIS2_PLACEMENT_3D('',#64490,#51244,#51245);
#42111=AXIS2_PLACEMENT_3D('',#64492,#51247,#51248);
#42112=AXIS2_PLACEMENT_3D('',#64494,#51250,#51251);
#42113=AXIS2_PLACEMENT_3D('',#64496,#51253,#51254);
#42114=AXIS2_PLACEMENT_3D('',#64497,#51255,#51256);
#42115=AXIS2_PLACEMENT_3D('',#64500,#51259,#51260);
#42116=AXIS2_PLACEMENT_3D('',#64502,#51262,#51263);
#42117=AXIS2_PLACEMENT_3D('',#64504,#51265,#51266);
#42118=AXIS2_PLACEMENT_3D('',#64506,#51268,#51269);
#42119=AXIS2_PLACEMENT_3D('',#64508,#51271,#51272);
#42120=AXIS2_PLACEMENT_3D('',#64509,#51273,#51274);
#42121=AXIS2_PLACEMENT_3D('',#64512,#51277,#51278);
#42122=AXIS2_PLACEMENT_3D('',#64514,#51280,#51281);
#42123=AXIS2_PLACEMENT_3D('',#64516,#51283,#51284);
#42124=AXIS2_PLACEMENT_3D('',#64518,#51286,#51287);
#42125=AXIS2_PLACEMENT_3D('',#64520,#51289,#51290);
#42126=AXIS2_PLACEMENT_3D('',#64521,#51291,#51292);
#42127=AXIS2_PLACEMENT_3D('',#64524,#51295,#51296);
#42128=AXIS2_PLACEMENT_3D('',#64526,#51298,#51299);
#42129=AXIS2_PLACEMENT_3D('',#64528,#51301,#51302);
#42130=AXIS2_PLACEMENT_3D('',#64530,#51304,#51305);
#42131=AXIS2_PLACEMENT_3D('',#64532,#51307,#51308);
#42132=AXIS2_PLACEMENT_3D('',#64533,#51309,#51310);
#42133=AXIS2_PLACEMENT_3D('',#64536,#51313,#51314);
#42134=AXIS2_PLACEMENT_3D('',#64538,#51316,#51317);
#42135=AXIS2_PLACEMENT_3D('',#64540,#51319,#51320);
#42136=AXIS2_PLACEMENT_3D('',#64542,#51322,#51323);
#42137=AXIS2_PLACEMENT_3D('',#64544,#51325,#51326);
#42138=AXIS2_PLACEMENT_3D('',#64545,#51327,#51328);
#42139=AXIS2_PLACEMENT_3D('',#64548,#51331,#51332);
#42140=AXIS2_PLACEMENT_3D('',#64550,#51334,#51335);
#42141=AXIS2_PLACEMENT_3D('',#64552,#51337,#51338);
#42142=AXIS2_PLACEMENT_3D('',#64554,#51340,#51341);
#42143=AXIS2_PLACEMENT_3D('',#64556,#51343,#51344);
#42144=AXIS2_PLACEMENT_3D('',#64557,#51345,#51346);
#42145=AXIS2_PLACEMENT_3D('',#64560,#51349,#51350);
#42146=AXIS2_PLACEMENT_3D('',#64562,#51352,#51353);
#42147=AXIS2_PLACEMENT_3D('',#64564,#51355,#51356);
#42148=AXIS2_PLACEMENT_3D('',#64566,#51358,#51359);
#42149=AXIS2_PLACEMENT_3D('',#64568,#51361,#51362);
#42150=AXIS2_PLACEMENT_3D('',#64569,#51363,#51364);
#42151=AXIS2_PLACEMENT_3D('',#64572,#51367,#51368);
#42152=AXIS2_PLACEMENT_3D('',#64574,#51370,#51371);
#42153=AXIS2_PLACEMENT_3D('',#64576,#51373,#51374);
#42154=AXIS2_PLACEMENT_3D('',#64578,#51376,#51377);
#42155=AXIS2_PLACEMENT_3D('',#64580,#51379,#51380);
#42156=AXIS2_PLACEMENT_3D('',#64581,#51381,#51382);
#42157=AXIS2_PLACEMENT_3D('',#64584,#51385,#51386);
#42158=AXIS2_PLACEMENT_3D('',#64586,#51388,#51389);
#42159=AXIS2_PLACEMENT_3D('',#64588,#51391,#51392);
#42160=AXIS2_PLACEMENT_3D('',#64590,#51394,#51395);
#42161=AXIS2_PLACEMENT_3D('',#64592,#51397,#51398);
#42162=AXIS2_PLACEMENT_3D('',#64593,#51399,#51400);
#42163=AXIS2_PLACEMENT_3D('',#64596,#51403,#51404);
#42164=AXIS2_PLACEMENT_3D('',#64598,#51406,#51407);
#42165=AXIS2_PLACEMENT_3D('',#64600,#51409,#51410);
#42166=AXIS2_PLACEMENT_3D('',#64602,#51412,#51413);
#42167=AXIS2_PLACEMENT_3D('',#64604,#51415,#51416);
#42168=AXIS2_PLACEMENT_3D('',#64605,#51417,#51418);
#42169=AXIS2_PLACEMENT_3D('',#64608,#51421,#51422);
#42170=AXIS2_PLACEMENT_3D('',#64610,#51424,#51425);
#42171=AXIS2_PLACEMENT_3D('',#64612,#51427,#51428);
#42172=AXIS2_PLACEMENT_3D('',#64614,#51430,#51431);
#42173=AXIS2_PLACEMENT_3D('',#64616,#51433,#51434);
#42174=AXIS2_PLACEMENT_3D('',#64617,#51435,#51436);
#42175=AXIS2_PLACEMENT_3D('',#64620,#51439,#51440);
#42176=AXIS2_PLACEMENT_3D('',#64622,#51442,#51443);
#42177=AXIS2_PLACEMENT_3D('',#64624,#51445,#51446);
#42178=AXIS2_PLACEMENT_3D('',#64626,#51448,#51449);
#42179=AXIS2_PLACEMENT_3D('',#64628,#51451,#51452);
#42180=AXIS2_PLACEMENT_3D('',#64629,#51453,#51454);
#42181=AXIS2_PLACEMENT_3D('',#64632,#51457,#51458);
#42182=AXIS2_PLACEMENT_3D('',#64634,#51460,#51461);
#42183=AXIS2_PLACEMENT_3D('',#64636,#51463,#51464);
#42184=AXIS2_PLACEMENT_3D('',#64638,#51466,#51467);
#42185=AXIS2_PLACEMENT_3D('',#64640,#51469,#51470);
#42186=AXIS2_PLACEMENT_3D('',#64641,#51471,#51472);
#42187=AXIS2_PLACEMENT_3D('',#64644,#51475,#51476);
#42188=AXIS2_PLACEMENT_3D('',#64646,#51478,#51479);
#42189=AXIS2_PLACEMENT_3D('',#64648,#51481,#51482);
#42190=AXIS2_PLACEMENT_3D('',#64650,#51484,#51485);
#42191=AXIS2_PLACEMENT_3D('',#64652,#51487,#51488);
#42192=AXIS2_PLACEMENT_3D('',#64653,#51489,#51490);
#42193=AXIS2_PLACEMENT_3D('',#64656,#51493,#51494);
#42194=AXIS2_PLACEMENT_3D('',#64658,#51496,#51497);
#42195=AXIS2_PLACEMENT_3D('',#64660,#51499,#51500);
#42196=AXIS2_PLACEMENT_3D('',#64662,#51502,#51503);
#42197=AXIS2_PLACEMENT_3D('',#64664,#51505,#51506);
#42198=AXIS2_PLACEMENT_3D('',#64665,#51507,#51508);
#42199=AXIS2_PLACEMENT_3D('',#64668,#51511,#51512);
#42200=AXIS2_PLACEMENT_3D('',#64670,#51514,#51515);
#42201=AXIS2_PLACEMENT_3D('',#64672,#51517,#51518);
#42202=AXIS2_PLACEMENT_3D('',#64674,#51520,#51521);
#42203=AXIS2_PLACEMENT_3D('',#64676,#51523,#51524);
#42204=AXIS2_PLACEMENT_3D('',#64677,#51525,#51526);
#42205=AXIS2_PLACEMENT_3D('',#64680,#51529,#51530);
#42206=AXIS2_PLACEMENT_3D('',#64682,#51532,#51533);
#42207=AXIS2_PLACEMENT_3D('',#64684,#51535,#51536);
#42208=AXIS2_PLACEMENT_3D('',#64686,#51538,#51539);
#42209=AXIS2_PLACEMENT_3D('',#64688,#51541,#51542);
#42210=AXIS2_PLACEMENT_3D('',#64689,#51543,#51544);
#42211=AXIS2_PLACEMENT_3D('',#64692,#51547,#51548);
#42212=AXIS2_PLACEMENT_3D('',#64694,#51550,#51551);
#42213=AXIS2_PLACEMENT_3D('',#64696,#51553,#51554);
#42214=AXIS2_PLACEMENT_3D('',#64698,#51556,#51557);
#42215=AXIS2_PLACEMENT_3D('',#64700,#51559,#51560);
#42216=AXIS2_PLACEMENT_3D('',#64701,#51561,#51562);
#42217=AXIS2_PLACEMENT_3D('',#64704,#51565,#51566);
#42218=AXIS2_PLACEMENT_3D('',#64706,#51568,#51569);
#42219=AXIS2_PLACEMENT_3D('',#64708,#51571,#51572);
#42220=AXIS2_PLACEMENT_3D('',#64710,#51574,#51575);
#42221=AXIS2_PLACEMENT_3D('',#64712,#51577,#51578);
#42222=AXIS2_PLACEMENT_3D('',#64713,#51579,#51580);
#42223=AXIS2_PLACEMENT_3D('',#64716,#51583,#51584);
#42224=AXIS2_PLACEMENT_3D('',#64718,#51586,#51587);
#42225=AXIS2_PLACEMENT_3D('',#64720,#51589,#51590);
#42226=AXIS2_PLACEMENT_3D('',#64722,#51592,#51593);
#42227=AXIS2_PLACEMENT_3D('',#64724,#51595,#51596);
#42228=AXIS2_PLACEMENT_3D('',#64725,#51597,#51598);
#42229=AXIS2_PLACEMENT_3D('',#64728,#51601,#51602);
#42230=AXIS2_PLACEMENT_3D('',#64730,#51604,#51605);
#42231=AXIS2_PLACEMENT_3D('',#64732,#51607,#51608);
#42232=AXIS2_PLACEMENT_3D('',#64734,#51610,#51611);
#42233=AXIS2_PLACEMENT_3D('',#64736,#51613,#51614);
#42234=AXIS2_PLACEMENT_3D('',#64737,#51615,#51616);
#42235=AXIS2_PLACEMENT_3D('',#64740,#51619,#51620);
#42236=AXIS2_PLACEMENT_3D('',#64742,#51622,#51623);
#42237=AXIS2_PLACEMENT_3D('',#64744,#51625,#51626);
#42238=AXIS2_PLACEMENT_3D('',#64746,#51628,#51629);
#42239=AXIS2_PLACEMENT_3D('',#64748,#51631,#51632);
#42240=AXIS2_PLACEMENT_3D('',#64749,#51633,#51634);
#42241=AXIS2_PLACEMENT_3D('',#64752,#51637,#51638);
#42242=AXIS2_PLACEMENT_3D('',#64754,#51640,#51641);
#42243=AXIS2_PLACEMENT_3D('',#64756,#51643,#51644);
#42244=AXIS2_PLACEMENT_3D('',#64758,#51646,#51647);
#42245=AXIS2_PLACEMENT_3D('',#64760,#51649,#51650);
#42246=AXIS2_PLACEMENT_3D('',#64761,#51651,#51652);
#42247=AXIS2_PLACEMENT_3D('',#64764,#51655,#51656);
#42248=AXIS2_PLACEMENT_3D('',#64766,#51658,#51659);
#42249=AXIS2_PLACEMENT_3D('',#64768,#51661,#51662);
#42250=AXIS2_PLACEMENT_3D('',#64770,#51664,#51665);
#42251=AXIS2_PLACEMENT_3D('',#64772,#51667,#51668);
#42252=AXIS2_PLACEMENT_3D('',#64773,#51669,#51670);
#42253=AXIS2_PLACEMENT_3D('',#64776,#51673,#51674);
#42254=AXIS2_PLACEMENT_3D('',#64778,#51676,#51677);
#42255=AXIS2_PLACEMENT_3D('',#64780,#51679,#51680);
#42256=AXIS2_PLACEMENT_3D('',#64782,#51682,#51683);
#42257=AXIS2_PLACEMENT_3D('',#64784,#51685,#51686);
#42258=AXIS2_PLACEMENT_3D('',#64785,#51687,#51688);
#42259=AXIS2_PLACEMENT_3D('',#64788,#51691,#51692);
#42260=AXIS2_PLACEMENT_3D('',#64790,#51694,#51695);
#42261=AXIS2_PLACEMENT_3D('',#64792,#51697,#51698);
#42262=AXIS2_PLACEMENT_3D('',#64794,#51700,#51701);
#42263=AXIS2_PLACEMENT_3D('',#64796,#51703,#51704);
#42264=AXIS2_PLACEMENT_3D('',#64797,#51705,#51706);
#42265=AXIS2_PLACEMENT_3D('',#64800,#51709,#51710);
#42266=AXIS2_PLACEMENT_3D('',#64802,#51712,#51713);
#42267=AXIS2_PLACEMENT_3D('',#64804,#51715,#51716);
#42268=AXIS2_PLACEMENT_3D('',#64806,#51718,#51719);
#42269=AXIS2_PLACEMENT_3D('',#64808,#51721,#51722);
#42270=AXIS2_PLACEMENT_3D('',#64809,#51723,#51724);
#42271=AXIS2_PLACEMENT_3D('',#64812,#51727,#51728);
#42272=AXIS2_PLACEMENT_3D('',#64814,#51730,#51731);
#42273=AXIS2_PLACEMENT_3D('',#64816,#51733,#51734);
#42274=AXIS2_PLACEMENT_3D('',#64818,#51736,#51737);
#42275=AXIS2_PLACEMENT_3D('',#64820,#51739,#51740);
#42276=AXIS2_PLACEMENT_3D('',#64821,#51741,#51742);
#42277=AXIS2_PLACEMENT_3D('',#64824,#51745,#51746);
#42278=AXIS2_PLACEMENT_3D('',#64826,#51748,#51749);
#42279=AXIS2_PLACEMENT_3D('',#64828,#51751,#51752);
#42280=AXIS2_PLACEMENT_3D('',#64830,#51754,#51755);
#42281=AXIS2_PLACEMENT_3D('',#64832,#51757,#51758);
#42282=AXIS2_PLACEMENT_3D('',#64833,#51759,#51760);
#42283=AXIS2_PLACEMENT_3D('',#64836,#51763,#51764);
#42284=AXIS2_PLACEMENT_3D('',#64838,#51766,#51767);
#42285=AXIS2_PLACEMENT_3D('',#64840,#51769,#51770);
#42286=AXIS2_PLACEMENT_3D('',#64842,#51772,#51773);
#42287=AXIS2_PLACEMENT_3D('',#64844,#51775,#51776);
#42288=AXIS2_PLACEMENT_3D('',#64845,#51777,#51778);
#42289=AXIS2_PLACEMENT_3D('',#64848,#51781,#51782);
#42290=AXIS2_PLACEMENT_3D('',#64850,#51784,#51785);
#42291=AXIS2_PLACEMENT_3D('',#64852,#51787,#51788);
#42292=AXIS2_PLACEMENT_3D('',#64854,#51790,#51791);
#42293=AXIS2_PLACEMENT_3D('',#64856,#51793,#51794);
#42294=AXIS2_PLACEMENT_3D('',#64857,#51795,#51796);
#42295=AXIS2_PLACEMENT_3D('',#64860,#51799,#51800);
#42296=AXIS2_PLACEMENT_3D('',#64862,#51802,#51803);
#42297=AXIS2_PLACEMENT_3D('',#64864,#51805,#51806);
#42298=AXIS2_PLACEMENT_3D('',#64866,#51808,#51809);
#42299=AXIS2_PLACEMENT_3D('',#64868,#51811,#51812);
#42300=AXIS2_PLACEMENT_3D('',#64869,#51813,#51814);
#42301=AXIS2_PLACEMENT_3D('',#64872,#51817,#51818);
#42302=AXIS2_PLACEMENT_3D('',#64874,#51820,#51821);
#42303=AXIS2_PLACEMENT_3D('',#64876,#51823,#51824);
#42304=AXIS2_PLACEMENT_3D('',#64878,#51826,#51827);
#42305=AXIS2_PLACEMENT_3D('',#64880,#51829,#51830);
#42306=AXIS2_PLACEMENT_3D('',#64881,#51831,#51832);
#42307=AXIS2_PLACEMENT_3D('',#64884,#51835,#51836);
#42308=AXIS2_PLACEMENT_3D('',#64886,#51838,#51839);
#42309=AXIS2_PLACEMENT_3D('',#64888,#51841,#51842);
#42310=AXIS2_PLACEMENT_3D('',#64890,#51844,#51845);
#42311=AXIS2_PLACEMENT_3D('',#64892,#51847,#51848);
#42312=AXIS2_PLACEMENT_3D('',#64893,#51849,#51850);
#42313=AXIS2_PLACEMENT_3D('',#64896,#51853,#51854);
#42314=AXIS2_PLACEMENT_3D('',#64898,#51856,#51857);
#42315=AXIS2_PLACEMENT_3D('',#64900,#51859,#51860);
#42316=AXIS2_PLACEMENT_3D('',#64902,#51862,#51863);
#42317=AXIS2_PLACEMENT_3D('',#64904,#51865,#51866);
#42318=AXIS2_PLACEMENT_3D('',#64905,#51867,#51868);
#42319=AXIS2_PLACEMENT_3D('',#64908,#51871,#51872);
#42320=AXIS2_PLACEMENT_3D('',#64910,#51874,#51875);
#42321=AXIS2_PLACEMENT_3D('',#64912,#51877,#51878);
#42322=AXIS2_PLACEMENT_3D('',#64914,#51880,#51881);
#42323=AXIS2_PLACEMENT_3D('',#64916,#51883,#51884);
#42324=AXIS2_PLACEMENT_3D('',#64917,#51885,#51886);
#42325=AXIS2_PLACEMENT_3D('',#64920,#51889,#51890);
#42326=AXIS2_PLACEMENT_3D('',#64922,#51892,#51893);
#42327=AXIS2_PLACEMENT_3D('',#64924,#51895,#51896);
#42328=AXIS2_PLACEMENT_3D('',#64926,#51898,#51899);
#42329=AXIS2_PLACEMENT_3D('',#64928,#51901,#51902);
#42330=AXIS2_PLACEMENT_3D('',#64929,#51903,#51904);
#42331=AXIS2_PLACEMENT_3D('',#64932,#51907,#51908);
#42332=AXIS2_PLACEMENT_3D('',#64934,#51910,#51911);
#42333=AXIS2_PLACEMENT_3D('',#64936,#51913,#51914);
#42334=AXIS2_PLACEMENT_3D('',#64938,#51916,#51917);
#42335=AXIS2_PLACEMENT_3D('',#64940,#51919,#51920);
#42336=AXIS2_PLACEMENT_3D('',#64941,#51921,#51922);
#42337=AXIS2_PLACEMENT_3D('',#64944,#51925,#51926);
#42338=AXIS2_PLACEMENT_3D('',#64946,#51928,#51929);
#42339=AXIS2_PLACEMENT_3D('',#64948,#51931,#51932);
#42340=AXIS2_PLACEMENT_3D('',#64950,#51934,#51935);
#42341=AXIS2_PLACEMENT_3D('',#64952,#51937,#51938);
#42342=AXIS2_PLACEMENT_3D('',#64953,#51939,#51940);
#42343=AXIS2_PLACEMENT_3D('',#64956,#51943,#51944);
#42344=AXIS2_PLACEMENT_3D('',#64958,#51946,#51947);
#42345=AXIS2_PLACEMENT_3D('',#64960,#51949,#51950);
#42346=AXIS2_PLACEMENT_3D('',#64962,#51952,#51953);
#42347=AXIS2_PLACEMENT_3D('',#64964,#51955,#51956);
#42348=AXIS2_PLACEMENT_3D('',#64965,#51957,#51958);
#42349=AXIS2_PLACEMENT_3D('',#64968,#51961,#51962);
#42350=AXIS2_PLACEMENT_3D('',#64970,#51964,#51965);
#42351=AXIS2_PLACEMENT_3D('',#64972,#51967,#51968);
#42352=AXIS2_PLACEMENT_3D('',#64974,#51970,#51971);
#42353=AXIS2_PLACEMENT_3D('',#64976,#51973,#51974);
#42354=AXIS2_PLACEMENT_3D('',#64977,#51975,#51976);
#42355=AXIS2_PLACEMENT_3D('',#64980,#51979,#51980);
#42356=AXIS2_PLACEMENT_3D('',#64982,#51982,#51983);
#42357=AXIS2_PLACEMENT_3D('',#64984,#51985,#51986);
#42358=AXIS2_PLACEMENT_3D('',#64986,#51988,#51989);
#42359=AXIS2_PLACEMENT_3D('',#64988,#51991,#51992);
#42360=AXIS2_PLACEMENT_3D('',#64989,#51993,#51994);
#42361=AXIS2_PLACEMENT_3D('',#64992,#51997,#51998);
#42362=AXIS2_PLACEMENT_3D('',#64994,#52000,#52001);
#42363=AXIS2_PLACEMENT_3D('',#64996,#52003,#52004);
#42364=AXIS2_PLACEMENT_3D('',#64998,#52006,#52007);
#42365=AXIS2_PLACEMENT_3D('',#65000,#52009,#52010);
#42366=AXIS2_PLACEMENT_3D('',#65001,#52011,#52012);
#42367=AXIS2_PLACEMENT_3D('',#65004,#52015,#52016);
#42368=AXIS2_PLACEMENT_3D('',#65006,#52018,#52019);
#42369=AXIS2_PLACEMENT_3D('',#65008,#52021,#52022);
#42370=AXIS2_PLACEMENT_3D('',#65010,#52024,#52025);
#42371=AXIS2_PLACEMENT_3D('',#65012,#52027,#52028);
#42372=AXIS2_PLACEMENT_3D('',#65013,#52029,#52030);
#42373=AXIS2_PLACEMENT_3D('',#65016,#52033,#52034);
#42374=AXIS2_PLACEMENT_3D('',#65018,#52036,#52037);
#42375=AXIS2_PLACEMENT_3D('',#65020,#52039,#52040);
#42376=AXIS2_PLACEMENT_3D('',#65022,#52042,#52043);
#42377=AXIS2_PLACEMENT_3D('',#65024,#52045,#52046);
#42378=AXIS2_PLACEMENT_3D('',#65025,#52047,#52048);
#42379=AXIS2_PLACEMENT_3D('',#65028,#52051,#52052);
#42380=AXIS2_PLACEMENT_3D('',#65030,#52054,#52055);
#42381=AXIS2_PLACEMENT_3D('',#65032,#52057,#52058);
#42382=AXIS2_PLACEMENT_3D('',#65034,#52060,#52061);
#42383=AXIS2_PLACEMENT_3D('',#65036,#52063,#52064);
#42384=AXIS2_PLACEMENT_3D('',#65037,#52065,#52066);
#42385=AXIS2_PLACEMENT_3D('',#65040,#52069,#52070);
#42386=AXIS2_PLACEMENT_3D('',#65042,#52072,#52073);
#42387=AXIS2_PLACEMENT_3D('',#65044,#52075,#52076);
#42388=AXIS2_PLACEMENT_3D('',#65046,#52078,#52079);
#42389=AXIS2_PLACEMENT_3D('',#65048,#52081,#52082);
#42390=AXIS2_PLACEMENT_3D('',#65049,#52083,#52084);
#42391=AXIS2_PLACEMENT_3D('',#65052,#52087,#52088);
#42392=AXIS2_PLACEMENT_3D('',#65054,#52090,#52091);
#42393=AXIS2_PLACEMENT_3D('',#65056,#52093,#52094);
#42394=AXIS2_PLACEMENT_3D('',#65058,#52096,#52097);
#42395=AXIS2_PLACEMENT_3D('',#65060,#52099,#52100);
#42396=AXIS2_PLACEMENT_3D('',#65061,#52101,#52102);
#42397=AXIS2_PLACEMENT_3D('',#65064,#52105,#52106);
#42398=AXIS2_PLACEMENT_3D('',#65066,#52108,#52109);
#42399=AXIS2_PLACEMENT_3D('',#65068,#52111,#52112);
#42400=AXIS2_PLACEMENT_3D('',#65070,#52114,#52115);
#42401=AXIS2_PLACEMENT_3D('',#65072,#52117,#52118);
#42402=AXIS2_PLACEMENT_3D('',#65073,#52119,#52120);
#42403=AXIS2_PLACEMENT_3D('',#65076,#52123,#52124);
#42404=AXIS2_PLACEMENT_3D('',#65078,#52126,#52127);
#42405=AXIS2_PLACEMENT_3D('',#65080,#52129,#52130);
#42406=AXIS2_PLACEMENT_3D('',#65082,#52132,#52133);
#42407=AXIS2_PLACEMENT_3D('',#65084,#52135,#52136);
#42408=AXIS2_PLACEMENT_3D('',#65085,#52137,#52138);
#42409=AXIS2_PLACEMENT_3D('',#65088,#52141,#52142);
#42410=AXIS2_PLACEMENT_3D('',#65090,#52144,#52145);
#42411=AXIS2_PLACEMENT_3D('',#65092,#52147,#52148);
#42412=AXIS2_PLACEMENT_3D('',#65094,#52150,#52151);
#42413=AXIS2_PLACEMENT_3D('',#65096,#52153,#52154);
#42414=AXIS2_PLACEMENT_3D('',#65097,#52155,#52156);
#42415=AXIS2_PLACEMENT_3D('',#65100,#52159,#52160);
#42416=AXIS2_PLACEMENT_3D('',#65102,#52162,#52163);
#42417=AXIS2_PLACEMENT_3D('',#65104,#52165,#52166);
#42418=AXIS2_PLACEMENT_3D('',#65106,#52168,#52169);
#42419=AXIS2_PLACEMENT_3D('',#65108,#52171,#52172);
#42420=AXIS2_PLACEMENT_3D('',#65109,#52173,#52174);
#42421=AXIS2_PLACEMENT_3D('',#65112,#52177,#52178);
#42422=AXIS2_PLACEMENT_3D('',#65114,#52180,#52181);
#42423=AXIS2_PLACEMENT_3D('',#65116,#52183,#52184);
#42424=AXIS2_PLACEMENT_3D('',#65118,#52186,#52187);
#42425=AXIS2_PLACEMENT_3D('',#65120,#52189,#52190);
#42426=AXIS2_PLACEMENT_3D('',#65121,#52191,#52192);
#42427=AXIS2_PLACEMENT_3D('',#65124,#52195,#52196);
#42428=AXIS2_PLACEMENT_3D('',#65126,#52198,#52199);
#42429=AXIS2_PLACEMENT_3D('',#65128,#52201,#52202);
#42430=AXIS2_PLACEMENT_3D('',#65130,#52204,#52205);
#42431=AXIS2_PLACEMENT_3D('',#65132,#52207,#52208);
#42432=AXIS2_PLACEMENT_3D('',#65133,#52209,#52210);
#42433=AXIS2_PLACEMENT_3D('',#65136,#52213,#52214);
#42434=AXIS2_PLACEMENT_3D('',#65138,#52216,#52217);
#42435=AXIS2_PLACEMENT_3D('',#65140,#52219,#52220);
#42436=AXIS2_PLACEMENT_3D('',#65142,#52222,#52223);
#42437=AXIS2_PLACEMENT_3D('',#65144,#52225,#52226);
#42438=AXIS2_PLACEMENT_3D('',#65145,#52227,#52228);
#42439=AXIS2_PLACEMENT_3D('',#65148,#52231,#52232);
#42440=AXIS2_PLACEMENT_3D('',#65150,#52234,#52235);
#42441=AXIS2_PLACEMENT_3D('',#65152,#52237,#52238);
#42442=AXIS2_PLACEMENT_3D('',#65154,#52240,#52241);
#42443=AXIS2_PLACEMENT_3D('',#65156,#52243,#52244);
#42444=AXIS2_PLACEMENT_3D('',#65157,#52245,#52246);
#42445=AXIS2_PLACEMENT_3D('',#65160,#52249,#52250);
#42446=AXIS2_PLACEMENT_3D('',#65162,#52252,#52253);
#42447=AXIS2_PLACEMENT_3D('',#65164,#52255,#52256);
#42448=AXIS2_PLACEMENT_3D('',#65166,#52258,#52259);
#42449=AXIS2_PLACEMENT_3D('',#65168,#52261,#52262);
#42450=AXIS2_PLACEMENT_3D('',#65169,#52263,#52264);
#42451=AXIS2_PLACEMENT_3D('',#65172,#52267,#52268);
#42452=AXIS2_PLACEMENT_3D('',#65174,#52270,#52271);
#42453=AXIS2_PLACEMENT_3D('',#65176,#52273,#52274);
#42454=AXIS2_PLACEMENT_3D('',#65178,#52276,#52277);
#42455=AXIS2_PLACEMENT_3D('',#65180,#52279,#52280);
#42456=AXIS2_PLACEMENT_3D('',#65181,#52281,#52282);
#42457=AXIS2_PLACEMENT_3D('',#65184,#52285,#52286);
#42458=AXIS2_PLACEMENT_3D('',#65186,#52288,#52289);
#42459=AXIS2_PLACEMENT_3D('',#65188,#52291,#52292);
#42460=AXIS2_PLACEMENT_3D('',#65190,#52294,#52295);
#42461=AXIS2_PLACEMENT_3D('',#65192,#52297,#52298);
#42462=AXIS2_PLACEMENT_3D('',#65193,#52299,#52300);
#42463=AXIS2_PLACEMENT_3D('',#65196,#52303,#52304);
#42464=AXIS2_PLACEMENT_3D('',#65198,#52306,#52307);
#42465=AXIS2_PLACEMENT_3D('',#65200,#52309,#52310);
#42466=AXIS2_PLACEMENT_3D('',#65202,#52312,#52313);
#42467=AXIS2_PLACEMENT_3D('',#65204,#52315,#52316);
#42468=AXIS2_PLACEMENT_3D('',#65205,#52317,#52318);
#42469=AXIS2_PLACEMENT_3D('',#65208,#52321,#52322);
#42470=AXIS2_PLACEMENT_3D('',#65210,#52324,#52325);
#42471=AXIS2_PLACEMENT_3D('',#65212,#52327,#52328);
#42472=AXIS2_PLACEMENT_3D('',#65214,#52330,#52331);
#42473=AXIS2_PLACEMENT_3D('',#65216,#52333,#52334);
#42474=AXIS2_PLACEMENT_3D('',#65217,#52335,#52336);
#42475=AXIS2_PLACEMENT_3D('',#65220,#52339,#52340);
#42476=AXIS2_PLACEMENT_3D('',#65222,#52342,#52343);
#42477=AXIS2_PLACEMENT_3D('',#65224,#52345,#52346);
#42478=AXIS2_PLACEMENT_3D('',#65226,#52348,#52349);
#42479=AXIS2_PLACEMENT_3D('',#65228,#52351,#52352);
#42480=AXIS2_PLACEMENT_3D('',#65229,#52353,#52354);
#42481=AXIS2_PLACEMENT_3D('',#65232,#52357,#52358);
#42482=AXIS2_PLACEMENT_3D('',#65234,#52360,#52361);
#42483=AXIS2_PLACEMENT_3D('',#65236,#52363,#52364);
#42484=AXIS2_PLACEMENT_3D('',#65238,#52366,#52367);
#42485=AXIS2_PLACEMENT_3D('',#65240,#52369,#52370);
#42486=AXIS2_PLACEMENT_3D('',#65241,#52371,#52372);
#42487=AXIS2_PLACEMENT_3D('',#65244,#52375,#52376);
#42488=AXIS2_PLACEMENT_3D('',#65246,#52378,#52379);
#42489=AXIS2_PLACEMENT_3D('',#65248,#52381,#52382);
#42490=AXIS2_PLACEMENT_3D('',#65250,#52384,#52385);
#42491=AXIS2_PLACEMENT_3D('',#65252,#52387,#52388);
#42492=AXIS2_PLACEMENT_3D('',#65253,#52389,#52390);
#42493=AXIS2_PLACEMENT_3D('',#65256,#52393,#52394);
#42494=AXIS2_PLACEMENT_3D('',#65258,#52396,#52397);
#42495=AXIS2_PLACEMENT_3D('',#65260,#52399,#52400);
#42496=AXIS2_PLACEMENT_3D('',#65262,#52402,#52403);
#42497=AXIS2_PLACEMENT_3D('',#65264,#52405,#52406);
#42498=AXIS2_PLACEMENT_3D('',#65265,#52407,#52408);
#42499=AXIS2_PLACEMENT_3D('',#65268,#52411,#52412);
#42500=AXIS2_PLACEMENT_3D('',#65270,#52414,#52415);
#42501=AXIS2_PLACEMENT_3D('',#65272,#52417,#52418);
#42502=AXIS2_PLACEMENT_3D('',#65274,#52420,#52421);
#42503=AXIS2_PLACEMENT_3D('',#65276,#52423,#52424);
#42504=AXIS2_PLACEMENT_3D('',#65277,#52425,#52426);
#42505=AXIS2_PLACEMENT_3D('',#65280,#52429,#52430);
#42506=AXIS2_PLACEMENT_3D('',#65282,#52432,#52433);
#42507=AXIS2_PLACEMENT_3D('',#65284,#52435,#52436);
#42508=AXIS2_PLACEMENT_3D('',#65286,#52438,#52439);
#42509=AXIS2_PLACEMENT_3D('',#65288,#52441,#52442);
#46601=DIRECTION('axis',(0.,0.,1.));
#46602=DIRECTION('refdir',(1.,0.,0.));
#46603=DIRECTION('center_axis',(0.,1.,0.));
#46604=DIRECTION('ref_axis',(1.,0.,0.));
#46605=DIRECTION('center_axis',(0.,1.,0.));
#46606=DIRECTION('ref_axis',(-1.,0.,0.));
#46607=DIRECTION('center_axis',(-1.48029736616688E-16,0.,-1.));
#46608=DIRECTION('ref_axis',(-1.,0.,1.48029736616688E-16));
#46609=DIRECTION('center_axis',(0.,1.,0.));
#46610=DIRECTION('ref_axis',(1.,0.,0.));
#46611=DIRECTION('center_axis',(0.,1.,0.));
#46612=DIRECTION('ref_axis',(1.,0.,0.));
#46613=DIRECTION('center_axis',(0.,1.,0.));
#46614=DIRECTION('ref_axis',(0.,0.,1.));
#46615=DIRECTION('center_axis',(-1.40646966953779E-16,0.,-1.));
#46616=DIRECTION('ref_axis',(-1.,0.,1.40646966953779E-16));
#46617=DIRECTION('center_axis',(0.,1.,0.));
#46618=DIRECTION('ref_axis',(0.,0.,1.));
#46619=DIRECTION('center_axis',(0.,1.,0.));
#46620=DIRECTION('ref_axis',(1.,0.,0.));
#46621=DIRECTION('center_axis',(0.,1.,0.));
#46622=DIRECTION('ref_axis',(0.,0.,1.));
#46623=DIRECTION('center_axis',(1.46081976924363E-16,0.,1.));
#46624=DIRECTION('ref_axis',(-1.,0.,1.46081976924363E-16));
#46625=DIRECTION('center_axis',(0.,1.,0.));
#46626=DIRECTION('ref_axis',(1.,0.,0.));
#46627=DIRECTION('center_axis',(0.,-1.,0.));
#46628=DIRECTION('ref_axis',(1.,0.,0.));
#46629=DIRECTION('center_axis',(1.38887491248569E-16,0.,1.));
#46630=DIRECTION('ref_axis',(-1.,0.,1.38887491248569E-16));
#46631=DIRECTION('center_axis',(0.,-1.,0.));
#46632=DIRECTION('ref_axis',(0.,0.,-1.));
#46633=DIRECTION('',(-1.,0.,0.));
#46634=DIRECTION('',(0.,0.,1.));
#46635=DIRECTION('',(-1.,0.,0.));
#46636=DIRECTION('',(0.,0.,1.));
#46637=DIRECTION('',(1.,0.,0.));
#46638=DIRECTION('',(0.,0.,1.));
#46639=DIRECTION('',(1.,0.,0.));
#46640=DIRECTION('',(1.38777878078145E-15,0.,1.));
#46641=DIRECTION('',(1.,0.,0.));
#46642=DIRECTION('',(0.,0.,1.));
#46643=DIRECTION('',(1.,0.,0.));
#46644=DIRECTION('',(0.,0.,1.));
#46645=DIRECTION('center_axis',(0.,-1.,0.));
#46646=DIRECTION('ref_axis',(0.,0.,-1.));
#46647=DIRECTION('',(0.,0.,-1.));
#46648=DIRECTION('',(1.,0.,0.));
#46649=DIRECTION('',(0.,0.,1.));
#46650=DIRECTION('',(1.,0.,0.));
#46651=DIRECTION('',(0.,0.,1.));
#46652=DIRECTION('',(-1.,0.,0.));
#46653=DIRECTION('',(-1.38777878078145E-15,0.,-1.));
#46654=DIRECTION('',(-1.,0.,0.));
#46655=DIRECTION('',(0.,0.,1.));
#46656=DIRECTION('',(1.,0.,0.));
#46657=DIRECTION('',(0.,0.,1.));
#46658=DIRECTION('',(1.,0.,0.));
#46659=DIRECTION('center_axis',(0.,0.,1.));
#46660=DIRECTION('ref_axis',(1.,0.,0.));
#46661=DIRECTION('',(0.,1.,0.));
#46662=DIRECTION('',(0.,-1.,0.));
#46663=DIRECTION('center_axis',(0.,0.,-1.));
#46664=DIRECTION('ref_axis',(-1.,0.,0.));
#46665=DIRECTION('',(0.,1.,0.));
#46666=DIRECTION('',(0.,-1.,0.));
#46667=DIRECTION('center_axis',(0.,0.,1.));
#46668=DIRECTION('ref_axis',(1.,0.,0.));
#46669=DIRECTION('',(0.,-1.,0.));
#46670=DIRECTION('',(0.,1.,0.));
#46671=DIRECTION('center_axis',(0.,0.,1.));
#46672=DIRECTION('ref_axis',(1.,0.,0.));
#46673=DIRECTION('',(0.,1.,0.));
#46674=DIRECTION('',(0.,1.,0.));
#46675=DIRECTION('center_axis',(1.,0.,0.));
#46676=DIRECTION('ref_axis',(0.,0.,-1.));
#46677=DIRECTION('center_axis',(0.,0.,-1.));
#46678=DIRECTION('ref_axis',(-1.,0.,0.));
#46679=DIRECTION('',(0.,1.,0.));
#46680=DIRECTION('',(0.,1.,0.));
#46681=DIRECTION('center_axis',(1.,0.,-1.38777878078145E-15));
#46682=DIRECTION('ref_axis',(-1.38777878078145E-15,0.,-1.));
#46683=DIRECTION('',(0.,1.,0.));
#46684=DIRECTION('center_axis',(0.,0.,-1.));
#46685=DIRECTION('ref_axis',(-1.,0.,0.));
#46686=DIRECTION('',(0.,-1.,0.));
#46687=DIRECTION('center_axis',(0.,0.,-1.));
#46688=DIRECTION('ref_axis',(-1.,0.,0.));
#46689=DIRECTION('',(-1.,-6.12323399573677E-17,8.67361737988424E-15));
#46690=DIRECTION('center_axis',(0.,0.,1.));
#46691=DIRECTION('ref_axis',(-1.,0.,0.));
#46692=DIRECTION('center_axis',(0.,0.,1.));
#46693=DIRECTION('ref_axis',(1.,0.,0.));
#46694=DIRECTION('center_axis',(0.,0.,1.));
#46695=DIRECTION('ref_axis',(1.,0.,0.));
#46696=DIRECTION('center_axis',(0.,0.,-1.));
#46697=DIRECTION('ref_axis',(-1.,0.,0.));
#46698=DIRECTION('',(-1.,0.,0.));
#46699=DIRECTION('center_axis',(0.,0.,-1.));
#46700=DIRECTION('ref_axis',(-1.,0.,0.));
#46701=DIRECTION('center_axis',(0.,0.,-1.));
#46702=DIRECTION('ref_axis',(-1.,0.,0.));
#46703=DIRECTION('',(0.,0.,1.));
#46704=DIRECTION('center_axis',(0.,0.,-1.));
#46705=DIRECTION('ref_axis',(-1.,0.,0.));
#46706=DIRECTION('',(0.,0.,1.));
#46707=DIRECTION('center_axis',(0.,0.,1.));
#46708=DIRECTION('ref_axis',(1.,0.,0.));
#46709=DIRECTION('center_axis',(0.,0.,-1.));
#46710=DIRECTION('ref_axis',(-1.,0.,0.));
#46711=DIRECTION('',(1.,6.12323399573677E-17,0.));
#46712=DIRECTION('center_axis',(0.,0.,-1.));
#46713=DIRECTION('ref_axis',(1.,0.,0.));
#46714=DIRECTION('center_axis',(0.,0.,-1.));
#46715=DIRECTION('ref_axis',(-1.,0.,0.));
#46716=DIRECTION('',(1.,0.,0.));
#46717=DIRECTION('center_axis',(0.,0.,1.));
#46718=DIRECTION('ref_axis',(-1.,0.,0.));
#46719=DIRECTION('center_axis',(0.,0.,1.));
#46720=DIRECTION('ref_axis',(1.,0.,0.));
#46721=DIRECTION('center_axis',(0.,0.,-1.));
#46722=DIRECTION('ref_axis',(-1.,0.,0.));
#46723=DIRECTION('',(0.,0.,1.));
#46724=DIRECTION('center_axis',(0.,0.,-1.));
#46725=DIRECTION('ref_axis',(-1.,0.,0.));
#46726=DIRECTION('',(0.,0.,1.));
#46727=DIRECTION('center_axis',(1.,0.,0.));
#46728=DIRECTION('ref_axis',(0.,1.,0.));
#46729=DIRECTION('center_axis',(1.,0.,0.));
#46730=DIRECTION('ref_axis',(0.,-1.,0.));
#46731=DIRECTION('',(1.,0.,0.));
#46732=DIRECTION('center_axis',(-1.,0.,0.));
#46733=DIRECTION('ref_axis',(0.,-1.,0.));
#46734=DIRECTION('',(-1.,0.,0.));
#46735=DIRECTION('center_axis',(6.12323399573677E-17,-1.,-1.38777878078145E-15));
#46736=DIRECTION('ref_axis',(-8.49769420904307E-32,1.38777878078145E-15,
-1.));
#46737=DIRECTION('',(0.,-1.38777878078145E-15,1.));
#46738=DIRECTION('',(1.,6.12323399573677E-17,0.));
#46739=DIRECTION('',(-8.49769420904308E-32,1.38777878078145E-15,-1.));
#46740=DIRECTION('',(1.,6.12323399573677E-17,0.));
#46741=DIRECTION('center_axis',(1.,0.,0.));
#46742=DIRECTION('ref_axis',(0.,1.,0.));
#46743=DIRECTION('center_axis',(1.,0.,0.));
#46744=DIRECTION('ref_axis',(0.,-1.,0.));
#46745=DIRECTION('',(1.,0.,0.));
#46746=DIRECTION('center_axis',(-1.,0.,0.));
#46747=DIRECTION('ref_axis',(0.,-1.,0.));
#46748=DIRECTION('',(-1.,0.,0.));
#46749=DIRECTION('center_axis',(0.,1.,0.));
#46750=DIRECTION('ref_axis',(0.,0.,1.));
#46751=DIRECTION('',(0.,0.,1.));
#46752=DIRECTION('',(0.,0.,1.));
#46753=DIRECTION('center_axis',(-1.,0.,0.));
#46754=DIRECTION('ref_axis',(0.,0.,1.));
#46755=DIRECTION('',(0.,-1.,0.));
#46756=DIRECTION('',(-6.12323399573677E-17,1.,0.));
#46757=DIRECTION('',(-6.12323399573677E-17,1.,0.));
#46758=DIRECTION('',(0.,-1.,0.));
#46759=DIRECTION('center_axis',(0.,0.,-1.));
#46760=DIRECTION('ref_axis',(-6.12323399573677E-17,1.,0.));
#46761=DIRECTION('',(0.,-1.,0.));
#46762=DIRECTION('center_axis',(-1.,0.,0.));
#46763=DIRECTION('ref_axis',(0.,0.,1.));
#46764=DIRECTION('',(0.,-1.,0.));
#46765=DIRECTION('',(0.,-1.,0.));
#46766=DIRECTION('',(0.,-1.,0.));
#46767=DIRECTION('center_axis',(0.,0.,-1.));
#46768=DIRECTION('ref_axis',(-1.,0.,0.));
#46769=DIRECTION('center_axis',(0.,0.,1.));
#46770=DIRECTION('ref_axis',(1.,0.,0.));
#46771=DIRECTION('center_axis',(0.,0.,-1.));
#46772=DIRECTION('ref_axis',(-6.12323399573677E-17,1.,0.));
#46773=DIRECTION('center_axis',(0.,0.,1.));
#46774=DIRECTION('ref_axis',(1.,0.,0.));
#46775=DIRECTION('',(1.,-6.12323399573677E-17,0.));
#46776=DIRECTION('center_axis',(0.,0.,-1.));
#46777=DIRECTION('ref_axis',(1.,0.,0.));
#46778=DIRECTION('center_axis',(0.,0.,-1.));
#46779=DIRECTION('ref_axis',(-1.,0.,0.));
#46780=DIRECTION('center_axis',(0.,0.,-1.));
#46781=DIRECTION('ref_axis',(-1.,0.,0.));
#46782=DIRECTION('center_axis',(0.,0.,1.));
#46783=DIRECTION('ref_axis',(1.,0.,0.));
#46784=DIRECTION('',(1.,0.,0.));
#46785=DIRECTION('center_axis',(0.,0.,1.));
#46786=DIRECTION('ref_axis',(1.,0.,0.));
#46787=DIRECTION('center_axis',(0.,0.,1.));
#46788=DIRECTION('ref_axis',(1.,0.,0.));
#46789=DIRECTION('',(0.,0.,1.));
#46790=DIRECTION('center_axis',(0.,0.,1.));
#46791=DIRECTION('ref_axis',(1.,0.,0.));
#46792=DIRECTION('',(0.,0.,1.));
#46793=DIRECTION('center_axis',(0.,0.,-1.));
#46794=DIRECTION('ref_axis',(-1.,0.,0.));
#46795=DIRECTION('center_axis',(0.,0.,1.));
#46796=DIRECTION('ref_axis',(1.,0.,0.));
#46797=DIRECTION('',(-1.,6.12323399573677E-17,-8.67361737988394E-15));
#46798=DIRECTION('center_axis',(0.,0.,1.));
#46799=DIRECTION('ref_axis',(-1.,0.,0.));
#46800=DIRECTION('center_axis',(0.,0.,1.));
#46801=DIRECTION('ref_axis',(1.,0.,0.));
#46802=DIRECTION('',(-1.,0.,0.));
#46803=DIRECTION('center_axis',(0.,0.,-1.));
#46804=DIRECTION('ref_axis',(1.,0.,0.));
#46805=DIRECTION('center_axis',(0.,0.,-1.));
#46806=DIRECTION('ref_axis',(-1.,0.,0.));
#46807=DIRECTION('center_axis',(0.,0.,1.));
#46808=DIRECTION('ref_axis',(1.,0.,0.));
#46809=DIRECTION('',(0.,0.,1.));
#46810=DIRECTION('center_axis',(0.,0.,1.));
#46811=DIRECTION('ref_axis',(1.,0.,0.));
#46812=DIRECTION('',(0.,0.,1.));
#46813=DIRECTION('center_axis',(-1.,0.,0.));
#46814=DIRECTION('ref_axis',(0.,-1.,0.));
#46815=DIRECTION('center_axis',(1.,0.,0.));
#46816=DIRECTION('ref_axis',(0.,1.,0.));
#46817=DIRECTION('',(1.,0.,0.));
#46818=DIRECTION('center_axis',(-1.,0.,0.));
#46819=DIRECTION('ref_axis',(0.,1.,0.));
#46820=DIRECTION('',(-1.,0.,0.));
#46821=DIRECTION('center_axis',(6.12323399573677E-17,1.,0.));
#46822=DIRECTION('ref_axis',(0.,0.,-1.));
#46823=DIRECTION('',(-1.,6.12323399573677E-17,0.));
#46824=DIRECTION('',(0.,0.,-1.));
#46825=DIRECTION('',(-1.,6.12323399573677E-17,0.));
#46826=DIRECTION('',(0.,0.,1.));
#46827=DIRECTION('center_axis',(1.,0.,0.));
#46828=DIRECTION('ref_axis',(0.,1.,0.));
#46829=DIRECTION('center_axis',(1.,0.,0.));
#46830=DIRECTION('ref_axis',(0.,1.,0.));
#46831=DIRECTION('',(1.,0.,0.));
#46832=DIRECTION('center_axis',(-1.,0.,0.));
#46833=DIRECTION('ref_axis',(0.,1.,0.));
#46834=DIRECTION('',(-1.,0.,0.));
#46835=DIRECTION('center_axis',(0.,1.,0.));
#46836=DIRECTION('ref_axis',(0.,0.,1.));
#46837=DIRECTION('',(0.,0.,1.));
#46838=DIRECTION('',(0.,0.,1.));
#46839=DIRECTION('center_axis',(1.,0.,0.));
#46840=DIRECTION('ref_axis',(0.,0.,-1.));
#46841=DIRECTION('',(0.,1.,0.));
#46842=DIRECTION('',(6.12323399573677E-17,1.,0.));
#46843=DIRECTION('',(6.12323399573677E-17,1.,0.));
#46844=DIRECTION('',(0.,1.,0.));
#46845=DIRECTION('center_axis',(0.,0.,1.));
#46846=DIRECTION('ref_axis',(6.12323399573677E-17,1.,0.));
#46847=DIRECTION('',(0.,-1.,0.));
#46848=DIRECTION('center_axis',(1.,0.,0.));
#46849=DIRECTION('ref_axis',(0.,0.,-1.));
#46850=DIRECTION('',(0.,1.,0.));
#46851=DIRECTION('',(0.,1.,0.));
#46852=DIRECTION('',(0.,-1.,0.));
#46853=DIRECTION('center_axis',(0.,0.,1.));
#46854=DIRECTION('ref_axis',(1.,0.,0.));
#46855=DIRECTION('center_axis',(0.,0.,1.));
#46856=DIRECTION('ref_axis',(1.,0.,0.));
#46857=DIRECTION('center_axis',(0.,0.,1.));
#46858=DIRECTION('ref_axis',(6.12323399573677E-17,1.,0.));
#46859=DIRECTION('center_axis',(0.,1.,0.));
#46860=DIRECTION('ref_axis',(1.,0.,0.));
#46861=DIRECTION('',(0.150042296859641,0.,-0.988679578606276));
#46862=DIRECTION('',(0.931242779705752,0.,-0.364399348580517));
#46863=DIRECTION('',(0.781200482846104,0.,0.624280230025758));
#46864=DIRECTION('',(-0.150042296859647,0.,0.988679578606275));
#46865=DIRECTION('',(-0.931242779705751,0.,0.364399348580519));
#46866=DIRECTION('',(-0.781200482846105,0.,-0.624280230025758));
#46867=DIRECTION('',(0.150042296859641,0.,-0.988679578606276));
#46868=DIRECTION('',(0.931242779705752,0.,-0.364399348580517));
#46869=DIRECTION('',(0.781200482846104,0.,0.624280230025758));
#46870=DIRECTION('',(-0.150042296859647,0.,0.988679578606275));
#46871=DIRECTION('',(-0.931242779705751,0.,0.364399348580519));
#46872=DIRECTION('',(-0.781200482846105,0.,-0.624280230025758));
#46873=DIRECTION('',(0.150042296859641,0.,-0.988679578606276));
#46874=DIRECTION('',(0.931242779705752,0.,-0.364399348580517));
#46875=DIRECTION('',(0.781200482846104,0.,0.624280230025758));
#46876=DIRECTION('',(-0.150042296859647,0.,0.988679578606275));
#46877=DIRECTION('',(-0.931242779705751,0.,0.364399348580519));
#46878=DIRECTION('',(-0.781200482846105,0.,-0.624280230025758));
#46879=DIRECTION('',(0.150042296859641,0.,-0.988679578606276));
#46880=DIRECTION('',(0.931242779705752,0.,-0.364399348580517));
#46881=DIRECTION('',(0.781200482846104,0.,0.624280230025758));
#46882=DIRECTION('',(-0.150042296859647,0.,0.988679578606275));
#46883=DIRECTION('',(-0.931242779705751,0.,0.364399348580519));
#46884=DIRECTION('',(-0.781200482846105,0.,-0.624280230025758));
#46885=DIRECTION('',(0.150042296859641,0.,-0.988679578606276));
#46886=DIRECTION('',(0.931242779705752,0.,-0.364399348580517));
#46887=DIRECTION('',(0.781200482846104,0.,0.624280230025758));
#46888=DIRECTION('',(-0.150042296859647,0.,0.988679578606275));
#46889=DIRECTION('',(-0.931242779705751,0.,0.364399348580519));
#46890=DIRECTION('',(-0.781200482846105,0.,-0.624280230025758));
#46891=DIRECTION('',(0.150042296859641,0.,-0.988679578606276));
#46892=DIRECTION('',(0.931242779705752,0.,-0.364399348580517));
#46893=DIRECTION('',(0.781200482846104,0.,0.624280230025758));
#46894=DIRECTION('',(-0.150042296859647,0.,0.988679578606275));
#46895=DIRECTION('',(-0.931242779705751,0.,0.364399348580519));
#46896=DIRECTION('',(-0.781200482846105,0.,-0.624280230025758));
#46897=DIRECTION('',(0.150042296859641,0.,-0.988679578606276));
#46898=DIRECTION('',(0.931242779705752,0.,-0.364399348580517));
#46899=DIRECTION('',(0.781200482846104,0.,0.624280230025758));
#46900=DIRECTION('',(-0.150042296859647,0.,0.988679578606275));
#46901=DIRECTION('',(-0.931242779705751,0.,0.364399348580519));
#46902=DIRECTION('',(-0.781200482846105,0.,-0.624280230025758));
#46903=DIRECTION('',(0.150042296859641,0.,-0.988679578606276));
#46904=DIRECTION('',(0.931242779705752,0.,-0.364399348580517));
#46905=DIRECTION('',(0.781200482846104,0.,0.624280230025758));
#46906=DIRECTION('',(-0.150042296859647,0.,0.988679578606275));
#46907=DIRECTION('',(-0.931242779705751,0.,0.364399348580519));
#46908=DIRECTION('',(-0.781200482846105,0.,-0.624280230025758));
#46909=DIRECTION('',(0.150042296859641,0.,-0.988679578606276));
#46910=DIRECTION('',(0.931242779705752,0.,-0.364399348580517));
#46911=DIRECTION('',(0.781200482846104,0.,0.624280230025758));
#46912=DIRECTION('',(-0.150042296859647,0.,0.988679578606275));
#46913=DIRECTION('',(-0.931242779705751,0.,0.364399348580519));
#46914=DIRECTION('',(-0.781200482846105,0.,-0.624280230025758));
#46915=DIRECTION('',(0.150042296859641,0.,-0.988679578606276));
#46916=DIRECTION('',(0.931242779705752,0.,-0.364399348580517));
#46917=DIRECTION('',(0.781200482846104,0.,0.624280230025758));
#46918=DIRECTION('',(-0.150042296859647,0.,0.988679578606275));
#46919=DIRECTION('',(-0.931242779705751,0.,0.364399348580519));
#46920=DIRECTION('',(-0.781200482846105,0.,-0.624280230025758));
#46921=DIRECTION('',(0.150042296859641,0.,-0.988679578606276));
#46922=DIRECTION('',(0.931242779705752,0.,-0.364399348580517));
#46923=DIRECTION('',(0.781200482846104,0.,0.624280230025758));
#46924=DIRECTION('',(-0.150042296859647,0.,0.988679578606275));
#46925=DIRECTION('',(-0.931242779705751,0.,0.364399348580519));
#46926=DIRECTION('',(-0.781200482846105,0.,-0.624280230025758));
#46927=DIRECTION('',(0.150042296859641,0.,-0.988679578606276));
#46928=DIRECTION('',(0.931242779705752,0.,-0.364399348580517));
#46929=DIRECTION('',(0.781200482846104,0.,0.624280230025758));
#46930=DIRECTION('',(-0.150042296859647,0.,0.988679578606275));
#46931=DIRECTION('',(-0.931242779705751,0.,0.364399348580519));
#46932=DIRECTION('',(-0.781200482846105,0.,-0.624280230025758));
#46933=DIRECTION('',(0.150042296859641,0.,-0.988679578606276));
#46934=DIRECTION('',(0.931242779705752,0.,-0.364399348580517));
#46935=DIRECTION('',(0.781200482846104,0.,0.624280230025758));
#46936=DIRECTION('',(-0.150042296859647,0.,0.988679578606275));
#46937=DIRECTION('',(-0.931242779705751,0.,0.364399348580519));
#46938=DIRECTION('',(-0.781200482846105,0.,-0.624280230025758));
#46939=DIRECTION('',(0.150042296859641,0.,-0.988679578606276));
#46940=DIRECTION('',(0.931242779705752,0.,-0.364399348580517));
#46941=DIRECTION('',(0.781200482846104,0.,0.624280230025758));
#46942=DIRECTION('',(-0.150042296859647,0.,0.988679578606275));
#46943=DIRECTION('',(-0.931242779705751,0.,0.364399348580519));
#46944=DIRECTION('',(-0.781200482846105,0.,-0.624280230025758));
#46945=DIRECTION('',(0.150042296859641,0.,-0.988679578606276));
#46946=DIRECTION('',(0.931242779705752,0.,-0.364399348580517));
#46947=DIRECTION('',(0.781200482846104,0.,0.624280230025758));
#46948=DIRECTION('',(-0.150042296859647,0.,0.988679578606275));
#46949=DIRECTION('',(-0.931242779705751,0.,0.364399348580519));
#46950=DIRECTION('',(-0.781200482846105,0.,-0.624280230025758));
#46951=DIRECTION('',(0.150042296859641,0.,-0.988679578606276));
#46952=DIRECTION('',(0.931242779705752,0.,-0.364399348580517));
#46953=DIRECTION('',(0.781200482846104,0.,0.624280230025758));
#46954=DIRECTION('',(-0.150042296859647,0.,0.988679578606275));
#46955=DIRECTION('',(-0.931242779705751,0.,0.364399348580519));
#46956=DIRECTION('',(-0.781200482846105,0.,-0.624280230025758));
#46957=DIRECTION('',(0.150042296859641,0.,-0.988679578606276));
#46958=DIRECTION('',(0.931242779705752,0.,-0.364399348580517));
#46959=DIRECTION('',(0.781200482846104,0.,0.624280230025758));
#46960=DIRECTION('',(-0.150042296859647,0.,0.988679578606275));
#46961=DIRECTION('',(-0.931242779705751,0.,0.364399348580519));
#46962=DIRECTION('',(-0.781200482846105,0.,-0.624280230025758));
#46963=DIRECTION('',(0.150042296859641,0.,-0.988679578606276));
#46964=DIRECTION('',(0.931242779705752,0.,-0.364399348580517));
#46965=DIRECTION('',(0.781200482846104,0.,0.624280230025758));
#46966=DIRECTION('',(-0.150042296859647,0.,0.988679578606275));
#46967=DIRECTION('',(-0.931242779705751,0.,0.364399348580519));
#46968=DIRECTION('',(-0.781200482846105,0.,-0.624280230025758));
#46969=DIRECTION('',(0.150042296859641,0.,-0.988679578606276));
#46970=DIRECTION('',(0.931242779705752,0.,-0.364399348580517));
#46971=DIRECTION('',(0.781200482846104,0.,0.624280230025758));
#46972=DIRECTION('',(-0.150042296859647,0.,0.988679578606275));
#46973=DIRECTION('',(-0.931242779705751,0.,0.364399348580519));
#46974=DIRECTION('',(-0.781200482846105,0.,-0.624280230025758));
#46975=DIRECTION('',(0.150042296859641,0.,-0.988679578606276));
#46976=DIRECTION('',(0.931242779705752,0.,-0.364399348580517));
#46977=DIRECTION('',(0.781200482846104,0.,0.624280230025758));
#46978=DIRECTION('',(-0.150042296859647,0.,0.988679578606275));
#46979=DIRECTION('',(-0.931242779705751,0.,0.364399348580519));
#46980=DIRECTION('',(-0.781200482846105,0.,-0.624280230025758));
#46981=DIRECTION('',(0.150042296859641,0.,-0.988679578606276));
#46982=DIRECTION('',(0.931242779705752,0.,-0.364399348580517));
#46983=DIRECTION('',(0.781200482846104,0.,0.624280230025758));
#46984=DIRECTION('',(-0.150042296859647,0.,0.988679578606275));
#46985=DIRECTION('',(-0.931242779705751,0.,0.364399348580519));
#46986=DIRECTION('',(-0.781200482846105,0.,-0.624280230025758));
#46987=DIRECTION('',(0.150042296859641,0.,-0.988679578606276));
#46988=DIRECTION('',(0.931242779705752,0.,-0.364399348580517));
#46989=DIRECTION('',(0.781200482846104,0.,0.624280230025758));
#46990=DIRECTION('',(-0.150042296859647,0.,0.988679578606275));
#46991=DIRECTION('',(-0.931242779705751,0.,0.364399348580519));
#46992=DIRECTION('',(-0.781200482846105,0.,-0.624280230025758));
#46993=DIRECTION('',(0.150042296859641,0.,-0.988679578606276));
#46994=DIRECTION('',(0.931242779705752,0.,-0.364399348580517));
#46995=DIRECTION('',(0.781200482846104,0.,0.624280230025758));
#46996=DIRECTION('',(-0.150042296859647,0.,0.988679578606275));
#46997=DIRECTION('',(-0.931242779705751,0.,0.364399348580519));
#46998=DIRECTION('',(-0.781200482846105,0.,-0.624280230025758));
#46999=DIRECTION('',(0.150042296859641,0.,-0.988679578606276));
#47000=DIRECTION('',(0.931242779705752,0.,-0.364399348580517));
#47001=DIRECTION('',(0.781200482846104,0.,0.624280230025758));
#47002=DIRECTION('',(-0.150042296859647,0.,0.988679578606275));
#47003=DIRECTION('',(-0.931242779705751,0.,0.364399348580519));
#47004=DIRECTION('',(-0.781200482846105,0.,-0.624280230025758));
#47005=DIRECTION('',(0.150042296859641,0.,-0.988679578606276));
#47006=DIRECTION('',(0.931242779705752,0.,-0.364399348580517));
#47007=DIRECTION('',(0.781200482846104,0.,0.624280230025758));
#47008=DIRECTION('',(-0.150042296859647,0.,0.988679578606275));
#47009=DIRECTION('',(-0.931242779705751,0.,0.364399348580519));
#47010=DIRECTION('',(-0.781200482846105,0.,-0.624280230025758));
#47011=DIRECTION('',(0.150042296859641,0.,-0.988679578606276));
#47012=DIRECTION('',(0.931242779705752,0.,-0.364399348580517));
#47013=DIRECTION('',(0.781200482846104,0.,0.624280230025758));
#47014=DIRECTION('',(-0.150042296859647,0.,0.988679578606275));
#47015=DIRECTION('',(-0.931242779705751,0.,0.364399348580519));
#47016=DIRECTION('',(-0.781200482846105,0.,-0.624280230025758));
#47017=DIRECTION('',(0.150042296859641,0.,-0.988679578606276));
#47018=DIRECTION('',(0.931242779705752,0.,-0.364399348580517));
#47019=DIRECTION('',(0.781200482846104,0.,0.624280230025758));
#47020=DIRECTION('',(-0.150042296859647,0.,0.988679578606275));
#47021=DIRECTION('',(-0.931242779705751,0.,0.364399348580519));
#47022=DIRECTION('',(-0.781200482846105,0.,-0.624280230025758));
#47023=DIRECTION('',(0.150042296859641,0.,-0.988679578606276));
#47024=DIRECTION('',(0.931242779705752,0.,-0.364399348580517));
#47025=DIRECTION('',(0.781200482846104,0.,0.624280230025758));
#47026=DIRECTION('',(-0.150042296859647,0.,0.988679578606275));
#47027=DIRECTION('',(-0.931242779705751,0.,0.364399348580519));
#47028=DIRECTION('',(-0.781200482846105,0.,-0.624280230025758));
#47029=DIRECTION('',(0.150042296859641,0.,-0.988679578606276));
#47030=DIRECTION('',(0.931242779705752,0.,-0.364399348580517));
#47031=DIRECTION('',(0.781200482846104,0.,0.624280230025758));
#47032=DIRECTION('',(-0.150042296859647,0.,0.988679578606275));
#47033=DIRECTION('',(-0.931242779705751,0.,0.364399348580519));
#47034=DIRECTION('',(-0.781200482846105,0.,-0.624280230025758));
#47035=DIRECTION('',(0.150042296859641,0.,-0.988679578606276));
#47036=DIRECTION('',(0.931242779705752,0.,-0.364399348580517));
#47037=DIRECTION('',(0.781200482846104,0.,0.624280230025758));
#47038=DIRECTION('',(-0.150042296859647,0.,0.988679578606275));
#47039=DIRECTION('',(-0.931242779705751,0.,0.364399348580519));
#47040=DIRECTION('',(-0.781200482846105,0.,-0.624280230025758));
#47041=DIRECTION('',(0.150042296859641,0.,-0.988679578606276));
#47042=DIRECTION('',(0.931242779705752,0.,-0.364399348580517));
#47043=DIRECTION('',(0.781200482846104,0.,0.624280230025758));
#47044=DIRECTION('',(-0.150042296859647,0.,0.988679578606275));
#47045=DIRECTION('',(-0.931242779705751,0.,0.364399348580519));
#47046=DIRECTION('',(-0.781200482846105,0.,-0.624280230025758));
#47047=DIRECTION('',(0.150042296859641,0.,-0.988679578606276));
#47048=DIRECTION('',(0.931242779705752,0.,-0.364399348580517));
#47049=DIRECTION('',(0.781200482846104,0.,0.624280230025758));
#47050=DIRECTION('',(-0.150042296859647,0.,0.988679578606275));
#47051=DIRECTION('',(-0.931242779705751,0.,0.364399348580519));
#47052=DIRECTION('',(-0.781200482846105,0.,-0.624280230025758));
#47053=DIRECTION('',(0.150042296859641,0.,-0.988679578606276));
#47054=DIRECTION('',(0.931242779705752,0.,-0.364399348580517));
#47055=DIRECTION('',(0.781200482846104,0.,0.624280230025758));
#47056=DIRECTION('',(-0.150042296859647,0.,0.988679578606275));
#47057=DIRECTION('',(-0.931242779705751,0.,0.364399348580519));
#47058=DIRECTION('',(-0.781200482846105,0.,-0.624280230025758));
#47059=DIRECTION('',(0.150042296859641,0.,-0.988679578606276));
#47060=DIRECTION('',(0.931242779705752,0.,-0.364399348580517));
#47061=DIRECTION('',(0.781200482846104,0.,0.624280230025758));
#47062=DIRECTION('',(-0.150042296859647,0.,0.988679578606275));
#47063=DIRECTION('',(-0.931242779705751,0.,0.364399348580519));
#47064=DIRECTION('',(-0.781200482846105,0.,-0.624280230025758));
#47065=DIRECTION('',(0.150042296859641,0.,-0.988679578606276));
#47066=DIRECTION('',(0.931242779705752,0.,-0.364399348580517));
#47067=DIRECTION('',(0.781200482846104,0.,0.624280230025758));
#47068=DIRECTION('',(-0.150042296859647,0.,0.988679578606275));
#47069=DIRECTION('',(-0.931242779705751,0.,0.364399348580519));
#47070=DIRECTION('',(-0.781200482846105,0.,-0.624280230025758));
#47071=DIRECTION('',(0.150042296859641,0.,-0.988679578606276));
#47072=DIRECTION('',(0.931242779705752,0.,-0.364399348580517));
#47073=DIRECTION('',(0.781200482846104,0.,0.624280230025758));
#47074=DIRECTION('',(-0.150042296859647,0.,0.988679578606275));
#47075=DIRECTION('',(-0.931242779705751,0.,0.364399348580519));
#47076=DIRECTION('',(-0.781200482846105,0.,-0.624280230025758));
#47077=DIRECTION('',(0.150042296859641,0.,-0.988679578606276));
#47078=DIRECTION('',(0.931242779705752,0.,-0.364399348580517));
#47079=DIRECTION('',(0.781200482846104,0.,0.624280230025758));
#47080=DIRECTION('',(-0.150042296859647,0.,0.988679578606275));
#47081=DIRECTION('',(-0.931242779705751,0.,0.364399348580519));
#47082=DIRECTION('',(-0.781200482846105,0.,-0.624280230025758));
#47083=DIRECTION('',(0.150042296859641,0.,-0.988679578606276));
#47084=DIRECTION('',(0.931242779705752,0.,-0.364399348580517));
#47085=DIRECTION('',(0.781200482846104,0.,0.624280230025758));
#47086=DIRECTION('',(-0.150042296859647,0.,0.988679578606275));
#47087=DIRECTION('',(-0.931242779705751,0.,0.364399348580519));
#47088=DIRECTION('',(-0.781200482846105,0.,-0.624280230025758));
#47089=DIRECTION('',(0.150042296859641,0.,-0.988679578606276));
#47090=DIRECTION('',(0.931242779705752,0.,-0.364399348580517));
#47091=DIRECTION('',(0.781200482846104,0.,0.624280230025758));
#47092=DIRECTION('',(-0.150042296859647,0.,0.988679578606275));
#47093=DIRECTION('',(-0.931242779705751,0.,0.364399348580519));
#47094=DIRECTION('',(-0.781200482846105,0.,-0.624280230025758));
#47095=DIRECTION('',(0.150042296859641,0.,-0.988679578606276));
#47096=DIRECTION('',(0.931242779705752,0.,-0.364399348580517));
#47097=DIRECTION('',(0.781200482846104,0.,0.624280230025758));
#47098=DIRECTION('',(-0.150042296859647,0.,0.988679578606275));
#47099=DIRECTION('',(-0.931242779705751,0.,0.364399348580519));
#47100=DIRECTION('',(-0.781200482846105,0.,-0.624280230025758));
#47101=DIRECTION('',(0.150042296859641,0.,-0.988679578606276));
#47102=DIRECTION('',(0.931242779705752,0.,-0.364399348580517));
#47103=DIRECTION('',(0.781200482846104,0.,0.624280230025758));
#47104=DIRECTION('',(-0.150042296859647,0.,0.988679578606275));
#47105=DIRECTION('',(-0.931242779705751,0.,0.364399348580519));
#47106=DIRECTION('',(-0.781200482846105,0.,-0.624280230025758));
#47107=DIRECTION('',(0.150042296859641,0.,-0.988679578606276));
#47108=DIRECTION('',(0.931242779705752,0.,-0.364399348580517));
#47109=DIRECTION('',(0.781200482846104,0.,0.624280230025758));
#47110=DIRECTION('',(-0.150042296859647,0.,0.988679578606275));
#47111=DIRECTION('',(-0.931242779705751,0.,0.364399348580519));
#47112=DIRECTION('',(-0.781200482846105,0.,-0.624280230025758));
#47113=DIRECTION('',(0.150042296859641,0.,-0.988679578606276));
#47114=DIRECTION('',(0.931242779705752,0.,-0.364399348580517));
#47115=DIRECTION('',(0.781200482846104,0.,0.624280230025758));
#47116=DIRECTION('',(-0.150042296859647,0.,0.988679578606275));
#47117=DIRECTION('',(-0.931242779705751,0.,0.364399348580519));
#47118=DIRECTION('',(-0.781200482846105,0.,-0.624280230025758));
#47119=DIRECTION('',(0.150042296859641,0.,-0.988679578606276));
#47120=DIRECTION('',(0.931242779705752,0.,-0.364399348580517));
#47121=DIRECTION('',(0.781200482846104,0.,0.624280230025758));
#47122=DIRECTION('',(-0.150042296859647,0.,0.988679578606275));
#47123=DIRECTION('',(-0.931242779705751,0.,0.364399348580519));
#47124=DIRECTION('',(-0.781200482846105,0.,-0.624280230025758));
#47125=DIRECTION('',(0.150042296859641,0.,-0.988679578606276));
#47126=DIRECTION('',(0.931242779705752,0.,-0.364399348580517));
#47127=DIRECTION('',(0.781200482846104,0.,0.624280230025758));
#47128=DIRECTION('',(-0.150042296859647,0.,0.988679578606275));
#47129=DIRECTION('',(-0.931242779705751,0.,0.364399348580519));
#47130=DIRECTION('',(-0.781200482846105,0.,-0.624280230025758));
#47131=DIRECTION('',(0.150042296859641,0.,-0.988679578606276));
#47132=DIRECTION('',(0.931242779705752,0.,-0.364399348580517));
#47133=DIRECTION('',(0.781200482846104,0.,0.624280230025758));
#47134=DIRECTION('',(-0.150042296859647,0.,0.988679578606275));
#47135=DIRECTION('',(-0.931242779705751,0.,0.364399348580519));
#47136=DIRECTION('',(-0.781200482846105,0.,-0.624280230025758));
#47137=DIRECTION('',(0.150042296859641,0.,-0.988679578606276));
#47138=DIRECTION('',(0.931242779705752,0.,-0.364399348580517));
#47139=DIRECTION('',(0.781200482846104,0.,0.624280230025758));
#47140=DIRECTION('',(-0.150042296859647,0.,0.988679578606275));
#47141=DIRECTION('',(-0.931242779705751,0.,0.364399348580519));
#47142=DIRECTION('',(-0.781200482846105,0.,-0.624280230025758));
#47143=DIRECTION('',(0.150042296859641,0.,-0.988679578606276));
#47144=DIRECTION('',(0.931242779705752,0.,-0.364399348580517));
#47145=DIRECTION('',(0.781200482846104,0.,0.624280230025758));
#47146=DIRECTION('',(-0.150042296859647,0.,0.988679578606275));
#47147=DIRECTION('',(-0.931242779705751,0.,0.364399348580519));
#47148=DIRECTION('',(-0.781200482846105,0.,-0.624280230025758));
#47149=DIRECTION('',(0.150042296859641,0.,-0.988679578606276));
#47150=DIRECTION('',(0.931242779705752,0.,-0.364399348580517));
#47151=DIRECTION('',(0.781200482846104,0.,0.624280230025758));
#47152=DIRECTION('',(-0.150042296859647,0.,0.988679578606275));
#47153=DIRECTION('',(-0.931242779705751,0.,0.364399348580519));
#47154=DIRECTION('',(-0.781200482846105,0.,-0.624280230025758));
#47155=DIRECTION('',(0.150042296859641,0.,-0.988679578606276));
#47156=DIRECTION('',(0.931242779705752,0.,-0.364399348580517));
#47157=DIRECTION('',(0.781200482846104,0.,0.624280230025758));
#47158=DIRECTION('',(-0.150042296859647,0.,0.988679578606275));
#47159=DIRECTION('',(-0.931242779705751,0.,0.364399348580519));
#47160=DIRECTION('',(-0.781200482846105,0.,-0.624280230025758));
#47161=DIRECTION('',(0.150042296859641,0.,-0.988679578606276));
#47162=DIRECTION('',(0.931242779705752,0.,-0.364399348580517));
#47163=DIRECTION('',(0.781200482846104,0.,0.624280230025758));
#47164=DIRECTION('',(-0.150042296859647,0.,0.988679578606275));
#47165=DIRECTION('',(-0.931242779705751,0.,0.364399348580519));
#47166=DIRECTION('',(-0.781200482846105,0.,-0.624280230025758));
#47167=DIRECTION('',(0.150042296859641,0.,-0.988679578606276));
#47168=DIRECTION('',(0.931242779705752,0.,-0.364399348580517));
#47169=DIRECTION('',(0.781200482846104,0.,0.624280230025758));
#47170=DIRECTION('',(-0.150042296859647,0.,0.988679578606275));
#47171=DIRECTION('',(-0.931242779705751,0.,0.364399348580519));
#47172=DIRECTION('',(-0.781200482846105,0.,-0.624280230025758));
#47173=DIRECTION('',(0.150042296859641,0.,-0.988679578606276));
#47174=DIRECTION('',(0.931242779705752,0.,-0.364399348580517));
#47175=DIRECTION('',(0.781200482846104,0.,0.624280230025758));
#47176=DIRECTION('',(-0.150042296859647,0.,0.988679578606275));
#47177=DIRECTION('',(-0.931242779705751,0.,0.364399348580519));
#47178=DIRECTION('',(-0.781200482846105,0.,-0.624280230025758));
#47179=DIRECTION('',(0.150042296859641,0.,-0.988679578606276));
#47180=DIRECTION('',(0.931242779705752,0.,-0.364399348580517));
#47181=DIRECTION('',(0.781200482846104,0.,0.624280230025758));
#47182=DIRECTION('',(-0.150042296859647,0.,0.988679578606275));
#47183=DIRECTION('',(-0.931242779705751,0.,0.364399348580519));
#47184=DIRECTION('',(-0.781200482846105,0.,-0.624280230025758));
#47185=DIRECTION('',(0.150042296859641,0.,-0.988679578606276));
#47186=DIRECTION('',(0.931242779705752,0.,-0.364399348580517));
#47187=DIRECTION('',(0.781200482846104,0.,0.624280230025758));
#47188=DIRECTION('',(-0.150042296859647,0.,0.988679578606275));
#47189=DIRECTION('',(-0.931242779705751,0.,0.364399348580519));
#47190=DIRECTION('',(-0.781200482846105,0.,-0.624280230025758));
#47191=DIRECTION('',(0.150042296859641,0.,-0.988679578606276));
#47192=DIRECTION('',(0.931242779705752,0.,-0.364399348580517));
#47193=DIRECTION('',(0.781200482846104,0.,0.624280230025758));
#47194=DIRECTION('',(-0.150042296859647,0.,0.988679578606275));
#47195=DIRECTION('',(-0.931242779705751,0.,0.364399348580519));
#47196=DIRECTION('',(-0.781200482846105,0.,-0.624280230025758));
#47197=DIRECTION('',(0.150042296859641,0.,-0.988679578606276));
#47198=DIRECTION('',(0.931242779705752,0.,-0.364399348580517));
#47199=DIRECTION('',(0.781200482846104,0.,0.624280230025758));
#47200=DIRECTION('',(-0.150042296859647,0.,0.988679578606275));
#47201=DIRECTION('',(-0.931242779705751,0.,0.364399348580519));
#47202=DIRECTION('',(-0.781200482846105,0.,-0.624280230025758));
#47203=DIRECTION('',(0.150042296859641,0.,-0.988679578606276));
#47204=DIRECTION('',(0.931242779705752,0.,-0.364399348580517));
#47205=DIRECTION('',(0.781200482846104,0.,0.624280230025758));
#47206=DIRECTION('',(-0.150042296859647,0.,0.988679578606275));
#47207=DIRECTION('',(-0.931242779705751,0.,0.364399348580519));
#47208=DIRECTION('',(-0.781200482846105,0.,-0.624280230025758));
#47209=DIRECTION('',(0.150042296859641,0.,-0.988679578606276));
#47210=DIRECTION('',(0.931242779705752,0.,-0.364399348580517));
#47211=DIRECTION('',(0.781200482846104,0.,0.624280230025758));
#47212=DIRECTION('',(-0.150042296859647,0.,0.988679578606275));
#47213=DIRECTION('',(-0.931242779705751,0.,0.364399348580519));
#47214=DIRECTION('',(-0.781200482846105,0.,-0.624280230025758));
#47215=DIRECTION('',(0.150042296859641,0.,-0.988679578606276));
#47216=DIRECTION('',(0.931242779705752,0.,-0.364399348580517));
#47217=DIRECTION('',(0.781200482846104,0.,0.624280230025758));
#47218=DIRECTION('',(-0.150042296859647,0.,0.988679578606275));
#47219=DIRECTION('',(-0.931242779705751,0.,0.364399348580519));
#47220=DIRECTION('',(-0.781200482846105,0.,-0.624280230025758));
#47221=DIRECTION('',(0.150042296859641,0.,-0.988679578606276));
#47222=DIRECTION('',(0.931242779705752,0.,-0.364399348580517));
#47223=DIRECTION('',(0.781200482846104,0.,0.624280230025758));
#47224=DIRECTION('',(-0.150042296859647,0.,0.988679578606275));
#47225=DIRECTION('',(-0.931242779705751,0.,0.364399348580519));
#47226=DIRECTION('',(-0.781200482846105,0.,-0.624280230025758));
#47227=DIRECTION('',(0.150042296859641,0.,-0.988679578606276));
#47228=DIRECTION('',(0.931242779705752,0.,-0.364399348580517));
#47229=DIRECTION('',(0.781200482846104,0.,0.624280230025758));
#47230=DIRECTION('',(-0.150042296859647,0.,0.988679578606275));
#47231=DIRECTION('',(-0.931242779705751,0.,0.364399348580519));
#47232=DIRECTION('',(-0.781200482846105,0.,-0.624280230025758));
#47233=DIRECTION('',(0.150042296859641,0.,-0.988679578606276));
#47234=DIRECTION('',(0.931242779705752,0.,-0.364399348580517));
#47235=DIRECTION('',(0.781200482846104,0.,0.624280230025758));
#47236=DIRECTION('',(-0.150042296859647,0.,0.988679578606275));
#47237=DIRECTION('',(-0.931242779705751,0.,0.364399348580519));
#47238=DIRECTION('',(-0.781200482846105,0.,-0.624280230025758));
#47239=DIRECTION('',(0.150042296859641,0.,-0.988679578606276));
#47240=DIRECTION('',(0.931242779705752,0.,-0.364399348580517));
#47241=DIRECTION('',(0.781200482846104,0.,0.624280230025758));
#47242=DIRECTION('',(-0.150042296859647,0.,0.988679578606275));
#47243=DIRECTION('',(-0.931242779705751,0.,0.364399348580519));
#47244=DIRECTION('',(-0.781200482846105,0.,-0.624280230025758));
#47245=DIRECTION('',(0.150042296859641,0.,-0.988679578606276));
#47246=DIRECTION('',(0.931242779705752,0.,-0.364399348580517));
#47247=DIRECTION('',(0.781200482846104,0.,0.624280230025758));
#47248=DIRECTION('',(-0.150042296859647,0.,0.988679578606275));
#47249=DIRECTION('',(-0.931242779705751,0.,0.364399348580519));
#47250=DIRECTION('',(-0.781200482846105,0.,-0.624280230025758));
#47251=DIRECTION('',(0.150042296859641,0.,-0.988679578606276));
#47252=DIRECTION('',(0.931242779705752,0.,-0.364399348580517));
#47253=DIRECTION('',(0.781200482846104,0.,0.624280230025758));
#47254=DIRECTION('',(-0.150042296859647,0.,0.988679578606275));
#47255=DIRECTION('',(-0.931242779705751,0.,0.364399348580519));
#47256=DIRECTION('',(-0.781200482846105,0.,-0.624280230025758));
#47257=DIRECTION('',(0.150042296859641,0.,-0.988679578606276));
#47258=DIRECTION('',(0.931242779705752,0.,-0.364399348580517));
#47259=DIRECTION('',(0.781200482846104,0.,0.624280230025758));
#47260=DIRECTION('',(-0.150042296859647,0.,0.988679578606275));
#47261=DIRECTION('',(-0.931242779705751,0.,0.364399348580519));
#47262=DIRECTION('',(-0.781200482846105,0.,-0.624280230025758));
#47263=DIRECTION('',(0.150042296859641,0.,-0.988679578606276));
#47264=DIRECTION('',(0.931242779705752,0.,-0.364399348580517));
#47265=DIRECTION('',(0.781200482846104,0.,0.624280230025758));
#47266=DIRECTION('',(-0.150042296859647,0.,0.988679578606275));
#47267=DIRECTION('',(-0.931242779705751,0.,0.364399348580519));
#47268=DIRECTION('',(-0.781200482846105,0.,-0.624280230025758));
#47269=DIRECTION('',(0.150042296859641,0.,-0.988679578606276));
#47270=DIRECTION('',(0.931242779705752,0.,-0.364399348580517));
#47271=DIRECTION('',(0.781200482846104,0.,0.624280230025758));
#47272=DIRECTION('',(-0.150042296859647,0.,0.988679578606275));
#47273=DIRECTION('',(-0.931242779705751,0.,0.364399348580519));
#47274=DIRECTION('',(-0.781200482846105,0.,-0.624280230025758));
#47275=DIRECTION('',(0.150042296859641,0.,-0.988679578606276));
#47276=DIRECTION('',(0.931242779705752,0.,-0.364399348580517));
#47277=DIRECTION('',(0.781200482846104,0.,0.624280230025758));
#47278=DIRECTION('',(-0.150042296859647,0.,0.988679578606275));
#47279=DIRECTION('',(-0.931242779705751,0.,0.364399348580519));
#47280=DIRECTION('',(-0.781200482846105,0.,-0.624280230025758));
#47281=DIRECTION('',(0.150042296859641,0.,-0.988679578606276));
#47282=DIRECTION('',(0.931242779705752,0.,-0.364399348580517));
#47283=DIRECTION('',(0.781200482846104,0.,0.624280230025758));
#47284=DIRECTION('',(-0.150042296859647,0.,0.988679578606275));
#47285=DIRECTION('',(-0.931242779705751,0.,0.364399348580519));
#47286=DIRECTION('',(-0.781200482846105,0.,-0.624280230025758));
#47287=DIRECTION('',(0.150042296859641,0.,-0.988679578606276));
#47288=DIRECTION('',(0.931242779705752,0.,-0.364399348580517));
#47289=DIRECTION('',(0.781200482846104,0.,0.624280230025758));
#47290=DIRECTION('',(-0.150042296859647,0.,0.988679578606275));
#47291=DIRECTION('',(-0.931242779705751,0.,0.364399348580519));
#47292=DIRECTION('',(-0.781200482846105,0.,-0.624280230025758));
#47293=DIRECTION('',(0.150042296859641,0.,-0.988679578606276));
#47294=DIRECTION('',(0.931242779705752,0.,-0.364399348580517));
#47295=DIRECTION('',(0.781200482846104,0.,0.624280230025758));
#47296=DIRECTION('',(-0.150042296859647,0.,0.988679578606275));
#47297=DIRECTION('',(-0.931242779705751,0.,0.364399348580519));
#47298=DIRECTION('',(-0.781200482846105,0.,-0.624280230025758));
#47299=DIRECTION('',(0.150042296859641,0.,-0.988679578606276));
#47300=DIRECTION('',(0.931242779705752,0.,-0.364399348580517));
#47301=DIRECTION('',(0.781200482846104,0.,0.624280230025758));
#47302=DIRECTION('',(-0.150042296859647,0.,0.988679578606275));
#47303=DIRECTION('',(-0.931242779705751,0.,0.364399348580519));
#47304=DIRECTION('',(-0.781200482846105,0.,-0.624280230025758));
#47305=DIRECTION('',(0.150042296859641,0.,-0.988679578606276));
#47306=DIRECTION('',(0.931242779705752,0.,-0.364399348580517));
#47307=DIRECTION('',(0.781200482846104,0.,0.624280230025758));
#47308=DIRECTION('',(-0.150042296859647,0.,0.988679578606275));
#47309=DIRECTION('',(-0.931242779705751,0.,0.364399348580519));
#47310=DIRECTION('',(-0.781200482846105,0.,-0.624280230025758));
#47311=DIRECTION('',(0.150042296859641,0.,-0.988679578606276));
#47312=DIRECTION('',(0.931242779705752,0.,-0.364399348580517));
#47313=DIRECTION('',(0.781200482846104,0.,0.624280230025758));
#47314=DIRECTION('',(-0.150042296859647,0.,0.988679578606275));
#47315=DIRECTION('',(-0.931242779705751,0.,0.364399348580519));
#47316=DIRECTION('',(-0.781200482846105,0.,-0.624280230025758));
#47317=DIRECTION('',(0.150042296859641,0.,-0.988679578606276));
#47318=DIRECTION('',(0.931242779705752,0.,-0.364399348580517));
#47319=DIRECTION('',(0.781200482846104,0.,0.624280230025758));
#47320=DIRECTION('',(-0.150042296859647,0.,0.988679578606275));
#47321=DIRECTION('',(-0.931242779705751,0.,0.364399348580519));
#47322=DIRECTION('',(-0.781200482846105,0.,-0.624280230025758));
#47323=DIRECTION('',(0.150042296859641,0.,-0.988679578606276));
#47324=DIRECTION('',(0.931242779705752,0.,-0.364399348580517));
#47325=DIRECTION('',(0.781200482846104,0.,0.624280230025758));
#47326=DIRECTION('',(-0.150042296859647,0.,0.988679578606275));
#47327=DIRECTION('',(-0.931242779705751,0.,0.364399348580519));
#47328=DIRECTION('',(-0.781200482846105,0.,-0.624280230025758));
#47329=DIRECTION('',(0.150042296859641,0.,-0.988679578606276));
#47330=DIRECTION('',(0.931242779705752,0.,-0.364399348580517));
#47331=DIRECTION('',(0.781200482846104,0.,0.624280230025758));
#47332=DIRECTION('',(-0.150042296859647,0.,0.988679578606275));
#47333=DIRECTION('',(-0.931242779705751,0.,0.364399348580519));
#47334=DIRECTION('',(-0.781200482846105,0.,-0.624280230025758));
#47335=DIRECTION('',(0.150042296859641,0.,-0.988679578606276));
#47336=DIRECTION('',(0.931242779705752,0.,-0.364399348580517));
#47337=DIRECTION('',(0.781200482846104,0.,0.624280230025758));
#47338=DIRECTION('',(-0.150042296859647,0.,0.988679578606275));
#47339=DIRECTION('',(-0.931242779705751,0.,0.364399348580519));
#47340=DIRECTION('',(-0.781200482846105,0.,-0.624280230025758));
#47341=DIRECTION('',(0.150042296859641,0.,-0.988679578606276));
#47342=DIRECTION('',(0.931242779705752,0.,-0.364399348580517));
#47343=DIRECTION('',(0.781200482846104,0.,0.624280230025758));
#47344=DIRECTION('',(-0.150042296859647,0.,0.988679578606275));
#47345=DIRECTION('',(-0.931242779705751,0.,0.364399348580519));
#47346=DIRECTION('',(-0.781200482846105,0.,-0.624280230025758));
#47347=DIRECTION('',(0.150042296859641,0.,-0.988679578606276));
#47348=DIRECTION('',(0.931242779705752,0.,-0.364399348580517));
#47349=DIRECTION('',(0.781200482846104,0.,0.624280230025758));
#47350=DIRECTION('',(-0.150042296859647,0.,0.988679578606275));
#47351=DIRECTION('',(-0.931242779705751,0.,0.364399348580519));
#47352=DIRECTION('',(-0.781200482846105,0.,-0.624280230025758));
#47353=DIRECTION('',(0.150042296859641,0.,-0.988679578606276));
#47354=DIRECTION('',(0.931242779705752,0.,-0.364399348580517));
#47355=DIRECTION('',(0.781200482846104,0.,0.624280230025758));
#47356=DIRECTION('',(-0.150042296859647,0.,0.988679578606275));
#47357=DIRECTION('',(-0.931242779705751,0.,0.364399348580519));
#47358=DIRECTION('',(-0.781200482846105,0.,-0.624280230025758));
#47359=DIRECTION('',(0.150042296859641,0.,-0.988679578606276));
#47360=DIRECTION('',(0.931242779705752,0.,-0.364399348580517));
#47361=DIRECTION('',(0.781200482846104,0.,0.624280230025758));
#47362=DIRECTION('',(-0.150042296859647,0.,0.988679578606275));
#47363=DIRECTION('',(-0.931242779705751,0.,0.364399348580519));
#47364=DIRECTION('',(-0.781200482846105,0.,-0.624280230025758));
#47365=DIRECTION('',(0.150042296859641,0.,-0.988679578606276));
#47366=DIRECTION('',(0.931242779705752,0.,-0.364399348580517));
#47367=DIRECTION('',(0.781200482846104,0.,0.624280230025758));
#47368=DIRECTION('',(-0.150042296859647,0.,0.988679578606275));
#47369=DIRECTION('',(-0.931242779705751,0.,0.364399348580519));
#47370=DIRECTION('',(-0.781200482846105,0.,-0.624280230025758));
#47371=DIRECTION('',(0.150042296859641,0.,-0.988679578606276));
#47372=DIRECTION('',(0.931242779705752,0.,-0.364399348580517));
#47373=DIRECTION('',(0.781200482846104,0.,0.624280230025758));
#47374=DIRECTION('',(-0.150042296859647,0.,0.988679578606275));
#47375=DIRECTION('',(-0.931242779705751,0.,0.364399348580519));
#47376=DIRECTION('',(-0.781200482846105,0.,-0.624280230025758));
#47377=DIRECTION('',(0.150042296859641,0.,-0.988679578606276));
#47378=DIRECTION('',(0.931242779705752,0.,-0.364399348580517));
#47379=DIRECTION('',(0.781200482846104,0.,0.624280230025758));
#47380=DIRECTION('',(-0.150042296859647,0.,0.988679578606275));
#47381=DIRECTION('',(-0.931242779705751,0.,0.364399348580519));
#47382=DIRECTION('',(-0.781200482846105,0.,-0.624280230025758));
#47383=DIRECTION('',(0.150042296859641,0.,-0.988679578606276));
#47384=DIRECTION('',(0.931242779705752,0.,-0.364399348580517));
#47385=DIRECTION('',(0.781200482846104,0.,0.624280230025758));
#47386=DIRECTION('',(-0.150042296859647,0.,0.988679578606275));
#47387=DIRECTION('',(-0.931242779705751,0.,0.364399348580519));
#47388=DIRECTION('',(-0.781200482846105,0.,-0.624280230025758));
#47389=DIRECTION('',(0.150042296859641,0.,-0.988679578606276));
#47390=DIRECTION('',(0.931242779705752,0.,-0.364399348580517));
#47391=DIRECTION('',(0.781200482846104,0.,0.624280230025758));
#47392=DIRECTION('',(-0.150042296859647,0.,0.988679578606275));
#47393=DIRECTION('',(-0.931242779705751,0.,0.364399348580519));
#47394=DIRECTION('',(-0.781200482846105,0.,-0.624280230025758));
#47395=DIRECTION('',(0.150042296859641,0.,-0.988679578606276));
#47396=DIRECTION('',(0.931242779705752,0.,-0.364399348580517));
#47397=DIRECTION('',(0.781200482846104,0.,0.624280230025758));
#47398=DIRECTION('',(-0.150042296859647,0.,0.988679578606275));
#47399=DIRECTION('',(-0.931242779705751,0.,0.364399348580519));
#47400=DIRECTION('',(-0.781200482846105,0.,-0.624280230025758));
#47401=DIRECTION('',(0.150042296859641,0.,-0.988679578606276));
#47402=DIRECTION('',(0.931242779705752,0.,-0.364399348580517));
#47403=DIRECTION('',(0.781200482846104,0.,0.624280230025758));
#47404=DIRECTION('',(-0.150042296859647,0.,0.988679578606275));
#47405=DIRECTION('',(-0.931242779705751,0.,0.364399348580519));
#47406=DIRECTION('',(-0.781200482846105,0.,-0.624280230025758));
#47407=DIRECTION('',(0.150042296859641,0.,-0.988679578606276));
#47408=DIRECTION('',(0.931242779705752,0.,-0.364399348580517));
#47409=DIRECTION('',(0.781200482846104,0.,0.624280230025758));
#47410=DIRECTION('',(-0.150042296859647,0.,0.988679578606275));
#47411=DIRECTION('',(-0.931242779705751,0.,0.364399348580519));
#47412=DIRECTION('',(-0.781200482846105,0.,-0.624280230025758));
#47413=DIRECTION('',(0.150042296859641,0.,-0.988679578606276));
#47414=DIRECTION('',(0.931242779705752,0.,-0.364399348580517));
#47415=DIRECTION('',(0.781200482846104,0.,0.624280230025758));
#47416=DIRECTION('',(-0.150042296859647,0.,0.988679578606275));
#47417=DIRECTION('',(-0.931242779705751,0.,0.364399348580519));
#47418=DIRECTION('',(-0.781200482846105,0.,-0.624280230025758));
#47419=DIRECTION('',(0.150042296859641,0.,-0.988679578606276));
#47420=DIRECTION('',(0.931242779705752,0.,-0.364399348580517));
#47421=DIRECTION('',(0.781200482846104,0.,0.624280230025758));
#47422=DIRECTION('',(-0.150042296859647,0.,0.988679578606275));
#47423=DIRECTION('',(-0.931242779705751,0.,0.364399348580519));
#47424=DIRECTION('',(-0.781200482846105,0.,-0.624280230025758));
#47425=DIRECTION('',(0.150042296859641,0.,-0.988679578606276));
#47426=DIRECTION('',(0.931242779705752,0.,-0.364399348580517));
#47427=DIRECTION('',(0.781200482846104,0.,0.624280230025758));
#47428=DIRECTION('',(-0.150042296859647,0.,0.988679578606275));
#47429=DIRECTION('',(-0.931242779705751,0.,0.364399348580519));
#47430=DIRECTION('',(-0.781200482846105,0.,-0.624280230025758));
#47431=DIRECTION('',(0.150042296859641,0.,-0.988679578606276));
#47432=DIRECTION('',(0.931242779705752,0.,-0.364399348580517));
#47433=DIRECTION('',(0.781200482846104,0.,0.624280230025758));
#47434=DIRECTION('',(-0.150042296859647,0.,0.988679578606275));
#47435=DIRECTION('',(-0.931242779705751,0.,0.364399348580519));
#47436=DIRECTION('',(-0.781200482846105,0.,-0.624280230025758));
#47437=DIRECTION('',(0.150042296859641,0.,-0.988679578606276));
#47438=DIRECTION('',(0.931242779705752,0.,-0.364399348580517));
#47439=DIRECTION('',(0.781200482846104,0.,0.624280230025758));
#47440=DIRECTION('',(-0.150042296859647,0.,0.988679578606275));
#47441=DIRECTION('',(-0.931242779705751,0.,0.364399348580519));
#47442=DIRECTION('',(-0.781200482846105,0.,-0.624280230025758));
#47443=DIRECTION('',(0.150042296859641,0.,-0.988679578606276));
#47444=DIRECTION('',(0.931242779705752,0.,-0.364399348580517));
#47445=DIRECTION('',(0.781200482846104,0.,0.624280230025758));
#47446=DIRECTION('',(-0.150042296859647,0.,0.988679578606275));
#47447=DIRECTION('',(-0.931242779705751,0.,0.364399348580519));
#47448=DIRECTION('',(-0.781200482846105,0.,-0.624280230025758));
#47449=DIRECTION('',(0.150042296859641,0.,-0.988679578606276));
#47450=DIRECTION('',(0.931242779705752,0.,-0.364399348580517));
#47451=DIRECTION('',(0.781200482846104,0.,0.624280230025758));
#47452=DIRECTION('',(-0.150042296859647,0.,0.988679578606275));
#47453=DIRECTION('',(-0.931242779705751,0.,0.364399348580519));
#47454=DIRECTION('',(-0.781200482846105,0.,-0.624280230025758));
#47455=DIRECTION('',(0.150042296859641,0.,-0.988679578606276));
#47456=DIRECTION('',(0.931242779705752,0.,-0.364399348580517));
#47457=DIRECTION('',(0.781200482846104,0.,0.624280230025758));
#47458=DIRECTION('',(-0.150042296859647,0.,0.988679578606275));
#47459=DIRECTION('',(-0.931242779705751,0.,0.364399348580519));
#47460=DIRECTION('',(-0.781200482846105,0.,-0.624280230025758));
#47461=DIRECTION('',(0.150042296859641,0.,-0.988679578606276));
#47462=DIRECTION('',(0.931242779705752,0.,-0.364399348580517));
#47463=DIRECTION('',(0.781200482846104,0.,0.624280230025758));
#47464=DIRECTION('',(-0.150042296859647,0.,0.988679578606275));
#47465=DIRECTION('',(-0.931242779705751,0.,0.364399348580519));
#47466=DIRECTION('',(-0.781200482846105,0.,-0.624280230025758));
#47467=DIRECTION('',(0.150042296859641,0.,-0.988679578606276));
#47468=DIRECTION('',(0.931242779705752,0.,-0.364399348580517));
#47469=DIRECTION('',(0.781200482846104,0.,0.624280230025758));
#47470=DIRECTION('',(-0.150042296859647,0.,0.988679578606275));
#47471=DIRECTION('',(-0.931242779705751,0.,0.364399348580519));
#47472=DIRECTION('',(-0.781200482846105,0.,-0.624280230025758));
#47473=DIRECTION('',(0.150042296859641,0.,-0.988679578606276));
#47474=DIRECTION('',(0.931242779705752,0.,-0.364399348580517));
#47475=DIRECTION('',(0.781200482846104,0.,0.624280230025758));
#47476=DIRECTION('',(-0.150042296859647,0.,0.988679578606275));
#47477=DIRECTION('',(-0.931242779705751,0.,0.364399348580519));
#47478=DIRECTION('',(-0.781200482846105,0.,-0.624280230025758));
#47479=DIRECTION('',(0.150042296859641,0.,-0.988679578606276));
#47480=DIRECTION('',(0.931242779705752,0.,-0.364399348580517));
#47481=DIRECTION('',(0.781200482846104,0.,0.624280230025758));
#47482=DIRECTION('',(-0.150042296859647,0.,0.988679578606275));
#47483=DIRECTION('',(-0.931242779705751,0.,0.364399348580519));
#47484=DIRECTION('',(-0.781200482846105,0.,-0.624280230025758));
#47485=DIRECTION('',(0.150042296859641,0.,-0.988679578606276));
#47486=DIRECTION('',(0.931242779705752,0.,-0.364399348580517));
#47487=DIRECTION('',(0.781200482846104,0.,0.624280230025758));
#47488=DIRECTION('',(-0.150042296859647,0.,0.988679578606275));
#47489=DIRECTION('',(-0.931242779705751,0.,0.364399348580519));
#47490=DIRECTION('',(-0.781200482846105,0.,-0.624280230025758));
#47491=DIRECTION('',(0.150042296859641,0.,-0.988679578606276));
#47492=DIRECTION('',(0.931242779705752,0.,-0.364399348580517));
#47493=DIRECTION('',(0.781200482846104,0.,0.624280230025758));
#47494=DIRECTION('',(-0.150042296859647,0.,0.988679578606275));
#47495=DIRECTION('',(-0.931242779705751,0.,0.364399348580519));
#47496=DIRECTION('',(-0.781200482846105,0.,-0.624280230025758));
#47497=DIRECTION('',(0.150042296859641,0.,-0.988679578606276));
#47498=DIRECTION('',(0.931242779705752,0.,-0.364399348580517));
#47499=DIRECTION('',(0.781200482846104,0.,0.624280230025758));
#47500=DIRECTION('',(-0.150042296859647,0.,0.988679578606275));
#47501=DIRECTION('',(-0.931242779705751,0.,0.364399348580519));
#47502=DIRECTION('',(-0.781200482846105,0.,-0.624280230025758));
#47503=DIRECTION('',(0.150042296859641,0.,-0.988679578606276));
#47504=DIRECTION('',(0.931242779705752,0.,-0.364399348580517));
#47505=DIRECTION('',(0.781200482846104,0.,0.624280230025758));
#47506=DIRECTION('',(-0.150042296859647,0.,0.988679578606275));
#47507=DIRECTION('',(-0.931242779705751,0.,0.364399348580519));
#47508=DIRECTION('',(-0.781200482846105,0.,-0.624280230025758));
#47509=DIRECTION('',(0.150042296859641,0.,-0.988679578606276));
#47510=DIRECTION('',(0.931242779705752,0.,-0.364399348580517));
#47511=DIRECTION('',(0.781200482846104,0.,0.624280230025758));
#47512=DIRECTION('',(-0.150042296859647,0.,0.988679578606275));
#47513=DIRECTION('',(-0.931242779705751,0.,0.364399348580519));
#47514=DIRECTION('',(-0.781200482846105,0.,-0.624280230025758));
#47515=DIRECTION('',(0.150042296859641,0.,-0.988679578606276));
#47516=DIRECTION('',(0.931242779705752,0.,-0.364399348580517));
#47517=DIRECTION('',(0.781200482846104,0.,0.624280230025758));
#47518=DIRECTION('',(-0.150042296859647,0.,0.988679578606275));
#47519=DIRECTION('',(-0.931242779705751,0.,0.364399348580519));
#47520=DIRECTION('',(-0.781200482846105,0.,-0.624280230025758));
#47521=DIRECTION('',(0.150042296859641,0.,-0.988679578606276));
#47522=DIRECTION('',(0.931242779705752,0.,-0.364399348580517));
#47523=DIRECTION('',(0.781200482846104,0.,0.624280230025758));
#47524=DIRECTION('',(-0.150042296859647,0.,0.988679578606275));
#47525=DIRECTION('',(-0.931242779705751,0.,0.364399348580519));
#47526=DIRECTION('',(-0.781200482846105,0.,-0.624280230025758));
#47527=DIRECTION('',(0.150042296859641,0.,-0.988679578606276));
#47528=DIRECTION('',(0.931242779705752,0.,-0.364399348580517));
#47529=DIRECTION('',(0.781200482846104,0.,0.624280230025758));
#47530=DIRECTION('',(-0.150042296859647,0.,0.988679578606275));
#47531=DIRECTION('',(-0.931242779705751,0.,0.364399348580519));
#47532=DIRECTION('',(-0.781200482846105,0.,-0.624280230025758));
#47533=DIRECTION('',(0.150042296859641,0.,-0.988679578606276));
#47534=DIRECTION('',(0.931242779705752,0.,-0.364399348580517));
#47535=DIRECTION('',(0.781200482846104,0.,0.624280230025758));
#47536=DIRECTION('',(-0.150042296859647,0.,0.988679578606275));
#47537=DIRECTION('',(-0.931242779705751,0.,0.364399348580519));
#47538=DIRECTION('',(-0.781200482846105,0.,-0.624280230025758));
#47539=DIRECTION('',(0.150042296859641,0.,-0.988679578606276));
#47540=DIRECTION('',(0.931242779705752,0.,-0.364399348580517));
#47541=DIRECTION('',(0.781200482846104,0.,0.624280230025758));
#47542=DIRECTION('',(-0.150042296859647,0.,0.988679578606275));
#47543=DIRECTION('',(-0.931242779705751,0.,0.364399348580519));
#47544=DIRECTION('',(-0.781200482846105,0.,-0.624280230025758));
#47545=DIRECTION('',(0.150042296859641,0.,-0.988679578606276));
#47546=DIRECTION('',(0.931242779705752,0.,-0.364399348580517));
#47547=DIRECTION('',(0.781200482846104,0.,0.624280230025758));
#47548=DIRECTION('',(-0.150042296859647,0.,0.988679578606275));
#47549=DIRECTION('',(-0.931242779705751,0.,0.364399348580519));
#47550=DIRECTION('',(-0.781200482846105,0.,-0.624280230025758));
#47551=DIRECTION('',(0.150042296859641,0.,-0.988679578606276));
#47552=DIRECTION('',(0.931242779705752,0.,-0.364399348580517));
#47553=DIRECTION('',(0.781200482846104,0.,0.624280230025758));
#47554=DIRECTION('',(-0.150042296859647,0.,0.988679578606275));
#47555=DIRECTION('',(-0.931242779705751,0.,0.364399348580519));
#47556=DIRECTION('',(-0.781200482846105,0.,-0.624280230025758));
#47557=DIRECTION('',(0.150042296859641,0.,-0.988679578606276));
#47558=DIRECTION('',(0.931242779705752,0.,-0.364399348580517));
#47559=DIRECTION('',(0.781200482846104,0.,0.624280230025758));
#47560=DIRECTION('',(-0.150042296859647,0.,0.988679578606275));
#47561=DIRECTION('',(-0.931242779705751,0.,0.364399348580519));
#47562=DIRECTION('',(-0.781200482846105,0.,-0.624280230025758));
#47563=DIRECTION('',(0.150042296859641,0.,-0.988679578606276));
#47564=DIRECTION('',(0.931242779705752,0.,-0.364399348580517));
#47565=DIRECTION('',(0.781200482846104,0.,0.624280230025758));
#47566=DIRECTION('',(-0.150042296859647,0.,0.988679578606275));
#47567=DIRECTION('',(-0.931242779705751,0.,0.364399348580519));
#47568=DIRECTION('',(-0.781200482846105,0.,-0.624280230025758));
#47569=DIRECTION('',(0.150042296859641,0.,-0.988679578606276));
#47570=DIRECTION('',(0.931242779705752,0.,-0.364399348580517));
#47571=DIRECTION('',(0.781200482846104,0.,0.624280230025758));
#47572=DIRECTION('',(-0.150042296859647,0.,0.988679578606275));
#47573=DIRECTION('',(-0.931242779705751,0.,0.364399348580519));
#47574=DIRECTION('',(-0.781200482846105,0.,-0.624280230025758));
#47575=DIRECTION('',(0.150042296859641,0.,-0.988679578606276));
#47576=DIRECTION('',(0.931242779705752,0.,-0.364399348580517));
#47577=DIRECTION('',(0.781200482846104,0.,0.624280230025758));
#47578=DIRECTION('',(-0.150042296859647,0.,0.988679578606275));
#47579=DIRECTION('',(-0.931242779705751,0.,0.364399348580519));
#47580=DIRECTION('',(-0.781200482846105,0.,-0.624280230025758));
#47581=DIRECTION('',(0.150042296859641,0.,-0.988679578606276));
#47582=DIRECTION('',(0.931242779705752,0.,-0.364399348580517));
#47583=DIRECTION('',(0.781200482846104,0.,0.624280230025758));
#47584=DIRECTION('',(-0.150042296859647,0.,0.988679578606275));
#47585=DIRECTION('',(-0.931242779705751,0.,0.364399348580519));
#47586=DIRECTION('',(-0.781200482846105,0.,-0.624280230025758));
#47587=DIRECTION('',(0.150042296859641,0.,-0.988679578606276));
#47588=DIRECTION('',(0.931242779705752,0.,-0.364399348580517));
#47589=DIRECTION('',(0.781200482846104,0.,0.624280230025758));
#47590=DIRECTION('',(-0.150042296859647,0.,0.988679578606275));
#47591=DIRECTION('',(-0.931242779705751,0.,0.364399348580519));
#47592=DIRECTION('',(-0.781200482846105,0.,-0.624280230025758));
#47593=DIRECTION('',(0.150042296859641,0.,-0.988679578606276));
#47594=DIRECTION('',(0.931242779705752,0.,-0.364399348580517));
#47595=DIRECTION('',(0.781200482846104,0.,0.624280230025758));
#47596=DIRECTION('',(-0.150042296859647,0.,0.988679578606275));
#47597=DIRECTION('',(-0.931242779705751,0.,0.364399348580519));
#47598=DIRECTION('',(-0.781200482846105,0.,-0.624280230025758));
#47599=DIRECTION('',(0.150042296859641,0.,-0.988679578606276));
#47600=DIRECTION('',(0.931242779705752,0.,-0.364399348580517));
#47601=DIRECTION('',(0.781200482846104,0.,0.624280230025758));
#47602=DIRECTION('',(-0.150042296859647,0.,0.988679578606275));
#47603=DIRECTION('',(-0.931242779705751,0.,0.364399348580519));
#47604=DIRECTION('',(-0.781200482846105,0.,-0.624280230025758));
#47605=DIRECTION('',(0.150042296859641,0.,-0.988679578606276));
#47606=DIRECTION('',(0.931242779705752,0.,-0.364399348580517));
#47607=DIRECTION('',(0.781200482846104,0.,0.624280230025758));
#47608=DIRECTION('',(-0.150042296859647,0.,0.988679578606275));
#47609=DIRECTION('',(-0.931242779705751,0.,0.364399348580519));
#47610=DIRECTION('',(-0.781200482846105,0.,-0.624280230025758));
#47611=DIRECTION('',(0.150042296859641,0.,-0.988679578606276));
#47612=DIRECTION('',(0.931242779705752,0.,-0.364399348580517));
#47613=DIRECTION('',(0.781200482846104,0.,0.624280230025758));
#47614=DIRECTION('',(-0.150042296859647,0.,0.988679578606275));
#47615=DIRECTION('',(-0.931242779705751,0.,0.364399348580519));
#47616=DIRECTION('',(-0.781200482846105,0.,-0.624280230025758));
#47617=DIRECTION('',(0.150042296859641,0.,-0.988679578606276));
#47618=DIRECTION('',(0.931242779705752,0.,-0.364399348580517));
#47619=DIRECTION('',(0.781200482846104,0.,0.624280230025758));
#47620=DIRECTION('',(-0.150042296859647,0.,0.988679578606275));
#47621=DIRECTION('',(-0.931242779705751,0.,0.364399348580519));
#47622=DIRECTION('',(-0.781200482846105,0.,-0.624280230025758));
#47623=DIRECTION('',(0.150042296859641,0.,-0.988679578606276));
#47624=DIRECTION('',(0.931242779705752,0.,-0.364399348580517));
#47625=DIRECTION('',(0.781200482846104,0.,0.624280230025758));
#47626=DIRECTION('',(-0.150042296859647,0.,0.988679578606275));
#47627=DIRECTION('',(-0.931242779705751,0.,0.364399348580519));
#47628=DIRECTION('',(-0.781200482846105,0.,-0.624280230025758));
#47629=DIRECTION('',(0.150042296859641,0.,-0.988679578606276));
#47630=DIRECTION('',(0.931242779705752,0.,-0.364399348580517));
#47631=DIRECTION('',(0.781200482846104,0.,0.624280230025758));
#47632=DIRECTION('',(-0.150042296859647,0.,0.988679578606275));
#47633=DIRECTION('',(-0.931242779705751,0.,0.364399348580519));
#47634=DIRECTION('',(-0.781200482846105,0.,-0.624280230025758));
#47635=DIRECTION('',(0.150042296859641,0.,-0.988679578606276));
#47636=DIRECTION('',(0.931242779705752,0.,-0.364399348580517));
#47637=DIRECTION('',(0.781200482846104,0.,0.624280230025758));
#47638=DIRECTION('',(-0.150042296859647,0.,0.988679578606275));
#47639=DIRECTION('',(-0.931242779705751,0.,0.364399348580519));
#47640=DIRECTION('',(-0.781200482846105,0.,-0.624280230025758));
#47641=DIRECTION('',(0.150042296859641,0.,-0.988679578606276));
#47642=DIRECTION('',(0.931242779705752,0.,-0.364399348580517));
#47643=DIRECTION('',(0.781200482846104,0.,0.624280230025758));
#47644=DIRECTION('',(-0.150042296859647,0.,0.988679578606275));
#47645=DIRECTION('',(-0.931242779705751,0.,0.364399348580519));
#47646=DIRECTION('',(-0.781200482846105,0.,-0.624280230025758));
#47647=DIRECTION('',(0.150042296859641,0.,-0.988679578606276));
#47648=DIRECTION('',(0.931242779705752,0.,-0.364399348580517));
#47649=DIRECTION('',(0.781200482846104,0.,0.624280230025758));
#47650=DIRECTION('',(-0.150042296859647,0.,0.988679578606275));
#47651=DIRECTION('',(-0.931242779705751,0.,0.364399348580519));
#47652=DIRECTION('',(-0.781200482846105,0.,-0.624280230025758));
#47653=DIRECTION('',(0.150042296859641,0.,-0.988679578606276));
#47654=DIRECTION('',(0.931242779705752,0.,-0.364399348580517));
#47655=DIRECTION('',(0.781200482846104,0.,0.624280230025758));
#47656=DIRECTION('',(-0.150042296859647,0.,0.988679578606275));
#47657=DIRECTION('',(-0.931242779705751,0.,0.364399348580519));
#47658=DIRECTION('',(-0.781200482846105,0.,-0.624280230025758));
#47659=DIRECTION('',(0.150042296859641,0.,-0.988679578606276));
#47660=DIRECTION('',(0.931242779705752,0.,-0.364399348580517));
#47661=DIRECTION('',(0.781200482846104,0.,0.624280230025758));
#47662=DIRECTION('',(-0.150042296859647,0.,0.988679578606275));
#47663=DIRECTION('',(-0.931242779705751,0.,0.364399348580519));
#47664=DIRECTION('',(-0.781200482846105,0.,-0.624280230025758));
#47665=DIRECTION('',(0.150042296859641,0.,-0.988679578606276));
#47666=DIRECTION('',(0.931242779705752,0.,-0.364399348580517));
#47667=DIRECTION('',(0.781200482846104,0.,0.624280230025758));
#47668=DIRECTION('',(-0.150042296859647,0.,0.988679578606275));
#47669=DIRECTION('',(-0.931242779705751,0.,0.364399348580519));
#47670=DIRECTION('',(-0.781200482846105,0.,-0.624280230025758));
#47671=DIRECTION('',(0.150042296859641,0.,-0.988679578606276));
#47672=DIRECTION('',(0.931242779705752,0.,-0.364399348580517));
#47673=DIRECTION('',(0.781200482846104,0.,0.624280230025758));
#47674=DIRECTION('',(-0.150042296859647,0.,0.988679578606275));
#47675=DIRECTION('',(-0.931242779705751,0.,0.364399348580519));
#47676=DIRECTION('',(-0.781200482846105,0.,-0.624280230025758));
#47677=DIRECTION('',(0.150042296859641,0.,-0.988679578606276));
#47678=DIRECTION('',(0.931242779705752,0.,-0.364399348580517));
#47679=DIRECTION('',(0.781200482846104,0.,0.624280230025758));
#47680=DIRECTION('',(-0.150042296859647,0.,0.988679578606275));
#47681=DIRECTION('',(-0.931242779705751,0.,0.364399348580519));
#47682=DIRECTION('',(-0.781200482846105,0.,-0.624280230025758));
#47683=DIRECTION('',(0.150042296859641,0.,-0.988679578606276));
#47684=DIRECTION('',(0.931242779705752,0.,-0.364399348580517));
#47685=DIRECTION('',(0.781200482846104,0.,0.624280230025758));
#47686=DIRECTION('',(-0.150042296859647,0.,0.988679578606275));
#47687=DIRECTION('',(-0.931242779705751,0.,0.364399348580519));
#47688=DIRECTION('',(-0.781200482846105,0.,-0.624280230025758));
#47689=DIRECTION('',(0.150042296859641,0.,-0.988679578606276));
#47690=DIRECTION('',(0.931242779705752,0.,-0.364399348580517));
#47691=DIRECTION('',(0.781200482846104,0.,0.624280230025758));
#47692=DIRECTION('',(-0.150042296859647,0.,0.988679578606275));
#47693=DIRECTION('',(-0.931242779705751,0.,0.364399348580519));
#47694=DIRECTION('',(-0.781200482846105,0.,-0.624280230025758));
#47695=DIRECTION('',(0.150042296859641,0.,-0.988679578606276));
#47696=DIRECTION('',(0.931242779705752,0.,-0.364399348580517));
#47697=DIRECTION('',(0.781200482846104,0.,0.624280230025758));
#47698=DIRECTION('',(-0.150042296859647,0.,0.988679578606275));
#47699=DIRECTION('',(-0.931242779705751,0.,0.364399348580519));
#47700=DIRECTION('',(-0.781200482846105,0.,-0.624280230025758));
#47701=DIRECTION('',(0.150042296859641,0.,-0.988679578606276));
#47702=DIRECTION('',(0.931242779705752,0.,-0.364399348580517));
#47703=DIRECTION('',(0.781200482846104,0.,0.624280230025758));
#47704=DIRECTION('',(-0.150042296859647,0.,0.988679578606275));
#47705=DIRECTION('',(-0.931242779705751,0.,0.364399348580519));
#47706=DIRECTION('',(-0.781200482846105,0.,-0.624280230025758));
#47707=DIRECTION('',(0.150042296859641,0.,-0.988679578606276));
#47708=DIRECTION('',(0.931242779705752,0.,-0.364399348580517));
#47709=DIRECTION('',(0.781200482846104,0.,0.624280230025758));
#47710=DIRECTION('',(-0.150042296859647,0.,0.988679578606275));
#47711=DIRECTION('',(-0.931242779705751,0.,0.364399348580519));
#47712=DIRECTION('',(-0.781200482846105,0.,-0.624280230025758));
#47713=DIRECTION('',(0.150042296859641,0.,-0.988679578606276));
#47714=DIRECTION('',(0.931242779705752,0.,-0.364399348580517));
#47715=DIRECTION('',(0.781200482846104,0.,0.624280230025758));
#47716=DIRECTION('',(-0.150042296859647,0.,0.988679578606275));
#47717=DIRECTION('',(-0.931242779705751,0.,0.364399348580519));
#47718=DIRECTION('',(-0.781200482846105,0.,-0.624280230025758));
#47719=DIRECTION('',(0.150042296859641,0.,-0.988679578606276));
#47720=DIRECTION('',(0.931242779705752,0.,-0.364399348580517));
#47721=DIRECTION('',(0.781200482846104,0.,0.624280230025758));
#47722=DIRECTION('',(-0.150042296859647,0.,0.988679578606275));
#47723=DIRECTION('',(-0.931242779705751,0.,0.364399348580519));
#47724=DIRECTION('',(-0.781200482846105,0.,-0.624280230025758));
#47725=DIRECTION('',(0.150042296859641,0.,-0.988679578606276));
#47726=DIRECTION('',(0.931242779705752,0.,-0.364399348580517));
#47727=DIRECTION('',(0.781200482846104,0.,0.624280230025758));
#47728=DIRECTION('',(-0.150042296859647,0.,0.988679578606275));
#47729=DIRECTION('',(-0.931242779705751,0.,0.364399348580519));
#47730=DIRECTION('',(-0.781200482846105,0.,-0.624280230025758));
#47731=DIRECTION('',(0.150042296859641,0.,-0.988679578606276));
#47732=DIRECTION('',(0.931242779705752,0.,-0.364399348580517));
#47733=DIRECTION('',(0.781200482846104,0.,0.624280230025758));
#47734=DIRECTION('',(-0.150042296859647,0.,0.988679578606275));
#47735=DIRECTION('',(-0.931242779705751,0.,0.364399348580519));
#47736=DIRECTION('',(-0.781200482846105,0.,-0.624280230025758));
#47737=DIRECTION('',(0.150042296859641,0.,-0.988679578606276));
#47738=DIRECTION('',(0.931242779705752,0.,-0.364399348580517));
#47739=DIRECTION('',(0.781200482846104,0.,0.624280230025758));
#47740=DIRECTION('',(-0.150042296859647,0.,0.988679578606275));
#47741=DIRECTION('',(-0.931242779705751,0.,0.364399348580519));
#47742=DIRECTION('',(-0.781200482846105,0.,-0.624280230025758));
#47743=DIRECTION('',(0.150042296859641,0.,-0.988679578606276));
#47744=DIRECTION('',(0.931242779705752,0.,-0.364399348580517));
#47745=DIRECTION('',(0.781200482846104,0.,0.624280230025758));
#47746=DIRECTION('',(-0.150042296859647,0.,0.988679578606275));
#47747=DIRECTION('',(-0.931242779705751,0.,0.364399348580519));
#47748=DIRECTION('',(-0.781200482846105,0.,-0.624280230025758));
#47749=DIRECTION('',(0.150042296859641,0.,-0.988679578606276));
#47750=DIRECTION('',(0.931242779705752,0.,-0.364399348580517));
#47751=DIRECTION('',(0.781200482846104,0.,0.624280230025758));
#47752=DIRECTION('',(-0.150042296859647,0.,0.988679578606275));
#47753=DIRECTION('',(-0.931242779705751,0.,0.364399348580519));
#47754=DIRECTION('',(-0.781200482846105,0.,-0.624280230025758));
#47755=DIRECTION('',(0.150042296859641,0.,-0.988679578606276));
#47756=DIRECTION('',(0.931242779705752,0.,-0.364399348580517));
#47757=DIRECTION('',(0.781200482846104,0.,0.624280230025758));
#47758=DIRECTION('',(-0.150042296859647,0.,0.988679578606275));
#47759=DIRECTION('',(-0.931242779705751,0.,0.364399348580519));
#47760=DIRECTION('',(-0.781200482846105,0.,-0.624280230025758));
#47761=DIRECTION('',(0.150042296859641,0.,-0.988679578606276));
#47762=DIRECTION('',(0.931242779705752,0.,-0.364399348580517));
#47763=DIRECTION('',(0.781200482846104,0.,0.624280230025758));
#47764=DIRECTION('',(-0.150042296859647,0.,0.988679578606275));
#47765=DIRECTION('',(-0.931242779705751,0.,0.364399348580519));
#47766=DIRECTION('',(-0.781200482846105,0.,-0.624280230025758));
#47767=DIRECTION('',(0.150042296859641,0.,-0.988679578606276));
#47768=DIRECTION('',(0.931242779705752,0.,-0.364399348580517));
#47769=DIRECTION('',(0.781200482846104,0.,0.624280230025758));
#47770=DIRECTION('',(-0.150042296859647,0.,0.988679578606275));
#47771=DIRECTION('',(-0.931242779705751,0.,0.364399348580519));
#47772=DIRECTION('',(-0.781200482846105,0.,-0.624280230025758));
#47773=DIRECTION('',(0.150042296859641,0.,-0.988679578606276));
#47774=DIRECTION('',(0.931242779705752,0.,-0.364399348580517));
#47775=DIRECTION('',(0.781200482846104,0.,0.624280230025758));
#47776=DIRECTION('',(-0.150042296859647,0.,0.988679578606275));
#47777=DIRECTION('',(-0.931242779705751,0.,0.364399348580519));
#47778=DIRECTION('',(-0.781200482846105,0.,-0.624280230025758));
#47779=DIRECTION('',(0.150042296859641,0.,-0.988679578606276));
#47780=DIRECTION('',(0.931242779705752,0.,-0.364399348580517));
#47781=DIRECTION('',(0.781200482846104,0.,0.624280230025758));
#47782=DIRECTION('',(-0.150042296859647,0.,0.988679578606275));
#47783=DIRECTION('',(-0.931242779705751,0.,0.364399348580519));
#47784=DIRECTION('',(-0.781200482846105,0.,-0.624280230025758));
#47785=DIRECTION('',(0.150042296859641,0.,-0.988679578606276));
#47786=DIRECTION('',(0.931242779705752,0.,-0.364399348580517));
#47787=DIRECTION('',(0.781200482846104,0.,0.624280230025758));
#47788=DIRECTION('',(-0.150042296859647,0.,0.988679578606275));
#47789=DIRECTION('',(-0.931242779705751,0.,0.364399348580519));
#47790=DIRECTION('',(-0.781200482846105,0.,-0.624280230025758));
#47791=DIRECTION('',(0.150042296859641,0.,-0.988679578606276));
#47792=DIRECTION('',(0.931242779705752,0.,-0.364399348580517));
#47793=DIRECTION('',(0.781200482846104,0.,0.624280230025758));
#47794=DIRECTION('',(-0.150042296859647,0.,0.988679578606275));
#47795=DIRECTION('',(-0.931242779705751,0.,0.364399348580519));
#47796=DIRECTION('',(-0.781200482846105,0.,-0.624280230025758));
#47797=DIRECTION('',(0.150042296859641,0.,-0.988679578606276));
#47798=DIRECTION('',(0.931242779705752,0.,-0.364399348580517));
#47799=DIRECTION('',(0.781200482846104,0.,0.624280230025758));
#47800=DIRECTION('',(-0.150042296859647,0.,0.988679578606275));
#47801=DIRECTION('',(-0.931242779705751,0.,0.364399348580519));
#47802=DIRECTION('',(-0.781200482846105,0.,-0.624280230025758));
#47803=DIRECTION('',(0.150042296859641,0.,-0.988679578606276));
#47804=DIRECTION('',(0.931242779705752,0.,-0.364399348580517));
#47805=DIRECTION('',(0.781200482846104,0.,0.624280230025758));
#47806=DIRECTION('',(-0.150042296859647,0.,0.988679578606275));
#47807=DIRECTION('',(-0.931242779705751,0.,0.364399348580519));
#47808=DIRECTION('',(-0.781200482846105,0.,-0.624280230025758));
#47809=DIRECTION('',(0.150042296859641,0.,-0.988679578606276));
#47810=DIRECTION('',(0.931242779705752,0.,-0.364399348580517));
#47811=DIRECTION('',(0.781200482846104,0.,0.624280230025758));
#47812=DIRECTION('',(-0.150042296859647,0.,0.988679578606275));
#47813=DIRECTION('',(-0.931242779705751,0.,0.364399348580519));
#47814=DIRECTION('',(-0.781200482846105,0.,-0.624280230025758));
#47815=DIRECTION('',(0.150042296859641,0.,-0.988679578606276));
#47816=DIRECTION('',(0.931242779705752,0.,-0.364399348580517));
#47817=DIRECTION('',(0.781200482846104,0.,0.624280230025758));
#47818=DIRECTION('',(-0.150042296859647,0.,0.988679578606275));
#47819=DIRECTION('',(-0.931242779705751,0.,0.364399348580519));
#47820=DIRECTION('',(-0.781200482846105,0.,-0.624280230025758));
#47821=DIRECTION('',(0.150042296859641,0.,-0.988679578606276));
#47822=DIRECTION('',(0.931242779705752,0.,-0.364399348580517));
#47823=DIRECTION('',(0.781200482846104,0.,0.624280230025758));
#47824=DIRECTION('',(-0.150042296859647,0.,0.988679578606275));
#47825=DIRECTION('',(-0.931242779705751,0.,0.364399348580519));
#47826=DIRECTION('',(-0.781200482846105,0.,-0.624280230025758));
#47827=DIRECTION('',(0.150042296859641,0.,-0.988679578606276));
#47828=DIRECTION('',(0.931242779705752,0.,-0.364399348580517));
#47829=DIRECTION('',(0.781200482846104,0.,0.624280230025758));
#47830=DIRECTION('',(-0.150042296859647,0.,0.988679578606275));
#47831=DIRECTION('',(-0.931242779705751,0.,0.364399348580519));
#47832=DIRECTION('',(-0.781200482846105,0.,-0.624280230025758));
#47833=DIRECTION('',(0.150042296859641,0.,-0.988679578606276));
#47834=DIRECTION('',(0.931242779705752,0.,-0.364399348580517));
#47835=DIRECTION('',(0.781200482846104,0.,0.624280230025758));
#47836=DIRECTION('',(-0.150042296859647,0.,0.988679578606275));
#47837=DIRECTION('',(-0.931242779705751,0.,0.364399348580519));
#47838=DIRECTION('',(-0.781200482846105,0.,-0.624280230025758));
#47839=DIRECTION('',(0.150042296859641,0.,-0.988679578606276));
#47840=DIRECTION('',(0.931242779705752,0.,-0.364399348580517));
#47841=DIRECTION('',(0.781200482846104,0.,0.624280230025758));
#47842=DIRECTION('',(-0.150042296859647,0.,0.988679578606275));
#47843=DIRECTION('',(-0.931242779705751,0.,0.364399348580519));
#47844=DIRECTION('',(-0.781200482846105,0.,-0.624280230025758));
#47845=DIRECTION('',(0.150042296859641,0.,-0.988679578606276));
#47846=DIRECTION('',(0.931242779705752,0.,-0.364399348580517));
#47847=DIRECTION('',(0.781200482846104,0.,0.624280230025758));
#47848=DIRECTION('',(-0.150042296859647,0.,0.988679578606275));
#47849=DIRECTION('',(-0.931242779705751,0.,0.364399348580519));
#47850=DIRECTION('',(-0.781200482846105,0.,-0.624280230025758));
#47851=DIRECTION('',(0.150042296859641,0.,-0.988679578606276));
#47852=DIRECTION('',(0.931242779705752,0.,-0.364399348580517));
#47853=DIRECTION('',(0.781200482846104,0.,0.624280230025758));
#47854=DIRECTION('',(-0.150042296859647,0.,0.988679578606275));
#47855=DIRECTION('',(-0.931242779705751,0.,0.364399348580519));
#47856=DIRECTION('',(-0.781200482846105,0.,-0.624280230025758));
#47857=DIRECTION('',(0.150042296859641,0.,-0.988679578606276));
#47858=DIRECTION('',(0.931242779705752,0.,-0.364399348580517));
#47859=DIRECTION('',(0.781200482846104,0.,0.624280230025758));
#47860=DIRECTION('',(-0.150042296859647,0.,0.988679578606275));
#47861=DIRECTION('',(-0.931242779705751,0.,0.364399348580519));
#47862=DIRECTION('',(-0.781200482846105,0.,-0.624280230025758));
#47863=DIRECTION('',(0.150042296859641,0.,-0.988679578606276));
#47864=DIRECTION('',(0.931242779705752,0.,-0.364399348580517));
#47865=DIRECTION('',(0.781200482846104,0.,0.624280230025758));
#47866=DIRECTION('',(-0.150042296859647,0.,0.988679578606275));
#47867=DIRECTION('',(-0.931242779705751,0.,0.364399348580519));
#47868=DIRECTION('',(-0.781200482846105,0.,-0.624280230025758));
#47869=DIRECTION('',(0.150042296859641,0.,-0.988679578606276));
#47870=DIRECTION('',(0.931242779705752,0.,-0.364399348580517));
#47871=DIRECTION('',(0.781200482846104,0.,0.624280230025758));
#47872=DIRECTION('',(-0.150042296859647,0.,0.988679578606275));
#47873=DIRECTION('',(-0.931242779705751,0.,0.364399348580519));
#47874=DIRECTION('',(-0.781200482846105,0.,-0.624280230025758));
#47875=DIRECTION('',(0.150042296859641,0.,-0.988679578606276));
#47876=DIRECTION('',(0.931242779705752,0.,-0.364399348580517));
#47877=DIRECTION('',(0.781200482846104,0.,0.624280230025758));
#47878=DIRECTION('',(-0.150042296859647,0.,0.988679578606275));
#47879=DIRECTION('',(-0.931242779705751,0.,0.364399348580519));
#47880=DIRECTION('',(-0.781200482846105,0.,-0.624280230025758));
#47881=DIRECTION('',(0.150042296859641,0.,-0.988679578606276));
#47882=DIRECTION('',(0.931242779705752,0.,-0.364399348580517));
#47883=DIRECTION('',(0.781200482846104,0.,0.624280230025758));
#47884=DIRECTION('',(-0.150042296859647,0.,0.988679578606275));
#47885=DIRECTION('',(-0.931242779705751,0.,0.364399348580519));
#47886=DIRECTION('',(-0.781200482846105,0.,-0.624280230025758));
#47887=DIRECTION('',(0.150042296859641,0.,-0.988679578606276));
#47888=DIRECTION('',(0.931242779705752,0.,-0.364399348580517));
#47889=DIRECTION('',(0.781200482846104,0.,0.624280230025758));
#47890=DIRECTION('',(-0.150042296859647,0.,0.988679578606275));
#47891=DIRECTION('',(-0.931242779705751,0.,0.364399348580519));
#47892=DIRECTION('',(-0.781200482846105,0.,-0.624280230025758));
#47893=DIRECTION('',(0.150042296859641,0.,-0.988679578606276));
#47894=DIRECTION('',(0.931242779705752,0.,-0.364399348580517));
#47895=DIRECTION('',(0.781200482846104,0.,0.624280230025758));
#47896=DIRECTION('',(-0.150042296859647,0.,0.988679578606275));
#47897=DIRECTION('',(-0.931242779705751,0.,0.364399348580519));
#47898=DIRECTION('',(-0.781200482846105,0.,-0.624280230025758));
#47899=DIRECTION('',(0.150042296859641,0.,-0.988679578606276));
#47900=DIRECTION('',(0.931242779705752,0.,-0.364399348580517));
#47901=DIRECTION('',(0.781200482846104,0.,0.624280230025758));
#47902=DIRECTION('',(-0.150042296859647,0.,0.988679578606275));
#47903=DIRECTION('',(-0.931242779705751,0.,0.364399348580519));
#47904=DIRECTION('',(-0.781200482846105,0.,-0.624280230025758));
#47905=DIRECTION('',(0.150042296859641,0.,-0.988679578606276));
#47906=DIRECTION('',(0.931242779705752,0.,-0.364399348580517));
#47907=DIRECTION('',(0.781200482846104,0.,0.624280230025758));
#47908=DIRECTION('',(-0.150042296859647,0.,0.988679578606275));
#47909=DIRECTION('',(-0.931242779705751,0.,0.364399348580519));
#47910=DIRECTION('',(-0.781200482846105,0.,-0.624280230025758));
#47911=DIRECTION('',(0.150042296859641,0.,-0.988679578606276));
#47912=DIRECTION('',(0.931242779705752,0.,-0.364399348580517));
#47913=DIRECTION('',(0.781200482846104,0.,0.624280230025758));
#47914=DIRECTION('',(-0.150042296859647,0.,0.988679578606275));
#47915=DIRECTION('',(-0.931242779705751,0.,0.364399348580519));
#47916=DIRECTION('',(-0.781200482846105,0.,-0.624280230025758));
#47917=DIRECTION('',(0.150042296859641,0.,-0.988679578606276));
#47918=DIRECTION('',(0.931242779705752,0.,-0.364399348580517));
#47919=DIRECTION('',(0.781200482846104,0.,0.624280230025758));
#47920=DIRECTION('',(-0.150042296859647,0.,0.988679578606275));
#47921=DIRECTION('',(-0.931242779705751,0.,0.364399348580519));
#47922=DIRECTION('',(-0.781200482846105,0.,-0.624280230025758));
#47923=DIRECTION('',(0.150042296859641,0.,-0.988679578606276));
#47924=DIRECTION('',(0.931242779705752,0.,-0.364399348580517));
#47925=DIRECTION('',(0.781200482846104,0.,0.624280230025758));
#47926=DIRECTION('',(-0.150042296859647,0.,0.988679578606275));
#47927=DIRECTION('',(-0.931242779705751,0.,0.364399348580519));
#47928=DIRECTION('',(-0.781200482846105,0.,-0.624280230025758));
#47929=DIRECTION('',(0.150042296859641,0.,-0.988679578606276));
#47930=DIRECTION('',(0.931242779705752,0.,-0.364399348580517));
#47931=DIRECTION('',(0.781200482846104,0.,0.624280230025758));
#47932=DIRECTION('',(-0.150042296859647,0.,0.988679578606275));
#47933=DIRECTION('',(-0.931242779705751,0.,0.364399348580519));
#47934=DIRECTION('',(-0.781200482846105,0.,-0.624280230025758));
#47935=DIRECTION('',(0.150042296859641,0.,-0.988679578606276));
#47936=DIRECTION('',(0.931242779705752,0.,-0.364399348580517));
#47937=DIRECTION('',(0.781200482846104,0.,0.624280230025758));
#47938=DIRECTION('',(-0.150042296859647,0.,0.988679578606275));
#47939=DIRECTION('',(-0.931242779705751,0.,0.364399348580519));
#47940=DIRECTION('',(-0.781200482846105,0.,-0.624280230025758));
#47941=DIRECTION('',(0.150042296859641,0.,-0.988679578606276));
#47942=DIRECTION('',(0.931242779705752,0.,-0.364399348580517));
#47943=DIRECTION('',(0.781200482846104,0.,0.624280230025758));
#47944=DIRECTION('',(-0.150042296859647,0.,0.988679578606275));
#47945=DIRECTION('',(-0.931242779705751,0.,0.364399348580519));
#47946=DIRECTION('',(-0.781200482846105,0.,-0.624280230025758));
#47947=DIRECTION('',(0.150042296859641,0.,-0.988679578606276));
#47948=DIRECTION('',(0.931242779705752,0.,-0.364399348580517));
#47949=DIRECTION('',(0.781200482846104,0.,0.624280230025758));
#47950=DIRECTION('',(-0.150042296859647,0.,0.988679578606275));
#47951=DIRECTION('',(-0.931242779705751,0.,0.364399348580519));
#47952=DIRECTION('',(-0.781200482846105,0.,-0.624280230025758));
#47953=DIRECTION('',(0.150042296859641,0.,-0.988679578606276));
#47954=DIRECTION('',(0.931242779705752,0.,-0.364399348580517));
#47955=DIRECTION('',(0.781200482846104,0.,0.624280230025758));
#47956=DIRECTION('',(-0.150042296859647,0.,0.988679578606275));
#47957=DIRECTION('',(-0.931242779705751,0.,0.364399348580519));
#47958=DIRECTION('',(-0.781200482846105,0.,-0.624280230025758));
#47959=DIRECTION('',(0.150042296859641,0.,-0.988679578606276));
#47960=DIRECTION('',(0.931242779705752,0.,-0.364399348580517));
#47961=DIRECTION('',(0.781200482846104,0.,0.624280230025758));
#47962=DIRECTION('',(-0.150042296859647,0.,0.988679578606275));
#47963=DIRECTION('',(-0.931242779705751,0.,0.364399348580519));
#47964=DIRECTION('',(-0.781200482846105,0.,-0.624280230025758));
#47965=DIRECTION('',(0.150042296859641,0.,-0.988679578606276));
#47966=DIRECTION('',(0.931242779705752,0.,-0.364399348580517));
#47967=DIRECTION('',(0.781200482846104,0.,0.624280230025758));
#47968=DIRECTION('',(-0.150042296859647,0.,0.988679578606275));
#47969=DIRECTION('',(-0.931242779705751,0.,0.364399348580519));
#47970=DIRECTION('',(-0.781200482846105,0.,-0.624280230025758));
#47971=DIRECTION('',(0.150042296859641,0.,-0.988679578606276));
#47972=DIRECTION('',(0.931242779705752,0.,-0.364399348580517));
#47973=DIRECTION('',(0.781200482846104,0.,0.624280230025758));
#47974=DIRECTION('',(-0.150042296859647,0.,0.988679578606275));
#47975=DIRECTION('',(-0.931242779705751,0.,0.364399348580519));
#47976=DIRECTION('',(-0.781200482846105,0.,-0.624280230025758));
#47977=DIRECTION('center_axis',(0.,1.,0.));
#47978=DIRECTION('ref_axis',(1.,0.,0.));
#47979=DIRECTION('',(0.931242779705752,0.,-0.364399348580517));
#47980=DIRECTION('',(0.150042296859641,0.,-0.988679578606276));
#47981=DIRECTION('',(-0.781200482846105,0.,-0.624280230025758));
#47982=DIRECTION('',(-0.931242779705751,0.,0.364399348580519));
#47983=DIRECTION('',(-0.150042296859647,0.,0.988679578606275));
#47984=DIRECTION('',(0.781200482846104,0.,0.624280230025758));
#47985=DIRECTION('',(0.931242779705752,0.,-0.364399348580517));
#47986=DIRECTION('',(0.150042296859641,0.,-0.988679578606276));
#47987=DIRECTION('',(-0.781200482846105,0.,-0.624280230025758));
#47988=DIRECTION('',(-0.931242779705751,0.,0.364399348580519));
#47989=DIRECTION('',(-0.150042296859647,0.,0.988679578606275));
#47990=DIRECTION('',(0.781200482846104,0.,0.624280230025758));
#47991=DIRECTION('',(0.931242779705752,0.,-0.364399348580517));
#47992=DIRECTION('',(0.150042296859641,0.,-0.988679578606276));
#47993=DIRECTION('',(-0.781200482846105,0.,-0.624280230025758));
#47994=DIRECTION('',(-0.931242779705751,0.,0.364399348580519));
#47995=DIRECTION('',(-0.150042296859647,0.,0.988679578606275));
#47996=DIRECTION('',(0.781200482846104,0.,0.624280230025758));
#47997=DIRECTION('',(0.931242779705752,0.,-0.364399348580517));
#47998=DIRECTION('',(0.150042296859641,0.,-0.988679578606276));
#47999=DIRECTION('',(-0.781200482846105,0.,-0.624280230025758));
#48000=DIRECTION('',(-0.931242779705751,0.,0.364399348580519));
#48001=DIRECTION('',(-0.150042296859647,0.,0.988679578606275));
#48002=DIRECTION('',(0.781200482846104,0.,0.624280230025758));
#48003=DIRECTION('',(0.931242779705752,0.,-0.364399348580517));
#48004=DIRECTION('',(0.150042296859641,0.,-0.988679578606276));
#48005=DIRECTION('',(-0.781200482846105,0.,-0.624280230025758));
#48006=DIRECTION('',(-0.931242779705751,0.,0.364399348580519));
#48007=DIRECTION('',(-0.150042296859647,0.,0.988679578606275));
#48008=DIRECTION('',(0.781200482846104,0.,0.624280230025758));
#48009=DIRECTION('',(0.931242779705752,0.,-0.364399348580517));
#48010=DIRECTION('',(0.150042296859641,0.,-0.988679578606276));
#48011=DIRECTION('',(-0.781200482846105,0.,-0.624280230025758));
#48012=DIRECTION('',(-0.931242779705751,0.,0.364399348580519));
#48013=DIRECTION('',(-0.150042296859647,0.,0.988679578606275));
#48014=DIRECTION('',(0.781200482846104,0.,0.624280230025758));
#48015=DIRECTION('',(0.931242779705752,0.,-0.364399348580517));
#48016=DIRECTION('',(0.150042296859641,0.,-0.988679578606276));
#48017=DIRECTION('',(-0.781200482846105,0.,-0.624280230025758));
#48018=DIRECTION('',(-0.931242779705751,0.,0.364399348580519));
#48019=DIRECTION('',(-0.150042296859647,0.,0.988679578606275));
#48020=DIRECTION('',(0.781200482846104,0.,0.624280230025758));
#48021=DIRECTION('',(0.931242779705752,0.,-0.364399348580517));
#48022=DIRECTION('',(0.150042296859641,0.,-0.988679578606276));
#48023=DIRECTION('',(-0.781200482846105,0.,-0.624280230025758));
#48024=DIRECTION('',(-0.931242779705751,0.,0.364399348580519));
#48025=DIRECTION('',(-0.150042296859647,0.,0.988679578606275));
#48026=DIRECTION('',(0.781200482846104,0.,0.624280230025758));
#48027=DIRECTION('',(0.931242779705752,0.,-0.364399348580517));
#48028=DIRECTION('',(0.150042296859641,0.,-0.988679578606276));
#48029=DIRECTION('',(-0.781200482846105,0.,-0.624280230025758));
#48030=DIRECTION('',(-0.931242779705751,0.,0.364399348580519));
#48031=DIRECTION('',(-0.150042296859647,0.,0.988679578606275));
#48032=DIRECTION('',(0.781200482846104,0.,0.624280230025758));
#48033=DIRECTION('',(0.931242779705752,0.,-0.364399348580517));
#48034=DIRECTION('',(0.150042296859641,0.,-0.988679578606276));
#48035=DIRECTION('',(-0.781200482846105,0.,-0.624280230025758));
#48036=DIRECTION('',(-0.931242779705751,0.,0.364399348580519));
#48037=DIRECTION('',(-0.150042296859647,0.,0.988679578606275));
#48038=DIRECTION('',(0.781200482846104,0.,0.624280230025758));
#48039=DIRECTION('',(0.931242779705752,0.,-0.364399348580517));
#48040=DIRECTION('',(0.150042296859641,0.,-0.988679578606276));
#48041=DIRECTION('',(-0.781200482846105,0.,-0.624280230025758));
#48042=DIRECTION('',(-0.931242779705751,0.,0.364399348580519));
#48043=DIRECTION('',(-0.150042296859647,0.,0.988679578606275));
#48044=DIRECTION('',(0.781200482846104,0.,0.624280230025758));
#48045=DIRECTION('',(0.931242779705752,0.,-0.364399348580517));
#48046=DIRECTION('',(0.150042296859641,0.,-0.988679578606276));
#48047=DIRECTION('',(-0.781200482846105,0.,-0.624280230025758));
#48048=DIRECTION('',(-0.931242779705751,0.,0.364399348580519));
#48049=DIRECTION('',(-0.150042296859647,0.,0.988679578606275));
#48050=DIRECTION('',(0.781200482846104,0.,0.624280230025758));
#48051=DIRECTION('',(0.931242779705752,0.,-0.364399348580517));
#48052=DIRECTION('',(0.150042296859641,0.,-0.988679578606276));
#48053=DIRECTION('',(-0.781200482846105,0.,-0.624280230025758));
#48054=DIRECTION('',(-0.931242779705751,0.,0.364399348580519));
#48055=DIRECTION('',(-0.150042296859647,0.,0.988679578606275));
#48056=DIRECTION('',(0.781200482846104,0.,0.624280230025758));
#48057=DIRECTION('',(0.931242779705752,0.,-0.364399348580517));
#48058=DIRECTION('',(0.150042296859641,0.,-0.988679578606276));
#48059=DIRECTION('',(-0.781200482846105,0.,-0.624280230025758));
#48060=DIRECTION('',(-0.931242779705751,0.,0.364399348580519));
#48061=DIRECTION('',(-0.150042296859647,0.,0.988679578606275));
#48062=DIRECTION('',(0.781200482846104,0.,0.624280230025758));
#48063=DIRECTION('',(0.931242779705752,0.,-0.364399348580517));
#48064=DIRECTION('',(0.150042296859641,0.,-0.988679578606276));
#48065=DIRECTION('',(-0.781200482846105,0.,-0.624280230025758));
#48066=DIRECTION('',(-0.931242779705751,0.,0.364399348580519));
#48067=DIRECTION('',(-0.150042296859647,0.,0.988679578606275));
#48068=DIRECTION('',(0.781200482846104,0.,0.624280230025758));
#48069=DIRECTION('',(0.931242779705752,0.,-0.364399348580517));
#48070=DIRECTION('',(0.150042296859641,0.,-0.988679578606276));
#48071=DIRECTION('',(-0.781200482846105,0.,-0.624280230025758));
#48072=DIRECTION('',(-0.931242779705751,0.,0.364399348580519));
#48073=DIRECTION('',(-0.150042296859647,0.,0.988679578606275));
#48074=DIRECTION('',(0.781200482846104,0.,0.624280230025758));
#48075=DIRECTION('',(0.931242779705752,0.,-0.364399348580517));
#48076=DIRECTION('',(0.150042296859641,0.,-0.988679578606276));
#48077=DIRECTION('',(-0.781200482846105,0.,-0.624280230025758));
#48078=DIRECTION('',(-0.931242779705751,0.,0.364399348580519));
#48079=DIRECTION('',(-0.150042296859647,0.,0.988679578606275));
#48080=DIRECTION('',(0.781200482846104,0.,0.624280230025758));
#48081=DIRECTION('',(0.931242779705752,0.,-0.364399348580517));
#48082=DIRECTION('',(0.150042296859641,0.,-0.988679578606276));
#48083=DIRECTION('',(-0.781200482846105,0.,-0.624280230025758));
#48084=DIRECTION('',(-0.931242779705751,0.,0.364399348580519));
#48085=DIRECTION('',(-0.150042296859647,0.,0.988679578606275));
#48086=DIRECTION('',(0.781200482846104,0.,0.624280230025758));
#48087=DIRECTION('',(0.931242779705752,0.,-0.364399348580517));
#48088=DIRECTION('',(0.150042296859641,0.,-0.988679578606276));
#48089=DIRECTION('',(-0.781200482846105,0.,-0.624280230025758));
#48090=DIRECTION('',(-0.931242779705751,0.,0.364399348580519));
#48091=DIRECTION('',(-0.150042296859647,0.,0.988679578606275));
#48092=DIRECTION('',(0.781200482846104,0.,0.624280230025758));
#48093=DIRECTION('',(0.931242779705752,0.,-0.364399348580517));
#48094=DIRECTION('',(0.150042296859641,0.,-0.988679578606276));
#48095=DIRECTION('',(-0.781200482846105,0.,-0.624280230025758));
#48096=DIRECTION('',(-0.931242779705751,0.,0.364399348580519));
#48097=DIRECTION('',(-0.150042296859647,0.,0.988679578606275));
#48098=DIRECTION('',(0.781200482846104,0.,0.624280230025758));
#48099=DIRECTION('',(0.931242779705752,0.,-0.364399348580517));
#48100=DIRECTION('',(0.150042296859641,0.,-0.988679578606276));
#48101=DIRECTION('',(-0.781200482846105,0.,-0.624280230025758));
#48102=DIRECTION('',(-0.931242779705751,0.,0.364399348580519));
#48103=DIRECTION('',(-0.150042296859647,0.,0.988679578606275));
#48104=DIRECTION('',(0.781200482846104,0.,0.624280230025758));
#48105=DIRECTION('',(0.931242779705752,0.,-0.364399348580517));
#48106=DIRECTION('',(0.150042296859641,0.,-0.988679578606276));
#48107=DIRECTION('',(-0.781200482846105,0.,-0.624280230025758));
#48108=DIRECTION('',(-0.931242779705751,0.,0.364399348580519));
#48109=DIRECTION('',(-0.150042296859647,0.,0.988679578606275));
#48110=DIRECTION('',(0.781200482846104,0.,0.624280230025758));
#48111=DIRECTION('',(0.931242779705752,0.,-0.364399348580517));
#48112=DIRECTION('',(0.150042296859641,0.,-0.988679578606276));
#48113=DIRECTION('',(-0.781200482846105,0.,-0.624280230025758));
#48114=DIRECTION('',(-0.931242779705751,0.,0.364399348580519));
#48115=DIRECTION('',(-0.150042296859647,0.,0.988679578606275));
#48116=DIRECTION('',(0.781200482846104,0.,0.624280230025758));
#48117=DIRECTION('',(0.931242779705752,0.,-0.364399348580517));
#48118=DIRECTION('',(0.150042296859641,0.,-0.988679578606276));
#48119=DIRECTION('',(-0.781200482846105,0.,-0.624280230025758));
#48120=DIRECTION('',(-0.931242779705751,0.,0.364399348580519));
#48121=DIRECTION('',(-0.150042296859647,0.,0.988679578606275));
#48122=DIRECTION('',(0.781200482846104,0.,0.624280230025758));
#48123=DIRECTION('',(0.931242779705752,0.,-0.364399348580517));
#48124=DIRECTION('',(0.150042296859641,0.,-0.988679578606276));
#48125=DIRECTION('',(-0.781200482846105,0.,-0.624280230025758));
#48126=DIRECTION('',(-0.931242779705751,0.,0.364399348580519));
#48127=DIRECTION('',(-0.150042296859647,0.,0.988679578606275));
#48128=DIRECTION('',(0.781200482846104,0.,0.624280230025758));
#48129=DIRECTION('',(0.931242779705752,0.,-0.364399348580517));
#48130=DIRECTION('',(0.150042296859641,0.,-0.988679578606276));
#48131=DIRECTION('',(-0.781200482846105,0.,-0.624280230025758));
#48132=DIRECTION('',(-0.931242779705751,0.,0.364399348580519));
#48133=DIRECTION('',(-0.150042296859647,0.,0.988679578606275));
#48134=DIRECTION('',(0.781200482846104,0.,0.624280230025758));
#48135=DIRECTION('',(0.931242779705752,0.,-0.364399348580517));
#48136=DIRECTION('',(0.150042296859641,0.,-0.988679578606276));
#48137=DIRECTION('',(-0.781200482846105,0.,-0.624280230025758));
#48138=DIRECTION('',(-0.931242779705751,0.,0.364399348580519));
#48139=DIRECTION('',(-0.150042296859647,0.,0.988679578606275));
#48140=DIRECTION('',(0.781200482846104,0.,0.624280230025758));
#48141=DIRECTION('',(0.931242779705752,0.,-0.364399348580517));
#48142=DIRECTION('',(0.150042296859641,0.,-0.988679578606276));
#48143=DIRECTION('',(-0.781200482846105,0.,-0.624280230025758));
#48144=DIRECTION('',(-0.931242779705751,0.,0.364399348580519));
#48145=DIRECTION('',(-0.150042296859647,0.,0.988679578606275));
#48146=DIRECTION('',(0.781200482846104,0.,0.624280230025758));
#48147=DIRECTION('',(0.931242779705752,0.,-0.364399348580517));
#48148=DIRECTION('',(0.150042296859641,0.,-0.988679578606276));
#48149=DIRECTION('',(-0.781200482846105,0.,-0.624280230025758));
#48150=DIRECTION('',(-0.931242779705751,0.,0.364399348580519));
#48151=DIRECTION('',(-0.150042296859647,0.,0.988679578606275));
#48152=DIRECTION('',(0.781200482846104,0.,0.624280230025758));
#48153=DIRECTION('',(0.931242779705752,0.,-0.364399348580517));
#48154=DIRECTION('',(0.150042296859641,0.,-0.988679578606276));
#48155=DIRECTION('',(-0.781200482846105,0.,-0.624280230025758));
#48156=DIRECTION('',(-0.931242779705751,0.,0.364399348580519));
#48157=DIRECTION('',(-0.150042296859647,0.,0.988679578606275));
#48158=DIRECTION('',(0.781200482846104,0.,0.624280230025758));
#48159=DIRECTION('',(0.931242779705752,0.,-0.364399348580517));
#48160=DIRECTION('',(0.150042296859641,0.,-0.988679578606276));
#48161=DIRECTION('',(-0.781200482846105,0.,-0.624280230025758));
#48162=DIRECTION('',(-0.931242779705751,0.,0.364399348580519));
#48163=DIRECTION('',(-0.150042296859647,0.,0.988679578606275));
#48164=DIRECTION('',(0.781200482846104,0.,0.624280230025758));
#48165=DIRECTION('',(0.931242779705752,0.,-0.364399348580517));
#48166=DIRECTION('',(0.150042296859641,0.,-0.988679578606276));
#48167=DIRECTION('',(-0.781200482846105,0.,-0.624280230025758));
#48168=DIRECTION('',(-0.931242779705751,0.,0.364399348580519));
#48169=DIRECTION('',(-0.150042296859647,0.,0.988679578606275));
#48170=DIRECTION('',(0.781200482846104,0.,0.624280230025758));
#48171=DIRECTION('',(0.931242779705752,0.,-0.364399348580517));
#48172=DIRECTION('',(0.150042296859641,0.,-0.988679578606276));
#48173=DIRECTION('',(-0.781200482846105,0.,-0.624280230025758));
#48174=DIRECTION('',(-0.931242779705751,0.,0.364399348580519));
#48175=DIRECTION('',(-0.150042296859647,0.,0.988679578606275));
#48176=DIRECTION('',(0.781200482846104,0.,0.624280230025758));
#48177=DIRECTION('',(0.931242779705752,0.,-0.364399348580517));
#48178=DIRECTION('',(0.150042296859641,0.,-0.988679578606276));
#48179=DIRECTION('',(-0.781200482846105,0.,-0.624280230025758));
#48180=DIRECTION('',(-0.931242779705751,0.,0.364399348580519));
#48181=DIRECTION('',(-0.150042296859647,0.,0.988679578606275));
#48182=DIRECTION('',(0.781200482846104,0.,0.624280230025758));
#48183=DIRECTION('',(0.931242779705752,0.,-0.364399348580517));
#48184=DIRECTION('',(0.150042296859641,0.,-0.988679578606276));
#48185=DIRECTION('',(-0.781200482846105,0.,-0.624280230025758));
#48186=DIRECTION('',(-0.931242779705751,0.,0.364399348580519));
#48187=DIRECTION('',(-0.150042296859647,0.,0.988679578606275));
#48188=DIRECTION('',(0.781200482846104,0.,0.624280230025758));
#48189=DIRECTION('',(0.931242779705752,0.,-0.364399348580517));
#48190=DIRECTION('',(0.150042296859641,0.,-0.988679578606276));
#48191=DIRECTION('',(-0.781200482846105,0.,-0.624280230025758));
#48192=DIRECTION('',(-0.931242779705751,0.,0.364399348580519));
#48193=DIRECTION('',(-0.150042296859647,0.,0.988679578606275));
#48194=DIRECTION('',(0.781200482846104,0.,0.624280230025758));
#48195=DIRECTION('',(0.931242779705752,0.,-0.364399348580517));
#48196=DIRECTION('',(0.150042296859641,0.,-0.988679578606276));
#48197=DIRECTION('',(-0.781200482846105,0.,-0.624280230025758));
#48198=DIRECTION('',(-0.931242779705751,0.,0.364399348580519));
#48199=DIRECTION('',(-0.150042296859647,0.,0.988679578606275));
#48200=DIRECTION('',(0.781200482846104,0.,0.624280230025758));
#48201=DIRECTION('',(0.931242779705752,0.,-0.364399348580517));
#48202=DIRECTION('',(0.150042296859641,0.,-0.988679578606276));
#48203=DIRECTION('',(-0.781200482846105,0.,-0.624280230025758));
#48204=DIRECTION('',(-0.931242779705751,0.,0.364399348580519));
#48205=DIRECTION('',(-0.150042296859647,0.,0.988679578606275));
#48206=DIRECTION('',(0.781200482846104,0.,0.624280230025758));
#48207=DIRECTION('',(0.931242779705752,0.,-0.364399348580517));
#48208=DIRECTION('',(0.150042296859641,0.,-0.988679578606276));
#48209=DIRECTION('',(-0.781200482846105,0.,-0.624280230025758));
#48210=DIRECTION('',(-0.931242779705751,0.,0.364399348580519));
#48211=DIRECTION('',(-0.150042296859647,0.,0.988679578606275));
#48212=DIRECTION('',(0.781200482846104,0.,0.624280230025758));
#48213=DIRECTION('',(0.931242779705752,0.,-0.364399348580517));
#48214=DIRECTION('',(0.150042296859641,0.,-0.988679578606276));
#48215=DIRECTION('',(-0.781200482846105,0.,-0.624280230025758));
#48216=DIRECTION('',(-0.931242779705751,0.,0.364399348580519));
#48217=DIRECTION('',(-0.150042296859647,0.,0.988679578606275));
#48218=DIRECTION('',(0.781200482846104,0.,0.624280230025758));
#48219=DIRECTION('',(0.931242779705752,0.,-0.364399348580517));
#48220=DIRECTION('',(0.150042296859641,0.,-0.988679578606276));
#48221=DIRECTION('',(-0.781200482846105,0.,-0.624280230025758));
#48222=DIRECTION('',(-0.931242779705751,0.,0.364399348580519));
#48223=DIRECTION('',(-0.150042296859647,0.,0.988679578606275));
#48224=DIRECTION('',(0.781200482846104,0.,0.624280230025758));
#48225=DIRECTION('',(0.931242779705752,0.,-0.364399348580517));
#48226=DIRECTION('',(0.150042296859641,0.,-0.988679578606276));
#48227=DIRECTION('',(-0.781200482846105,0.,-0.624280230025758));
#48228=DIRECTION('',(-0.931242779705751,0.,0.364399348580519));
#48229=DIRECTION('',(-0.150042296859647,0.,0.988679578606275));
#48230=DIRECTION('',(0.781200482846104,0.,0.624280230025758));
#48231=DIRECTION('',(0.931242779705752,0.,-0.364399348580517));
#48232=DIRECTION('',(0.150042296859641,0.,-0.988679578606276));
#48233=DIRECTION('',(-0.781200482846105,0.,-0.624280230025758));
#48234=DIRECTION('',(-0.931242779705751,0.,0.364399348580519));
#48235=DIRECTION('',(-0.150042296859647,0.,0.988679578606275));
#48236=DIRECTION('',(0.781200482846104,0.,0.624280230025758));
#48237=DIRECTION('',(0.931242779705752,0.,-0.364399348580517));
#48238=DIRECTION('',(0.150042296859641,0.,-0.988679578606276));
#48239=DIRECTION('',(-0.781200482846105,0.,-0.624280230025758));
#48240=DIRECTION('',(-0.931242779705751,0.,0.364399348580519));
#48241=DIRECTION('',(-0.150042296859647,0.,0.988679578606275));
#48242=DIRECTION('',(0.781200482846104,0.,0.624280230025758));
#48243=DIRECTION('',(0.931242779705752,0.,-0.364399348580517));
#48244=DIRECTION('',(0.150042296859641,0.,-0.988679578606276));
#48245=DIRECTION('',(-0.781200482846105,0.,-0.624280230025758));
#48246=DIRECTION('',(-0.931242779705751,0.,0.364399348580519));
#48247=DIRECTION('',(-0.150042296859647,0.,0.988679578606275));
#48248=DIRECTION('',(0.781200482846104,0.,0.624280230025758));
#48249=DIRECTION('',(0.931242779705752,0.,-0.364399348580517));
#48250=DIRECTION('',(0.150042296859641,0.,-0.988679578606276));
#48251=DIRECTION('',(-0.781200482846105,0.,-0.624280230025758));
#48252=DIRECTION('',(-0.931242779705751,0.,0.364399348580519));
#48253=DIRECTION('',(-0.150042296859647,0.,0.988679578606275));
#48254=DIRECTION('',(0.781200482846104,0.,0.624280230025758));
#48255=DIRECTION('',(0.931242779705752,0.,-0.364399348580517));
#48256=DIRECTION('',(0.150042296859641,0.,-0.988679578606276));
#48257=DIRECTION('',(-0.781200482846105,0.,-0.624280230025758));
#48258=DIRECTION('',(-0.931242779705751,0.,0.364399348580519));
#48259=DIRECTION('',(-0.150042296859647,0.,0.988679578606275));
#48260=DIRECTION('',(0.781200482846104,0.,0.624280230025758));
#48261=DIRECTION('',(0.931242779705752,0.,-0.364399348580517));
#48262=DIRECTION('',(0.150042296859641,0.,-0.988679578606276));
#48263=DIRECTION('',(-0.781200482846105,0.,-0.624280230025758));
#48264=DIRECTION('',(-0.931242779705751,0.,0.364399348580519));
#48265=DIRECTION('',(-0.150042296859647,0.,0.988679578606275));
#48266=DIRECTION('',(0.781200482846104,0.,0.624280230025758));
#48267=DIRECTION('',(0.931242779705752,0.,-0.364399348580517));
#48268=DIRECTION('',(0.150042296859641,0.,-0.988679578606276));
#48269=DIRECTION('',(-0.781200482846105,0.,-0.624280230025758));
#48270=DIRECTION('',(-0.931242779705751,0.,0.364399348580519));
#48271=DIRECTION('',(-0.150042296859647,0.,0.988679578606275));
#48272=DIRECTION('',(0.781200482846104,0.,0.624280230025758));
#48273=DIRECTION('',(0.931242779705752,0.,-0.364399348580517));
#48274=DIRECTION('',(0.150042296859641,0.,-0.988679578606276));
#48275=DIRECTION('',(-0.781200482846105,0.,-0.624280230025758));
#48276=DIRECTION('',(-0.931242779705751,0.,0.364399348580519));
#48277=DIRECTION('',(-0.150042296859647,0.,0.988679578606275));
#48278=DIRECTION('',(0.781200482846104,0.,0.624280230025758));
#48279=DIRECTION('',(0.931242779705752,0.,-0.364399348580517));
#48280=DIRECTION('',(0.150042296859641,0.,-0.988679578606276));
#48281=DIRECTION('',(-0.781200482846105,0.,-0.624280230025758));
#48282=DIRECTION('',(-0.931242779705751,0.,0.364399348580519));
#48283=DIRECTION('',(-0.150042296859647,0.,0.988679578606275));
#48284=DIRECTION('',(0.781200482846104,0.,0.624280230025758));
#48285=DIRECTION('',(0.931242779705752,0.,-0.364399348580517));
#48286=DIRECTION('',(0.150042296859641,0.,-0.988679578606276));
#48287=DIRECTION('',(-0.781200482846105,0.,-0.624280230025758));
#48288=DIRECTION('',(-0.931242779705751,0.,0.364399348580519));
#48289=DIRECTION('',(-0.150042296859647,0.,0.988679578606275));
#48290=DIRECTION('',(0.781200482846104,0.,0.624280230025758));
#48291=DIRECTION('',(0.931242779705752,0.,-0.364399348580517));
#48292=DIRECTION('',(0.150042296859641,0.,-0.988679578606276));
#48293=DIRECTION('',(-0.781200482846105,0.,-0.624280230025758));
#48294=DIRECTION('',(-0.931242779705751,0.,0.364399348580519));
#48295=DIRECTION('',(-0.150042296859647,0.,0.988679578606275));
#48296=DIRECTION('',(0.781200482846104,0.,0.624280230025758));
#48297=DIRECTION('',(0.931242779705752,0.,-0.364399348580517));
#48298=DIRECTION('',(0.150042296859641,0.,-0.988679578606276));
#48299=DIRECTION('',(-0.781200482846105,0.,-0.624280230025758));
#48300=DIRECTION('',(-0.931242779705751,0.,0.364399348580519));
#48301=DIRECTION('',(-0.150042296859647,0.,0.988679578606275));
#48302=DIRECTION('',(0.781200482846104,0.,0.624280230025758));
#48303=DIRECTION('',(0.931242779705752,0.,-0.364399348580517));
#48304=DIRECTION('',(0.150042296859641,0.,-0.988679578606276));
#48305=DIRECTION('',(-0.781200482846105,0.,-0.624280230025758));
#48306=DIRECTION('',(-0.931242779705751,0.,0.364399348580519));
#48307=DIRECTION('',(-0.150042296859647,0.,0.988679578606275));
#48308=DIRECTION('',(0.781200482846104,0.,0.624280230025758));
#48309=DIRECTION('',(0.931242779705752,0.,-0.364399348580517));
#48310=DIRECTION('',(0.150042296859641,0.,-0.988679578606276));
#48311=DIRECTION('',(-0.781200482846105,0.,-0.624280230025758));
#48312=DIRECTION('',(-0.931242779705751,0.,0.364399348580519));
#48313=DIRECTION('',(-0.150042296859647,0.,0.988679578606275));
#48314=DIRECTION('',(0.781200482846104,0.,0.624280230025758));
#48315=DIRECTION('',(0.931242779705752,0.,-0.364399348580517));
#48316=DIRECTION('',(0.150042296859641,0.,-0.988679578606276));
#48317=DIRECTION('',(-0.781200482846105,0.,-0.624280230025758));
#48318=DIRECTION('',(-0.931242779705751,0.,0.364399348580519));
#48319=DIRECTION('',(-0.150042296859647,0.,0.988679578606275));
#48320=DIRECTION('',(0.781200482846104,0.,0.624280230025758));
#48321=DIRECTION('',(0.931242779705752,0.,-0.364399348580517));
#48322=DIRECTION('',(0.150042296859641,0.,-0.988679578606276));
#48323=DIRECTION('',(-0.781200482846105,0.,-0.624280230025758));
#48324=DIRECTION('',(-0.931242779705751,0.,0.364399348580519));
#48325=DIRECTION('',(-0.150042296859647,0.,0.988679578606275));
#48326=DIRECTION('',(0.781200482846104,0.,0.624280230025758));
#48327=DIRECTION('',(0.931242779705752,0.,-0.364399348580517));
#48328=DIRECTION('',(0.150042296859641,0.,-0.988679578606276));
#48329=DIRECTION('',(-0.781200482846105,0.,-0.624280230025758));
#48330=DIRECTION('',(-0.931242779705751,0.,0.364399348580519));
#48331=DIRECTION('',(-0.150042296859647,0.,0.988679578606275));
#48332=DIRECTION('',(0.781200482846104,0.,0.624280230025758));
#48333=DIRECTION('',(0.931242779705752,0.,-0.364399348580517));
#48334=DIRECTION('',(0.150042296859641,0.,-0.988679578606276));
#48335=DIRECTION('',(-0.781200482846105,0.,-0.624280230025758));
#48336=DIRECTION('',(-0.931242779705751,0.,0.364399348580519));
#48337=DIRECTION('',(-0.150042296859647,0.,0.988679578606275));
#48338=DIRECTION('',(0.781200482846104,0.,0.624280230025758));
#48339=DIRECTION('',(0.931242779705752,0.,-0.364399348580517));
#48340=DIRECTION('',(0.150042296859641,0.,-0.988679578606276));
#48341=DIRECTION('',(-0.781200482846105,0.,-0.624280230025758));
#48342=DIRECTION('',(-0.931242779705751,0.,0.364399348580519));
#48343=DIRECTION('',(-0.150042296859647,0.,0.988679578606275));
#48344=DIRECTION('',(0.781200482846104,0.,0.624280230025758));
#48345=DIRECTION('',(0.931242779705752,0.,-0.364399348580517));
#48346=DIRECTION('',(0.150042296859641,0.,-0.988679578606276));
#48347=DIRECTION('',(-0.781200482846105,0.,-0.624280230025758));
#48348=DIRECTION('',(-0.931242779705751,0.,0.364399348580519));
#48349=DIRECTION('',(-0.150042296859647,0.,0.988679578606275));
#48350=DIRECTION('',(0.781200482846104,0.,0.624280230025758));
#48351=DIRECTION('',(0.931242779705752,0.,-0.364399348580517));
#48352=DIRECTION('',(0.150042296859641,0.,-0.988679578606276));
#48353=DIRECTION('',(-0.781200482846105,0.,-0.624280230025758));
#48354=DIRECTION('',(-0.931242779705751,0.,0.364399348580519));
#48355=DIRECTION('',(-0.150042296859647,0.,0.988679578606275));
#48356=DIRECTION('',(0.781200482846104,0.,0.624280230025758));
#48357=DIRECTION('',(0.931242779705752,0.,-0.364399348580517));
#48358=DIRECTION('',(0.150042296859641,0.,-0.988679578606276));
#48359=DIRECTION('',(-0.781200482846105,0.,-0.624280230025758));
#48360=DIRECTION('',(-0.931242779705751,0.,0.364399348580519));
#48361=DIRECTION('',(-0.150042296859647,0.,0.988679578606275));
#48362=DIRECTION('',(0.781200482846104,0.,0.624280230025758));
#48363=DIRECTION('',(0.931242779705752,0.,-0.364399348580517));
#48364=DIRECTION('',(0.150042296859641,0.,-0.988679578606276));
#48365=DIRECTION('',(-0.781200482846105,0.,-0.624280230025758));
#48366=DIRECTION('',(-0.931242779705751,0.,0.364399348580519));
#48367=DIRECTION('',(-0.150042296859647,0.,0.988679578606275));
#48368=DIRECTION('',(0.781200482846104,0.,0.624280230025758));
#48369=DIRECTION('',(0.931242779705752,0.,-0.364399348580517));
#48370=DIRECTION('',(0.150042296859641,0.,-0.988679578606276));
#48371=DIRECTION('',(-0.781200482846105,0.,-0.624280230025758));
#48372=DIRECTION('',(-0.931242779705751,0.,0.364399348580519));
#48373=DIRECTION('',(-0.150042296859647,0.,0.988679578606275));
#48374=DIRECTION('',(0.781200482846104,0.,0.624280230025758));
#48375=DIRECTION('',(0.931242779705752,0.,-0.364399348580517));
#48376=DIRECTION('',(0.150042296859641,0.,-0.988679578606276));
#48377=DIRECTION('',(-0.781200482846105,0.,-0.624280230025758));
#48378=DIRECTION('',(-0.931242779705751,0.,0.364399348580519));
#48379=DIRECTION('',(-0.150042296859647,0.,0.988679578606275));
#48380=DIRECTION('',(0.781200482846104,0.,0.624280230025758));
#48381=DIRECTION('',(0.931242779705752,0.,-0.364399348580517));
#48382=DIRECTION('',(0.150042296859641,0.,-0.988679578606276));
#48383=DIRECTION('',(-0.781200482846105,0.,-0.624280230025758));
#48384=DIRECTION('',(-0.931242779705751,0.,0.364399348580519));
#48385=DIRECTION('',(-0.150042296859647,0.,0.988679578606275));
#48386=DIRECTION('',(0.781200482846104,0.,0.624280230025758));
#48387=DIRECTION('',(0.931242779705752,0.,-0.364399348580517));
#48388=DIRECTION('',(0.150042296859641,0.,-0.988679578606276));
#48389=DIRECTION('',(-0.781200482846105,0.,-0.624280230025758));
#48390=DIRECTION('',(-0.931242779705751,0.,0.364399348580519));
#48391=DIRECTION('',(-0.150042296859647,0.,0.988679578606275));
#48392=DIRECTION('',(0.781200482846104,0.,0.624280230025758));
#48393=DIRECTION('',(0.931242779705752,0.,-0.364399348580517));
#48394=DIRECTION('',(0.150042296859641,0.,-0.988679578606276));
#48395=DIRECTION('',(-0.781200482846105,0.,-0.624280230025758));
#48396=DIRECTION('',(-0.931242779705751,0.,0.364399348580519));
#48397=DIRECTION('',(-0.150042296859647,0.,0.988679578606275));
#48398=DIRECTION('',(0.781200482846104,0.,0.624280230025758));
#48399=DIRECTION('',(0.931242779705752,0.,-0.364399348580517));
#48400=DIRECTION('',(0.150042296859641,0.,-0.988679578606276));
#48401=DIRECTION('',(-0.781200482846105,0.,-0.624280230025758));
#48402=DIRECTION('',(-0.931242779705751,0.,0.364399348580519));
#48403=DIRECTION('',(-0.150042296859647,0.,0.988679578606275));
#48404=DIRECTION('',(0.781200482846104,0.,0.624280230025758));
#48405=DIRECTION('',(0.931242779705752,0.,-0.364399348580517));
#48406=DIRECTION('',(0.150042296859641,0.,-0.988679578606276));
#48407=DIRECTION('',(-0.781200482846105,0.,-0.624280230025758));
#48408=DIRECTION('',(-0.931242779705751,0.,0.364399348580519));
#48409=DIRECTION('',(-0.150042296859647,0.,0.988679578606275));
#48410=DIRECTION('',(0.781200482846104,0.,0.624280230025758));
#48411=DIRECTION('',(0.931242779705752,0.,-0.364399348580517));
#48412=DIRECTION('',(0.150042296859641,0.,-0.988679578606276));
#48413=DIRECTION('',(-0.781200482846105,0.,-0.624280230025758));
#48414=DIRECTION('',(-0.931242779705751,0.,0.364399348580519));
#48415=DIRECTION('',(-0.150042296859647,0.,0.988679578606275));
#48416=DIRECTION('',(0.781200482846104,0.,0.624280230025758));
#48417=DIRECTION('',(0.931242779705752,0.,-0.364399348580517));
#48418=DIRECTION('',(0.150042296859641,0.,-0.988679578606276));
#48419=DIRECTION('',(-0.781200482846105,0.,-0.624280230025758));
#48420=DIRECTION('',(-0.931242779705751,0.,0.364399348580519));
#48421=DIRECTION('',(-0.150042296859647,0.,0.988679578606275));
#48422=DIRECTION('',(0.781200482846104,0.,0.624280230025758));
#48423=DIRECTION('',(0.931242779705752,0.,-0.364399348580517));
#48424=DIRECTION('',(0.150042296859641,0.,-0.988679578606276));
#48425=DIRECTION('',(-0.781200482846105,0.,-0.624280230025758));
#48426=DIRECTION('',(-0.931242779705751,0.,0.364399348580519));
#48427=DIRECTION('',(-0.150042296859647,0.,0.988679578606275));
#48428=DIRECTION('',(0.781200482846104,0.,0.624280230025758));
#48429=DIRECTION('',(0.931242779705752,0.,-0.364399348580517));
#48430=DIRECTION('',(0.150042296859641,0.,-0.988679578606276));
#48431=DIRECTION('',(-0.781200482846105,0.,-0.624280230025758));
#48432=DIRECTION('',(-0.931242779705751,0.,0.364399348580519));
#48433=DIRECTION('',(-0.150042296859647,0.,0.988679578606275));
#48434=DIRECTION('',(0.781200482846104,0.,0.624280230025758));
#48435=DIRECTION('',(0.931242779705752,0.,-0.364399348580517));
#48436=DIRECTION('',(0.150042296859641,0.,-0.988679578606276));
#48437=DIRECTION('',(-0.781200482846105,0.,-0.624280230025758));
#48438=DIRECTION('',(-0.931242779705751,0.,0.364399348580519));
#48439=DIRECTION('',(-0.150042296859647,0.,0.988679578606275));
#48440=DIRECTION('',(0.781200482846104,0.,0.624280230025758));
#48441=DIRECTION('',(0.931242779705752,0.,-0.364399348580517));
#48442=DIRECTION('',(0.150042296859641,0.,-0.988679578606276));
#48443=DIRECTION('',(-0.781200482846105,0.,-0.624280230025758));
#48444=DIRECTION('',(-0.931242779705751,0.,0.364399348580519));
#48445=DIRECTION('',(-0.150042296859647,0.,0.988679578606275));
#48446=DIRECTION('',(0.781200482846104,0.,0.624280230025758));
#48447=DIRECTION('',(0.931242779705752,0.,-0.364399348580517));
#48448=DIRECTION('',(0.150042296859641,0.,-0.988679578606276));
#48449=DIRECTION('',(-0.781200482846105,0.,-0.624280230025758));
#48450=DIRECTION('',(-0.931242779705751,0.,0.364399348580519));
#48451=DIRECTION('',(-0.150042296859647,0.,0.988679578606275));
#48452=DIRECTION('',(0.781200482846104,0.,0.624280230025758));
#48453=DIRECTION('',(0.931242779705752,0.,-0.364399348580517));
#48454=DIRECTION('',(0.150042296859641,0.,-0.988679578606276));
#48455=DIRECTION('',(-0.781200482846105,0.,-0.624280230025758));
#48456=DIRECTION('',(-0.931242779705751,0.,0.364399348580519));
#48457=DIRECTION('',(-0.150042296859647,0.,0.988679578606275));
#48458=DIRECTION('',(0.781200482846104,0.,0.624280230025758));
#48459=DIRECTION('',(0.931242779705752,0.,-0.364399348580517));
#48460=DIRECTION('',(0.150042296859641,0.,-0.988679578606276));
#48461=DIRECTION('',(-0.781200482846105,0.,-0.624280230025758));
#48462=DIRECTION('',(-0.931242779705751,0.,0.364399348580519));
#48463=DIRECTION('',(-0.150042296859647,0.,0.988679578606275));
#48464=DIRECTION('',(0.781200482846104,0.,0.624280230025758));
#48465=DIRECTION('',(0.931242779705752,0.,-0.364399348580517));
#48466=DIRECTION('',(0.150042296859641,0.,-0.988679578606276));
#48467=DIRECTION('',(-0.781200482846105,0.,-0.624280230025758));
#48468=DIRECTION('',(-0.931242779705751,0.,0.364399348580519));
#48469=DIRECTION('',(-0.150042296859647,0.,0.988679578606275));
#48470=DIRECTION('',(0.781200482846104,0.,0.624280230025758));
#48471=DIRECTION('',(0.931242779705752,0.,-0.364399348580517));
#48472=DIRECTION('',(0.150042296859641,0.,-0.988679578606276));
#48473=DIRECTION('',(-0.781200482846105,0.,-0.624280230025758));
#48474=DIRECTION('',(-0.931242779705751,0.,0.364399348580519));
#48475=DIRECTION('',(-0.150042296859647,0.,0.988679578606275));
#48476=DIRECTION('',(0.781200482846104,0.,0.624280230025758));
#48477=DIRECTION('',(0.931242779705752,0.,-0.364399348580517));
#48478=DIRECTION('',(0.150042296859641,0.,-0.988679578606276));
#48479=DIRECTION('',(-0.781200482846105,0.,-0.624280230025758));
#48480=DIRECTION('',(-0.931242779705751,0.,0.364399348580519));
#48481=DIRECTION('',(-0.150042296859647,0.,0.988679578606275));
#48482=DIRECTION('',(0.781200482846104,0.,0.624280230025758));
#48483=DIRECTION('',(0.931242779705752,0.,-0.364399348580517));
#48484=DIRECTION('',(0.150042296859641,0.,-0.988679578606276));
#48485=DIRECTION('',(-0.781200482846105,0.,-0.624280230025758));
#48486=DIRECTION('',(-0.931242779705751,0.,0.364399348580519));
#48487=DIRECTION('',(-0.150042296859647,0.,0.988679578606275));
#48488=DIRECTION('',(0.781200482846104,0.,0.624280230025758));
#48489=DIRECTION('',(0.931242779705752,0.,-0.364399348580517));
#48490=DIRECTION('',(0.150042296859641,0.,-0.988679578606276));
#48491=DIRECTION('',(-0.781200482846105,0.,-0.624280230025758));
#48492=DIRECTION('',(-0.931242779705751,0.,0.364399348580519));
#48493=DIRECTION('',(-0.150042296859647,0.,0.988679578606275));
#48494=DIRECTION('',(0.781200482846104,0.,0.624280230025758));
#48495=DIRECTION('',(0.931242779705752,0.,-0.364399348580517));
#48496=DIRECTION('',(0.150042296859641,0.,-0.988679578606276));
#48497=DIRECTION('',(-0.781200482846105,0.,-0.624280230025758));
#48498=DIRECTION('',(-0.931242779705751,0.,0.364399348580519));
#48499=DIRECTION('',(-0.150042296859647,0.,0.988679578606275));
#48500=DIRECTION('',(0.781200482846104,0.,0.624280230025758));
#48501=DIRECTION('',(0.931242779705752,0.,-0.364399348580517));
#48502=DIRECTION('',(0.150042296859641,0.,-0.988679578606276));
#48503=DIRECTION('',(-0.781200482846105,0.,-0.624280230025758));
#48504=DIRECTION('',(-0.931242779705751,0.,0.364399348580519));
#48505=DIRECTION('',(-0.150042296859647,0.,0.988679578606275));
#48506=DIRECTION('',(0.781200482846104,0.,0.624280230025758));
#48507=DIRECTION('',(0.931242779705752,0.,-0.364399348580517));
#48508=DIRECTION('',(0.150042296859641,0.,-0.988679578606276));
#48509=DIRECTION('',(-0.781200482846105,0.,-0.624280230025758));
#48510=DIRECTION('',(-0.931242779705751,0.,0.364399348580519));
#48511=DIRECTION('',(-0.150042296859647,0.,0.988679578606275));
#48512=DIRECTION('',(0.781200482846104,0.,0.624280230025758));
#48513=DIRECTION('',(0.931242779705752,0.,-0.364399348580517));
#48514=DIRECTION('',(0.150042296859641,0.,-0.988679578606276));
#48515=DIRECTION('',(-0.781200482846105,0.,-0.624280230025758));
#48516=DIRECTION('',(-0.931242779705751,0.,0.364399348580519));
#48517=DIRECTION('',(-0.150042296859647,0.,0.988679578606275));
#48518=DIRECTION('',(0.781200482846104,0.,0.624280230025758));
#48519=DIRECTION('',(0.931242779705752,0.,-0.364399348580517));
#48520=DIRECTION('',(0.150042296859641,0.,-0.988679578606276));
#48521=DIRECTION('',(-0.781200482846105,0.,-0.624280230025758));
#48522=DIRECTION('',(-0.931242779705751,0.,0.364399348580519));
#48523=DIRECTION('',(-0.150042296859647,0.,0.988679578606275));
#48524=DIRECTION('',(0.781200482846104,0.,0.624280230025758));
#48525=DIRECTION('',(0.931242779705752,0.,-0.364399348580517));
#48526=DIRECTION('',(0.150042296859641,0.,-0.988679578606276));
#48527=DIRECTION('',(-0.781200482846105,0.,-0.624280230025758));
#48528=DIRECTION('',(-0.931242779705751,0.,0.364399348580519));
#48529=DIRECTION('',(-0.150042296859647,0.,0.988679578606275));
#48530=DIRECTION('',(0.781200482846104,0.,0.624280230025758));
#48531=DIRECTION('',(0.931242779705752,0.,-0.364399348580517));
#48532=DIRECTION('',(0.150042296859641,0.,-0.988679578606276));
#48533=DIRECTION('',(-0.781200482846105,0.,-0.624280230025758));
#48534=DIRECTION('',(-0.931242779705751,0.,0.364399348580519));
#48535=DIRECTION('',(-0.150042296859647,0.,0.988679578606275));
#48536=DIRECTION('',(0.781200482846104,0.,0.624280230025758));
#48537=DIRECTION('',(0.931242779705752,0.,-0.364399348580517));
#48538=DIRECTION('',(0.150042296859641,0.,-0.988679578606276));
#48539=DIRECTION('',(-0.781200482846105,0.,-0.624280230025758));
#48540=DIRECTION('',(-0.931242779705751,0.,0.364399348580519));
#48541=DIRECTION('',(-0.150042296859647,0.,0.988679578606275));
#48542=DIRECTION('',(0.781200482846104,0.,0.624280230025758));
#48543=DIRECTION('',(0.931242779705752,0.,-0.364399348580517));
#48544=DIRECTION('',(0.150042296859641,0.,-0.988679578606276));
#48545=DIRECTION('',(-0.781200482846105,0.,-0.624280230025758));
#48546=DIRECTION('',(-0.931242779705751,0.,0.364399348580519));
#48547=DIRECTION('',(-0.150042296859647,0.,0.988679578606275));
#48548=DIRECTION('',(0.781200482846104,0.,0.624280230025758));
#48549=DIRECTION('',(0.931242779705752,0.,-0.364399348580517));
#48550=DIRECTION('',(0.150042296859641,0.,-0.988679578606276));
#48551=DIRECTION('',(-0.781200482846105,0.,-0.624280230025758));
#48552=DIRECTION('',(-0.931242779705751,0.,0.364399348580519));
#48553=DIRECTION('',(-0.150042296859647,0.,0.988679578606275));
#48554=DIRECTION('',(0.781200482846104,0.,0.624280230025758));
#48555=DIRECTION('',(0.931242779705752,0.,-0.364399348580517));
#48556=DIRECTION('',(0.150042296859641,0.,-0.988679578606276));
#48557=DIRECTION('',(-0.781200482846105,0.,-0.624280230025758));
#48558=DIRECTION('',(-0.931242779705751,0.,0.364399348580519));
#48559=DIRECTION('',(-0.150042296859647,0.,0.988679578606275));
#48560=DIRECTION('',(0.781200482846104,0.,0.624280230025758));
#48561=DIRECTION('',(0.931242779705752,0.,-0.364399348580517));
#48562=DIRECTION('',(0.150042296859641,0.,-0.988679578606276));
#48563=DIRECTION('',(-0.781200482846105,0.,-0.624280230025758));
#48564=DIRECTION('',(-0.931242779705751,0.,0.364399348580519));
#48565=DIRECTION('',(-0.150042296859647,0.,0.988679578606275));
#48566=DIRECTION('',(0.781200482846104,0.,0.624280230025758));
#48567=DIRECTION('',(0.931242779705752,0.,-0.364399348580517));
#48568=DIRECTION('',(0.150042296859641,0.,-0.988679578606276));
#48569=DIRECTION('',(-0.781200482846105,0.,-0.624280230025758));
#48570=DIRECTION('',(-0.931242779705751,0.,0.364399348580519));
#48571=DIRECTION('',(-0.150042296859647,0.,0.988679578606275));
#48572=DIRECTION('',(0.781200482846104,0.,0.624280230025758));
#48573=DIRECTION('',(0.931242779705752,0.,-0.364399348580517));
#48574=DIRECTION('',(0.150042296859641,0.,-0.988679578606276));
#48575=DIRECTION('',(-0.781200482846105,0.,-0.624280230025758));
#48576=DIRECTION('',(-0.931242779705751,0.,0.364399348580519));
#48577=DIRECTION('',(-0.150042296859647,0.,0.988679578606275));
#48578=DIRECTION('',(0.781200482846104,0.,0.624280230025758));
#48579=DIRECTION('',(0.931242779705752,0.,-0.364399348580517));
#48580=DIRECTION('',(0.150042296859641,0.,-0.988679578606276));
#48581=DIRECTION('',(-0.781200482846105,0.,-0.624280230025758));
#48582=DIRECTION('',(-0.931242779705751,0.,0.364399348580519));
#48583=DIRECTION('',(-0.150042296859647,0.,0.988679578606275));
#48584=DIRECTION('',(0.781200482846104,0.,0.624280230025758));
#48585=DIRECTION('',(0.931242779705752,0.,-0.364399348580517));
#48586=DIRECTION('',(0.150042296859641,0.,-0.988679578606276));
#48587=DIRECTION('',(-0.781200482846105,0.,-0.624280230025758));
#48588=DIRECTION('',(-0.931242779705751,0.,0.364399348580519));
#48589=DIRECTION('',(-0.150042296859647,0.,0.988679578606275));
#48590=DIRECTION('',(0.781200482846104,0.,0.624280230025758));
#48591=DIRECTION('',(0.931242779705752,0.,-0.364399348580517));
#48592=DIRECTION('',(0.150042296859641,0.,-0.988679578606276));
#48593=DIRECTION('',(-0.781200482846105,0.,-0.624280230025758));
#48594=DIRECTION('',(-0.931242779705751,0.,0.364399348580519));
#48595=DIRECTION('',(-0.150042296859647,0.,0.988679578606275));
#48596=DIRECTION('',(0.781200482846104,0.,0.624280230025758));
#48597=DIRECTION('',(0.931242779705752,0.,-0.364399348580517));
#48598=DIRECTION('',(0.150042296859641,0.,-0.988679578606276));
#48599=DIRECTION('',(-0.781200482846105,0.,-0.624280230025758));
#48600=DIRECTION('',(-0.931242779705751,0.,0.364399348580519));
#48601=DIRECTION('',(-0.150042296859647,0.,0.988679578606275));
#48602=DIRECTION('',(0.781200482846104,0.,0.624280230025758));
#48603=DIRECTION('',(0.931242779705752,0.,-0.364399348580517));
#48604=DIRECTION('',(0.150042296859641,0.,-0.988679578606276));
#48605=DIRECTION('',(-0.781200482846105,0.,-0.624280230025758));
#48606=DIRECTION('',(-0.931242779705751,0.,0.364399348580519));
#48607=DIRECTION('',(-0.150042296859647,0.,0.988679578606275));
#48608=DIRECTION('',(0.781200482846104,0.,0.624280230025758));
#48609=DIRECTION('',(0.931242779705752,0.,-0.364399348580517));
#48610=DIRECTION('',(0.150042296859641,0.,-0.988679578606276));
#48611=DIRECTION('',(-0.781200482846105,0.,-0.624280230025758));
#48612=DIRECTION('',(-0.931242779705751,0.,0.364399348580519));
#48613=DIRECTION('',(-0.150042296859647,0.,0.988679578606275));
#48614=DIRECTION('',(0.781200482846104,0.,0.624280230025758));
#48615=DIRECTION('',(0.931242779705752,0.,-0.364399348580517));
#48616=DIRECTION('',(0.150042296859641,0.,-0.988679578606276));
#48617=DIRECTION('',(-0.781200482846105,0.,-0.624280230025758));
#48618=DIRECTION('',(-0.931242779705751,0.,0.364399348580519));
#48619=DIRECTION('',(-0.150042296859647,0.,0.988679578606275));
#48620=DIRECTION('',(0.781200482846104,0.,0.624280230025758));
#48621=DIRECTION('',(0.931242779705752,0.,-0.364399348580517));
#48622=DIRECTION('',(0.150042296859641,0.,-0.988679578606276));
#48623=DIRECTION('',(-0.781200482846105,0.,-0.624280230025758));
#48624=DIRECTION('',(-0.931242779705751,0.,0.364399348580519));
#48625=DIRECTION('',(-0.150042296859647,0.,0.988679578606275));
#48626=DIRECTION('',(0.781200482846104,0.,0.624280230025758));
#48627=DIRECTION('',(0.931242779705752,0.,-0.364399348580517));
#48628=DIRECTION('',(0.150042296859641,0.,-0.988679578606276));
#48629=DIRECTION('',(-0.781200482846105,0.,-0.624280230025758));
#48630=DIRECTION('',(-0.931242779705751,0.,0.364399348580519));
#48631=DIRECTION('',(-0.150042296859647,0.,0.988679578606275));
#48632=DIRECTION('',(0.781200482846104,0.,0.624280230025758));
#48633=DIRECTION('',(0.931242779705752,0.,-0.364399348580517));
#48634=DIRECTION('',(0.150042296859641,0.,-0.988679578606276));
#48635=DIRECTION('',(-0.781200482846105,0.,-0.624280230025758));
#48636=DIRECTION('',(-0.931242779705751,0.,0.364399348580519));
#48637=DIRECTION('',(-0.150042296859647,0.,0.988679578606275));
#48638=DIRECTION('',(0.781200482846104,0.,0.624280230025758));
#48639=DIRECTION('',(0.931242779705752,0.,-0.364399348580517));
#48640=DIRECTION('',(0.150042296859641,0.,-0.988679578606276));
#48641=DIRECTION('',(-0.781200482846105,0.,-0.624280230025758));
#48642=DIRECTION('',(-0.931242779705751,0.,0.364399348580519));
#48643=DIRECTION('',(-0.150042296859647,0.,0.988679578606275));
#48644=DIRECTION('',(0.781200482846104,0.,0.624280230025758));
#48645=DIRECTION('',(0.931242779705752,0.,-0.364399348580517));
#48646=DIRECTION('',(0.150042296859641,0.,-0.988679578606276));
#48647=DIRECTION('',(-0.781200482846105,0.,-0.624280230025758));
#48648=DIRECTION('',(-0.931242779705751,0.,0.364399348580519));
#48649=DIRECTION('',(-0.150042296859647,0.,0.988679578606275));
#48650=DIRECTION('',(0.781200482846104,0.,0.624280230025758));
#48651=DIRECTION('',(0.931242779705752,0.,-0.364399348580517));
#48652=DIRECTION('',(0.150042296859641,0.,-0.988679578606276));
#48653=DIRECTION('',(-0.781200482846105,0.,-0.624280230025758));
#48654=DIRECTION('',(-0.931242779705751,0.,0.364399348580519));
#48655=DIRECTION('',(-0.150042296859647,0.,0.988679578606275));
#48656=DIRECTION('',(0.781200482846104,0.,0.624280230025758));
#48657=DIRECTION('',(0.931242779705752,0.,-0.364399348580517));
#48658=DIRECTION('',(0.150042296859641,0.,-0.988679578606276));
#48659=DIRECTION('',(-0.781200482846105,0.,-0.624280230025758));
#48660=DIRECTION('',(-0.931242779705751,0.,0.364399348580519));
#48661=DIRECTION('',(-0.150042296859647,0.,0.988679578606275));
#48662=DIRECTION('',(0.781200482846104,0.,0.624280230025758));
#48663=DIRECTION('',(0.931242779705752,0.,-0.364399348580517));
#48664=DIRECTION('',(0.150042296859641,0.,-0.988679578606276));
#48665=DIRECTION('',(-0.781200482846105,0.,-0.624280230025758));
#48666=DIRECTION('',(-0.931242779705751,0.,0.364399348580519));
#48667=DIRECTION('',(-0.150042296859647,0.,0.988679578606275));
#48668=DIRECTION('',(0.781200482846104,0.,0.624280230025758));
#48669=DIRECTION('',(0.931242779705752,0.,-0.364399348580517));
#48670=DIRECTION('',(0.150042296859641,0.,-0.988679578606276));
#48671=DIRECTION('',(-0.781200482846105,0.,-0.624280230025758));
#48672=DIRECTION('',(-0.931242779705751,0.,0.364399348580519));
#48673=DIRECTION('',(-0.150042296859647,0.,0.988679578606275));
#48674=DIRECTION('',(0.781200482846104,0.,0.624280230025758));
#48675=DIRECTION('',(0.931242779705752,0.,-0.364399348580517));
#48676=DIRECTION('',(0.150042296859641,0.,-0.988679578606276));
#48677=DIRECTION('',(-0.781200482846105,0.,-0.624280230025758));
#48678=DIRECTION('',(-0.931242779705751,0.,0.364399348580519));
#48679=DIRECTION('',(-0.150042296859647,0.,0.988679578606275));
#48680=DIRECTION('',(0.781200482846104,0.,0.624280230025758));
#48681=DIRECTION('',(0.931242779705752,0.,-0.364399348580517));
#48682=DIRECTION('',(0.150042296859641,0.,-0.988679578606276));
#48683=DIRECTION('',(-0.781200482846105,0.,-0.624280230025758));
#48684=DIRECTION('',(-0.931242779705751,0.,0.364399348580519));
#48685=DIRECTION('',(-0.150042296859647,0.,0.988679578606275));
#48686=DIRECTION('',(0.781200482846104,0.,0.624280230025758));
#48687=DIRECTION('',(0.931242779705752,0.,-0.364399348580517));
#48688=DIRECTION('',(0.150042296859641,0.,-0.988679578606276));
#48689=DIRECTION('',(-0.781200482846105,0.,-0.624280230025758));
#48690=DIRECTION('',(-0.931242779705751,0.,0.364399348580519));
#48691=DIRECTION('',(-0.150042296859647,0.,0.988679578606275));
#48692=DIRECTION('',(0.781200482846104,0.,0.624280230025758));
#48693=DIRECTION('',(0.931242779705752,0.,-0.364399348580517));
#48694=DIRECTION('',(0.150042296859641,0.,-0.988679578606276));
#48695=DIRECTION('',(-0.781200482846105,0.,-0.624280230025758));
#48696=DIRECTION('',(-0.931242779705751,0.,0.364399348580519));
#48697=DIRECTION('',(-0.150042296859647,0.,0.988679578606275));
#48698=DIRECTION('',(0.781200482846104,0.,0.624280230025758));
#48699=DIRECTION('',(0.931242779705752,0.,-0.364399348580517));
#48700=DIRECTION('',(0.150042296859641,0.,-0.988679578606276));
#48701=DIRECTION('',(-0.781200482846105,0.,-0.624280230025758));
#48702=DIRECTION('',(-0.931242779705751,0.,0.364399348580519));
#48703=DIRECTION('',(-0.150042296859647,0.,0.988679578606275));
#48704=DIRECTION('',(0.781200482846104,0.,0.624280230025758));
#48705=DIRECTION('',(0.931242779705752,0.,-0.364399348580517));
#48706=DIRECTION('',(0.150042296859641,0.,-0.988679578606276));
#48707=DIRECTION('',(-0.781200482846105,0.,-0.624280230025758));
#48708=DIRECTION('',(-0.931242779705751,0.,0.364399348580519));
#48709=DIRECTION('',(-0.150042296859647,0.,0.988679578606275));
#48710=DIRECTION('',(0.781200482846104,0.,0.624280230025758));
#48711=DIRECTION('',(0.931242779705752,0.,-0.364399348580517));
#48712=DIRECTION('',(0.150042296859641,0.,-0.988679578606276));
#48713=DIRECTION('',(-0.781200482846105,0.,-0.624280230025758));
#48714=DIRECTION('',(-0.931242779705751,0.,0.364399348580519));
#48715=DIRECTION('',(-0.150042296859647,0.,0.988679578606275));
#48716=DIRECTION('',(0.781200482846104,0.,0.624280230025758));
#48717=DIRECTION('',(0.931242779705752,0.,-0.364399348580517));
#48718=DIRECTION('',(0.150042296859641,0.,-0.988679578606276));
#48719=DIRECTION('',(-0.781200482846105,0.,-0.624280230025758));
#48720=DIRECTION('',(-0.931242779705751,0.,0.364399348580519));
#48721=DIRECTION('',(-0.150042296859647,0.,0.988679578606275));
#48722=DIRECTION('',(0.781200482846104,0.,0.624280230025758));
#48723=DIRECTION('',(0.931242779705752,0.,-0.364399348580517));
#48724=DIRECTION('',(0.150042296859641,0.,-0.988679578606276));
#48725=DIRECTION('',(-0.781200482846105,0.,-0.624280230025758));
#48726=DIRECTION('',(-0.931242779705751,0.,0.364399348580519));
#48727=DIRECTION('',(-0.150042296859647,0.,0.988679578606275));
#48728=DIRECTION('',(0.781200482846104,0.,0.624280230025758));
#48729=DIRECTION('',(0.931242779705752,0.,-0.364399348580517));
#48730=DIRECTION('',(0.150042296859641,0.,-0.988679578606276));
#48731=DIRECTION('',(-0.781200482846105,0.,-0.624280230025758));
#48732=DIRECTION('',(-0.931242779705751,0.,0.364399348580519));
#48733=DIRECTION('',(-0.150042296859647,0.,0.988679578606275));
#48734=DIRECTION('',(0.781200482846104,0.,0.624280230025758));
#48735=DIRECTION('',(0.931242779705752,0.,-0.364399348580517));
#48736=DIRECTION('',(0.150042296859641,0.,-0.988679578606276));
#48737=DIRECTION('',(-0.781200482846105,0.,-0.624280230025758));
#48738=DIRECTION('',(-0.931242779705751,0.,0.364399348580519));
#48739=DIRECTION('',(-0.150042296859647,0.,0.988679578606275));
#48740=DIRECTION('',(0.781200482846104,0.,0.624280230025758));
#48741=DIRECTION('',(0.931242779705752,0.,-0.364399348580517));
#48742=DIRECTION('',(0.150042296859641,0.,-0.988679578606276));
#48743=DIRECTION('',(-0.781200482846105,0.,-0.624280230025758));
#48744=DIRECTION('',(-0.931242779705751,0.,0.364399348580519));
#48745=DIRECTION('',(-0.150042296859647,0.,0.988679578606275));
#48746=DIRECTION('',(0.781200482846104,0.,0.624280230025758));
#48747=DIRECTION('',(0.931242779705752,0.,-0.364399348580517));
#48748=DIRECTION('',(0.150042296859641,0.,-0.988679578606276));
#48749=DIRECTION('',(-0.781200482846105,0.,-0.624280230025758));
#48750=DIRECTION('',(-0.931242779705751,0.,0.364399348580519));
#48751=DIRECTION('',(-0.150042296859647,0.,0.988679578606275));
#48752=DIRECTION('',(0.781200482846104,0.,0.624280230025758));
#48753=DIRECTION('',(0.931242779705752,0.,-0.364399348580517));
#48754=DIRECTION('',(0.150042296859641,0.,-0.988679578606276));
#48755=DIRECTION('',(-0.781200482846105,0.,-0.624280230025758));
#48756=DIRECTION('',(-0.931242779705751,0.,0.364399348580519));
#48757=DIRECTION('',(-0.150042296859647,0.,0.988679578606275));
#48758=DIRECTION('',(0.781200482846104,0.,0.624280230025758));
#48759=DIRECTION('',(0.931242779705752,0.,-0.364399348580517));
#48760=DIRECTION('',(0.150042296859641,0.,-0.988679578606276));
#48761=DIRECTION('',(-0.781200482846105,0.,-0.624280230025758));
#48762=DIRECTION('',(-0.931242779705751,0.,0.364399348580519));
#48763=DIRECTION('',(-0.150042296859647,0.,0.988679578606275));
#48764=DIRECTION('',(0.781200482846104,0.,0.624280230025758));
#48765=DIRECTION('',(0.931242779705752,0.,-0.364399348580517));
#48766=DIRECTION('',(0.150042296859641,0.,-0.988679578606276));
#48767=DIRECTION('',(-0.781200482846105,0.,-0.624280230025758));
#48768=DIRECTION('',(-0.931242779705751,0.,0.364399348580519));
#48769=DIRECTION('',(-0.150042296859647,0.,0.988679578606275));
#48770=DIRECTION('',(0.781200482846104,0.,0.624280230025758));
#48771=DIRECTION('',(0.931242779705752,0.,-0.364399348580517));
#48772=DIRECTION('',(0.150042296859641,0.,-0.988679578606276));
#48773=DIRECTION('',(-0.781200482846105,0.,-0.624280230025758));
#48774=DIRECTION('',(-0.931242779705751,0.,0.364399348580519));
#48775=DIRECTION('',(-0.150042296859647,0.,0.988679578606275));
#48776=DIRECTION('',(0.781200482846104,0.,0.624280230025758));
#48777=DIRECTION('',(0.931242779705752,0.,-0.364399348580517));
#48778=DIRECTION('',(0.150042296859641,0.,-0.988679578606276));
#48779=DIRECTION('',(-0.781200482846105,0.,-0.624280230025758));
#48780=DIRECTION('',(-0.931242779705751,0.,0.364399348580519));
#48781=DIRECTION('',(-0.150042296859647,0.,0.988679578606275));
#48782=DIRECTION('',(0.781200482846104,0.,0.624280230025758));
#48783=DIRECTION('',(0.931242779705752,0.,-0.364399348580517));
#48784=DIRECTION('',(0.150042296859641,0.,-0.988679578606276));
#48785=DIRECTION('',(-0.781200482846105,0.,-0.624280230025758));
#48786=DIRECTION('',(-0.931242779705751,0.,0.364399348580519));
#48787=DIRECTION('',(-0.150042296859647,0.,0.988679578606275));
#48788=DIRECTION('',(0.781200482846104,0.,0.624280230025758));
#48789=DIRECTION('',(0.931242779705752,0.,-0.364399348580517));
#48790=DIRECTION('',(0.150042296859641,0.,-0.988679578606276));
#48791=DIRECTION('',(-0.781200482846105,0.,-0.624280230025758));
#48792=DIRECTION('',(-0.931242779705751,0.,0.364399348580519));
#48793=DIRECTION('',(-0.150042296859647,0.,0.988679578606275));
#48794=DIRECTION('',(0.781200482846104,0.,0.624280230025758));
#48795=DIRECTION('',(0.931242779705752,0.,-0.364399348580517));
#48796=DIRECTION('',(0.150042296859641,0.,-0.988679578606276));
#48797=DIRECTION('',(-0.781200482846105,0.,-0.624280230025758));
#48798=DIRECTION('',(-0.931242779705751,0.,0.364399348580519));
#48799=DIRECTION('',(-0.150042296859647,0.,0.988679578606275));
#48800=DIRECTION('',(0.781200482846104,0.,0.624280230025758));
#48801=DIRECTION('',(0.931242779705752,0.,-0.364399348580517));
#48802=DIRECTION('',(0.150042296859641,0.,-0.988679578606276));
#48803=DIRECTION('',(-0.781200482846105,0.,-0.624280230025758));
#48804=DIRECTION('',(-0.931242779705751,0.,0.364399348580519));
#48805=DIRECTION('',(-0.150042296859647,0.,0.988679578606275));
#48806=DIRECTION('',(0.781200482846104,0.,0.624280230025758));
#48807=DIRECTION('',(0.931242779705752,0.,-0.364399348580517));
#48808=DIRECTION('',(0.150042296859641,0.,-0.988679578606276));
#48809=DIRECTION('',(-0.781200482846105,0.,-0.624280230025758));
#48810=DIRECTION('',(-0.931242779705751,0.,0.364399348580519));
#48811=DIRECTION('',(-0.150042296859647,0.,0.988679578606275));
#48812=DIRECTION('',(0.781200482846104,0.,0.624280230025758));
#48813=DIRECTION('',(0.931242779705752,0.,-0.364399348580517));
#48814=DIRECTION('',(0.150042296859641,0.,-0.988679578606276));
#48815=DIRECTION('',(-0.781200482846105,0.,-0.624280230025758));
#48816=DIRECTION('',(-0.931242779705751,0.,0.364399348580519));
#48817=DIRECTION('',(-0.150042296859647,0.,0.988679578606275));
#48818=DIRECTION('',(0.781200482846104,0.,0.624280230025758));
#48819=DIRECTION('',(0.931242779705752,0.,-0.364399348580517));
#48820=DIRECTION('',(0.150042296859641,0.,-0.988679578606276));
#48821=DIRECTION('',(-0.781200482846105,0.,-0.624280230025758));
#48822=DIRECTION('',(-0.931242779705751,0.,0.364399348580519));
#48823=DIRECTION('',(-0.150042296859647,0.,0.988679578606275));
#48824=DIRECTION('',(0.781200482846104,0.,0.624280230025758));
#48825=DIRECTION('',(0.931242779705752,0.,-0.364399348580517));
#48826=DIRECTION('',(0.150042296859641,0.,-0.988679578606276));
#48827=DIRECTION('',(-0.781200482846105,0.,-0.624280230025758));
#48828=DIRECTION('',(-0.931242779705751,0.,0.364399348580519));
#48829=DIRECTION('',(-0.150042296859647,0.,0.988679578606275));
#48830=DIRECTION('',(0.781200482846104,0.,0.624280230025758));
#48831=DIRECTION('',(0.931242779705752,0.,-0.364399348580517));
#48832=DIRECTION('',(0.150042296859641,0.,-0.988679578606276));
#48833=DIRECTION('',(-0.781200482846105,0.,-0.624280230025758));
#48834=DIRECTION('',(-0.931242779705751,0.,0.364399348580519));
#48835=DIRECTION('',(-0.150042296859647,0.,0.988679578606275));
#48836=DIRECTION('',(0.781200482846104,0.,0.624280230025758));
#48837=DIRECTION('',(0.931242779705752,0.,-0.364399348580517));
#48838=DIRECTION('',(0.150042296859641,0.,-0.988679578606276));
#48839=DIRECTION('',(-0.781200482846105,0.,-0.624280230025758));
#48840=DIRECTION('',(-0.931242779705751,0.,0.364399348580519));
#48841=DIRECTION('',(-0.150042296859647,0.,0.988679578606275));
#48842=DIRECTION('',(0.781200482846104,0.,0.624280230025758));
#48843=DIRECTION('',(0.931242779705752,0.,-0.364399348580517));
#48844=DIRECTION('',(0.150042296859641,0.,-0.988679578606276));
#48845=DIRECTION('',(-0.781200482846105,0.,-0.624280230025758));
#48846=DIRECTION('',(-0.931242779705751,0.,0.364399348580519));
#48847=DIRECTION('',(-0.150042296859647,0.,0.988679578606275));
#48848=DIRECTION('',(0.781200482846104,0.,0.624280230025758));
#48849=DIRECTION('',(0.931242779705752,0.,-0.364399348580517));
#48850=DIRECTION('',(0.150042296859641,0.,-0.988679578606276));
#48851=DIRECTION('',(-0.781200482846105,0.,-0.624280230025758));
#48852=DIRECTION('',(-0.931242779705751,0.,0.364399348580519));
#48853=DIRECTION('',(-0.150042296859647,0.,0.988679578606275));
#48854=DIRECTION('',(0.781200482846104,0.,0.624280230025758));
#48855=DIRECTION('',(0.931242779705752,0.,-0.364399348580517));
#48856=DIRECTION('',(0.150042296859641,0.,-0.988679578606276));
#48857=DIRECTION('',(-0.781200482846105,0.,-0.624280230025758));
#48858=DIRECTION('',(-0.931242779705751,0.,0.364399348580519));
#48859=DIRECTION('',(-0.150042296859647,0.,0.988679578606275));
#48860=DIRECTION('',(0.781200482846104,0.,0.624280230025758));
#48861=DIRECTION('',(0.931242779705752,0.,-0.364399348580517));
#48862=DIRECTION('',(0.150042296859641,0.,-0.988679578606276));
#48863=DIRECTION('',(-0.781200482846105,0.,-0.624280230025758));
#48864=DIRECTION('',(-0.931242779705751,0.,0.364399348580519));
#48865=DIRECTION('',(-0.150042296859647,0.,0.988679578606275));
#48866=DIRECTION('',(0.781200482846104,0.,0.624280230025758));
#48867=DIRECTION('',(0.931242779705752,0.,-0.364399348580517));
#48868=DIRECTION('',(0.150042296859641,0.,-0.988679578606276));
#48869=DIRECTION('',(-0.781200482846105,0.,-0.624280230025758));
#48870=DIRECTION('',(-0.931242779705751,0.,0.364399348580519));
#48871=DIRECTION('',(-0.150042296859647,0.,0.988679578606275));
#48872=DIRECTION('',(0.781200482846104,0.,0.624280230025758));
#48873=DIRECTION('',(0.931242779705752,0.,-0.364399348580517));
#48874=DIRECTION('',(0.150042296859641,0.,-0.988679578606276));
#48875=DIRECTION('',(-0.781200482846105,0.,-0.624280230025758));
#48876=DIRECTION('',(-0.931242779705751,0.,0.364399348580519));
#48877=DIRECTION('',(-0.150042296859647,0.,0.988679578606275));
#48878=DIRECTION('',(0.781200482846104,0.,0.624280230025758));
#48879=DIRECTION('',(0.931242779705752,0.,-0.364399348580517));
#48880=DIRECTION('',(0.150042296859641,0.,-0.988679578606276));
#48881=DIRECTION('',(-0.781200482846105,0.,-0.624280230025758));
#48882=DIRECTION('',(-0.931242779705751,0.,0.364399348580519));
#48883=DIRECTION('',(-0.150042296859647,0.,0.988679578606275));
#48884=DIRECTION('',(0.781200482846104,0.,0.624280230025758));
#48885=DIRECTION('',(0.931242779705752,0.,-0.364399348580517));
#48886=DIRECTION('',(0.150042296859641,0.,-0.988679578606276));
#48887=DIRECTION('',(-0.781200482846105,0.,-0.624280230025758));
#48888=DIRECTION('',(-0.931242779705751,0.,0.364399348580519));
#48889=DIRECTION('',(-0.150042296859647,0.,0.988679578606275));
#48890=DIRECTION('',(0.781200482846104,0.,0.624280230025758));
#48891=DIRECTION('',(0.931242779705752,0.,-0.364399348580517));
#48892=DIRECTION('',(0.150042296859641,0.,-0.988679578606276));
#48893=DIRECTION('',(-0.781200482846105,0.,-0.624280230025758));
#48894=DIRECTION('',(-0.931242779705751,0.,0.364399348580519));
#48895=DIRECTION('',(-0.150042296859647,0.,0.988679578606275));
#48896=DIRECTION('',(0.781200482846104,0.,0.624280230025758));
#48897=DIRECTION('',(0.931242779705752,0.,-0.364399348580517));
#48898=DIRECTION('',(0.150042296859641,0.,-0.988679578606276));
#48899=DIRECTION('',(-0.781200482846105,0.,-0.624280230025758));
#48900=DIRECTION('',(-0.931242779705751,0.,0.364399348580519));
#48901=DIRECTION('',(-0.150042296859647,0.,0.988679578606275));
#48902=DIRECTION('',(0.781200482846104,0.,0.624280230025758));
#48903=DIRECTION('',(0.931242779705752,0.,-0.364399348580517));
#48904=DIRECTION('',(0.150042296859641,0.,-0.988679578606276));
#48905=DIRECTION('',(-0.781200482846105,0.,-0.624280230025758));
#48906=DIRECTION('',(-0.931242779705751,0.,0.364399348580519));
#48907=DIRECTION('',(-0.150042296859647,0.,0.988679578606275));
#48908=DIRECTION('',(0.781200482846104,0.,0.624280230025758));
#48909=DIRECTION('',(0.931242779705752,0.,-0.364399348580517));
#48910=DIRECTION('',(0.150042296859641,0.,-0.988679578606276));
#48911=DIRECTION('',(-0.781200482846105,0.,-0.624280230025758));
#48912=DIRECTION('',(-0.931242779705751,0.,0.364399348580519));
#48913=DIRECTION('',(-0.150042296859647,0.,0.988679578606275));
#48914=DIRECTION('',(0.781200482846104,0.,0.624280230025758));
#48915=DIRECTION('',(0.931242779705752,0.,-0.364399348580517));
#48916=DIRECTION('',(0.150042296859641,0.,-0.988679578606276));
#48917=DIRECTION('',(-0.781200482846105,0.,-0.624280230025758));
#48918=DIRECTION('',(-0.931242779705751,0.,0.364399348580519));
#48919=DIRECTION('',(-0.150042296859647,0.,0.988679578606275));
#48920=DIRECTION('',(0.781200482846104,0.,0.624280230025758));
#48921=DIRECTION('',(0.931242779705752,0.,-0.364399348580517));
#48922=DIRECTION('',(0.150042296859641,0.,-0.988679578606276));
#48923=DIRECTION('',(-0.781200482846105,0.,-0.624280230025758));
#48924=DIRECTION('',(-0.931242779705751,0.,0.364399348580519));
#48925=DIRECTION('',(-0.150042296859647,0.,0.988679578606275));
#48926=DIRECTION('',(0.781200482846104,0.,0.624280230025758));
#48927=DIRECTION('',(0.931242779705752,0.,-0.364399348580517));
#48928=DIRECTION('',(0.150042296859641,0.,-0.988679578606276));
#48929=DIRECTION('',(-0.781200482846105,0.,-0.624280230025758));
#48930=DIRECTION('',(-0.931242779705751,0.,0.364399348580519));
#48931=DIRECTION('',(-0.150042296859647,0.,0.988679578606275));
#48932=DIRECTION('',(0.781200482846104,0.,0.624280230025758));
#48933=DIRECTION('',(0.931242779705752,0.,-0.364399348580517));
#48934=DIRECTION('',(0.150042296859641,0.,-0.988679578606276));
#48935=DIRECTION('',(-0.781200482846105,0.,-0.624280230025758));
#48936=DIRECTION('',(-0.931242779705751,0.,0.364399348580519));
#48937=DIRECTION('',(-0.150042296859647,0.,0.988679578606275));
#48938=DIRECTION('',(0.781200482846104,0.,0.624280230025758));
#48939=DIRECTION('',(0.931242779705752,0.,-0.364399348580517));
#48940=DIRECTION('',(0.150042296859641,0.,-0.988679578606276));
#48941=DIRECTION('',(-0.781200482846105,0.,-0.624280230025758));
#48942=DIRECTION('',(-0.931242779705751,0.,0.364399348580519));
#48943=DIRECTION('',(-0.150042296859647,0.,0.988679578606275));
#48944=DIRECTION('',(0.781200482846104,0.,0.624280230025758));
#48945=DIRECTION('',(0.931242779705752,0.,-0.364399348580517));
#48946=DIRECTION('',(0.150042296859641,0.,-0.988679578606276));
#48947=DIRECTION('',(-0.781200482846105,0.,-0.624280230025758));
#48948=DIRECTION('',(-0.931242779705751,0.,0.364399348580519));
#48949=DIRECTION('',(-0.150042296859647,0.,0.988679578606275));
#48950=DIRECTION('',(0.781200482846104,0.,0.624280230025758));
#48951=DIRECTION('',(0.931242779705752,0.,-0.364399348580517));
#48952=DIRECTION('',(0.150042296859641,0.,-0.988679578606276));
#48953=DIRECTION('',(-0.781200482846105,0.,-0.624280230025758));
#48954=DIRECTION('',(-0.931242779705751,0.,0.364399348580519));
#48955=DIRECTION('',(-0.150042296859647,0.,0.988679578606275));
#48956=DIRECTION('',(0.781200482846104,0.,0.624280230025758));
#48957=DIRECTION('',(0.931242779705752,0.,-0.364399348580517));
#48958=DIRECTION('',(0.150042296859641,0.,-0.988679578606276));
#48959=DIRECTION('',(-0.781200482846105,0.,-0.624280230025758));
#48960=DIRECTION('',(-0.931242779705751,0.,0.364399348580519));
#48961=DIRECTION('',(-0.150042296859647,0.,0.988679578606275));
#48962=DIRECTION('',(0.781200482846104,0.,0.624280230025758));
#48963=DIRECTION('',(0.931242779705752,0.,-0.364399348580517));
#48964=DIRECTION('',(0.150042296859641,0.,-0.988679578606276));
#48965=DIRECTION('',(-0.781200482846105,0.,-0.624280230025758));
#48966=DIRECTION('',(-0.931242779705751,0.,0.364399348580519));
#48967=DIRECTION('',(-0.150042296859647,0.,0.988679578606275));
#48968=DIRECTION('',(0.781200482846104,0.,0.624280230025758));
#48969=DIRECTION('',(0.931242779705752,0.,-0.364399348580517));
#48970=DIRECTION('',(0.150042296859641,0.,-0.988679578606276));
#48971=DIRECTION('',(-0.781200482846105,0.,-0.624280230025758));
#48972=DIRECTION('',(-0.931242779705751,0.,0.364399348580519));
#48973=DIRECTION('',(-0.150042296859647,0.,0.988679578606275));
#48974=DIRECTION('',(0.781200482846104,0.,0.624280230025758));
#48975=DIRECTION('',(0.931242779705752,0.,-0.364399348580517));
#48976=DIRECTION('',(0.150042296859641,0.,-0.988679578606276));
#48977=DIRECTION('',(-0.781200482846105,0.,-0.624280230025758));
#48978=DIRECTION('',(-0.931242779705751,0.,0.364399348580519));
#48979=DIRECTION('',(-0.150042296859647,0.,0.988679578606275));
#48980=DIRECTION('',(0.781200482846104,0.,0.624280230025758));
#48981=DIRECTION('',(0.931242779705752,0.,-0.364399348580517));
#48982=DIRECTION('',(0.150042296859641,0.,-0.988679578606276));
#48983=DIRECTION('',(-0.781200482846105,0.,-0.624280230025758));
#48984=DIRECTION('',(-0.931242779705751,0.,0.364399348580519));
#48985=DIRECTION('',(-0.150042296859647,0.,0.988679578606275));
#48986=DIRECTION('',(0.781200482846104,0.,0.624280230025758));
#48987=DIRECTION('',(0.931242779705752,0.,-0.364399348580517));
#48988=DIRECTION('',(0.150042296859641,0.,-0.988679578606276));
#48989=DIRECTION('',(-0.781200482846105,0.,-0.624280230025758));
#48990=DIRECTION('',(-0.931242779705751,0.,0.364399348580519));
#48991=DIRECTION('',(-0.150042296859647,0.,0.988679578606275));
#48992=DIRECTION('',(0.781200482846104,0.,0.624280230025758));
#48993=DIRECTION('',(0.931242779705752,0.,-0.364399348580517));
#48994=DIRECTION('',(0.150042296859641,0.,-0.988679578606276));
#48995=DIRECTION('',(-0.781200482846105,0.,-0.624280230025758));
#48996=DIRECTION('',(-0.931242779705751,0.,0.364399348580519));
#48997=DIRECTION('',(-0.150042296859647,0.,0.988679578606275));
#48998=DIRECTION('',(0.781200482846104,0.,0.624280230025758));
#48999=DIRECTION('',(0.931242779705752,0.,-0.364399348580517));
#49000=DIRECTION('',(0.150042296859641,0.,-0.988679578606276));
#49001=DIRECTION('',(-0.781200482846105,0.,-0.624280230025758));
#49002=DIRECTION('',(-0.931242779705751,0.,0.364399348580519));
#49003=DIRECTION('',(-0.150042296859647,0.,0.988679578606275));
#49004=DIRECTION('',(0.781200482846104,0.,0.624280230025758));
#49005=DIRECTION('',(0.931242779705752,0.,-0.364399348580517));
#49006=DIRECTION('',(0.150042296859641,0.,-0.988679578606276));
#49007=DIRECTION('',(-0.781200482846105,0.,-0.624280230025758));
#49008=DIRECTION('',(-0.931242779705751,0.,0.364399348580519));
#49009=DIRECTION('',(-0.150042296859647,0.,0.988679578606275));
#49010=DIRECTION('',(0.781200482846104,0.,0.624280230025758));
#49011=DIRECTION('',(0.931242779705752,0.,-0.364399348580517));
#49012=DIRECTION('',(0.150042296859641,0.,-0.988679578606276));
#49013=DIRECTION('',(-0.781200482846105,0.,-0.624280230025758));
#49014=DIRECTION('',(-0.931242779705751,0.,0.364399348580519));
#49015=DIRECTION('',(-0.150042296859647,0.,0.988679578606275));
#49016=DIRECTION('',(0.781200482846104,0.,0.624280230025758));
#49017=DIRECTION('',(0.931242779705752,0.,-0.364399348580517));
#49018=DIRECTION('',(0.150042296859641,0.,-0.988679578606276));
#49019=DIRECTION('',(-0.781200482846105,0.,-0.624280230025758));
#49020=DIRECTION('',(-0.931242779705751,0.,0.364399348580519));
#49021=DIRECTION('',(-0.150042296859647,0.,0.988679578606275));
#49022=DIRECTION('',(0.781200482846104,0.,0.624280230025758));
#49023=DIRECTION('',(0.931242779705752,0.,-0.364399348580517));
#49024=DIRECTION('',(0.150042296859641,0.,-0.988679578606276));
#49025=DIRECTION('',(-0.781200482846105,0.,-0.624280230025758));
#49026=DIRECTION('',(-0.931242779705751,0.,0.364399348580519));
#49027=DIRECTION('',(-0.150042296859647,0.,0.988679578606275));
#49028=DIRECTION('',(0.781200482846104,0.,0.624280230025758));
#49029=DIRECTION('',(0.931242779705752,0.,-0.364399348580517));
#49030=DIRECTION('',(0.150042296859641,0.,-0.988679578606276));
#49031=DIRECTION('',(-0.781200482846105,0.,-0.624280230025758));
#49032=DIRECTION('',(-0.931242779705751,0.,0.364399348580519));
#49033=DIRECTION('',(-0.150042296859647,0.,0.988679578606275));
#49034=DIRECTION('',(0.781200482846104,0.,0.624280230025758));
#49035=DIRECTION('',(0.931242779705752,0.,-0.364399348580517));
#49036=DIRECTION('',(0.150042296859641,0.,-0.988679578606276));
#49037=DIRECTION('',(-0.781200482846105,0.,-0.624280230025758));
#49038=DIRECTION('',(-0.931242779705751,0.,0.364399348580519));
#49039=DIRECTION('',(-0.150042296859647,0.,0.988679578606275));
#49040=DIRECTION('',(0.781200482846104,0.,0.624280230025758));
#49041=DIRECTION('',(0.931242779705752,0.,-0.364399348580517));
#49042=DIRECTION('',(0.150042296859641,0.,-0.988679578606276));
#49043=DIRECTION('',(-0.781200482846105,0.,-0.624280230025758));
#49044=DIRECTION('',(-0.931242779705751,0.,0.364399348580519));
#49045=DIRECTION('',(-0.150042296859647,0.,0.988679578606275));
#49046=DIRECTION('',(0.781200482846104,0.,0.624280230025758));
#49047=DIRECTION('',(0.931242779705752,0.,-0.364399348580517));
#49048=DIRECTION('',(0.150042296859641,0.,-0.988679578606276));
#49049=DIRECTION('',(-0.781200482846105,0.,-0.624280230025758));
#49050=DIRECTION('',(-0.931242779705751,0.,0.364399348580519));
#49051=DIRECTION('',(-0.150042296859647,0.,0.988679578606275));
#49052=DIRECTION('',(0.781200482846104,0.,0.624280230025758));
#49053=DIRECTION('',(0.931242779705752,0.,-0.364399348580517));
#49054=DIRECTION('',(0.150042296859641,0.,-0.988679578606276));
#49055=DIRECTION('',(-0.781200482846105,0.,-0.624280230025758));
#49056=DIRECTION('',(-0.931242779705751,0.,0.364399348580519));
#49057=DIRECTION('',(-0.150042296859647,0.,0.988679578606275));
#49058=DIRECTION('',(0.781200482846104,0.,0.624280230025758));
#49059=DIRECTION('',(0.931242779705752,0.,-0.364399348580517));
#49060=DIRECTION('',(0.150042296859641,0.,-0.988679578606276));
#49061=DIRECTION('',(-0.781200482846105,0.,-0.624280230025758));
#49062=DIRECTION('',(-0.931242779705751,0.,0.364399348580519));
#49063=DIRECTION('',(-0.150042296859647,0.,0.988679578606275));
#49064=DIRECTION('',(0.781200482846104,0.,0.624280230025758));
#49065=DIRECTION('',(0.931242779705752,0.,-0.364399348580517));
#49066=DIRECTION('',(0.150042296859641,0.,-0.988679578606276));
#49067=DIRECTION('',(-0.781200482846105,0.,-0.624280230025758));
#49068=DIRECTION('',(-0.931242779705751,0.,0.364399348580519));
#49069=DIRECTION('',(-0.150042296859647,0.,0.988679578606275));
#49070=DIRECTION('',(0.781200482846104,0.,0.624280230025758));
#49071=DIRECTION('',(0.931242779705752,0.,-0.364399348580517));
#49072=DIRECTION('',(0.150042296859641,0.,-0.988679578606276));
#49073=DIRECTION('',(-0.781200482846105,0.,-0.624280230025758));
#49074=DIRECTION('',(-0.931242779705751,0.,0.364399348580519));
#49075=DIRECTION('',(-0.150042296859647,0.,0.988679578606275));
#49076=DIRECTION('',(0.781200482846104,0.,0.624280230025758));
#49077=DIRECTION('',(0.931242779705752,0.,-0.364399348580517));
#49078=DIRECTION('',(0.150042296859641,0.,-0.988679578606276));
#49079=DIRECTION('',(-0.781200482846105,0.,-0.624280230025758));
#49080=DIRECTION('',(-0.931242779705751,0.,0.364399348580519));
#49081=DIRECTION('',(-0.150042296859647,0.,0.988679578606275));
#49082=DIRECTION('',(0.781200482846104,0.,0.624280230025758));
#49083=DIRECTION('',(0.931242779705752,0.,-0.364399348580517));
#49084=DIRECTION('',(0.150042296859641,0.,-0.988679578606276));
#49085=DIRECTION('',(-0.781200482846105,0.,-0.624280230025758));
#49086=DIRECTION('',(-0.931242779705751,0.,0.364399348580519));
#49087=DIRECTION('',(-0.150042296859647,0.,0.988679578606275));
#49088=DIRECTION('',(0.781200482846104,0.,0.624280230025758));
#49089=DIRECTION('',(0.931242779705752,0.,-0.364399348580517));
#49090=DIRECTION('',(0.150042296859641,0.,-0.988679578606276));
#49091=DIRECTION('',(-0.781200482846105,0.,-0.624280230025758));
#49092=DIRECTION('',(-0.931242779705751,0.,0.364399348580519));
#49093=DIRECTION('',(-0.150042296859647,0.,0.988679578606275));
#49094=DIRECTION('',(0.781200482846104,0.,0.624280230025758));
#49095=DIRECTION('center_axis',(0.988679578606276,0.,0.150042296859641));
#49096=DIRECTION('ref_axis',(0.150042296859641,0.,-0.988679578606276));
#49097=DIRECTION('',(0.,1.,0.));
#49098=DIRECTION('',(0.,1.,0.));
#49099=DIRECTION('center_axis',(0.364399348580517,0.,0.931242779705752));
#49100=DIRECTION('ref_axis',(0.931242779705752,0.,-0.364399348580517));
#49101=DIRECTION('',(0.,1.,0.));
#49102=DIRECTION('center_axis',(-0.624280230025758,0.,0.781200482846104));
#49103=DIRECTION('ref_axis',(0.781200482846104,0.,0.624280230025758));
#49104=DIRECTION('',(0.,1.,0.));
#49105=DIRECTION('center_axis',(-0.988679578606275,0.,-0.150042296859647));
#49106=DIRECTION('ref_axis',(-0.150042296859647,0.,0.988679578606275));
#49107=DIRECTION('',(0.,1.,0.));
#49108=DIRECTION('center_axis',(-0.364399348580519,0.,-0.931242779705751));
#49109=DIRECTION('ref_axis',(-0.931242779705751,0.,0.364399348580519));
#49110=DIRECTION('',(0.,1.,0.));
#49111=DIRECTION('center_axis',(0.624280230025758,0.,-0.781200482846105));
#49112=DIRECTION('ref_axis',(-0.781200482846105,0.,-0.624280230025758));
#49113=DIRECTION('center_axis',(0.988679578606276,0.,0.150042296859641));
#49114=DIRECTION('ref_axis',(0.150042296859641,0.,-0.988679578606276));
#49115=DIRECTION('',(0.,1.,0.));
#49116=DIRECTION('',(0.,1.,0.));
#49117=DIRECTION('center_axis',(0.364399348580517,0.,0.931242779705752));
#49118=DIRECTION('ref_axis',(0.931242779705752,0.,-0.364399348580517));
#49119=DIRECTION('',(0.,1.,0.));
#49120=DIRECTION('center_axis',(-0.624280230025758,0.,0.781200482846104));
#49121=DIRECTION('ref_axis',(0.781200482846104,0.,0.624280230025758));
#49122=DIRECTION('',(0.,1.,0.));
#49123=DIRECTION('center_axis',(-0.988679578606275,0.,-0.150042296859647));
#49124=DIRECTION('ref_axis',(-0.150042296859647,0.,0.988679578606275));
#49125=DIRECTION('',(0.,1.,0.));
#49126=DIRECTION('center_axis',(-0.364399348580519,0.,-0.931242779705751));
#49127=DIRECTION('ref_axis',(-0.931242779705751,0.,0.364399348580519));
#49128=DIRECTION('',(0.,1.,0.));
#49129=DIRECTION('center_axis',(0.624280230025758,0.,-0.781200482846105));
#49130=DIRECTION('ref_axis',(-0.781200482846105,0.,-0.624280230025758));
#49131=DIRECTION('center_axis',(0.988679578606276,0.,0.150042296859641));
#49132=DIRECTION('ref_axis',(0.150042296859641,0.,-0.988679578606276));
#49133=DIRECTION('',(0.,1.,0.));
#49134=DIRECTION('',(0.,1.,0.));
#49135=DIRECTION('center_axis',(0.364399348580517,0.,0.931242779705752));
#49136=DIRECTION('ref_axis',(0.931242779705752,0.,-0.364399348580517));
#49137=DIRECTION('',(0.,1.,0.));
#49138=DIRECTION('center_axis',(-0.624280230025758,0.,0.781200482846104));
#49139=DIRECTION('ref_axis',(0.781200482846104,0.,0.624280230025758));
#49140=DIRECTION('',(0.,1.,0.));
#49141=DIRECTION('center_axis',(-0.988679578606275,0.,-0.150042296859647));
#49142=DIRECTION('ref_axis',(-0.150042296859647,0.,0.988679578606275));
#49143=DIRECTION('',(0.,1.,0.));
#49144=DIRECTION('center_axis',(-0.364399348580519,0.,-0.931242779705751));
#49145=DIRECTION('ref_axis',(-0.931242779705751,0.,0.364399348580519));
#49146=DIRECTION('',(0.,1.,0.));
#49147=DIRECTION('center_axis',(0.624280230025758,0.,-0.781200482846105));
#49148=DIRECTION('ref_axis',(-0.781200482846105,0.,-0.624280230025758));
#49149=DIRECTION('center_axis',(0.988679578606276,0.,0.150042296859641));
#49150=DIRECTION('ref_axis',(0.150042296859641,0.,-0.988679578606276));
#49151=DIRECTION('',(0.,1.,0.));
#49152=DIRECTION('',(0.,1.,0.));
#49153=DIRECTION('center_axis',(0.364399348580517,0.,0.931242779705752));
#49154=DIRECTION('ref_axis',(0.931242779705752,0.,-0.364399348580517));
#49155=DIRECTION('',(0.,1.,0.));
#49156=DIRECTION('center_axis',(-0.624280230025758,0.,0.781200482846104));
#49157=DIRECTION('ref_axis',(0.781200482846104,0.,0.624280230025758));
#49158=DIRECTION('',(0.,1.,0.));
#49159=DIRECTION('center_axis',(-0.988679578606275,0.,-0.150042296859647));
#49160=DIRECTION('ref_axis',(-0.150042296859647,0.,0.988679578606275));
#49161=DIRECTION('',(0.,1.,0.));
#49162=DIRECTION('center_axis',(-0.364399348580519,0.,-0.931242779705751));
#49163=DIRECTION('ref_axis',(-0.931242779705751,0.,0.364399348580519));
#49164=DIRECTION('',(0.,1.,0.));
#49165=DIRECTION('center_axis',(0.624280230025758,0.,-0.781200482846105));
#49166=DIRECTION('ref_axis',(-0.781200482846105,0.,-0.624280230025758));
#49167=DIRECTION('center_axis',(0.988679578606276,0.,0.150042296859641));
#49168=DIRECTION('ref_axis',(0.150042296859641,0.,-0.988679578606276));
#49169=DIRECTION('',(0.,1.,0.));
#49170=DIRECTION('',(0.,1.,0.));
#49171=DIRECTION('center_axis',(0.364399348580517,0.,0.931242779705752));
#49172=DIRECTION('ref_axis',(0.931242779705752,0.,-0.364399348580517));
#49173=DIRECTION('',(0.,1.,0.));
#49174=DIRECTION('center_axis',(-0.624280230025758,0.,0.781200482846104));
#49175=DIRECTION('ref_axis',(0.781200482846104,0.,0.624280230025758));
#49176=DIRECTION('',(0.,1.,0.));
#49177=DIRECTION('center_axis',(-0.988679578606275,0.,-0.150042296859647));
#49178=DIRECTION('ref_axis',(-0.150042296859647,0.,0.988679578606275));
#49179=DIRECTION('',(0.,1.,0.));
#49180=DIRECTION('center_axis',(-0.364399348580519,0.,-0.931242779705751));
#49181=DIRECTION('ref_axis',(-0.931242779705751,0.,0.364399348580519));
#49182=DIRECTION('',(0.,1.,0.));
#49183=DIRECTION('center_axis',(0.624280230025758,0.,-0.781200482846105));
#49184=DIRECTION('ref_axis',(-0.781200482846105,0.,-0.624280230025758));
#49185=DIRECTION('center_axis',(0.988679578606276,0.,0.150042296859641));
#49186=DIRECTION('ref_axis',(0.150042296859641,0.,-0.988679578606276));
#49187=DIRECTION('',(0.,1.,0.));
#49188=DIRECTION('',(0.,1.,0.));
#49189=DIRECTION('center_axis',(0.364399348580517,0.,0.931242779705752));
#49190=DIRECTION('ref_axis',(0.931242779705752,0.,-0.364399348580517));
#49191=DIRECTION('',(0.,1.,0.));
#49192=DIRECTION('center_axis',(-0.624280230025758,0.,0.781200482846104));
#49193=DIRECTION('ref_axis',(0.781200482846104,0.,0.624280230025758));
#49194=DIRECTION('',(0.,1.,0.));
#49195=DIRECTION('center_axis',(-0.988679578606275,0.,-0.150042296859647));
#49196=DIRECTION('ref_axis',(-0.150042296859647,0.,0.988679578606275));
#49197=DIRECTION('',(0.,1.,0.));
#49198=DIRECTION('center_axis',(-0.364399348580519,0.,-0.931242779705751));
#49199=DIRECTION('ref_axis',(-0.931242779705751,0.,0.364399348580519));
#49200=DIRECTION('',(0.,1.,0.));
#49201=DIRECTION('center_axis',(0.624280230025758,0.,-0.781200482846105));
#49202=DIRECTION('ref_axis',(-0.781200482846105,0.,-0.624280230025758));
#49203=DIRECTION('center_axis',(0.988679578606276,0.,0.150042296859641));
#49204=DIRECTION('ref_axis',(0.150042296859641,0.,-0.988679578606276));
#49205=DIRECTION('',(0.,1.,0.));
#49206=DIRECTION('',(0.,1.,0.));
#49207=DIRECTION('center_axis',(0.364399348580517,0.,0.931242779705752));
#49208=DIRECTION('ref_axis',(0.931242779705752,0.,-0.364399348580517));
#49209=DIRECTION('',(0.,1.,0.));
#49210=DIRECTION('center_axis',(-0.624280230025758,0.,0.781200482846104));
#49211=DIRECTION('ref_axis',(0.781200482846104,0.,0.624280230025758));
#49212=DIRECTION('',(0.,1.,0.));
#49213=DIRECTION('center_axis',(-0.988679578606275,0.,-0.150042296859647));
#49214=DIRECTION('ref_axis',(-0.150042296859647,0.,0.988679578606275));
#49215=DIRECTION('',(0.,1.,0.));
#49216=DIRECTION('center_axis',(-0.364399348580519,0.,-0.931242779705751));
#49217=DIRECTION('ref_axis',(-0.931242779705751,0.,0.364399348580519));
#49218=DIRECTION('',(0.,1.,0.));
#49219=DIRECTION('center_axis',(0.624280230025758,0.,-0.781200482846105));
#49220=DIRECTION('ref_axis',(-0.781200482846105,0.,-0.624280230025758));
#49221=DIRECTION('center_axis',(0.988679578606276,0.,0.150042296859641));
#49222=DIRECTION('ref_axis',(0.150042296859641,0.,-0.988679578606276));
#49223=DIRECTION('',(0.,1.,0.));
#49224=DIRECTION('',(0.,1.,0.));
#49225=DIRECTION('center_axis',(0.364399348580517,0.,0.931242779705752));
#49226=DIRECTION('ref_axis',(0.931242779705752,0.,-0.364399348580517));
#49227=DIRECTION('',(0.,1.,0.));
#49228=DIRECTION('center_axis',(-0.624280230025758,0.,0.781200482846104));
#49229=DIRECTION('ref_axis',(0.781200482846104,0.,0.624280230025758));
#49230=DIRECTION('',(0.,1.,0.));
#49231=DIRECTION('center_axis',(-0.988679578606275,0.,-0.150042296859647));
#49232=DIRECTION('ref_axis',(-0.150042296859647,0.,0.988679578606275));
#49233=DIRECTION('',(0.,1.,0.));
#49234=DIRECTION('center_axis',(-0.364399348580519,0.,-0.931242779705751));
#49235=DIRECTION('ref_axis',(-0.931242779705751,0.,0.364399348580519));
#49236=DIRECTION('',(0.,1.,0.));
#49237=DIRECTION('center_axis',(0.624280230025758,0.,-0.781200482846105));
#49238=DIRECTION('ref_axis',(-0.781200482846105,0.,-0.624280230025758));
#49239=DIRECTION('center_axis',(0.988679578606276,0.,0.150042296859641));
#49240=DIRECTION('ref_axis',(0.150042296859641,0.,-0.988679578606276));
#49241=DIRECTION('',(0.,1.,0.));
#49242=DIRECTION('',(0.,1.,0.));
#49243=DIRECTION('center_axis',(0.364399348580517,0.,0.931242779705752));
#49244=DIRECTION('ref_axis',(0.931242779705752,0.,-0.364399348580517));
#49245=DIRECTION('',(0.,1.,0.));
#49246=DIRECTION('center_axis',(-0.624280230025758,0.,0.781200482846104));
#49247=DIRECTION('ref_axis',(0.781200482846104,0.,0.624280230025758));
#49248=DIRECTION('',(0.,1.,0.));
#49249=DIRECTION('center_axis',(-0.988679578606275,0.,-0.150042296859647));
#49250=DIRECTION('ref_axis',(-0.150042296859647,0.,0.988679578606275));
#49251=DIRECTION('',(0.,1.,0.));
#49252=DIRECTION('center_axis',(-0.364399348580519,0.,-0.931242779705751));
#49253=DIRECTION('ref_axis',(-0.931242779705751,0.,0.364399348580519));
#49254=DIRECTION('',(0.,1.,0.));
#49255=DIRECTION('center_axis',(0.624280230025758,0.,-0.781200482846105));
#49256=DIRECTION('ref_axis',(-0.781200482846105,0.,-0.624280230025758));
#49257=DIRECTION('center_axis',(0.988679578606276,0.,0.150042296859641));
#49258=DIRECTION('ref_axis',(0.150042296859641,0.,-0.988679578606276));
#49259=DIRECTION('',(0.,1.,0.));
#49260=DIRECTION('',(0.,1.,0.));
#49261=DIRECTION('center_axis',(0.364399348580517,0.,0.931242779705752));
#49262=DIRECTION('ref_axis',(0.931242779705752,0.,-0.364399348580517));
#49263=DIRECTION('',(0.,1.,0.));
#49264=DIRECTION('center_axis',(-0.624280230025758,0.,0.781200482846104));
#49265=DIRECTION('ref_axis',(0.781200482846104,0.,0.624280230025758));
#49266=DIRECTION('',(0.,1.,0.));
#49267=DIRECTION('center_axis',(-0.988679578606275,0.,-0.150042296859647));
#49268=DIRECTION('ref_axis',(-0.150042296859647,0.,0.988679578606275));
#49269=DIRECTION('',(0.,1.,0.));
#49270=DIRECTION('center_axis',(-0.364399348580519,0.,-0.931242779705751));
#49271=DIRECTION('ref_axis',(-0.931242779705751,0.,0.364399348580519));
#49272=DIRECTION('',(0.,1.,0.));
#49273=DIRECTION('center_axis',(0.624280230025758,0.,-0.781200482846105));
#49274=DIRECTION('ref_axis',(-0.781200482846105,0.,-0.624280230025758));
#49275=DIRECTION('center_axis',(0.988679578606276,0.,0.150042296859641));
#49276=DIRECTION('ref_axis',(0.150042296859641,0.,-0.988679578606276));
#49277=DIRECTION('',(0.,1.,0.));
#49278=DIRECTION('',(0.,1.,0.));
#49279=DIRECTION('center_axis',(0.364399348580517,0.,0.931242779705752));
#49280=DIRECTION('ref_axis',(0.931242779705752,0.,-0.364399348580517));
#49281=DIRECTION('',(0.,1.,0.));
#49282=DIRECTION('center_axis',(-0.624280230025758,0.,0.781200482846104));
#49283=DIRECTION('ref_axis',(0.781200482846104,0.,0.624280230025758));
#49284=DIRECTION('',(0.,1.,0.));
#49285=DIRECTION('center_axis',(-0.988679578606275,0.,-0.150042296859647));
#49286=DIRECTION('ref_axis',(-0.150042296859647,0.,0.988679578606275));
#49287=DIRECTION('',(0.,1.,0.));
#49288=DIRECTION('center_axis',(-0.364399348580519,0.,-0.931242779705751));
#49289=DIRECTION('ref_axis',(-0.931242779705751,0.,0.364399348580519));
#49290=DIRECTION('',(0.,1.,0.));
#49291=DIRECTION('center_axis',(0.624280230025758,0.,-0.781200482846105));
#49292=DIRECTION('ref_axis',(-0.781200482846105,0.,-0.624280230025758));
#49293=DIRECTION('center_axis',(0.988679578606276,0.,0.150042296859641));
#49294=DIRECTION('ref_axis',(0.150042296859641,0.,-0.988679578606276));
#49295=DIRECTION('',(0.,1.,0.));
#49296=DIRECTION('',(0.,1.,0.));
#49297=DIRECTION('center_axis',(0.364399348580517,0.,0.931242779705752));
#49298=DIRECTION('ref_axis',(0.931242779705752,0.,-0.364399348580517));
#49299=DIRECTION('',(0.,1.,0.));
#49300=DIRECTION('center_axis',(-0.624280230025758,0.,0.781200482846104));
#49301=DIRECTION('ref_axis',(0.781200482846104,0.,0.624280230025758));
#49302=DIRECTION('',(0.,1.,0.));
#49303=DIRECTION('center_axis',(-0.988679578606275,0.,-0.150042296859647));
#49304=DIRECTION('ref_axis',(-0.150042296859647,0.,0.988679578606275));
#49305=DIRECTION('',(0.,1.,0.));
#49306=DIRECTION('center_axis',(-0.364399348580519,0.,-0.931242779705751));
#49307=DIRECTION('ref_axis',(-0.931242779705751,0.,0.364399348580519));
#49308=DIRECTION('',(0.,1.,0.));
#49309=DIRECTION('center_axis',(0.624280230025758,0.,-0.781200482846105));
#49310=DIRECTION('ref_axis',(-0.781200482846105,0.,-0.624280230025758));
#49311=DIRECTION('center_axis',(0.988679578606276,0.,0.150042296859641));
#49312=DIRECTION('ref_axis',(0.150042296859641,0.,-0.988679578606276));
#49313=DIRECTION('',(0.,1.,0.));
#49314=DIRECTION('',(0.,1.,0.));
#49315=DIRECTION('center_axis',(0.364399348580517,0.,0.931242779705752));
#49316=DIRECTION('ref_axis',(0.931242779705752,0.,-0.364399348580517));
#49317=DIRECTION('',(0.,1.,0.));
#49318=DIRECTION('center_axis',(-0.624280230025758,0.,0.781200482846104));
#49319=DIRECTION('ref_axis',(0.781200482846104,0.,0.624280230025758));
#49320=DIRECTION('',(0.,1.,0.));
#49321=DIRECTION('center_axis',(-0.988679578606275,0.,-0.150042296859647));
#49322=DIRECTION('ref_axis',(-0.150042296859647,0.,0.988679578606275));
#49323=DIRECTION('',(0.,1.,0.));
#49324=DIRECTION('center_axis',(-0.364399348580519,0.,-0.931242779705751));
#49325=DIRECTION('ref_axis',(-0.931242779705751,0.,0.364399348580519));
#49326=DIRECTION('',(0.,1.,0.));
#49327=DIRECTION('center_axis',(0.624280230025758,0.,-0.781200482846105));
#49328=DIRECTION('ref_axis',(-0.781200482846105,0.,-0.624280230025758));
#49329=DIRECTION('center_axis',(0.988679578606276,0.,0.150042296859641));
#49330=DIRECTION('ref_axis',(0.150042296859641,0.,-0.988679578606276));
#49331=DIRECTION('',(0.,1.,0.));
#49332=DIRECTION('',(0.,1.,0.));
#49333=DIRECTION('center_axis',(0.364399348580517,0.,0.931242779705752));
#49334=DIRECTION('ref_axis',(0.931242779705752,0.,-0.364399348580517));
#49335=DIRECTION('',(0.,1.,0.));
#49336=DIRECTION('center_axis',(-0.624280230025758,0.,0.781200482846104));
#49337=DIRECTION('ref_axis',(0.781200482846104,0.,0.624280230025758));
#49338=DIRECTION('',(0.,1.,0.));
#49339=DIRECTION('center_axis',(-0.988679578606275,0.,-0.150042296859647));
#49340=DIRECTION('ref_axis',(-0.150042296859647,0.,0.988679578606275));
#49341=DIRECTION('',(0.,1.,0.));
#49342=DIRECTION('center_axis',(-0.364399348580519,0.,-0.931242779705751));
#49343=DIRECTION('ref_axis',(-0.931242779705751,0.,0.364399348580519));
#49344=DIRECTION('',(0.,1.,0.));
#49345=DIRECTION('center_axis',(0.624280230025758,0.,-0.781200482846105));
#49346=DIRECTION('ref_axis',(-0.781200482846105,0.,-0.624280230025758));
#49347=DIRECTION('center_axis',(0.988679578606276,0.,0.150042296859641));
#49348=DIRECTION('ref_axis',(0.150042296859641,0.,-0.988679578606276));
#49349=DIRECTION('',(0.,1.,0.));
#49350=DIRECTION('',(0.,1.,0.));
#49351=DIRECTION('center_axis',(0.364399348580517,0.,0.931242779705752));
#49352=DIRECTION('ref_axis',(0.931242779705752,0.,-0.364399348580517));
#49353=DIRECTION('',(0.,1.,0.));
#49354=DIRECTION('center_axis',(-0.624280230025758,0.,0.781200482846104));
#49355=DIRECTION('ref_axis',(0.781200482846104,0.,0.624280230025758));
#49356=DIRECTION('',(0.,1.,0.));
#49357=DIRECTION('center_axis',(-0.988679578606275,0.,-0.150042296859647));
#49358=DIRECTION('ref_axis',(-0.150042296859647,0.,0.988679578606275));
#49359=DIRECTION('',(0.,1.,0.));
#49360=DIRECTION('center_axis',(-0.364399348580519,0.,-0.931242779705751));
#49361=DIRECTION('ref_axis',(-0.931242779705751,0.,0.364399348580519));
#49362=DIRECTION('',(0.,1.,0.));
#49363=DIRECTION('center_axis',(0.624280230025758,0.,-0.781200482846105));
#49364=DIRECTION('ref_axis',(-0.781200482846105,0.,-0.624280230025758));
#49365=DIRECTION('center_axis',(0.988679578606276,0.,0.150042296859641));
#49366=DIRECTION('ref_axis',(0.150042296859641,0.,-0.988679578606276));
#49367=DIRECTION('',(0.,1.,0.));
#49368=DIRECTION('',(0.,1.,0.));
#49369=DIRECTION('center_axis',(0.364399348580517,0.,0.931242779705752));
#49370=DIRECTION('ref_axis',(0.931242779705752,0.,-0.364399348580517));
#49371=DIRECTION('',(0.,1.,0.));
#49372=DIRECTION('center_axis',(-0.624280230025758,0.,0.781200482846104));
#49373=DIRECTION('ref_axis',(0.781200482846104,0.,0.624280230025758));
#49374=DIRECTION('',(0.,1.,0.));
#49375=DIRECTION('center_axis',(-0.988679578606275,0.,-0.150042296859647));
#49376=DIRECTION('ref_axis',(-0.150042296859647,0.,0.988679578606275));
#49377=DIRECTION('',(0.,1.,0.));
#49378=DIRECTION('center_axis',(-0.364399348580519,0.,-0.931242779705751));
#49379=DIRECTION('ref_axis',(-0.931242779705751,0.,0.364399348580519));
#49380=DIRECTION('',(0.,1.,0.));
#49381=DIRECTION('center_axis',(0.624280230025758,0.,-0.781200482846105));
#49382=DIRECTION('ref_axis',(-0.781200482846105,0.,-0.624280230025758));
#49383=DIRECTION('center_axis',(0.988679578606276,0.,0.150042296859641));
#49384=DIRECTION('ref_axis',(0.150042296859641,0.,-0.988679578606276));
#49385=DIRECTION('',(0.,1.,0.));
#49386=DIRECTION('',(0.,1.,0.));
#49387=DIRECTION('center_axis',(0.364399348580517,0.,0.931242779705752));
#49388=DIRECTION('ref_axis',(0.931242779705752,0.,-0.364399348580517));
#49389=DIRECTION('',(0.,1.,0.));
#49390=DIRECTION('center_axis',(-0.624280230025758,0.,0.781200482846104));
#49391=DIRECTION('ref_axis',(0.781200482846104,0.,0.624280230025758));
#49392=DIRECTION('',(0.,1.,0.));
#49393=DIRECTION('center_axis',(-0.988679578606275,0.,-0.150042296859647));
#49394=DIRECTION('ref_axis',(-0.150042296859647,0.,0.988679578606275));
#49395=DIRECTION('',(0.,1.,0.));
#49396=DIRECTION('center_axis',(-0.364399348580519,0.,-0.931242779705751));
#49397=DIRECTION('ref_axis',(-0.931242779705751,0.,0.364399348580519));
#49398=DIRECTION('',(0.,1.,0.));
#49399=DIRECTION('center_axis',(0.624280230025758,0.,-0.781200482846105));
#49400=DIRECTION('ref_axis',(-0.781200482846105,0.,-0.624280230025758));
#49401=DIRECTION('center_axis',(0.988679578606276,0.,0.150042296859641));
#49402=DIRECTION('ref_axis',(0.150042296859641,0.,-0.988679578606276));
#49403=DIRECTION('',(0.,1.,0.));
#49404=DIRECTION('',(0.,1.,0.));
#49405=DIRECTION('center_axis',(0.364399348580517,0.,0.931242779705752));
#49406=DIRECTION('ref_axis',(0.931242779705752,0.,-0.364399348580517));
#49407=DIRECTION('',(0.,1.,0.));
#49408=DIRECTION('center_axis',(-0.624280230025758,0.,0.781200482846104));
#49409=DIRECTION('ref_axis',(0.781200482846104,0.,0.624280230025758));
#49410=DIRECTION('',(0.,1.,0.));
#49411=DIRECTION('center_axis',(-0.988679578606275,0.,-0.150042296859647));
#49412=DIRECTION('ref_axis',(-0.150042296859647,0.,0.988679578606275));
#49413=DIRECTION('',(0.,1.,0.));
#49414=DIRECTION('center_axis',(-0.364399348580519,0.,-0.931242779705751));
#49415=DIRECTION('ref_axis',(-0.931242779705751,0.,0.364399348580519));
#49416=DIRECTION('',(0.,1.,0.));
#49417=DIRECTION('center_axis',(0.624280230025758,0.,-0.781200482846105));
#49418=DIRECTION('ref_axis',(-0.781200482846105,0.,-0.624280230025758));
#49419=DIRECTION('center_axis',(0.988679578606276,0.,0.150042296859641));
#49420=DIRECTION('ref_axis',(0.150042296859641,0.,-0.988679578606276));
#49421=DIRECTION('',(0.,1.,0.));
#49422=DIRECTION('',(0.,1.,0.));
#49423=DIRECTION('center_axis',(0.364399348580517,0.,0.931242779705752));
#49424=DIRECTION('ref_axis',(0.931242779705752,0.,-0.364399348580517));
#49425=DIRECTION('',(0.,1.,0.));
#49426=DIRECTION('center_axis',(-0.624280230025758,0.,0.781200482846104));
#49427=DIRECTION('ref_axis',(0.781200482846104,0.,0.624280230025758));
#49428=DIRECTION('',(0.,1.,0.));
#49429=DIRECTION('center_axis',(-0.988679578606275,0.,-0.150042296859647));
#49430=DIRECTION('ref_axis',(-0.150042296859647,0.,0.988679578606275));
#49431=DIRECTION('',(0.,1.,0.));
#49432=DIRECTION('center_axis',(-0.364399348580519,0.,-0.931242779705751));
#49433=DIRECTION('ref_axis',(-0.931242779705751,0.,0.364399348580519));
#49434=DIRECTION('',(0.,1.,0.));
#49435=DIRECTION('center_axis',(0.624280230025758,0.,-0.781200482846105));
#49436=DIRECTION('ref_axis',(-0.781200482846105,0.,-0.624280230025758));
#49437=DIRECTION('center_axis',(0.988679578606276,0.,0.150042296859641));
#49438=DIRECTION('ref_axis',(0.150042296859641,0.,-0.988679578606276));
#49439=DIRECTION('',(0.,1.,0.));
#49440=DIRECTION('',(0.,1.,0.));
#49441=DIRECTION('center_axis',(0.364399348580517,0.,0.931242779705752));
#49442=DIRECTION('ref_axis',(0.931242779705752,0.,-0.364399348580517));
#49443=DIRECTION('',(0.,1.,0.));
#49444=DIRECTION('center_axis',(-0.624280230025758,0.,0.781200482846104));
#49445=DIRECTION('ref_axis',(0.781200482846104,0.,0.624280230025758));
#49446=DIRECTION('',(0.,1.,0.));
#49447=DIRECTION('center_axis',(-0.988679578606275,0.,-0.150042296859647));
#49448=DIRECTION('ref_axis',(-0.150042296859647,0.,0.988679578606275));
#49449=DIRECTION('',(0.,1.,0.));
#49450=DIRECTION('center_axis',(-0.364399348580519,0.,-0.931242779705751));
#49451=DIRECTION('ref_axis',(-0.931242779705751,0.,0.364399348580519));
#49452=DIRECTION('',(0.,1.,0.));
#49453=DIRECTION('center_axis',(0.624280230025758,0.,-0.781200482846105));
#49454=DIRECTION('ref_axis',(-0.781200482846105,0.,-0.624280230025758));
#49455=DIRECTION('center_axis',(0.988679578606276,0.,0.150042296859641));
#49456=DIRECTION('ref_axis',(0.150042296859641,0.,-0.988679578606276));
#49457=DIRECTION('',(0.,1.,0.));
#49458=DIRECTION('',(0.,1.,0.));
#49459=DIRECTION('center_axis',(0.364399348580517,0.,0.931242779705752));
#49460=DIRECTION('ref_axis',(0.931242779705752,0.,-0.364399348580517));
#49461=DIRECTION('',(0.,1.,0.));
#49462=DIRECTION('center_axis',(-0.624280230025758,0.,0.781200482846104));
#49463=DIRECTION('ref_axis',(0.781200482846104,0.,0.624280230025758));
#49464=DIRECTION('',(0.,1.,0.));
#49465=DIRECTION('center_axis',(-0.988679578606275,0.,-0.150042296859647));
#49466=DIRECTION('ref_axis',(-0.150042296859647,0.,0.988679578606275));
#49467=DIRECTION('',(0.,1.,0.));
#49468=DIRECTION('center_axis',(-0.364399348580519,0.,-0.931242779705751));
#49469=DIRECTION('ref_axis',(-0.931242779705751,0.,0.364399348580519));
#49470=DIRECTION('',(0.,1.,0.));
#49471=DIRECTION('center_axis',(0.624280230025758,0.,-0.781200482846105));
#49472=DIRECTION('ref_axis',(-0.781200482846105,0.,-0.624280230025758));
#49473=DIRECTION('center_axis',(0.988679578606276,0.,0.150042296859641));
#49474=DIRECTION('ref_axis',(0.150042296859641,0.,-0.988679578606276));
#49475=DIRECTION('',(0.,1.,0.));
#49476=DIRECTION('',(0.,1.,0.));
#49477=DIRECTION('center_axis',(0.364399348580517,0.,0.931242779705752));
#49478=DIRECTION('ref_axis',(0.931242779705752,0.,-0.364399348580517));
#49479=DIRECTION('',(0.,1.,0.));
#49480=DIRECTION('center_axis',(-0.624280230025758,0.,0.781200482846104));
#49481=DIRECTION('ref_axis',(0.781200482846104,0.,0.624280230025758));
#49482=DIRECTION('',(0.,1.,0.));
#49483=DIRECTION('center_axis',(-0.988679578606275,0.,-0.150042296859647));
#49484=DIRECTION('ref_axis',(-0.150042296859647,0.,0.988679578606275));
#49485=DIRECTION('',(0.,1.,0.));
#49486=DIRECTION('center_axis',(-0.364399348580519,0.,-0.931242779705751));
#49487=DIRECTION('ref_axis',(-0.931242779705751,0.,0.364399348580519));
#49488=DIRECTION('',(0.,1.,0.));
#49489=DIRECTION('center_axis',(0.624280230025758,0.,-0.781200482846105));
#49490=DIRECTION('ref_axis',(-0.781200482846105,0.,-0.624280230025758));
#49491=DIRECTION('center_axis',(0.988679578606276,0.,0.150042296859641));
#49492=DIRECTION('ref_axis',(0.150042296859641,0.,-0.988679578606276));
#49493=DIRECTION('',(0.,1.,0.));
#49494=DIRECTION('',(0.,1.,0.));
#49495=DIRECTION('center_axis',(0.364399348580517,0.,0.931242779705752));
#49496=DIRECTION('ref_axis',(0.931242779705752,0.,-0.364399348580517));
#49497=DIRECTION('',(0.,1.,0.));
#49498=DIRECTION('center_axis',(-0.624280230025758,0.,0.781200482846104));
#49499=DIRECTION('ref_axis',(0.781200482846104,0.,0.624280230025758));
#49500=DIRECTION('',(0.,1.,0.));
#49501=DIRECTION('center_axis',(-0.988679578606275,0.,-0.150042296859647));
#49502=DIRECTION('ref_axis',(-0.150042296859647,0.,0.988679578606275));
#49503=DIRECTION('',(0.,1.,0.));
#49504=DIRECTION('center_axis',(-0.364399348580519,0.,-0.931242779705751));
#49505=DIRECTION('ref_axis',(-0.931242779705751,0.,0.364399348580519));
#49506=DIRECTION('',(0.,1.,0.));
#49507=DIRECTION('center_axis',(0.624280230025758,0.,-0.781200482846105));
#49508=DIRECTION('ref_axis',(-0.781200482846105,0.,-0.624280230025758));
#49509=DIRECTION('center_axis',(0.988679578606276,0.,0.150042296859641));
#49510=DIRECTION('ref_axis',(0.150042296859641,0.,-0.988679578606276));
#49511=DIRECTION('',(0.,1.,0.));
#49512=DIRECTION('',(0.,1.,0.));
#49513=DIRECTION('center_axis',(0.364399348580517,0.,0.931242779705752));
#49514=DIRECTION('ref_axis',(0.931242779705752,0.,-0.364399348580517));
#49515=DIRECTION('',(0.,1.,0.));
#49516=DIRECTION('center_axis',(-0.624280230025758,0.,0.781200482846104));
#49517=DIRECTION('ref_axis',(0.781200482846104,0.,0.624280230025758));
#49518=DIRECTION('',(0.,1.,0.));
#49519=DIRECTION('center_axis',(-0.988679578606275,0.,-0.150042296859647));
#49520=DIRECTION('ref_axis',(-0.150042296859647,0.,0.988679578606275));
#49521=DIRECTION('',(0.,1.,0.));
#49522=DIRECTION('center_axis',(-0.364399348580519,0.,-0.931242779705751));
#49523=DIRECTION('ref_axis',(-0.931242779705751,0.,0.364399348580519));
#49524=DIRECTION('',(0.,1.,0.));
#49525=DIRECTION('center_axis',(0.624280230025758,0.,-0.781200482846105));
#49526=DIRECTION('ref_axis',(-0.781200482846105,0.,-0.624280230025758));
#49527=DIRECTION('center_axis',(0.988679578606276,0.,0.150042296859641));
#49528=DIRECTION('ref_axis',(0.150042296859641,0.,-0.988679578606276));
#49529=DIRECTION('',(0.,1.,0.));
#49530=DIRECTION('',(0.,1.,0.));
#49531=DIRECTION('center_axis',(0.364399348580517,0.,0.931242779705752));
#49532=DIRECTION('ref_axis',(0.931242779705752,0.,-0.364399348580517));
#49533=DIRECTION('',(0.,1.,0.));
#49534=DIRECTION('center_axis',(-0.624280230025758,0.,0.781200482846104));
#49535=DIRECTION('ref_axis',(0.781200482846104,0.,0.624280230025758));
#49536=DIRECTION('',(0.,1.,0.));
#49537=DIRECTION('center_axis',(-0.988679578606275,0.,-0.150042296859647));
#49538=DIRECTION('ref_axis',(-0.150042296859647,0.,0.988679578606275));
#49539=DIRECTION('',(0.,1.,0.));
#49540=DIRECTION('center_axis',(-0.364399348580519,0.,-0.931242779705751));
#49541=DIRECTION('ref_axis',(-0.931242779705751,0.,0.364399348580519));
#49542=DIRECTION('',(0.,1.,0.));
#49543=DIRECTION('center_axis',(0.624280230025758,0.,-0.781200482846105));
#49544=DIRECTION('ref_axis',(-0.781200482846105,0.,-0.624280230025758));
#49545=DIRECTION('center_axis',(0.988679578606276,0.,0.150042296859641));
#49546=DIRECTION('ref_axis',(0.150042296859641,0.,-0.988679578606276));
#49547=DIRECTION('',(0.,1.,0.));
#49548=DIRECTION('',(0.,1.,0.));
#49549=DIRECTION('center_axis',(0.364399348580517,0.,0.931242779705752));
#49550=DIRECTION('ref_axis',(0.931242779705752,0.,-0.364399348580517));
#49551=DIRECTION('',(0.,1.,0.));
#49552=DIRECTION('center_axis',(-0.624280230025758,0.,0.781200482846104));
#49553=DIRECTION('ref_axis',(0.781200482846104,0.,0.624280230025758));
#49554=DIRECTION('',(0.,1.,0.));
#49555=DIRECTION('center_axis',(-0.988679578606275,0.,-0.150042296859647));
#49556=DIRECTION('ref_axis',(-0.150042296859647,0.,0.988679578606275));
#49557=DIRECTION('',(0.,1.,0.));
#49558=DIRECTION('center_axis',(-0.364399348580519,0.,-0.931242779705751));
#49559=DIRECTION('ref_axis',(-0.931242779705751,0.,0.364399348580519));
#49560=DIRECTION('',(0.,1.,0.));
#49561=DIRECTION('center_axis',(0.624280230025758,0.,-0.781200482846105));
#49562=DIRECTION('ref_axis',(-0.781200482846105,0.,-0.624280230025758));
#49563=DIRECTION('center_axis',(0.988679578606276,0.,0.150042296859641));
#49564=DIRECTION('ref_axis',(0.150042296859641,0.,-0.988679578606276));
#49565=DIRECTION('',(0.,1.,0.));
#49566=DIRECTION('',(0.,1.,0.));
#49567=DIRECTION('center_axis',(0.364399348580517,0.,0.931242779705752));
#49568=DIRECTION('ref_axis',(0.931242779705752,0.,-0.364399348580517));
#49569=DIRECTION('',(0.,1.,0.));
#49570=DIRECTION('center_axis',(-0.624280230025758,0.,0.781200482846104));
#49571=DIRECTION('ref_axis',(0.781200482846104,0.,0.624280230025758));
#49572=DIRECTION('',(0.,1.,0.));
#49573=DIRECTION('center_axis',(-0.988679578606275,0.,-0.150042296859647));
#49574=DIRECTION('ref_axis',(-0.150042296859647,0.,0.988679578606275));
#49575=DIRECTION('',(0.,1.,0.));
#49576=DIRECTION('center_axis',(-0.364399348580519,0.,-0.931242779705751));
#49577=DIRECTION('ref_axis',(-0.931242779705751,0.,0.364399348580519));
#49578=DIRECTION('',(0.,1.,0.));
#49579=DIRECTION('center_axis',(0.624280230025758,0.,-0.781200482846105));
#49580=DIRECTION('ref_axis',(-0.781200482846105,0.,-0.624280230025758));
#49581=DIRECTION('center_axis',(0.988679578606276,0.,0.150042296859641));
#49582=DIRECTION('ref_axis',(0.150042296859641,0.,-0.988679578606276));
#49583=DIRECTION('',(0.,1.,0.));
#49584=DIRECTION('',(0.,1.,0.));
#49585=DIRECTION('center_axis',(0.364399348580517,0.,0.931242779705752));
#49586=DIRECTION('ref_axis',(0.931242779705752,0.,-0.364399348580517));
#49587=DIRECTION('',(0.,1.,0.));
#49588=DIRECTION('center_axis',(-0.624280230025758,0.,0.781200482846104));
#49589=DIRECTION('ref_axis',(0.781200482846104,0.,0.624280230025758));
#49590=DIRECTION('',(0.,1.,0.));
#49591=DIRECTION('center_axis',(-0.988679578606275,0.,-0.150042296859647));
#49592=DIRECTION('ref_axis',(-0.150042296859647,0.,0.988679578606275));
#49593=DIRECTION('',(0.,1.,0.));
#49594=DIRECTION('center_axis',(-0.364399348580519,0.,-0.931242779705751));
#49595=DIRECTION('ref_axis',(-0.931242779705751,0.,0.364399348580519));
#49596=DIRECTION('',(0.,1.,0.));
#49597=DIRECTION('center_axis',(0.624280230025758,0.,-0.781200482846105));
#49598=DIRECTION('ref_axis',(-0.781200482846105,0.,-0.624280230025758));
#49599=DIRECTION('center_axis',(0.988679578606276,0.,0.150042296859641));
#49600=DIRECTION('ref_axis',(0.150042296859641,0.,-0.988679578606276));
#49601=DIRECTION('',(0.,1.,0.));
#49602=DIRECTION('',(0.,1.,0.));
#49603=DIRECTION('center_axis',(0.364399348580517,0.,0.931242779705752));
#49604=DIRECTION('ref_axis',(0.931242779705752,0.,-0.364399348580517));
#49605=DIRECTION('',(0.,1.,0.));
#49606=DIRECTION('center_axis',(-0.624280230025758,0.,0.781200482846104));
#49607=DIRECTION('ref_axis',(0.781200482846104,0.,0.624280230025758));
#49608=DIRECTION('',(0.,1.,0.));
#49609=DIRECTION('center_axis',(-0.988679578606275,0.,-0.150042296859647));
#49610=DIRECTION('ref_axis',(-0.150042296859647,0.,0.988679578606275));
#49611=DIRECTION('',(0.,1.,0.));
#49612=DIRECTION('center_axis',(-0.364399348580519,0.,-0.931242779705751));
#49613=DIRECTION('ref_axis',(-0.931242779705751,0.,0.364399348580519));
#49614=DIRECTION('',(0.,1.,0.));
#49615=DIRECTION('center_axis',(0.624280230025758,0.,-0.781200482846105));
#49616=DIRECTION('ref_axis',(-0.781200482846105,0.,-0.624280230025758));
#49617=DIRECTION('center_axis',(0.988679578606276,0.,0.150042296859641));
#49618=DIRECTION('ref_axis',(0.150042296859641,0.,-0.988679578606276));
#49619=DIRECTION('',(0.,1.,0.));
#49620=DIRECTION('',(0.,1.,0.));
#49621=DIRECTION('center_axis',(0.364399348580517,0.,0.931242779705752));
#49622=DIRECTION('ref_axis',(0.931242779705752,0.,-0.364399348580517));
#49623=DIRECTION('',(0.,1.,0.));
#49624=DIRECTION('center_axis',(-0.624280230025758,0.,0.781200482846104));
#49625=DIRECTION('ref_axis',(0.781200482846104,0.,0.624280230025758));
#49626=DIRECTION('',(0.,1.,0.));
#49627=DIRECTION('center_axis',(-0.988679578606275,0.,-0.150042296859647));
#49628=DIRECTION('ref_axis',(-0.150042296859647,0.,0.988679578606275));
#49629=DIRECTION('',(0.,1.,0.));
#49630=DIRECTION('center_axis',(-0.364399348580519,0.,-0.931242779705751));
#49631=DIRECTION('ref_axis',(-0.931242779705751,0.,0.364399348580519));
#49632=DIRECTION('',(0.,1.,0.));
#49633=DIRECTION('center_axis',(0.624280230025758,0.,-0.781200482846105));
#49634=DIRECTION('ref_axis',(-0.781200482846105,0.,-0.624280230025758));
#49635=DIRECTION('center_axis',(0.988679578606276,0.,0.150042296859641));
#49636=DIRECTION('ref_axis',(0.150042296859641,0.,-0.988679578606276));
#49637=DIRECTION('',(0.,1.,0.));
#49638=DIRECTION('',(0.,1.,0.));
#49639=DIRECTION('center_axis',(0.364399348580517,0.,0.931242779705752));
#49640=DIRECTION('ref_axis',(0.931242779705752,0.,-0.364399348580517));
#49641=DIRECTION('',(0.,1.,0.));
#49642=DIRECTION('center_axis',(-0.624280230025758,0.,0.781200482846104));
#49643=DIRECTION('ref_axis',(0.781200482846104,0.,0.624280230025758));
#49644=DIRECTION('',(0.,1.,0.));
#49645=DIRECTION('center_axis',(-0.988679578606275,0.,-0.150042296859647));
#49646=DIRECTION('ref_axis',(-0.150042296859647,0.,0.988679578606275));
#49647=DIRECTION('',(0.,1.,0.));
#49648=DIRECTION('center_axis',(-0.364399348580519,0.,-0.931242779705751));
#49649=DIRECTION('ref_axis',(-0.931242779705751,0.,0.364399348580519));
#49650=DIRECTION('',(0.,1.,0.));
#49651=DIRECTION('center_axis',(0.624280230025758,0.,-0.781200482846105));
#49652=DIRECTION('ref_axis',(-0.781200482846105,0.,-0.624280230025758));
#49653=DIRECTION('center_axis',(0.988679578606276,0.,0.150042296859641));
#49654=DIRECTION('ref_axis',(0.150042296859641,0.,-0.988679578606276));
#49655=DIRECTION('',(0.,1.,0.));
#49656=DIRECTION('',(0.,1.,0.));
#49657=DIRECTION('center_axis',(0.364399348580517,0.,0.931242779705752));
#49658=DIRECTION('ref_axis',(0.931242779705752,0.,-0.364399348580517));
#49659=DIRECTION('',(0.,1.,0.));
#49660=DIRECTION('center_axis',(-0.624280230025758,0.,0.781200482846104));
#49661=DIRECTION('ref_axis',(0.781200482846104,0.,0.624280230025758));
#49662=DIRECTION('',(0.,1.,0.));
#49663=DIRECTION('center_axis',(-0.988679578606275,0.,-0.150042296859647));
#49664=DIRECTION('ref_axis',(-0.150042296859647,0.,0.988679578606275));
#49665=DIRECTION('',(0.,1.,0.));
#49666=DIRECTION('center_axis',(-0.364399348580519,0.,-0.931242779705751));
#49667=DIRECTION('ref_axis',(-0.931242779705751,0.,0.364399348580519));
#49668=DIRECTION('',(0.,1.,0.));
#49669=DIRECTION('center_axis',(0.624280230025758,0.,-0.781200482846105));
#49670=DIRECTION('ref_axis',(-0.781200482846105,0.,-0.624280230025758));
#49671=DIRECTION('center_axis',(0.988679578606276,0.,0.150042296859641));
#49672=DIRECTION('ref_axis',(0.150042296859641,0.,-0.988679578606276));
#49673=DIRECTION('',(0.,1.,0.));
#49674=DIRECTION('',(0.,1.,0.));
#49675=DIRECTION('center_axis',(0.364399348580517,0.,0.931242779705752));
#49676=DIRECTION('ref_axis',(0.931242779705752,0.,-0.364399348580517));
#49677=DIRECTION('',(0.,1.,0.));
#49678=DIRECTION('center_axis',(-0.624280230025758,0.,0.781200482846104));
#49679=DIRECTION('ref_axis',(0.781200482846104,0.,0.624280230025758));
#49680=DIRECTION('',(0.,1.,0.));
#49681=DIRECTION('center_axis',(-0.988679578606275,0.,-0.150042296859647));
#49682=DIRECTION('ref_axis',(-0.150042296859647,0.,0.988679578606275));
#49683=DIRECTION('',(0.,1.,0.));
#49684=DIRECTION('center_axis',(-0.364399348580519,0.,-0.931242779705751));
#49685=DIRECTION('ref_axis',(-0.931242779705751,0.,0.364399348580519));
#49686=DIRECTION('',(0.,1.,0.));
#49687=DIRECTION('center_axis',(0.624280230025758,0.,-0.781200482846105));
#49688=DIRECTION('ref_axis',(-0.781200482846105,0.,-0.624280230025758));
#49689=DIRECTION('center_axis',(0.988679578606276,0.,0.150042296859641));
#49690=DIRECTION('ref_axis',(0.150042296859641,0.,-0.988679578606276));
#49691=DIRECTION('',(0.,1.,0.));
#49692=DIRECTION('',(0.,1.,0.));
#49693=DIRECTION('center_axis',(0.364399348580517,0.,0.931242779705752));
#49694=DIRECTION('ref_axis',(0.931242779705752,0.,-0.364399348580517));
#49695=DIRECTION('',(0.,1.,0.));
#49696=DIRECTION('center_axis',(-0.624280230025758,0.,0.781200482846104));
#49697=DIRECTION('ref_axis',(0.781200482846104,0.,0.624280230025758));
#49698=DIRECTION('',(0.,1.,0.));
#49699=DIRECTION('center_axis',(-0.988679578606275,0.,-0.150042296859647));
#49700=DIRECTION('ref_axis',(-0.150042296859647,0.,0.988679578606275));
#49701=DIRECTION('',(0.,1.,0.));
#49702=DIRECTION('center_axis',(-0.364399348580519,0.,-0.931242779705751));
#49703=DIRECTION('ref_axis',(-0.931242779705751,0.,0.364399348580519));
#49704=DIRECTION('',(0.,1.,0.));
#49705=DIRECTION('center_axis',(0.624280230025758,0.,-0.781200482846105));
#49706=DIRECTION('ref_axis',(-0.781200482846105,0.,-0.624280230025758));
#49707=DIRECTION('center_axis',(0.988679578606276,0.,0.150042296859641));
#49708=DIRECTION('ref_axis',(0.150042296859641,0.,-0.988679578606276));
#49709=DIRECTION('',(0.,1.,0.));
#49710=DIRECTION('',(0.,1.,0.));
#49711=DIRECTION('center_axis',(0.364399348580517,0.,0.931242779705752));
#49712=DIRECTION('ref_axis',(0.931242779705752,0.,-0.364399348580517));
#49713=DIRECTION('',(0.,1.,0.));
#49714=DIRECTION('center_axis',(-0.624280230025758,0.,0.781200482846104));
#49715=DIRECTION('ref_axis',(0.781200482846104,0.,0.624280230025758));
#49716=DIRECTION('',(0.,1.,0.));
#49717=DIRECTION('center_axis',(-0.988679578606275,0.,-0.150042296859647));
#49718=DIRECTION('ref_axis',(-0.150042296859647,0.,0.988679578606275));
#49719=DIRECTION('',(0.,1.,0.));
#49720=DIRECTION('center_axis',(-0.364399348580519,0.,-0.931242779705751));
#49721=DIRECTION('ref_axis',(-0.931242779705751,0.,0.364399348580519));
#49722=DIRECTION('',(0.,1.,0.));
#49723=DIRECTION('center_axis',(0.624280230025758,0.,-0.781200482846105));
#49724=DIRECTION('ref_axis',(-0.781200482846105,0.,-0.624280230025758));
#49725=DIRECTION('center_axis',(0.988679578606276,0.,0.150042296859641));
#49726=DIRECTION('ref_axis',(0.150042296859641,0.,-0.988679578606276));
#49727=DIRECTION('',(0.,1.,0.));
#49728=DIRECTION('',(0.,1.,0.));
#49729=DIRECTION('center_axis',(0.364399348580517,0.,0.931242779705752));
#49730=DIRECTION('ref_axis',(0.931242779705752,0.,-0.364399348580517));
#49731=DIRECTION('',(0.,1.,0.));
#49732=DIRECTION('center_axis',(-0.624280230025758,0.,0.781200482846104));
#49733=DIRECTION('ref_axis',(0.781200482846104,0.,0.624280230025758));
#49734=DIRECTION('',(0.,1.,0.));
#49735=DIRECTION('center_axis',(-0.988679578606275,0.,-0.150042296859647));
#49736=DIRECTION('ref_axis',(-0.150042296859647,0.,0.988679578606275));
#49737=DIRECTION('',(0.,1.,0.));
#49738=DIRECTION('center_axis',(-0.364399348580519,0.,-0.931242779705751));
#49739=DIRECTION('ref_axis',(-0.931242779705751,0.,0.364399348580519));
#49740=DIRECTION('',(0.,1.,0.));
#49741=DIRECTION('center_axis',(0.624280230025758,0.,-0.781200482846105));
#49742=DIRECTION('ref_axis',(-0.781200482846105,0.,-0.624280230025758));
#49743=DIRECTION('center_axis',(0.988679578606276,0.,0.150042296859641));
#49744=DIRECTION('ref_axis',(0.150042296859641,0.,-0.988679578606276));
#49745=DIRECTION('',(0.,1.,0.));
#49746=DIRECTION('',(0.,1.,0.));
#49747=DIRECTION('center_axis',(0.364399348580517,0.,0.931242779705752));
#49748=DIRECTION('ref_axis',(0.931242779705752,0.,-0.364399348580517));
#49749=DIRECTION('',(0.,1.,0.));
#49750=DIRECTION('center_axis',(-0.624280230025758,0.,0.781200482846104));
#49751=DIRECTION('ref_axis',(0.781200482846104,0.,0.624280230025758));
#49752=DIRECTION('',(0.,1.,0.));
#49753=DIRECTION('center_axis',(-0.988679578606275,0.,-0.150042296859647));
#49754=DIRECTION('ref_axis',(-0.150042296859647,0.,0.988679578606275));
#49755=DIRECTION('',(0.,1.,0.));
#49756=DIRECTION('center_axis',(-0.364399348580519,0.,-0.931242779705751));
#49757=DIRECTION('ref_axis',(-0.931242779705751,0.,0.364399348580519));
#49758=DIRECTION('',(0.,1.,0.));
#49759=DIRECTION('center_axis',(0.624280230025758,0.,-0.781200482846105));
#49760=DIRECTION('ref_axis',(-0.781200482846105,0.,-0.624280230025758));
#49761=DIRECTION('center_axis',(0.988679578606276,0.,0.150042296859641));
#49762=DIRECTION('ref_axis',(0.150042296859641,0.,-0.988679578606276));
#49763=DIRECTION('',(0.,1.,0.));
#49764=DIRECTION('',(0.,1.,0.));
#49765=DIRECTION('center_axis',(0.364399348580517,0.,0.931242779705752));
#49766=DIRECTION('ref_axis',(0.931242779705752,0.,-0.364399348580517));
#49767=DIRECTION('',(0.,1.,0.));
#49768=DIRECTION('center_axis',(-0.624280230025758,0.,0.781200482846104));
#49769=DIRECTION('ref_axis',(0.781200482846104,0.,0.624280230025758));
#49770=DIRECTION('',(0.,1.,0.));
#49771=DIRECTION('center_axis',(-0.988679578606275,0.,-0.150042296859647));
#49772=DIRECTION('ref_axis',(-0.150042296859647,0.,0.988679578606275));
#49773=DIRECTION('',(0.,1.,0.));
#49774=DIRECTION('center_axis',(-0.364399348580519,0.,-0.931242779705751));
#49775=DIRECTION('ref_axis',(-0.931242779705751,0.,0.364399348580519));
#49776=DIRECTION('',(0.,1.,0.));
#49777=DIRECTION('center_axis',(0.624280230025758,0.,-0.781200482846105));
#49778=DIRECTION('ref_axis',(-0.781200482846105,0.,-0.624280230025758));
#49779=DIRECTION('center_axis',(0.988679578606276,0.,0.150042296859641));
#49780=DIRECTION('ref_axis',(0.150042296859641,0.,-0.988679578606276));
#49781=DIRECTION('',(0.,1.,0.));
#49782=DIRECTION('',(0.,1.,0.));
#49783=DIRECTION('center_axis',(0.364399348580517,0.,0.931242779705752));
#49784=DIRECTION('ref_axis',(0.931242779705752,0.,-0.364399348580517));
#49785=DIRECTION('',(0.,1.,0.));
#49786=DIRECTION('center_axis',(-0.624280230025758,0.,0.781200482846104));
#49787=DIRECTION('ref_axis',(0.781200482846104,0.,0.624280230025758));
#49788=DIRECTION('',(0.,1.,0.));
#49789=DIRECTION('center_axis',(-0.988679578606275,0.,-0.150042296859647));
#49790=DIRECTION('ref_axis',(-0.150042296859647,0.,0.988679578606275));
#49791=DIRECTION('',(0.,1.,0.));
#49792=DIRECTION('center_axis',(-0.364399348580519,0.,-0.931242779705751));
#49793=DIRECTION('ref_axis',(-0.931242779705751,0.,0.364399348580519));
#49794=DIRECTION('',(0.,1.,0.));
#49795=DIRECTION('center_axis',(0.624280230025758,0.,-0.781200482846105));
#49796=DIRECTION('ref_axis',(-0.781200482846105,0.,-0.624280230025758));
#49797=DIRECTION('center_axis',(0.988679578606276,0.,0.150042296859641));
#49798=DIRECTION('ref_axis',(0.150042296859641,0.,-0.988679578606276));
#49799=DIRECTION('',(0.,1.,0.));
#49800=DIRECTION('',(0.,1.,0.));
#49801=DIRECTION('center_axis',(0.364399348580517,0.,0.931242779705752));
#49802=DIRECTION('ref_axis',(0.931242779705752,0.,-0.364399348580517));
#49803=DIRECTION('',(0.,1.,0.));
#49804=DIRECTION('center_axis',(-0.624280230025758,0.,0.781200482846104));
#49805=DIRECTION('ref_axis',(0.781200482846104,0.,0.624280230025758));
#49806=DIRECTION('',(0.,1.,0.));
#49807=DIRECTION('center_axis',(-0.988679578606275,0.,-0.150042296859647));
#49808=DIRECTION('ref_axis',(-0.150042296859647,0.,0.988679578606275));
#49809=DIRECTION('',(0.,1.,0.));
#49810=DIRECTION('center_axis',(-0.364399348580519,0.,-0.931242779705751));
#49811=DIRECTION('ref_axis',(-0.931242779705751,0.,0.364399348580519));
#49812=DIRECTION('',(0.,1.,0.));
#49813=DIRECTION('center_axis',(0.624280230025758,0.,-0.781200482846105));
#49814=DIRECTION('ref_axis',(-0.781200482846105,0.,-0.624280230025758));
#49815=DIRECTION('center_axis',(0.988679578606276,0.,0.150042296859641));
#49816=DIRECTION('ref_axis',(0.150042296859641,0.,-0.988679578606276));
#49817=DIRECTION('',(0.,1.,0.));
#49818=DIRECTION('',(0.,1.,0.));
#49819=DIRECTION('center_axis',(0.364399348580517,0.,0.931242779705752));
#49820=DIRECTION('ref_axis',(0.931242779705752,0.,-0.364399348580517));
#49821=DIRECTION('',(0.,1.,0.));
#49822=DIRECTION('center_axis',(-0.624280230025758,0.,0.781200482846104));
#49823=DIRECTION('ref_axis',(0.781200482846104,0.,0.624280230025758));
#49824=DIRECTION('',(0.,1.,0.));
#49825=DIRECTION('center_axis',(-0.988679578606275,0.,-0.150042296859647));
#49826=DIRECTION('ref_axis',(-0.150042296859647,0.,0.988679578606275));
#49827=DIRECTION('',(0.,1.,0.));
#49828=DIRECTION('center_axis',(-0.364399348580519,0.,-0.931242779705751));
#49829=DIRECTION('ref_axis',(-0.931242779705751,0.,0.364399348580519));
#49830=DIRECTION('',(0.,1.,0.));
#49831=DIRECTION('center_axis',(0.624280230025758,0.,-0.781200482846105));
#49832=DIRECTION('ref_axis',(-0.781200482846105,0.,-0.624280230025758));
#49833=DIRECTION('center_axis',(0.988679578606276,0.,0.150042296859641));
#49834=DIRECTION('ref_axis',(0.150042296859641,0.,-0.988679578606276));
#49835=DIRECTION('',(0.,1.,0.));
#49836=DIRECTION('',(0.,1.,0.));
#49837=DIRECTION('center_axis',(0.364399348580517,0.,0.931242779705752));
#49838=DIRECTION('ref_axis',(0.931242779705752,0.,-0.364399348580517));
#49839=DIRECTION('',(0.,1.,0.));
#49840=DIRECTION('center_axis',(-0.624280230025758,0.,0.781200482846104));
#49841=DIRECTION('ref_axis',(0.781200482846104,0.,0.624280230025758));
#49842=DIRECTION('',(0.,1.,0.));
#49843=DIRECTION('center_axis',(-0.988679578606275,0.,-0.150042296859647));
#49844=DIRECTION('ref_axis',(-0.150042296859647,0.,0.988679578606275));
#49845=DIRECTION('',(0.,1.,0.));
#49846=DIRECTION('center_axis',(-0.364399348580519,0.,-0.931242779705751));
#49847=DIRECTION('ref_axis',(-0.931242779705751,0.,0.364399348580519));
#49848=DIRECTION('',(0.,1.,0.));
#49849=DIRECTION('center_axis',(0.624280230025758,0.,-0.781200482846105));
#49850=DIRECTION('ref_axis',(-0.781200482846105,0.,-0.624280230025758));
#49851=DIRECTION('center_axis',(0.988679578606276,0.,0.150042296859641));
#49852=DIRECTION('ref_axis',(0.150042296859641,0.,-0.988679578606276));
#49853=DIRECTION('',(0.,1.,0.));
#49854=DIRECTION('',(0.,1.,0.));
#49855=DIRECTION('center_axis',(0.364399348580517,0.,0.931242779705752));
#49856=DIRECTION('ref_axis',(0.931242779705752,0.,-0.364399348580517));
#49857=DIRECTION('',(0.,1.,0.));
#49858=DIRECTION('center_axis',(-0.624280230025758,0.,0.781200482846104));
#49859=DIRECTION('ref_axis',(0.781200482846104,0.,0.624280230025758));
#49860=DIRECTION('',(0.,1.,0.));
#49861=DIRECTION('center_axis',(-0.988679578606275,0.,-0.150042296859647));
#49862=DIRECTION('ref_axis',(-0.150042296859647,0.,0.988679578606275));
#49863=DIRECTION('',(0.,1.,0.));
#49864=DIRECTION('center_axis',(-0.364399348580519,0.,-0.931242779705751));
#49865=DIRECTION('ref_axis',(-0.931242779705751,0.,0.364399348580519));
#49866=DIRECTION('',(0.,1.,0.));
#49867=DIRECTION('center_axis',(0.624280230025758,0.,-0.781200482846105));
#49868=DIRECTION('ref_axis',(-0.781200482846105,0.,-0.624280230025758));
#49869=DIRECTION('center_axis',(0.988679578606276,0.,0.150042296859641));
#49870=DIRECTION('ref_axis',(0.150042296859641,0.,-0.988679578606276));
#49871=DIRECTION('',(0.,1.,0.));
#49872=DIRECTION('',(0.,1.,0.));
#49873=DIRECTION('center_axis',(0.364399348580517,0.,0.931242779705752));
#49874=DIRECTION('ref_axis',(0.931242779705752,0.,-0.364399348580517));
#49875=DIRECTION('',(0.,1.,0.));
#49876=DIRECTION('center_axis',(-0.624280230025758,0.,0.781200482846104));
#49877=DIRECTION('ref_axis',(0.781200482846104,0.,0.624280230025758));
#49878=DIRECTION('',(0.,1.,0.));
#49879=DIRECTION('center_axis',(-0.988679578606275,0.,-0.150042296859647));
#49880=DIRECTION('ref_axis',(-0.150042296859647,0.,0.988679578606275));
#49881=DIRECTION('',(0.,1.,0.));
#49882=DIRECTION('center_axis',(-0.364399348580519,0.,-0.931242779705751));
#49883=DIRECTION('ref_axis',(-0.931242779705751,0.,0.364399348580519));
#49884=DIRECTION('',(0.,1.,0.));
#49885=DIRECTION('center_axis',(0.624280230025758,0.,-0.781200482846105));
#49886=DIRECTION('ref_axis',(-0.781200482846105,0.,-0.624280230025758));
#49887=DIRECTION('center_axis',(0.988679578606276,0.,0.150042296859641));
#49888=DIRECTION('ref_axis',(0.150042296859641,0.,-0.988679578606276));
#49889=DIRECTION('',(0.,1.,0.));
#49890=DIRECTION('',(0.,1.,0.));
#49891=DIRECTION('center_axis',(0.364399348580517,0.,0.931242779705752));
#49892=DIRECTION('ref_axis',(0.931242779705752,0.,-0.364399348580517));
#49893=DIRECTION('',(0.,1.,0.));
#49894=DIRECTION('center_axis',(-0.624280230025758,0.,0.781200482846104));
#49895=DIRECTION('ref_axis',(0.781200482846104,0.,0.624280230025758));
#49896=DIRECTION('',(0.,1.,0.));
#49897=DIRECTION('center_axis',(-0.988679578606275,0.,-0.150042296859647));
#49898=DIRECTION('ref_axis',(-0.150042296859647,0.,0.988679578606275));
#49899=DIRECTION('',(0.,1.,0.));
#49900=DIRECTION('center_axis',(-0.364399348580519,0.,-0.931242779705751));
#49901=DIRECTION('ref_axis',(-0.931242779705751,0.,0.364399348580519));
#49902=DIRECTION('',(0.,1.,0.));
#49903=DIRECTION('center_axis',(0.624280230025758,0.,-0.781200482846105));
#49904=DIRECTION('ref_axis',(-0.781200482846105,0.,-0.624280230025758));
#49905=DIRECTION('center_axis',(0.988679578606276,0.,0.150042296859641));
#49906=DIRECTION('ref_axis',(0.150042296859641,0.,-0.988679578606276));
#49907=DIRECTION('',(0.,1.,0.));
#49908=DIRECTION('',(0.,1.,0.));
#49909=DIRECTION('center_axis',(0.364399348580517,0.,0.931242779705752));
#49910=DIRECTION('ref_axis',(0.931242779705752,0.,-0.364399348580517));
#49911=DIRECTION('',(0.,1.,0.));
#49912=DIRECTION('center_axis',(-0.624280230025758,0.,0.781200482846104));
#49913=DIRECTION('ref_axis',(0.781200482846104,0.,0.624280230025758));
#49914=DIRECTION('',(0.,1.,0.));
#49915=DIRECTION('center_axis',(-0.988679578606275,0.,-0.150042296859647));
#49916=DIRECTION('ref_axis',(-0.150042296859647,0.,0.988679578606275));
#49917=DIRECTION('',(0.,1.,0.));
#49918=DIRECTION('center_axis',(-0.364399348580519,0.,-0.931242779705751));
#49919=DIRECTION('ref_axis',(-0.931242779705751,0.,0.364399348580519));
#49920=DIRECTION('',(0.,1.,0.));
#49921=DIRECTION('center_axis',(0.624280230025758,0.,-0.781200482846105));
#49922=DIRECTION('ref_axis',(-0.781200482846105,0.,-0.624280230025758));
#49923=DIRECTION('center_axis',(0.988679578606276,0.,0.150042296859641));
#49924=DIRECTION('ref_axis',(0.150042296859641,0.,-0.988679578606276));
#49925=DIRECTION('',(0.,1.,0.));
#49926=DIRECTION('',(0.,1.,0.));
#49927=DIRECTION('center_axis',(0.364399348580517,0.,0.931242779705752));
#49928=DIRECTION('ref_axis',(0.931242779705752,0.,-0.364399348580517));
#49929=DIRECTION('',(0.,1.,0.));
#49930=DIRECTION('center_axis',(-0.624280230025758,0.,0.781200482846104));
#49931=DIRECTION('ref_axis',(0.781200482846104,0.,0.624280230025758));
#49932=DIRECTION('',(0.,1.,0.));
#49933=DIRECTION('center_axis',(-0.988679578606275,0.,-0.150042296859647));
#49934=DIRECTION('ref_axis',(-0.150042296859647,0.,0.988679578606275));
#49935=DIRECTION('',(0.,1.,0.));
#49936=DIRECTION('center_axis',(-0.364399348580519,0.,-0.931242779705751));
#49937=DIRECTION('ref_axis',(-0.931242779705751,0.,0.364399348580519));
#49938=DIRECTION('',(0.,1.,0.));
#49939=DIRECTION('center_axis',(0.624280230025758,0.,-0.781200482846105));
#49940=DIRECTION('ref_axis',(-0.781200482846105,0.,-0.624280230025758));
#49941=DIRECTION('center_axis',(0.988679578606276,0.,0.150042296859641));
#49942=DIRECTION('ref_axis',(0.150042296859641,0.,-0.988679578606276));
#49943=DIRECTION('',(0.,1.,0.));
#49944=DIRECTION('',(0.,1.,0.));
#49945=DIRECTION('center_axis',(0.364399348580517,0.,0.931242779705752));
#49946=DIRECTION('ref_axis',(0.931242779705752,0.,-0.364399348580517));
#49947=DIRECTION('',(0.,1.,0.));
#49948=DIRECTION('center_axis',(-0.624280230025758,0.,0.781200482846104));
#49949=DIRECTION('ref_axis',(0.781200482846104,0.,0.624280230025758));
#49950=DIRECTION('',(0.,1.,0.));
#49951=DIRECTION('center_axis',(-0.988679578606275,0.,-0.150042296859647));
#49952=DIRECTION('ref_axis',(-0.150042296859647,0.,0.988679578606275));
#49953=DIRECTION('',(0.,1.,0.));
#49954=DIRECTION('center_axis',(-0.364399348580519,0.,-0.931242779705751));
#49955=DIRECTION('ref_axis',(-0.931242779705751,0.,0.364399348580519));
#49956=DIRECTION('',(0.,1.,0.));
#49957=DIRECTION('center_axis',(0.624280230025758,0.,-0.781200482846105));
#49958=DIRECTION('ref_axis',(-0.781200482846105,0.,-0.624280230025758));
#49959=DIRECTION('center_axis',(0.988679578606276,0.,0.150042296859641));
#49960=DIRECTION('ref_axis',(0.150042296859641,0.,-0.988679578606276));
#49961=DIRECTION('',(0.,1.,0.));
#49962=DIRECTION('',(0.,1.,0.));
#49963=DIRECTION('center_axis',(0.364399348580517,0.,0.931242779705752));
#49964=DIRECTION('ref_axis',(0.931242779705752,0.,-0.364399348580517));
#49965=DIRECTION('',(0.,1.,0.));
#49966=DIRECTION('center_axis',(-0.624280230025758,0.,0.781200482846104));
#49967=DIRECTION('ref_axis',(0.781200482846104,0.,0.624280230025758));
#49968=DIRECTION('',(0.,1.,0.));
#49969=DIRECTION('center_axis',(-0.988679578606275,0.,-0.150042296859647));
#49970=DIRECTION('ref_axis',(-0.150042296859647,0.,0.988679578606275));
#49971=DIRECTION('',(0.,1.,0.));
#49972=DIRECTION('center_axis',(-0.364399348580519,0.,-0.931242779705751));
#49973=DIRECTION('ref_axis',(-0.931242779705751,0.,0.364399348580519));
#49974=DIRECTION('',(0.,1.,0.));
#49975=DIRECTION('center_axis',(0.624280230025758,0.,-0.781200482846105));
#49976=DIRECTION('ref_axis',(-0.781200482846105,0.,-0.624280230025758));
#49977=DIRECTION('center_axis',(0.988679578606276,0.,0.150042296859641));
#49978=DIRECTION('ref_axis',(0.150042296859641,0.,-0.988679578606276));
#49979=DIRECTION('',(0.,1.,0.));
#49980=DIRECTION('',(0.,1.,0.));
#49981=DIRECTION('center_axis',(0.364399348580517,0.,0.931242779705752));
#49982=DIRECTION('ref_axis',(0.931242779705752,0.,-0.364399348580517));
#49983=DIRECTION('',(0.,1.,0.));
#49984=DIRECTION('center_axis',(-0.624280230025758,0.,0.781200482846104));
#49985=DIRECTION('ref_axis',(0.781200482846104,0.,0.624280230025758));
#49986=DIRECTION('',(0.,1.,0.));
#49987=DIRECTION('center_axis',(-0.988679578606275,0.,-0.150042296859647));
#49988=DIRECTION('ref_axis',(-0.150042296859647,0.,0.988679578606275));
#49989=DIRECTION('',(0.,1.,0.));
#49990=DIRECTION('center_axis',(-0.364399348580519,0.,-0.931242779705751));
#49991=DIRECTION('ref_axis',(-0.931242779705751,0.,0.364399348580519));
#49992=DIRECTION('',(0.,1.,0.));
#49993=DIRECTION('center_axis',(0.624280230025758,0.,-0.781200482846105));
#49994=DIRECTION('ref_axis',(-0.781200482846105,0.,-0.624280230025758));
#49995=DIRECTION('center_axis',(0.988679578606276,0.,0.150042296859641));
#49996=DIRECTION('ref_axis',(0.150042296859641,0.,-0.988679578606276));
#49997=DIRECTION('',(0.,1.,0.));
#49998=DIRECTION('',(0.,1.,0.));
#49999=DIRECTION('center_axis',(0.364399348580517,0.,0.931242779705752));
#50000=DIRECTION('ref_axis',(0.931242779705752,0.,-0.364399348580517));
#50001=DIRECTION('',(0.,1.,0.));
#50002=DIRECTION('center_axis',(-0.624280230025758,0.,0.781200482846104));
#50003=DIRECTION('ref_axis',(0.781200482846104,0.,0.624280230025758));
#50004=DIRECTION('',(0.,1.,0.));
#50005=DIRECTION('center_axis',(-0.988679578606275,0.,-0.150042296859647));
#50006=DIRECTION('ref_axis',(-0.150042296859647,0.,0.988679578606275));
#50007=DIRECTION('',(0.,1.,0.));
#50008=DIRECTION('center_axis',(-0.364399348580519,0.,-0.931242779705751));
#50009=DIRECTION('ref_axis',(-0.931242779705751,0.,0.364399348580519));
#50010=DIRECTION('',(0.,1.,0.));
#50011=DIRECTION('center_axis',(0.624280230025758,0.,-0.781200482846105));
#50012=DIRECTION('ref_axis',(-0.781200482846105,0.,-0.624280230025758));
#50013=DIRECTION('center_axis',(0.988679578606276,0.,0.150042296859641));
#50014=DIRECTION('ref_axis',(0.150042296859641,0.,-0.988679578606276));
#50015=DIRECTION('',(0.,1.,0.));
#50016=DIRECTION('',(0.,1.,0.));
#50017=DIRECTION('center_axis',(0.364399348580517,0.,0.931242779705752));
#50018=DIRECTION('ref_axis',(0.931242779705752,0.,-0.364399348580517));
#50019=DIRECTION('',(0.,1.,0.));
#50020=DIRECTION('center_axis',(-0.624280230025758,0.,0.781200482846104));
#50021=DIRECTION('ref_axis',(0.781200482846104,0.,0.624280230025758));
#50022=DIRECTION('',(0.,1.,0.));
#50023=DIRECTION('center_axis',(-0.988679578606275,0.,-0.150042296859647));
#50024=DIRECTION('ref_axis',(-0.150042296859647,0.,0.988679578606275));
#50025=DIRECTION('',(0.,1.,0.));
#50026=DIRECTION('center_axis',(-0.364399348580519,0.,-0.931242779705751));
#50027=DIRECTION('ref_axis',(-0.931242779705751,0.,0.364399348580519));
#50028=DIRECTION('',(0.,1.,0.));
#50029=DIRECTION('center_axis',(0.624280230025758,0.,-0.781200482846105));
#50030=DIRECTION('ref_axis',(-0.781200482846105,0.,-0.624280230025758));
#50031=DIRECTION('center_axis',(0.988679578606276,0.,0.150042296859641));
#50032=DIRECTION('ref_axis',(0.150042296859641,0.,-0.988679578606276));
#50033=DIRECTION('',(0.,1.,0.));
#50034=DIRECTION('',(0.,1.,0.));
#50035=DIRECTION('center_axis',(0.364399348580517,0.,0.931242779705752));
#50036=DIRECTION('ref_axis',(0.931242779705752,0.,-0.364399348580517));
#50037=DIRECTION('',(0.,1.,0.));
#50038=DIRECTION('center_axis',(-0.624280230025758,0.,0.781200482846104));
#50039=DIRECTION('ref_axis',(0.781200482846104,0.,0.624280230025758));
#50040=DIRECTION('',(0.,1.,0.));
#50041=DIRECTION('center_axis',(-0.988679578606275,0.,-0.150042296859647));
#50042=DIRECTION('ref_axis',(-0.150042296859647,0.,0.988679578606275));
#50043=DIRECTION('',(0.,1.,0.));
#50044=DIRECTION('center_axis',(-0.364399348580519,0.,-0.931242779705751));
#50045=DIRECTION('ref_axis',(-0.931242779705751,0.,0.364399348580519));
#50046=DIRECTION('',(0.,1.,0.));
#50047=DIRECTION('center_axis',(0.624280230025758,0.,-0.781200482846105));
#50048=DIRECTION('ref_axis',(-0.781200482846105,0.,-0.624280230025758));
#50049=DIRECTION('center_axis',(0.988679578606276,0.,0.150042296859641));
#50050=DIRECTION('ref_axis',(0.150042296859641,0.,-0.988679578606276));
#50051=DIRECTION('',(0.,1.,0.));
#50052=DIRECTION('',(0.,1.,0.));
#50053=DIRECTION('center_axis',(0.364399348580517,0.,0.931242779705752));
#50054=DIRECTION('ref_axis',(0.931242779705752,0.,-0.364399348580517));
#50055=DIRECTION('',(0.,1.,0.));
#50056=DIRECTION('center_axis',(-0.624280230025758,0.,0.781200482846104));
#50057=DIRECTION('ref_axis',(0.781200482846104,0.,0.624280230025758));
#50058=DIRECTION('',(0.,1.,0.));
#50059=DIRECTION('center_axis',(-0.988679578606275,0.,-0.150042296859647));
#50060=DIRECTION('ref_axis',(-0.150042296859647,0.,0.988679578606275));
#50061=DIRECTION('',(0.,1.,0.));
#50062=DIRECTION('center_axis',(-0.364399348580519,0.,-0.931242779705751));
#50063=DIRECTION('ref_axis',(-0.931242779705751,0.,0.364399348580519));
#50064=DIRECTION('',(0.,1.,0.));
#50065=DIRECTION('center_axis',(0.624280230025758,0.,-0.781200482846105));
#50066=DIRECTION('ref_axis',(-0.781200482846105,0.,-0.624280230025758));
#50067=DIRECTION('center_axis',(0.988679578606276,0.,0.150042296859641));
#50068=DIRECTION('ref_axis',(0.150042296859641,0.,-0.988679578606276));
#50069=DIRECTION('',(0.,1.,0.));
#50070=DIRECTION('',(0.,1.,0.));
#50071=DIRECTION('center_axis',(0.364399348580517,0.,0.931242779705752));
#50072=DIRECTION('ref_axis',(0.931242779705752,0.,-0.364399348580517));
#50073=DIRECTION('',(0.,1.,0.));
#50074=DIRECTION('center_axis',(-0.624280230025758,0.,0.781200482846104));
#50075=DIRECTION('ref_axis',(0.781200482846104,0.,0.624280230025758));
#50076=DIRECTION('',(0.,1.,0.));
#50077=DIRECTION('center_axis',(-0.988679578606275,0.,-0.150042296859647));
#50078=DIRECTION('ref_axis',(-0.150042296859647,0.,0.988679578606275));
#50079=DIRECTION('',(0.,1.,0.));
#50080=DIRECTION('center_axis',(-0.364399348580519,0.,-0.931242779705751));
#50081=DIRECTION('ref_axis',(-0.931242779705751,0.,0.364399348580519));
#50082=DIRECTION('',(0.,1.,0.));
#50083=DIRECTION('center_axis',(0.624280230025758,0.,-0.781200482846105));
#50084=DIRECTION('ref_axis',(-0.781200482846105,0.,-0.624280230025758));
#50085=DIRECTION('center_axis',(0.988679578606276,0.,0.150042296859641));
#50086=DIRECTION('ref_axis',(0.150042296859641,0.,-0.988679578606276));
#50087=DIRECTION('',(0.,1.,0.));
#50088=DIRECTION('',(0.,1.,0.));
#50089=DIRECTION('center_axis',(0.364399348580517,0.,0.931242779705752));
#50090=DIRECTION('ref_axis',(0.931242779705752,0.,-0.364399348580517));
#50091=DIRECTION('',(0.,1.,0.));
#50092=DIRECTION('center_axis',(-0.624280230025758,0.,0.781200482846104));
#50093=DIRECTION('ref_axis',(0.781200482846104,0.,0.624280230025758));
#50094=DIRECTION('',(0.,1.,0.));
#50095=DIRECTION('center_axis',(-0.988679578606275,0.,-0.150042296859647));
#50096=DIRECTION('ref_axis',(-0.150042296859647,0.,0.988679578606275));
#50097=DIRECTION('',(0.,1.,0.));
#50098=DIRECTION('center_axis',(-0.364399348580519,0.,-0.931242779705751));
#50099=DIRECTION('ref_axis',(-0.931242779705751,0.,0.364399348580519));
#50100=DIRECTION('',(0.,1.,0.));
#50101=DIRECTION('center_axis',(0.624280230025758,0.,-0.781200482846105));
#50102=DIRECTION('ref_axis',(-0.781200482846105,0.,-0.624280230025758));
#50103=DIRECTION('center_axis',(0.988679578606276,0.,0.150042296859641));
#50104=DIRECTION('ref_axis',(0.150042296859641,0.,-0.988679578606276));
#50105=DIRECTION('',(0.,1.,0.));
#50106=DIRECTION('',(0.,1.,0.));
#50107=DIRECTION('center_axis',(0.364399348580517,0.,0.931242779705752));
#50108=DIRECTION('ref_axis',(0.931242779705752,0.,-0.364399348580517));
#50109=DIRECTION('',(0.,1.,0.));
#50110=DIRECTION('center_axis',(-0.624280230025758,0.,0.781200482846104));
#50111=DIRECTION('ref_axis',(0.781200482846104,0.,0.624280230025758));
#50112=DIRECTION('',(0.,1.,0.));
#50113=DIRECTION('center_axis',(-0.988679578606275,0.,-0.150042296859647));
#50114=DIRECTION('ref_axis',(-0.150042296859647,0.,0.988679578606275));
#50115=DIRECTION('',(0.,1.,0.));
#50116=DIRECTION('center_axis',(-0.364399348580519,0.,-0.931242779705751));
#50117=DIRECTION('ref_axis',(-0.931242779705751,0.,0.364399348580519));
#50118=DIRECTION('',(0.,1.,0.));
#50119=DIRECTION('center_axis',(0.624280230025758,0.,-0.781200482846105));
#50120=DIRECTION('ref_axis',(-0.781200482846105,0.,-0.624280230025758));
#50121=DIRECTION('center_axis',(0.988679578606276,0.,0.150042296859641));
#50122=DIRECTION('ref_axis',(0.150042296859641,0.,-0.988679578606276));
#50123=DIRECTION('',(0.,1.,0.));
#50124=DIRECTION('',(0.,1.,0.));
#50125=DIRECTION('center_axis',(0.364399348580517,0.,0.931242779705752));
#50126=DIRECTION('ref_axis',(0.931242779705752,0.,-0.364399348580517));
#50127=DIRECTION('',(0.,1.,0.));
#50128=DIRECTION('center_axis',(-0.624280230025758,0.,0.781200482846104));
#50129=DIRECTION('ref_axis',(0.781200482846104,0.,0.624280230025758));
#50130=DIRECTION('',(0.,1.,0.));
#50131=DIRECTION('center_axis',(-0.988679578606275,0.,-0.150042296859647));
#50132=DIRECTION('ref_axis',(-0.150042296859647,0.,0.988679578606275));
#50133=DIRECTION('',(0.,1.,0.));
#50134=DIRECTION('center_axis',(-0.364399348580519,0.,-0.931242779705751));
#50135=DIRECTION('ref_axis',(-0.931242779705751,0.,0.364399348580519));
#50136=DIRECTION('',(0.,1.,0.));
#50137=DIRECTION('center_axis',(0.624280230025758,0.,-0.781200482846105));
#50138=DIRECTION('ref_axis',(-0.781200482846105,0.,-0.624280230025758));
#50139=DIRECTION('center_axis',(0.988679578606276,0.,0.150042296859641));
#50140=DIRECTION('ref_axis',(0.150042296859641,0.,-0.988679578606276));
#50141=DIRECTION('',(0.,1.,0.));
#50142=DIRECTION('',(0.,1.,0.));
#50143=DIRECTION('center_axis',(0.364399348580517,0.,0.931242779705752));
#50144=DIRECTION('ref_axis',(0.931242779705752,0.,-0.364399348580517));
#50145=DIRECTION('',(0.,1.,0.));
#50146=DIRECTION('center_axis',(-0.624280230025758,0.,0.781200482846104));
#50147=DIRECTION('ref_axis',(0.781200482846104,0.,0.624280230025758));
#50148=DIRECTION('',(0.,1.,0.));
#50149=DIRECTION('center_axis',(-0.988679578606275,0.,-0.150042296859647));
#50150=DIRECTION('ref_axis',(-0.150042296859647,0.,0.988679578606275));
#50151=DIRECTION('',(0.,1.,0.));
#50152=DIRECTION('center_axis',(-0.364399348580519,0.,-0.931242779705751));
#50153=DIRECTION('ref_axis',(-0.931242779705751,0.,0.364399348580519));
#50154=DIRECTION('',(0.,1.,0.));
#50155=DIRECTION('center_axis',(0.624280230025758,0.,-0.781200482846105));
#50156=DIRECTION('ref_axis',(-0.781200482846105,0.,-0.624280230025758));
#50157=DIRECTION('center_axis',(0.988679578606276,0.,0.150042296859641));
#50158=DIRECTION('ref_axis',(0.150042296859641,0.,-0.988679578606276));
#50159=DIRECTION('',(0.,1.,0.));
#50160=DIRECTION('',(0.,1.,0.));
#50161=DIRECTION('center_axis',(0.364399348580517,0.,0.931242779705752));
#50162=DIRECTION('ref_axis',(0.931242779705752,0.,-0.364399348580517));
#50163=DIRECTION('',(0.,1.,0.));
#50164=DIRECTION('center_axis',(-0.624280230025758,0.,0.781200482846104));
#50165=DIRECTION('ref_axis',(0.781200482846104,0.,0.624280230025758));
#50166=DIRECTION('',(0.,1.,0.));
#50167=DIRECTION('center_axis',(-0.988679578606275,0.,-0.150042296859647));
#50168=DIRECTION('ref_axis',(-0.150042296859647,0.,0.988679578606275));
#50169=DIRECTION('',(0.,1.,0.));
#50170=DIRECTION('center_axis',(-0.364399348580519,0.,-0.931242779705751));
#50171=DIRECTION('ref_axis',(-0.931242779705751,0.,0.364399348580519));
#50172=DIRECTION('',(0.,1.,0.));
#50173=DIRECTION('center_axis',(0.624280230025758,0.,-0.781200482846105));
#50174=DIRECTION('ref_axis',(-0.781200482846105,0.,-0.624280230025758));
#50175=DIRECTION('center_axis',(0.988679578606276,0.,0.150042296859641));
#50176=DIRECTION('ref_axis',(0.150042296859641,0.,-0.988679578606276));
#50177=DIRECTION('',(0.,1.,0.));
#50178=DIRECTION('',(0.,1.,0.));
#50179=DIRECTION('center_axis',(0.364399348580517,0.,0.931242779705752));
#50180=DIRECTION('ref_axis',(0.931242779705752,0.,-0.364399348580517));
#50181=DIRECTION('',(0.,1.,0.));
#50182=DIRECTION('center_axis',(-0.624280230025758,0.,0.781200482846104));
#50183=DIRECTION('ref_axis',(0.781200482846104,0.,0.624280230025758));
#50184=DIRECTION('',(0.,1.,0.));
#50185=DIRECTION('center_axis',(-0.988679578606275,0.,-0.150042296859647));
#50186=DIRECTION('ref_axis',(-0.150042296859647,0.,0.988679578606275));
#50187=DIRECTION('',(0.,1.,0.));
#50188=DIRECTION('center_axis',(-0.364399348580519,0.,-0.931242779705751));
#50189=DIRECTION('ref_axis',(-0.931242779705751,0.,0.364399348580519));
#50190=DIRECTION('',(0.,1.,0.));
#50191=DIRECTION('center_axis',(0.624280230025758,0.,-0.781200482846105));
#50192=DIRECTION('ref_axis',(-0.781200482846105,0.,-0.624280230025758));
#50193=DIRECTION('center_axis',(0.988679578606276,0.,0.150042296859641));
#50194=DIRECTION('ref_axis',(0.150042296859641,0.,-0.988679578606276));
#50195=DIRECTION('',(0.,1.,0.));
#50196=DIRECTION('',(0.,1.,0.));
#50197=DIRECTION('center_axis',(0.364399348580517,0.,0.931242779705752));
#50198=DIRECTION('ref_axis',(0.931242779705752,0.,-0.364399348580517));
#50199=DIRECTION('',(0.,1.,0.));
#50200=DIRECTION('center_axis',(-0.624280230025758,0.,0.781200482846104));
#50201=DIRECTION('ref_axis',(0.781200482846104,0.,0.624280230025758));
#50202=DIRECTION('',(0.,1.,0.));
#50203=DIRECTION('center_axis',(-0.988679578606275,0.,-0.150042296859647));
#50204=DIRECTION('ref_axis',(-0.150042296859647,0.,0.988679578606275));
#50205=DIRECTION('',(0.,1.,0.));
#50206=DIRECTION('center_axis',(-0.364399348580519,0.,-0.931242779705751));
#50207=DIRECTION('ref_axis',(-0.931242779705751,0.,0.364399348580519));
#50208=DIRECTION('',(0.,1.,0.));
#50209=DIRECTION('center_axis',(0.624280230025758,0.,-0.781200482846105));
#50210=DIRECTION('ref_axis',(-0.781200482846105,0.,-0.624280230025758));
#50211=DIRECTION('center_axis',(0.988679578606276,0.,0.150042296859641));
#50212=DIRECTION('ref_axis',(0.150042296859641,0.,-0.988679578606276));
#50213=DIRECTION('',(0.,1.,0.));
#50214=DIRECTION('',(0.,1.,0.));
#50215=DIRECTION('center_axis',(0.364399348580517,0.,0.931242779705752));
#50216=DIRECTION('ref_axis',(0.931242779705752,0.,-0.364399348580517));
#50217=DIRECTION('',(0.,1.,0.));
#50218=DIRECTION('center_axis',(-0.624280230025758,0.,0.781200482846104));
#50219=DIRECTION('ref_axis',(0.781200482846104,0.,0.624280230025758));
#50220=DIRECTION('',(0.,1.,0.));
#50221=DIRECTION('center_axis',(-0.988679578606275,0.,-0.150042296859647));
#50222=DIRECTION('ref_axis',(-0.150042296859647,0.,0.988679578606275));
#50223=DIRECTION('',(0.,1.,0.));
#50224=DIRECTION('center_axis',(-0.364399348580519,0.,-0.931242779705751));
#50225=DIRECTION('ref_axis',(-0.931242779705751,0.,0.364399348580519));
#50226=DIRECTION('',(0.,1.,0.));
#50227=DIRECTION('center_axis',(0.624280230025758,0.,-0.781200482846105));
#50228=DIRECTION('ref_axis',(-0.781200482846105,0.,-0.624280230025758));
#50229=DIRECTION('center_axis',(0.988679578606276,0.,0.150042296859641));
#50230=DIRECTION('ref_axis',(0.150042296859641,0.,-0.988679578606276));
#50231=DIRECTION('',(0.,1.,0.));
#50232=DIRECTION('',(0.,1.,0.));
#50233=DIRECTION('center_axis',(0.364399348580517,0.,0.931242779705752));
#50234=DIRECTION('ref_axis',(0.931242779705752,0.,-0.364399348580517));
#50235=DIRECTION('',(0.,1.,0.));
#50236=DIRECTION('center_axis',(-0.624280230025758,0.,0.781200482846104));
#50237=DIRECTION('ref_axis',(0.781200482846104,0.,0.624280230025758));
#50238=DIRECTION('',(0.,1.,0.));
#50239=DIRECTION('center_axis',(-0.988679578606275,0.,-0.150042296859647));
#50240=DIRECTION('ref_axis',(-0.150042296859647,0.,0.988679578606275));
#50241=DIRECTION('',(0.,1.,0.));
#50242=DIRECTION('center_axis',(-0.364399348580519,0.,-0.931242779705751));
#50243=DIRECTION('ref_axis',(-0.931242779705751,0.,0.364399348580519));
#50244=DIRECTION('',(0.,1.,0.));
#50245=DIRECTION('center_axis',(0.624280230025758,0.,-0.781200482846105));
#50246=DIRECTION('ref_axis',(-0.781200482846105,0.,-0.624280230025758));
#50247=DIRECTION('center_axis',(0.988679578606276,0.,0.150042296859641));
#50248=DIRECTION('ref_axis',(0.150042296859641,0.,-0.988679578606276));
#50249=DIRECTION('',(0.,1.,0.));
#50250=DIRECTION('',(0.,1.,0.));
#50251=DIRECTION('center_axis',(0.364399348580517,0.,0.931242779705752));
#50252=DIRECTION('ref_axis',(0.931242779705752,0.,-0.364399348580517));
#50253=DIRECTION('',(0.,1.,0.));
#50254=DIRECTION('center_axis',(-0.624280230025758,0.,0.781200482846104));
#50255=DIRECTION('ref_axis',(0.781200482846104,0.,0.624280230025758));
#50256=DIRECTION('',(0.,1.,0.));
#50257=DIRECTION('center_axis',(-0.988679578606275,0.,-0.150042296859647));
#50258=DIRECTION('ref_axis',(-0.150042296859647,0.,0.988679578606275));
#50259=DIRECTION('',(0.,1.,0.));
#50260=DIRECTION('center_axis',(-0.364399348580519,0.,-0.931242779705751));
#50261=DIRECTION('ref_axis',(-0.931242779705751,0.,0.364399348580519));
#50262=DIRECTION('',(0.,1.,0.));
#50263=DIRECTION('center_axis',(0.624280230025758,0.,-0.781200482846105));
#50264=DIRECTION('ref_axis',(-0.781200482846105,0.,-0.624280230025758));
#50265=DIRECTION('center_axis',(0.988679578606276,0.,0.150042296859641));
#50266=DIRECTION('ref_axis',(0.150042296859641,0.,-0.988679578606276));
#50267=DIRECTION('',(0.,1.,0.));
#50268=DIRECTION('',(0.,1.,0.));
#50269=DIRECTION('center_axis',(0.364399348580517,0.,0.931242779705752));
#50270=DIRECTION('ref_axis',(0.931242779705752,0.,-0.364399348580517));
#50271=DIRECTION('',(0.,1.,0.));
#50272=DIRECTION('center_axis',(-0.624280230025758,0.,0.781200482846104));
#50273=DIRECTION('ref_axis',(0.781200482846104,0.,0.624280230025758));
#50274=DIRECTION('',(0.,1.,0.));
#50275=DIRECTION('center_axis',(-0.988679578606275,0.,-0.150042296859647));
#50276=DIRECTION('ref_axis',(-0.150042296859647,0.,0.988679578606275));
#50277=DIRECTION('',(0.,1.,0.));
#50278=DIRECTION('center_axis',(-0.364399348580519,0.,-0.931242779705751));
#50279=DIRECTION('ref_axis',(-0.931242779705751,0.,0.364399348580519));
#50280=DIRECTION('',(0.,1.,0.));
#50281=DIRECTION('center_axis',(0.624280230025758,0.,-0.781200482846105));
#50282=DIRECTION('ref_axis',(-0.781200482846105,0.,-0.624280230025758));
#50283=DIRECTION('center_axis',(0.988679578606276,0.,0.150042296859641));
#50284=DIRECTION('ref_axis',(0.150042296859641,0.,-0.988679578606276));
#50285=DIRECTION('',(0.,1.,0.));
#50286=DIRECTION('',(0.,1.,0.));
#50287=DIRECTION('center_axis',(0.364399348580517,0.,0.931242779705752));
#50288=DIRECTION('ref_axis',(0.931242779705752,0.,-0.364399348580517));
#50289=DIRECTION('',(0.,1.,0.));
#50290=DIRECTION('center_axis',(-0.624280230025758,0.,0.781200482846104));
#50291=DIRECTION('ref_axis',(0.781200482846104,0.,0.624280230025758));
#50292=DIRECTION('',(0.,1.,0.));
#50293=DIRECTION('center_axis',(-0.988679578606275,0.,-0.150042296859647));
#50294=DIRECTION('ref_axis',(-0.150042296859647,0.,0.988679578606275));
#50295=DIRECTION('',(0.,1.,0.));
#50296=DIRECTION('center_axis',(-0.364399348580519,0.,-0.931242779705751));
#50297=DIRECTION('ref_axis',(-0.931242779705751,0.,0.364399348580519));
#50298=DIRECTION('',(0.,1.,0.));
#50299=DIRECTION('center_axis',(0.624280230025758,0.,-0.781200482846105));
#50300=DIRECTION('ref_axis',(-0.781200482846105,0.,-0.624280230025758));
#50301=DIRECTION('center_axis',(0.988679578606276,0.,0.150042296859641));
#50302=DIRECTION('ref_axis',(0.150042296859641,0.,-0.988679578606276));
#50303=DIRECTION('',(0.,1.,0.));
#50304=DIRECTION('',(0.,1.,0.));
#50305=DIRECTION('center_axis',(0.364399348580517,0.,0.931242779705752));
#50306=DIRECTION('ref_axis',(0.931242779705752,0.,-0.364399348580517));
#50307=DIRECTION('',(0.,1.,0.));
#50308=DIRECTION('center_axis',(-0.624280230025758,0.,0.781200482846104));
#50309=DIRECTION('ref_axis',(0.781200482846104,0.,0.624280230025758));
#50310=DIRECTION('',(0.,1.,0.));
#50311=DIRECTION('center_axis',(-0.988679578606275,0.,-0.150042296859647));
#50312=DIRECTION('ref_axis',(-0.150042296859647,0.,0.988679578606275));
#50313=DIRECTION('',(0.,1.,0.));
#50314=DIRECTION('center_axis',(-0.364399348580519,0.,-0.931242779705751));
#50315=DIRECTION('ref_axis',(-0.931242779705751,0.,0.364399348580519));
#50316=DIRECTION('',(0.,1.,0.));
#50317=DIRECTION('center_axis',(0.624280230025758,0.,-0.781200482846105));
#50318=DIRECTION('ref_axis',(-0.781200482846105,0.,-0.624280230025758));
#50319=DIRECTION('center_axis',(0.988679578606276,0.,0.150042296859641));
#50320=DIRECTION('ref_axis',(0.150042296859641,0.,-0.988679578606276));
#50321=DIRECTION('',(0.,1.,0.));
#50322=DIRECTION('',(0.,1.,0.));
#50323=DIRECTION('center_axis',(0.364399348580517,0.,0.931242779705752));
#50324=DIRECTION('ref_axis',(0.931242779705752,0.,-0.364399348580517));
#50325=DIRECTION('',(0.,1.,0.));
#50326=DIRECTION('center_axis',(-0.624280230025758,0.,0.781200482846104));
#50327=DIRECTION('ref_axis',(0.781200482846104,0.,0.624280230025758));
#50328=DIRECTION('',(0.,1.,0.));
#50329=DIRECTION('center_axis',(-0.988679578606275,0.,-0.150042296859647));
#50330=DIRECTION('ref_axis',(-0.150042296859647,0.,0.988679578606275));
#50331=DIRECTION('',(0.,1.,0.));
#50332=DIRECTION('center_axis',(-0.364399348580519,0.,-0.931242779705751));
#50333=DIRECTION('ref_axis',(-0.931242779705751,0.,0.364399348580519));
#50334=DIRECTION('',(0.,1.,0.));
#50335=DIRECTION('center_axis',(0.624280230025758,0.,-0.781200482846105));
#50336=DIRECTION('ref_axis',(-0.781200482846105,0.,-0.624280230025758));
#50337=DIRECTION('center_axis',(0.988679578606276,0.,0.150042296859641));
#50338=DIRECTION('ref_axis',(0.150042296859641,0.,-0.988679578606276));
#50339=DIRECTION('',(0.,1.,0.));
#50340=DIRECTION('',(0.,1.,0.));
#50341=DIRECTION('center_axis',(0.364399348580517,0.,0.931242779705752));
#50342=DIRECTION('ref_axis',(0.931242779705752,0.,-0.364399348580517));
#50343=DIRECTION('',(0.,1.,0.));
#50344=DIRECTION('center_axis',(-0.624280230025758,0.,0.781200482846104));
#50345=DIRECTION('ref_axis',(0.781200482846104,0.,0.624280230025758));
#50346=DIRECTION('',(0.,1.,0.));
#50347=DIRECTION('center_axis',(-0.988679578606275,0.,-0.150042296859647));
#50348=DIRECTION('ref_axis',(-0.150042296859647,0.,0.988679578606275));
#50349=DIRECTION('',(0.,1.,0.));
#50350=DIRECTION('center_axis',(-0.364399348580519,0.,-0.931242779705751));
#50351=DIRECTION('ref_axis',(-0.931242779705751,0.,0.364399348580519));
#50352=DIRECTION('',(0.,1.,0.));
#50353=DIRECTION('center_axis',(0.624280230025758,0.,-0.781200482846105));
#50354=DIRECTION('ref_axis',(-0.781200482846105,0.,-0.624280230025758));
#50355=DIRECTION('center_axis',(0.988679578606276,0.,0.150042296859641));
#50356=DIRECTION('ref_axis',(0.150042296859641,0.,-0.988679578606276));
#50357=DIRECTION('',(0.,1.,0.));
#50358=DIRECTION('',(0.,1.,0.));
#50359=DIRECTION('center_axis',(0.364399348580517,0.,0.931242779705752));
#50360=DIRECTION('ref_axis',(0.931242779705752,0.,-0.364399348580517));
#50361=DIRECTION('',(0.,1.,0.));
#50362=DIRECTION('center_axis',(-0.624280230025758,0.,0.781200482846104));
#50363=DIRECTION('ref_axis',(0.781200482846104,0.,0.624280230025758));
#50364=DIRECTION('',(0.,1.,0.));
#50365=DIRECTION('center_axis',(-0.988679578606275,0.,-0.150042296859647));
#50366=DIRECTION('ref_axis',(-0.150042296859647,0.,0.988679578606275));
#50367=DIRECTION('',(0.,1.,0.));
#50368=DIRECTION('center_axis',(-0.364399348580519,0.,-0.931242779705751));
#50369=DIRECTION('ref_axis',(-0.931242779705751,0.,0.364399348580519));
#50370=DIRECTION('',(0.,1.,0.));
#50371=DIRECTION('center_axis',(0.624280230025758,0.,-0.781200482846105));
#50372=DIRECTION('ref_axis',(-0.781200482846105,0.,-0.624280230025758));
#50373=DIRECTION('center_axis',(0.988679578606276,0.,0.150042296859641));
#50374=DIRECTION('ref_axis',(0.150042296859641,0.,-0.988679578606276));
#50375=DIRECTION('',(0.,1.,0.));
#50376=DIRECTION('',(0.,1.,0.));
#50377=DIRECTION('center_axis',(0.364399348580517,0.,0.931242779705752));
#50378=DIRECTION('ref_axis',(0.931242779705752,0.,-0.364399348580517));
#50379=DIRECTION('',(0.,1.,0.));
#50380=DIRECTION('center_axis',(-0.624280230025758,0.,0.781200482846104));
#50381=DIRECTION('ref_axis',(0.781200482846104,0.,0.624280230025758));
#50382=DIRECTION('',(0.,1.,0.));
#50383=DIRECTION('center_axis',(-0.988679578606275,0.,-0.150042296859647));
#50384=DIRECTION('ref_axis',(-0.150042296859647,0.,0.988679578606275));
#50385=DIRECTION('',(0.,1.,0.));
#50386=DIRECTION('center_axis',(-0.364399348580519,0.,-0.931242779705751));
#50387=DIRECTION('ref_axis',(-0.931242779705751,0.,0.364399348580519));
#50388=DIRECTION('',(0.,1.,0.));
#50389=DIRECTION('center_axis',(0.624280230025758,0.,-0.781200482846105));
#50390=DIRECTION('ref_axis',(-0.781200482846105,0.,-0.624280230025758));
#50391=DIRECTION('center_axis',(0.988679578606276,0.,0.150042296859641));
#50392=DIRECTION('ref_axis',(0.150042296859641,0.,-0.988679578606276));
#50393=DIRECTION('',(0.,1.,0.));
#50394=DIRECTION('',(0.,1.,0.));
#50395=DIRECTION('center_axis',(0.364399348580517,0.,0.931242779705752));
#50396=DIRECTION('ref_axis',(0.931242779705752,0.,-0.364399348580517));
#50397=DIRECTION('',(0.,1.,0.));
#50398=DIRECTION('center_axis',(-0.624280230025758,0.,0.781200482846104));
#50399=DIRECTION('ref_axis',(0.781200482846104,0.,0.624280230025758));
#50400=DIRECTION('',(0.,1.,0.));
#50401=DIRECTION('center_axis',(-0.988679578606275,0.,-0.150042296859647));
#50402=DIRECTION('ref_axis',(-0.150042296859647,0.,0.988679578606275));
#50403=DIRECTION('',(0.,1.,0.));
#50404=DIRECTION('center_axis',(-0.364399348580519,0.,-0.931242779705751));
#50405=DIRECTION('ref_axis',(-0.931242779705751,0.,0.364399348580519));
#50406=DIRECTION('',(0.,1.,0.));
#50407=DIRECTION('center_axis',(0.624280230025758,0.,-0.781200482846105));
#50408=DIRECTION('ref_axis',(-0.781200482846105,0.,-0.624280230025758));
#50409=DIRECTION('center_axis',(0.988679578606276,0.,0.150042296859641));
#50410=DIRECTION('ref_axis',(0.150042296859641,0.,-0.988679578606276));
#50411=DIRECTION('',(0.,1.,0.));
#50412=DIRECTION('',(0.,1.,0.));
#50413=DIRECTION('center_axis',(0.364399348580517,0.,0.931242779705752));
#50414=DIRECTION('ref_axis',(0.931242779705752,0.,-0.364399348580517));
#50415=DIRECTION('',(0.,1.,0.));
#50416=DIRECTION('center_axis',(-0.624280230025758,0.,0.781200482846104));
#50417=DIRECTION('ref_axis',(0.781200482846104,0.,0.624280230025758));
#50418=DIRECTION('',(0.,1.,0.));
#50419=DIRECTION('center_axis',(-0.988679578606275,0.,-0.150042296859647));
#50420=DIRECTION('ref_axis',(-0.150042296859647,0.,0.988679578606275));
#50421=DIRECTION('',(0.,1.,0.));
#50422=DIRECTION('center_axis',(-0.364399348580519,0.,-0.931242779705751));
#50423=DIRECTION('ref_axis',(-0.931242779705751,0.,0.364399348580519));
#50424=DIRECTION('',(0.,1.,0.));
#50425=DIRECTION('center_axis',(0.624280230025758,0.,-0.781200482846105));
#50426=DIRECTION('ref_axis',(-0.781200482846105,0.,-0.624280230025758));
#50427=DIRECTION('center_axis',(0.988679578606276,0.,0.150042296859641));
#50428=DIRECTION('ref_axis',(0.150042296859641,0.,-0.988679578606276));
#50429=DIRECTION('',(0.,1.,0.));
#50430=DIRECTION('',(0.,1.,0.));
#50431=DIRECTION('center_axis',(0.364399348580517,0.,0.931242779705752));
#50432=DIRECTION('ref_axis',(0.931242779705752,0.,-0.364399348580517));
#50433=DIRECTION('',(0.,1.,0.));
#50434=DIRECTION('center_axis',(-0.624280230025758,0.,0.781200482846104));
#50435=DIRECTION('ref_axis',(0.781200482846104,0.,0.624280230025758));
#50436=DIRECTION('',(0.,1.,0.));
#50437=DIRECTION('center_axis',(-0.988679578606275,0.,-0.150042296859647));
#50438=DIRECTION('ref_axis',(-0.150042296859647,0.,0.988679578606275));
#50439=DIRECTION('',(0.,1.,0.));
#50440=DIRECTION('center_axis',(-0.364399348580519,0.,-0.931242779705751));
#50441=DIRECTION('ref_axis',(-0.931242779705751,0.,0.364399348580519));
#50442=DIRECTION('',(0.,1.,0.));
#50443=DIRECTION('center_axis',(0.624280230025758,0.,-0.781200482846105));
#50444=DIRECTION('ref_axis',(-0.781200482846105,0.,-0.624280230025758));
#50445=DIRECTION('center_axis',(0.988679578606276,0.,0.150042296859641));
#50446=DIRECTION('ref_axis',(0.150042296859641,0.,-0.988679578606276));
#50447=DIRECTION('',(0.,1.,0.));
#50448=DIRECTION('',(0.,1.,0.));
#50449=DIRECTION('center_axis',(0.364399348580517,0.,0.931242779705752));
#50450=DIRECTION('ref_axis',(0.931242779705752,0.,-0.364399348580517));
#50451=DIRECTION('',(0.,1.,0.));
#50452=DIRECTION('center_axis',(-0.624280230025758,0.,0.781200482846104));
#50453=DIRECTION('ref_axis',(0.781200482846104,0.,0.624280230025758));
#50454=DIRECTION('',(0.,1.,0.));
#50455=DIRECTION('center_axis',(-0.988679578606275,0.,-0.150042296859647));
#50456=DIRECTION('ref_axis',(-0.150042296859647,0.,0.988679578606275));
#50457=DIRECTION('',(0.,1.,0.));
#50458=DIRECTION('center_axis',(-0.364399348580519,0.,-0.931242779705751));
#50459=DIRECTION('ref_axis',(-0.931242779705751,0.,0.364399348580519));
#50460=DIRECTION('',(0.,1.,0.));
#50461=DIRECTION('center_axis',(0.624280230025758,0.,-0.781200482846105));
#50462=DIRECTION('ref_axis',(-0.781200482846105,0.,-0.624280230025758));
#50463=DIRECTION('center_axis',(0.988679578606276,0.,0.150042296859641));
#50464=DIRECTION('ref_axis',(0.150042296859641,0.,-0.988679578606276));
#50465=DIRECTION('',(0.,1.,0.));
#50466=DIRECTION('',(0.,1.,0.));
#50467=DIRECTION('center_axis',(0.364399348580517,0.,0.931242779705752));
#50468=DIRECTION('ref_axis',(0.931242779705752,0.,-0.364399348580517));
#50469=DIRECTION('',(0.,1.,0.));
#50470=DIRECTION('center_axis',(-0.624280230025758,0.,0.781200482846104));
#50471=DIRECTION('ref_axis',(0.781200482846104,0.,0.624280230025758));
#50472=DIRECTION('',(0.,1.,0.));
#50473=DIRECTION('center_axis',(-0.988679578606275,0.,-0.150042296859647));
#50474=DIRECTION('ref_axis',(-0.150042296859647,0.,0.988679578606275));
#50475=DIRECTION('',(0.,1.,0.));
#50476=DIRECTION('center_axis',(-0.364399348580519,0.,-0.931242779705751));
#50477=DIRECTION('ref_axis',(-0.931242779705751,0.,0.364399348580519));
#50478=DIRECTION('',(0.,1.,0.));
#50479=DIRECTION('center_axis',(0.624280230025758,0.,-0.781200482846105));
#50480=DIRECTION('ref_axis',(-0.781200482846105,0.,-0.624280230025758));
#50481=DIRECTION('center_axis',(0.988679578606276,0.,0.150042296859641));
#50482=DIRECTION('ref_axis',(0.150042296859641,0.,-0.988679578606276));
#50483=DIRECTION('',(0.,1.,0.));
#50484=DIRECTION('',(0.,1.,0.));
#50485=DIRECTION('center_axis',(0.364399348580517,0.,0.931242779705752));
#50486=DIRECTION('ref_axis',(0.931242779705752,0.,-0.364399348580517));
#50487=DIRECTION('',(0.,1.,0.));
#50488=DIRECTION('center_axis',(-0.624280230025758,0.,0.781200482846104));
#50489=DIRECTION('ref_axis',(0.781200482846104,0.,0.624280230025758));
#50490=DIRECTION('',(0.,1.,0.));
#50491=DIRECTION('center_axis',(-0.988679578606275,0.,-0.150042296859647));
#50492=DIRECTION('ref_axis',(-0.150042296859647,0.,0.988679578606275));
#50493=DIRECTION('',(0.,1.,0.));
#50494=DIRECTION('center_axis',(-0.364399348580519,0.,-0.931242779705751));
#50495=DIRECTION('ref_axis',(-0.931242779705751,0.,0.364399348580519));
#50496=DIRECTION('',(0.,1.,0.));
#50497=DIRECTION('center_axis',(0.624280230025758,0.,-0.781200482846105));
#50498=DIRECTION('ref_axis',(-0.781200482846105,0.,-0.624280230025758));
#50499=DIRECTION('center_axis',(0.988679578606276,0.,0.150042296859641));
#50500=DIRECTION('ref_axis',(0.150042296859641,0.,-0.988679578606276));
#50501=DIRECTION('',(0.,1.,0.));
#50502=DIRECTION('',(0.,1.,0.));
#50503=DIRECTION('center_axis',(0.364399348580517,0.,0.931242779705752));
#50504=DIRECTION('ref_axis',(0.931242779705752,0.,-0.364399348580517));
#50505=DIRECTION('',(0.,1.,0.));
#50506=DIRECTION('center_axis',(-0.624280230025758,0.,0.781200482846104));
#50507=DIRECTION('ref_axis',(0.781200482846104,0.,0.624280230025758));
#50508=DIRECTION('',(0.,1.,0.));
#50509=DIRECTION('center_axis',(-0.988679578606275,0.,-0.150042296859647));
#50510=DIRECTION('ref_axis',(-0.150042296859647,0.,0.988679578606275));
#50511=DIRECTION('',(0.,1.,0.));
#50512=DIRECTION('center_axis',(-0.364399348580519,0.,-0.931242779705751));
#50513=DIRECTION('ref_axis',(-0.931242779705751,0.,0.364399348580519));
#50514=DIRECTION('',(0.,1.,0.));
#50515=DIRECTION('center_axis',(0.624280230025758,0.,-0.781200482846105));
#50516=DIRECTION('ref_axis',(-0.781200482846105,0.,-0.624280230025758));
#50517=DIRECTION('center_axis',(0.988679578606276,0.,0.150042296859641));
#50518=DIRECTION('ref_axis',(0.150042296859641,0.,-0.988679578606276));
#50519=DIRECTION('',(0.,1.,0.));
#50520=DIRECTION('',(0.,1.,0.));
#50521=DIRECTION('center_axis',(0.364399348580517,0.,0.931242779705752));
#50522=DIRECTION('ref_axis',(0.931242779705752,0.,-0.364399348580517));
#50523=DIRECTION('',(0.,1.,0.));
#50524=DIRECTION('center_axis',(-0.624280230025758,0.,0.781200482846104));
#50525=DIRECTION('ref_axis',(0.781200482846104,0.,0.624280230025758));
#50526=DIRECTION('',(0.,1.,0.));
#50527=DIRECTION('center_axis',(-0.988679578606275,0.,-0.150042296859647));
#50528=DIRECTION('ref_axis',(-0.150042296859647,0.,0.988679578606275));
#50529=DIRECTION('',(0.,1.,0.));
#50530=DIRECTION('center_axis',(-0.364399348580519,0.,-0.931242779705751));
#50531=DIRECTION('ref_axis',(-0.931242779705751,0.,0.364399348580519));
#50532=DIRECTION('',(0.,1.,0.));
#50533=DIRECTION('center_axis',(0.624280230025758,0.,-0.781200482846105));
#50534=DIRECTION('ref_axis',(-0.781200482846105,0.,-0.624280230025758));
#50535=DIRECTION('center_axis',(0.988679578606276,0.,0.150042296859641));
#50536=DIRECTION('ref_axis',(0.150042296859641,0.,-0.988679578606276));
#50537=DIRECTION('',(0.,1.,0.));
#50538=DIRECTION('',(0.,1.,0.));
#50539=DIRECTION('center_axis',(0.364399348580517,0.,0.931242779705752));
#50540=DIRECTION('ref_axis',(0.931242779705752,0.,-0.364399348580517));
#50541=DIRECTION('',(0.,1.,0.));
#50542=DIRECTION('center_axis',(-0.624280230025758,0.,0.781200482846104));
#50543=DIRECTION('ref_axis',(0.781200482846104,0.,0.624280230025758));
#50544=DIRECTION('',(0.,1.,0.));
#50545=DIRECTION('center_axis',(-0.988679578606275,0.,-0.150042296859647));
#50546=DIRECTION('ref_axis',(-0.150042296859647,0.,0.988679578606275));
#50547=DIRECTION('',(0.,1.,0.));
#50548=DIRECTION('center_axis',(-0.364399348580519,0.,-0.931242779705751));
#50549=DIRECTION('ref_axis',(-0.931242779705751,0.,0.364399348580519));
#50550=DIRECTION('',(0.,1.,0.));
#50551=DIRECTION('center_axis',(0.624280230025758,0.,-0.781200482846105));
#50552=DIRECTION('ref_axis',(-0.781200482846105,0.,-0.624280230025758));
#50553=DIRECTION('center_axis',(0.988679578606276,0.,0.150042296859641));
#50554=DIRECTION('ref_axis',(0.150042296859641,0.,-0.988679578606276));
#50555=DIRECTION('',(0.,1.,0.));
#50556=DIRECTION('',(0.,1.,0.));
#50557=DIRECTION('center_axis',(0.364399348580517,0.,0.931242779705752));
#50558=DIRECTION('ref_axis',(0.931242779705752,0.,-0.364399348580517));
#50559=DIRECTION('',(0.,1.,0.));
#50560=DIRECTION('center_axis',(-0.624280230025758,0.,0.781200482846104));
#50561=DIRECTION('ref_axis',(0.781200482846104,0.,0.624280230025758));
#50562=DIRECTION('',(0.,1.,0.));
#50563=DIRECTION('center_axis',(-0.988679578606275,0.,-0.150042296859647));
#50564=DIRECTION('ref_axis',(-0.150042296859647,0.,0.988679578606275));
#50565=DIRECTION('',(0.,1.,0.));
#50566=DIRECTION('center_axis',(-0.364399348580519,0.,-0.931242779705751));
#50567=DIRECTION('ref_axis',(-0.931242779705751,0.,0.364399348580519));
#50568=DIRECTION('',(0.,1.,0.));
#50569=DIRECTION('center_axis',(0.624280230025758,0.,-0.781200482846105));
#50570=DIRECTION('ref_axis',(-0.781200482846105,0.,-0.624280230025758));
#50571=DIRECTION('center_axis',(0.988679578606276,0.,0.150042296859641));
#50572=DIRECTION('ref_axis',(0.150042296859641,0.,-0.988679578606276));
#50573=DIRECTION('',(0.,1.,0.));
#50574=DIRECTION('',(0.,1.,0.));
#50575=DIRECTION('center_axis',(0.364399348580517,0.,0.931242779705752));
#50576=DIRECTION('ref_axis',(0.931242779705752,0.,-0.364399348580517));
#50577=DIRECTION('',(0.,1.,0.));
#50578=DIRECTION('center_axis',(-0.624280230025758,0.,0.781200482846104));
#50579=DIRECTION('ref_axis',(0.781200482846104,0.,0.624280230025758));
#50580=DIRECTION('',(0.,1.,0.));
#50581=DIRECTION('center_axis',(-0.988679578606275,0.,-0.150042296859647));
#50582=DIRECTION('ref_axis',(-0.150042296859647,0.,0.988679578606275));
#50583=DIRECTION('',(0.,1.,0.));
#50584=DIRECTION('center_axis',(-0.364399348580519,0.,-0.931242779705751));
#50585=DIRECTION('ref_axis',(-0.931242779705751,0.,0.364399348580519));
#50586=DIRECTION('',(0.,1.,0.));
#50587=DIRECTION('center_axis',(0.624280230025758,0.,-0.781200482846105));
#50588=DIRECTION('ref_axis',(-0.781200482846105,0.,-0.624280230025758));
#50589=DIRECTION('center_axis',(0.988679578606276,0.,0.150042296859641));
#50590=DIRECTION('ref_axis',(0.150042296859641,0.,-0.988679578606276));
#50591=DIRECTION('',(0.,1.,0.));
#50592=DIRECTION('',(0.,1.,0.));
#50593=DIRECTION('center_axis',(0.364399348580517,0.,0.931242779705752));
#50594=DIRECTION('ref_axis',(0.931242779705752,0.,-0.364399348580517));
#50595=DIRECTION('',(0.,1.,0.));
#50596=DIRECTION('center_axis',(-0.624280230025758,0.,0.781200482846104));
#50597=DIRECTION('ref_axis',(0.781200482846104,0.,0.624280230025758));
#50598=DIRECTION('',(0.,1.,0.));
#50599=DIRECTION('center_axis',(-0.988679578606275,0.,-0.150042296859647));
#50600=DIRECTION('ref_axis',(-0.150042296859647,0.,0.988679578606275));
#50601=DIRECTION('',(0.,1.,0.));
#50602=DIRECTION('center_axis',(-0.364399348580519,0.,-0.931242779705751));
#50603=DIRECTION('ref_axis',(-0.931242779705751,0.,0.364399348580519));
#50604=DIRECTION('',(0.,1.,0.));
#50605=DIRECTION('center_axis',(0.624280230025758,0.,-0.781200482846105));
#50606=DIRECTION('ref_axis',(-0.781200482846105,0.,-0.624280230025758));
#50607=DIRECTION('center_axis',(0.988679578606276,0.,0.150042296859641));
#50608=DIRECTION('ref_axis',(0.150042296859641,0.,-0.988679578606276));
#50609=DIRECTION('',(0.,1.,0.));
#50610=DIRECTION('',(0.,1.,0.));
#50611=DIRECTION('center_axis',(0.364399348580517,0.,0.931242779705752));
#50612=DIRECTION('ref_axis',(0.931242779705752,0.,-0.364399348580517));
#50613=DIRECTION('',(0.,1.,0.));
#50614=DIRECTION('center_axis',(-0.624280230025758,0.,0.781200482846104));
#50615=DIRECTION('ref_axis',(0.781200482846104,0.,0.624280230025758));
#50616=DIRECTION('',(0.,1.,0.));
#50617=DIRECTION('center_axis',(-0.988679578606275,0.,-0.150042296859647));
#50618=DIRECTION('ref_axis',(-0.150042296859647,0.,0.988679578606275));
#50619=DIRECTION('',(0.,1.,0.));
#50620=DIRECTION('center_axis',(-0.364399348580519,0.,-0.931242779705751));
#50621=DIRECTION('ref_axis',(-0.931242779705751,0.,0.364399348580519));
#50622=DIRECTION('',(0.,1.,0.));
#50623=DIRECTION('center_axis',(0.624280230025758,0.,-0.781200482846105));
#50624=DIRECTION('ref_axis',(-0.781200482846105,0.,-0.624280230025758));
#50625=DIRECTION('center_axis',(0.988679578606276,0.,0.150042296859641));
#50626=DIRECTION('ref_axis',(0.150042296859641,0.,-0.988679578606276));
#50627=DIRECTION('',(0.,1.,0.));
#50628=DIRECTION('',(0.,1.,0.));
#50629=DIRECTION('center_axis',(0.364399348580517,0.,0.931242779705752));
#50630=DIRECTION('ref_axis',(0.931242779705752,0.,-0.364399348580517));
#50631=DIRECTION('',(0.,1.,0.));
#50632=DIRECTION('center_axis',(-0.624280230025758,0.,0.781200482846104));
#50633=DIRECTION('ref_axis',(0.781200482846104,0.,0.624280230025758));
#50634=DIRECTION('',(0.,1.,0.));
#50635=DIRECTION('center_axis',(-0.988679578606275,0.,-0.150042296859647));
#50636=DIRECTION('ref_axis',(-0.150042296859647,0.,0.988679578606275));
#50637=DIRECTION('',(0.,1.,0.));
#50638=DIRECTION('center_axis',(-0.364399348580519,0.,-0.931242779705751));
#50639=DIRECTION('ref_axis',(-0.931242779705751,0.,0.364399348580519));
#50640=DIRECTION('',(0.,1.,0.));
#50641=DIRECTION('center_axis',(0.624280230025758,0.,-0.781200482846105));
#50642=DIRECTION('ref_axis',(-0.781200482846105,0.,-0.624280230025758));
#50643=DIRECTION('center_axis',(0.988679578606276,0.,0.150042296859641));
#50644=DIRECTION('ref_axis',(0.150042296859641,0.,-0.988679578606276));
#50645=DIRECTION('',(0.,1.,0.));
#50646=DIRECTION('',(0.,1.,0.));
#50647=DIRECTION('center_axis',(0.364399348580517,0.,0.931242779705752));
#50648=DIRECTION('ref_axis',(0.931242779705752,0.,-0.364399348580517));
#50649=DIRECTION('',(0.,1.,0.));
#50650=DIRECTION('center_axis',(-0.624280230025758,0.,0.781200482846104));
#50651=DIRECTION('ref_axis',(0.781200482846104,0.,0.624280230025758));
#50652=DIRECTION('',(0.,1.,0.));
#50653=DIRECTION('center_axis',(-0.988679578606275,0.,-0.150042296859647));
#50654=DIRECTION('ref_axis',(-0.150042296859647,0.,0.988679578606275));
#50655=DIRECTION('',(0.,1.,0.));
#50656=DIRECTION('center_axis',(-0.364399348580519,0.,-0.931242779705751));
#50657=DIRECTION('ref_axis',(-0.931242779705751,0.,0.364399348580519));
#50658=DIRECTION('',(0.,1.,0.));
#50659=DIRECTION('center_axis',(0.624280230025758,0.,-0.781200482846105));
#50660=DIRECTION('ref_axis',(-0.781200482846105,0.,-0.624280230025758));
#50661=DIRECTION('center_axis',(0.988679578606276,0.,0.150042296859641));
#50662=DIRECTION('ref_axis',(0.150042296859641,0.,-0.988679578606276));
#50663=DIRECTION('',(0.,1.,0.));
#50664=DIRECTION('',(0.,1.,0.));
#50665=DIRECTION('center_axis',(0.364399348580517,0.,0.931242779705752));
#50666=DIRECTION('ref_axis',(0.931242779705752,0.,-0.364399348580517));
#50667=DIRECTION('',(0.,1.,0.));
#50668=DIRECTION('center_axis',(-0.624280230025758,0.,0.781200482846104));
#50669=DIRECTION('ref_axis',(0.781200482846104,0.,0.624280230025758));
#50670=DIRECTION('',(0.,1.,0.));
#50671=DIRECTION('center_axis',(-0.988679578606275,0.,-0.150042296859647));
#50672=DIRECTION('ref_axis',(-0.150042296859647,0.,0.988679578606275));
#50673=DIRECTION('',(0.,1.,0.));
#50674=DIRECTION('center_axis',(-0.364399348580519,0.,-0.931242779705751));
#50675=DIRECTION('ref_axis',(-0.931242779705751,0.,0.364399348580519));
#50676=DIRECTION('',(0.,1.,0.));
#50677=DIRECTION('center_axis',(0.624280230025758,0.,-0.781200482846105));
#50678=DIRECTION('ref_axis',(-0.781200482846105,0.,-0.624280230025758));
#50679=DIRECTION('center_axis',(0.988679578606276,0.,0.150042296859641));
#50680=DIRECTION('ref_axis',(0.150042296859641,0.,-0.988679578606276));
#50681=DIRECTION('',(0.,1.,0.));
#50682=DIRECTION('',(0.,1.,0.));
#50683=DIRECTION('center_axis',(0.364399348580517,0.,0.931242779705752));
#50684=DIRECTION('ref_axis',(0.931242779705752,0.,-0.364399348580517));
#50685=DIRECTION('',(0.,1.,0.));
#50686=DIRECTION('center_axis',(-0.624280230025758,0.,0.781200482846104));
#50687=DIRECTION('ref_axis',(0.781200482846104,0.,0.624280230025758));
#50688=DIRECTION('',(0.,1.,0.));
#50689=DIRECTION('center_axis',(-0.988679578606275,0.,-0.150042296859647));
#50690=DIRECTION('ref_axis',(-0.150042296859647,0.,0.988679578606275));
#50691=DIRECTION('',(0.,1.,0.));
#50692=DIRECTION('center_axis',(-0.364399348580519,0.,-0.931242779705751));
#50693=DIRECTION('ref_axis',(-0.931242779705751,0.,0.364399348580519));
#50694=DIRECTION('',(0.,1.,0.));
#50695=DIRECTION('center_axis',(0.624280230025758,0.,-0.781200482846105));
#50696=DIRECTION('ref_axis',(-0.781200482846105,0.,-0.624280230025758));
#50697=DIRECTION('center_axis',(0.988679578606276,0.,0.150042296859641));
#50698=DIRECTION('ref_axis',(0.150042296859641,0.,-0.988679578606276));
#50699=DIRECTION('',(0.,1.,0.));
#50700=DIRECTION('',(0.,1.,0.));
#50701=DIRECTION('center_axis',(0.364399348580517,0.,0.931242779705752));
#50702=DIRECTION('ref_axis',(0.931242779705752,0.,-0.364399348580517));
#50703=DIRECTION('',(0.,1.,0.));
#50704=DIRECTION('center_axis',(-0.624280230025758,0.,0.781200482846104));
#50705=DIRECTION('ref_axis',(0.781200482846104,0.,0.624280230025758));
#50706=DIRECTION('',(0.,1.,0.));
#50707=DIRECTION('center_axis',(-0.988679578606275,0.,-0.150042296859647));
#50708=DIRECTION('ref_axis',(-0.150042296859647,0.,0.988679578606275));
#50709=DIRECTION('',(0.,1.,0.));
#50710=DIRECTION('center_axis',(-0.364399348580519,0.,-0.931242779705751));
#50711=DIRECTION('ref_axis',(-0.931242779705751,0.,0.364399348580519));
#50712=DIRECTION('',(0.,1.,0.));
#50713=DIRECTION('center_axis',(0.624280230025758,0.,-0.781200482846105));
#50714=DIRECTION('ref_axis',(-0.781200482846105,0.,-0.624280230025758));
#50715=DIRECTION('center_axis',(0.988679578606276,0.,0.150042296859641));
#50716=DIRECTION('ref_axis',(0.150042296859641,0.,-0.988679578606276));
#50717=DIRECTION('',(0.,1.,0.));
#50718=DIRECTION('',(0.,1.,0.));
#50719=DIRECTION('center_axis',(0.364399348580517,0.,0.931242779705752));
#50720=DIRECTION('ref_axis',(0.931242779705752,0.,-0.364399348580517));
#50721=DIRECTION('',(0.,1.,0.));
#50722=DIRECTION('center_axis',(-0.624280230025758,0.,0.781200482846104));
#50723=DIRECTION('ref_axis',(0.781200482846104,0.,0.624280230025758));
#50724=DIRECTION('',(0.,1.,0.));
#50725=DIRECTION('center_axis',(-0.988679578606275,0.,-0.150042296859647));
#50726=DIRECTION('ref_axis',(-0.150042296859647,0.,0.988679578606275));
#50727=DIRECTION('',(0.,1.,0.));
#50728=DIRECTION('center_axis',(-0.364399348580519,0.,-0.931242779705751));
#50729=DIRECTION('ref_axis',(-0.931242779705751,0.,0.364399348580519));
#50730=DIRECTION('',(0.,1.,0.));
#50731=DIRECTION('center_axis',(0.624280230025758,0.,-0.781200482846105));
#50732=DIRECTION('ref_axis',(-0.781200482846105,0.,-0.624280230025758));
#50733=DIRECTION('center_axis',(0.988679578606276,0.,0.150042296859641));
#50734=DIRECTION('ref_axis',(0.150042296859641,0.,-0.988679578606276));
#50735=DIRECTION('',(0.,1.,0.));
#50736=DIRECTION('',(0.,1.,0.));
#50737=DIRECTION('center_axis',(0.364399348580517,0.,0.931242779705752));
#50738=DIRECTION('ref_axis',(0.931242779705752,0.,-0.364399348580517));
#50739=DIRECTION('',(0.,1.,0.));
#50740=DIRECTION('center_axis',(-0.624280230025758,0.,0.781200482846104));
#50741=DIRECTION('ref_axis',(0.781200482846104,0.,0.624280230025758));
#50742=DIRECTION('',(0.,1.,0.));
#50743=DIRECTION('center_axis',(-0.988679578606275,0.,-0.150042296859647));
#50744=DIRECTION('ref_axis',(-0.150042296859647,0.,0.988679578606275));
#50745=DIRECTION('',(0.,1.,0.));
#50746=DIRECTION('center_axis',(-0.364399348580519,0.,-0.931242779705751));
#50747=DIRECTION('ref_axis',(-0.931242779705751,0.,0.364399348580519));
#50748=DIRECTION('',(0.,1.,0.));
#50749=DIRECTION('center_axis',(0.624280230025758,0.,-0.781200482846105));
#50750=DIRECTION('ref_axis',(-0.781200482846105,0.,-0.624280230025758));
#50751=DIRECTION('center_axis',(0.988679578606276,0.,0.150042296859641));
#50752=DIRECTION('ref_axis',(0.150042296859641,0.,-0.988679578606276));
#50753=DIRECTION('',(0.,1.,0.));
#50754=DIRECTION('',(0.,1.,0.));
#50755=DIRECTION('center_axis',(0.364399348580517,0.,0.931242779705752));
#50756=DIRECTION('ref_axis',(0.931242779705752,0.,-0.364399348580517));
#50757=DIRECTION('',(0.,1.,0.));
#50758=DIRECTION('center_axis',(-0.624280230025758,0.,0.781200482846104));
#50759=DIRECTION('ref_axis',(0.781200482846104,0.,0.624280230025758));
#50760=DIRECTION('',(0.,1.,0.));
#50761=DIRECTION('center_axis',(-0.988679578606275,0.,-0.150042296859647));
#50762=DIRECTION('ref_axis',(-0.150042296859647,0.,0.988679578606275));
#50763=DIRECTION('',(0.,1.,0.));
#50764=DIRECTION('center_axis',(-0.364399348580519,0.,-0.931242779705751));
#50765=DIRECTION('ref_axis',(-0.931242779705751,0.,0.364399348580519));
#50766=DIRECTION('',(0.,1.,0.));
#50767=DIRECTION('center_axis',(0.624280230025758,0.,-0.781200482846105));
#50768=DIRECTION('ref_axis',(-0.781200482846105,0.,-0.624280230025758));
#50769=DIRECTION('center_axis',(0.988679578606276,0.,0.150042296859641));
#50770=DIRECTION('ref_axis',(0.150042296859641,0.,-0.988679578606276));
#50771=DIRECTION('',(0.,1.,0.));
#50772=DIRECTION('',(0.,1.,0.));
#50773=DIRECTION('center_axis',(0.364399348580517,0.,0.931242779705752));
#50774=DIRECTION('ref_axis',(0.931242779705752,0.,-0.364399348580517));
#50775=DIRECTION('',(0.,1.,0.));
#50776=DIRECTION('center_axis',(-0.624280230025758,0.,0.781200482846104));
#50777=DIRECTION('ref_axis',(0.781200482846104,0.,0.624280230025758));
#50778=DIRECTION('',(0.,1.,0.));
#50779=DIRECTION('center_axis',(-0.988679578606275,0.,-0.150042296859647));
#50780=DIRECTION('ref_axis',(-0.150042296859647,0.,0.988679578606275));
#50781=DIRECTION('',(0.,1.,0.));
#50782=DIRECTION('center_axis',(-0.364399348580519,0.,-0.931242779705751));
#50783=DIRECTION('ref_axis',(-0.931242779705751,0.,0.364399348580519));
#50784=DIRECTION('',(0.,1.,0.));
#50785=DIRECTION('center_axis',(0.624280230025758,0.,-0.781200482846105));
#50786=DIRECTION('ref_axis',(-0.781200482846105,0.,-0.624280230025758));
#50787=DIRECTION('center_axis',(0.988679578606276,0.,0.150042296859641));
#50788=DIRECTION('ref_axis',(0.150042296859641,0.,-0.988679578606276));
#50789=DIRECTION('',(0.,1.,0.));
#50790=DIRECTION('',(0.,1.,0.));
#50791=DIRECTION('center_axis',(0.364399348580517,0.,0.931242779705752));
#50792=DIRECTION('ref_axis',(0.931242779705752,0.,-0.364399348580517));
#50793=DIRECTION('',(0.,1.,0.));
#50794=DIRECTION('center_axis',(-0.624280230025758,0.,0.781200482846104));
#50795=DIRECTION('ref_axis',(0.781200482846104,0.,0.624280230025758));
#50796=DIRECTION('',(0.,1.,0.));
#50797=DIRECTION('center_axis',(-0.988679578606275,0.,-0.150042296859647));
#50798=DIRECTION('ref_axis',(-0.150042296859647,0.,0.988679578606275));
#50799=DIRECTION('',(0.,1.,0.));
#50800=DIRECTION('center_axis',(-0.364399348580519,0.,-0.931242779705751));
#50801=DIRECTION('ref_axis',(-0.931242779705751,0.,0.364399348580519));
#50802=DIRECTION('',(0.,1.,0.));
#50803=DIRECTION('center_axis',(0.624280230025758,0.,-0.781200482846105));
#50804=DIRECTION('ref_axis',(-0.781200482846105,0.,-0.624280230025758));
#50805=DIRECTION('center_axis',(0.988679578606276,0.,0.150042296859641));
#50806=DIRECTION('ref_axis',(0.150042296859641,0.,-0.988679578606276));
#50807=DIRECTION('',(0.,1.,0.));
#50808=DIRECTION('',(0.,1.,0.));
#50809=DIRECTION('center_axis',(0.364399348580517,0.,0.931242779705752));
#50810=DIRECTION('ref_axis',(0.931242779705752,0.,-0.364399348580517));
#50811=DIRECTION('',(0.,1.,0.));
#50812=DIRECTION('center_axis',(-0.624280230025758,0.,0.781200482846104));
#50813=DIRECTION('ref_axis',(0.781200482846104,0.,0.624280230025758));
#50814=DIRECTION('',(0.,1.,0.));
#50815=DIRECTION('center_axis',(-0.988679578606275,0.,-0.150042296859647));
#50816=DIRECTION('ref_axis',(-0.150042296859647,0.,0.988679578606275));
#50817=DIRECTION('',(0.,1.,0.));
#50818=DIRECTION('center_axis',(-0.364399348580519,0.,-0.931242779705751));
#50819=DIRECTION('ref_axis',(-0.931242779705751,0.,0.364399348580519));
#50820=DIRECTION('',(0.,1.,0.));
#50821=DIRECTION('center_axis',(0.624280230025758,0.,-0.781200482846105));
#50822=DIRECTION('ref_axis',(-0.781200482846105,0.,-0.624280230025758));
#50823=DIRECTION('center_axis',(0.988679578606276,0.,0.150042296859641));
#50824=DIRECTION('ref_axis',(0.150042296859641,0.,-0.988679578606276));
#50825=DIRECTION('',(0.,1.,0.));
#50826=DIRECTION('',(0.,1.,0.));
#50827=DIRECTION('center_axis',(0.364399348580517,0.,0.931242779705752));
#50828=DIRECTION('ref_axis',(0.931242779705752,0.,-0.364399348580517));
#50829=DIRECTION('',(0.,1.,0.));
#50830=DIRECTION('center_axis',(-0.624280230025758,0.,0.781200482846104));
#50831=DIRECTION('ref_axis',(0.781200482846104,0.,0.624280230025758));
#50832=DIRECTION('',(0.,1.,0.));
#50833=DIRECTION('center_axis',(-0.988679578606275,0.,-0.150042296859647));
#50834=DIRECTION('ref_axis',(-0.150042296859647,0.,0.988679578606275));
#50835=DIRECTION('',(0.,1.,0.));
#50836=DIRECTION('center_axis',(-0.364399348580519,0.,-0.931242779705751));
#50837=DIRECTION('ref_axis',(-0.931242779705751,0.,0.364399348580519));
#50838=DIRECTION('',(0.,1.,0.));
#50839=DIRECTION('center_axis',(0.624280230025758,0.,-0.781200482846105));
#50840=DIRECTION('ref_axis',(-0.781200482846105,0.,-0.624280230025758));
#50841=DIRECTION('center_axis',(0.988679578606276,0.,0.150042296859641));
#50842=DIRECTION('ref_axis',(0.150042296859641,0.,-0.988679578606276));
#50843=DIRECTION('',(0.,1.,0.));
#50844=DIRECTION('',(0.,1.,0.));
#50845=DIRECTION('center_axis',(0.364399348580517,0.,0.931242779705752));
#50846=DIRECTION('ref_axis',(0.931242779705752,0.,-0.364399348580517));
#50847=DIRECTION('',(0.,1.,0.));
#50848=DIRECTION('center_axis',(-0.624280230025758,0.,0.781200482846104));
#50849=DIRECTION('ref_axis',(0.781200482846104,0.,0.624280230025758));
#50850=DIRECTION('',(0.,1.,0.));
#50851=DIRECTION('center_axis',(-0.988679578606275,0.,-0.150042296859647));
#50852=DIRECTION('ref_axis',(-0.150042296859647,0.,0.988679578606275));
#50853=DIRECTION('',(0.,1.,0.));
#50854=DIRECTION('center_axis',(-0.364399348580519,0.,-0.931242779705751));
#50855=DIRECTION('ref_axis',(-0.931242779705751,0.,0.364399348580519));
#50856=DIRECTION('',(0.,1.,0.));
#50857=DIRECTION('center_axis',(0.624280230025758,0.,-0.781200482846105));
#50858=DIRECTION('ref_axis',(-0.781200482846105,0.,-0.624280230025758));
#50859=DIRECTION('center_axis',(0.988679578606276,0.,0.150042296859641));
#50860=DIRECTION('ref_axis',(0.150042296859641,0.,-0.988679578606276));
#50861=DIRECTION('',(0.,1.,0.));
#50862=DIRECTION('',(0.,1.,0.));
#50863=DIRECTION('center_axis',(0.364399348580517,0.,0.931242779705752));
#50864=DIRECTION('ref_axis',(0.931242779705752,0.,-0.364399348580517));
#50865=DIRECTION('',(0.,1.,0.));
#50866=DIRECTION('center_axis',(-0.624280230025758,0.,0.781200482846104));
#50867=DIRECTION('ref_axis',(0.781200482846104,0.,0.624280230025758));
#50868=DIRECTION('',(0.,1.,0.));
#50869=DIRECTION('center_axis',(-0.988679578606275,0.,-0.150042296859647));
#50870=DIRECTION('ref_axis',(-0.150042296859647,0.,0.988679578606275));
#50871=DIRECTION('',(0.,1.,0.));
#50872=DIRECTION('center_axis',(-0.364399348580519,0.,-0.931242779705751));
#50873=DIRECTION('ref_axis',(-0.931242779705751,0.,0.364399348580519));
#50874=DIRECTION('',(0.,1.,0.));
#50875=DIRECTION('center_axis',(0.624280230025758,0.,-0.781200482846105));
#50876=DIRECTION('ref_axis',(-0.781200482846105,0.,-0.624280230025758));
#50877=DIRECTION('center_axis',(0.988679578606276,0.,0.150042296859641));
#50878=DIRECTION('ref_axis',(0.150042296859641,0.,-0.988679578606276));
#50879=DIRECTION('',(0.,1.,0.));
#50880=DIRECTION('',(0.,1.,0.));
#50881=DIRECTION('center_axis',(0.364399348580517,0.,0.931242779705752));
#50882=DIRECTION('ref_axis',(0.931242779705752,0.,-0.364399348580517));
#50883=DIRECTION('',(0.,1.,0.));
#50884=DIRECTION('center_axis',(-0.624280230025758,0.,0.781200482846104));
#50885=DIRECTION('ref_axis',(0.781200482846104,0.,0.624280230025758));
#50886=DIRECTION('',(0.,1.,0.));
#50887=DIRECTION('center_axis',(-0.988679578606275,0.,-0.150042296859647));
#50888=DIRECTION('ref_axis',(-0.150042296859647,0.,0.988679578606275));
#50889=DIRECTION('',(0.,1.,0.));
#50890=DIRECTION('center_axis',(-0.364399348580519,0.,-0.931242779705751));
#50891=DIRECTION('ref_axis',(-0.931242779705751,0.,0.364399348580519));
#50892=DIRECTION('',(0.,1.,0.));
#50893=DIRECTION('center_axis',(0.624280230025758,0.,-0.781200482846105));
#50894=DIRECTION('ref_axis',(-0.781200482846105,0.,-0.624280230025758));
#50895=DIRECTION('center_axis',(0.988679578606276,0.,0.150042296859641));
#50896=DIRECTION('ref_axis',(0.150042296859641,0.,-0.988679578606276));
#50897=DIRECTION('',(0.,1.,0.));
#50898=DIRECTION('',(0.,1.,0.));
#50899=DIRECTION('center_axis',(0.364399348580517,0.,0.931242779705752));
#50900=DIRECTION('ref_axis',(0.931242779705752,0.,-0.364399348580517));
#50901=DIRECTION('',(0.,1.,0.));
#50902=DIRECTION('center_axis',(-0.624280230025758,0.,0.781200482846104));
#50903=DIRECTION('ref_axis',(0.781200482846104,0.,0.624280230025758));
#50904=DIRECTION('',(0.,1.,0.));
#50905=DIRECTION('center_axis',(-0.988679578606275,0.,-0.150042296859647));
#50906=DIRECTION('ref_axis',(-0.150042296859647,0.,0.988679578606275));
#50907=DIRECTION('',(0.,1.,0.));
#50908=DIRECTION('center_axis',(-0.364399348580519,0.,-0.931242779705751));
#50909=DIRECTION('ref_axis',(-0.931242779705751,0.,0.364399348580519));
#50910=DIRECTION('',(0.,1.,0.));
#50911=DIRECTION('center_axis',(0.624280230025758,0.,-0.781200482846105));
#50912=DIRECTION('ref_axis',(-0.781200482846105,0.,-0.624280230025758));
#50913=DIRECTION('center_axis',(0.988679578606276,0.,0.150042296859641));
#50914=DIRECTION('ref_axis',(0.150042296859641,0.,-0.988679578606276));
#50915=DIRECTION('',(0.,1.,0.));
#50916=DIRECTION('',(0.,1.,0.));
#50917=DIRECTION('center_axis',(0.364399348580517,0.,0.931242779705752));
#50918=DIRECTION('ref_axis',(0.931242779705752,0.,-0.364399348580517));
#50919=DIRECTION('',(0.,1.,0.));
#50920=DIRECTION('center_axis',(-0.624280230025758,0.,0.781200482846104));
#50921=DIRECTION('ref_axis',(0.781200482846104,0.,0.624280230025758));
#50922=DIRECTION('',(0.,1.,0.));
#50923=DIRECTION('center_axis',(-0.988679578606275,0.,-0.150042296859647));
#50924=DIRECTION('ref_axis',(-0.150042296859647,0.,0.988679578606275));
#50925=DIRECTION('',(0.,1.,0.));
#50926=DIRECTION('center_axis',(-0.364399348580519,0.,-0.931242779705751));
#50927=DIRECTION('ref_axis',(-0.931242779705751,0.,0.364399348580519));
#50928=DIRECTION('',(0.,1.,0.));
#50929=DIRECTION('center_axis',(0.624280230025758,0.,-0.781200482846105));
#50930=DIRECTION('ref_axis',(-0.781200482846105,0.,-0.624280230025758));
#50931=DIRECTION('center_axis',(0.988679578606276,0.,0.150042296859641));
#50932=DIRECTION('ref_axis',(0.150042296859641,0.,-0.988679578606276));
#50933=DIRECTION('',(0.,1.,0.));
#50934=DIRECTION('',(0.,1.,0.));
#50935=DIRECTION('center_axis',(0.364399348580517,0.,0.931242779705752));
#50936=DIRECTION('ref_axis',(0.931242779705752,0.,-0.364399348580517));
#50937=DIRECTION('',(0.,1.,0.));
#50938=DIRECTION('center_axis',(-0.624280230025758,0.,0.781200482846104));
#50939=DIRECTION('ref_axis',(0.781200482846104,0.,0.624280230025758));
#50940=DIRECTION('',(0.,1.,0.));
#50941=DIRECTION('center_axis',(-0.988679578606275,0.,-0.150042296859647));
#50942=DIRECTION('ref_axis',(-0.150042296859647,0.,0.988679578606275));
#50943=DIRECTION('',(0.,1.,0.));
#50944=DIRECTION('center_axis',(-0.364399348580519,0.,-0.931242779705751));
#50945=DIRECTION('ref_axis',(-0.931242779705751,0.,0.364399348580519));
#50946=DIRECTION('',(0.,1.,0.));
#50947=DIRECTION('center_axis',(0.624280230025758,0.,-0.781200482846105));
#50948=DIRECTION('ref_axis',(-0.781200482846105,0.,-0.624280230025758));
#50949=DIRECTION('center_axis',(0.988679578606276,0.,0.150042296859641));
#50950=DIRECTION('ref_axis',(0.150042296859641,0.,-0.988679578606276));
#50951=DIRECTION('',(0.,1.,0.));
#50952=DIRECTION('',(0.,1.,0.));
#50953=DIRECTION('center_axis',(0.364399348580517,0.,0.931242779705752));
#50954=DIRECTION('ref_axis',(0.931242779705752,0.,-0.364399348580517));
#50955=DIRECTION('',(0.,1.,0.));
#50956=DIRECTION('center_axis',(-0.624280230025758,0.,0.781200482846104));
#50957=DIRECTION('ref_axis',(0.781200482846104,0.,0.624280230025758));
#50958=DIRECTION('',(0.,1.,0.));
#50959=DIRECTION('center_axis',(-0.988679578606275,0.,-0.150042296859647));
#50960=DIRECTION('ref_axis',(-0.150042296859647,0.,0.988679578606275));
#50961=DIRECTION('',(0.,1.,0.));
#50962=DIRECTION('center_axis',(-0.364399348580519,0.,-0.931242779705751));
#50963=DIRECTION('ref_axis',(-0.931242779705751,0.,0.364399348580519));
#50964=DIRECTION('',(0.,1.,0.));
#50965=DIRECTION('center_axis',(0.624280230025758,0.,-0.781200482846105));
#50966=DIRECTION('ref_axis',(-0.781200482846105,0.,-0.624280230025758));
#50967=DIRECTION('center_axis',(0.988679578606276,0.,0.150042296859641));
#50968=DIRECTION('ref_axis',(0.150042296859641,0.,-0.988679578606276));
#50969=DIRECTION('',(0.,1.,0.));
#50970=DIRECTION('',(0.,1.,0.));
#50971=DIRECTION('center_axis',(0.364399348580517,0.,0.931242779705752));
#50972=DIRECTION('ref_axis',(0.931242779705752,0.,-0.364399348580517));
#50973=DIRECTION('',(0.,1.,0.));
#50974=DIRECTION('center_axis',(-0.624280230025758,0.,0.781200482846104));
#50975=DIRECTION('ref_axis',(0.781200482846104,0.,0.624280230025758));
#50976=DIRECTION('',(0.,1.,0.));
#50977=DIRECTION('center_axis',(-0.988679578606275,0.,-0.150042296859647));
#50978=DIRECTION('ref_axis',(-0.150042296859647,0.,0.988679578606275));
#50979=DIRECTION('',(0.,1.,0.));
#50980=DIRECTION('center_axis',(-0.364399348580519,0.,-0.931242779705751));
#50981=DIRECTION('ref_axis',(-0.931242779705751,0.,0.364399348580519));
#50982=DIRECTION('',(0.,1.,0.));
#50983=DIRECTION('center_axis',(0.624280230025758,0.,-0.781200482846105));
#50984=DIRECTION('ref_axis',(-0.781200482846105,0.,-0.624280230025758));
#50985=DIRECTION('center_axis',(0.988679578606276,0.,0.150042296859641));
#50986=DIRECTION('ref_axis',(0.150042296859641,0.,-0.988679578606276));
#50987=DIRECTION('',(0.,1.,0.));
#50988=DIRECTION('',(0.,1.,0.));
#50989=DIRECTION('center_axis',(0.364399348580517,0.,0.931242779705752));
#50990=DIRECTION('ref_axis',(0.931242779705752,0.,-0.364399348580517));
#50991=DIRECTION('',(0.,1.,0.));
#50992=DIRECTION('center_axis',(-0.624280230025758,0.,0.781200482846104));
#50993=DIRECTION('ref_axis',(0.781200482846104,0.,0.624280230025758));
#50994=DIRECTION('',(0.,1.,0.));
#50995=DIRECTION('center_axis',(-0.988679578606275,0.,-0.150042296859647));
#50996=DIRECTION('ref_axis',(-0.150042296859647,0.,0.988679578606275));
#50997=DIRECTION('',(0.,1.,0.));
#50998=DIRECTION('center_axis',(-0.364399348580519,0.,-0.931242779705751));
#50999=DIRECTION('ref_axis',(-0.931242779705751,0.,0.364399348580519));
#51000=DIRECTION('',(0.,1.,0.));
#51001=DIRECTION('center_axis',(0.624280230025758,0.,-0.781200482846105));
#51002=DIRECTION('ref_axis',(-0.781200482846105,0.,-0.624280230025758));
#51003=DIRECTION('center_axis',(0.988679578606276,0.,0.150042296859641));
#51004=DIRECTION('ref_axis',(0.150042296859641,0.,-0.988679578606276));
#51005=DIRECTION('',(0.,1.,0.));
#51006=DIRECTION('',(0.,1.,0.));
#51007=DIRECTION('center_axis',(0.364399348580517,0.,0.931242779705752));
#51008=DIRECTION('ref_axis',(0.931242779705752,0.,-0.364399348580517));
#51009=DIRECTION('',(0.,1.,0.));
#51010=DIRECTION('center_axis',(-0.624280230025758,0.,0.781200482846104));
#51011=DIRECTION('ref_axis',(0.781200482846104,0.,0.624280230025758));
#51012=DIRECTION('',(0.,1.,0.));
#51013=DIRECTION('center_axis',(-0.988679578606275,0.,-0.150042296859647));
#51014=DIRECTION('ref_axis',(-0.150042296859647,0.,0.988679578606275));
#51015=DIRECTION('',(0.,1.,0.));
#51016=DIRECTION('center_axis',(-0.364399348580519,0.,-0.931242779705751));
#51017=DIRECTION('ref_axis',(-0.931242779705751,0.,0.364399348580519));
#51018=DIRECTION('',(0.,1.,0.));
#51019=DIRECTION('center_axis',(0.624280230025758,0.,-0.781200482846105));
#51020=DIRECTION('ref_axis',(-0.781200482846105,0.,-0.624280230025758));
#51021=DIRECTION('center_axis',(0.988679578606276,0.,0.150042296859641));
#51022=DIRECTION('ref_axis',(0.150042296859641,0.,-0.988679578606276));
#51023=DIRECTION('',(0.,1.,0.));
#51024=DIRECTION('',(0.,1.,0.));
#51025=DIRECTION('center_axis',(0.364399348580517,0.,0.931242779705752));
#51026=DIRECTION('ref_axis',(0.931242779705752,0.,-0.364399348580517));
#51027=DIRECTION('',(0.,1.,0.));
#51028=DIRECTION('center_axis',(-0.624280230025758,0.,0.781200482846104));
#51029=DIRECTION('ref_axis',(0.781200482846104,0.,0.624280230025758));
#51030=DIRECTION('',(0.,1.,0.));
#51031=DIRECTION('center_axis',(-0.988679578606275,0.,-0.150042296859647));
#51032=DIRECTION('ref_axis',(-0.150042296859647,0.,0.988679578606275));
#51033=DIRECTION('',(0.,1.,0.));
#51034=DIRECTION('center_axis',(-0.364399348580519,0.,-0.931242779705751));
#51035=DIRECTION('ref_axis',(-0.931242779705751,0.,0.364399348580519));
#51036=DIRECTION('',(0.,1.,0.));
#51037=DIRECTION('center_axis',(0.624280230025758,0.,-0.781200482846105));
#51038=DIRECTION('ref_axis',(-0.781200482846105,0.,-0.624280230025758));
#51039=DIRECTION('center_axis',(0.988679578606276,0.,0.150042296859641));
#51040=DIRECTION('ref_axis',(0.150042296859641,0.,-0.988679578606276));
#51041=DIRECTION('',(0.,1.,0.));
#51042=DIRECTION('',(0.,1.,0.));
#51043=DIRECTION('center_axis',(0.364399348580517,0.,0.931242779705752));
#51044=DIRECTION('ref_axis',(0.931242779705752,0.,-0.364399348580517));
#51045=DIRECTION('',(0.,1.,0.));
#51046=DIRECTION('center_axis',(-0.624280230025758,0.,0.781200482846104));
#51047=DIRECTION('ref_axis',(0.781200482846104,0.,0.624280230025758));
#51048=DIRECTION('',(0.,1.,0.));
#51049=DIRECTION('center_axis',(-0.988679578606275,0.,-0.150042296859647));
#51050=DIRECTION('ref_axis',(-0.150042296859647,0.,0.988679578606275));
#51051=DIRECTION('',(0.,1.,0.));
#51052=DIRECTION('center_axis',(-0.364399348580519,0.,-0.931242779705751));
#51053=DIRECTION('ref_axis',(-0.931242779705751,0.,0.364399348580519));
#51054=DIRECTION('',(0.,1.,0.));
#51055=DIRECTION('center_axis',(0.624280230025758,0.,-0.781200482846105));
#51056=DIRECTION('ref_axis',(-0.781200482846105,0.,-0.624280230025758));
#51057=DIRECTION('center_axis',(0.988679578606276,0.,0.150042296859641));
#51058=DIRECTION('ref_axis',(0.150042296859641,0.,-0.988679578606276));
#51059=DIRECTION('',(0.,1.,0.));
#51060=DIRECTION('',(0.,1.,0.));
#51061=DIRECTION('center_axis',(0.364399348580517,0.,0.931242779705752));
#51062=DIRECTION('ref_axis',(0.931242779705752,0.,-0.364399348580517));
#51063=DIRECTION('',(0.,1.,0.));
#51064=DIRECTION('center_axis',(-0.624280230025758,0.,0.781200482846104));
#51065=DIRECTION('ref_axis',(0.781200482846104,0.,0.624280230025758));
#51066=DIRECTION('',(0.,1.,0.));
#51067=DIRECTION('center_axis',(-0.988679578606275,0.,-0.150042296859647));
#51068=DIRECTION('ref_axis',(-0.150042296859647,0.,0.988679578606275));
#51069=DIRECTION('',(0.,1.,0.));
#51070=DIRECTION('center_axis',(-0.364399348580519,0.,-0.931242779705751));
#51071=DIRECTION('ref_axis',(-0.931242779705751,0.,0.364399348580519));
#51072=DIRECTION('',(0.,1.,0.));
#51073=DIRECTION('center_axis',(0.624280230025758,0.,-0.781200482846105));
#51074=DIRECTION('ref_axis',(-0.781200482846105,0.,-0.624280230025758));
#51075=DIRECTION('center_axis',(0.988679578606276,0.,0.150042296859641));
#51076=DIRECTION('ref_axis',(0.150042296859641,0.,-0.988679578606276));
#51077=DIRECTION('',(0.,1.,0.));
#51078=DIRECTION('',(0.,1.,0.));
#51079=DIRECTION('center_axis',(0.364399348580517,0.,0.931242779705752));
#51080=DIRECTION('ref_axis',(0.931242779705752,0.,-0.364399348580517));
#51081=DIRECTION('',(0.,1.,0.));
#51082=DIRECTION('center_axis',(-0.624280230025758,0.,0.781200482846104));
#51083=DIRECTION('ref_axis',(0.781200482846104,0.,0.624280230025758));
#51084=DIRECTION('',(0.,1.,0.));
#51085=DIRECTION('center_axis',(-0.988679578606275,0.,-0.150042296859647));
#51086=DIRECTION('ref_axis',(-0.150042296859647,0.,0.988679578606275));
#51087=DIRECTION('',(0.,1.,0.));
#51088=DIRECTION('center_axis',(-0.364399348580519,0.,-0.931242779705751));
#51089=DIRECTION('ref_axis',(-0.931242779705751,0.,0.364399348580519));
#51090=DIRECTION('',(0.,1.,0.));
#51091=DIRECTION('center_axis',(0.624280230025758,0.,-0.781200482846105));
#51092=DIRECTION('ref_axis',(-0.781200482846105,0.,-0.624280230025758));
#51093=DIRECTION('center_axis',(0.988679578606276,0.,0.150042296859641));
#51094=DIRECTION('ref_axis',(0.150042296859641,0.,-0.988679578606276));
#51095=DIRECTION('',(0.,1.,0.));
#51096=DIRECTION('',(0.,1.,0.));
#51097=DIRECTION('center_axis',(0.364399348580517,0.,0.931242779705752));
#51098=DIRECTION('ref_axis',(0.931242779705752,0.,-0.364399348580517));
#51099=DIRECTION('',(0.,1.,0.));
#51100=DIRECTION('center_axis',(-0.624280230025758,0.,0.781200482846104));
#51101=DIRECTION('ref_axis',(0.781200482846104,0.,0.624280230025758));
#51102=DIRECTION('',(0.,1.,0.));
#51103=DIRECTION('center_axis',(-0.988679578606275,0.,-0.150042296859647));
#51104=DIRECTION('ref_axis',(-0.150042296859647,0.,0.988679578606275));
#51105=DIRECTION('',(0.,1.,0.));
#51106=DIRECTION('center_axis',(-0.364399348580519,0.,-0.931242779705751));
#51107=DIRECTION('ref_axis',(-0.931242779705751,0.,0.364399348580519));
#51108=DIRECTION('',(0.,1.,0.));
#51109=DIRECTION('center_axis',(0.624280230025758,0.,-0.781200482846105));
#51110=DIRECTION('ref_axis',(-0.781200482846105,0.,-0.624280230025758));
#51111=DIRECTION('center_axis',(0.988679578606276,0.,0.150042296859641));
#51112=DIRECTION('ref_axis',(0.150042296859641,0.,-0.988679578606276));
#51113=DIRECTION('',(0.,1.,0.));
#51114=DIRECTION('',(0.,1.,0.));
#51115=DIRECTION('center_axis',(0.364399348580517,0.,0.931242779705752));
#51116=DIRECTION('ref_axis',(0.931242779705752,0.,-0.364399348580517));
#51117=DIRECTION('',(0.,1.,0.));
#51118=DIRECTION('center_axis',(-0.624280230025758,0.,0.781200482846104));
#51119=DIRECTION('ref_axis',(0.781200482846104,0.,0.624280230025758));
#51120=DIRECTION('',(0.,1.,0.));
#51121=DIRECTION('center_axis',(-0.988679578606275,0.,-0.150042296859647));
#51122=DIRECTION('ref_axis',(-0.150042296859647,0.,0.988679578606275));
#51123=DIRECTION('',(0.,1.,0.));
#51124=DIRECTION('center_axis',(-0.364399348580519,0.,-0.931242779705751));
#51125=DIRECTION('ref_axis',(-0.931242779705751,0.,0.364399348580519));
#51126=DIRECTION('',(0.,1.,0.));
#51127=DIRECTION('center_axis',(0.624280230025758,0.,-0.781200482846105));
#51128=DIRECTION('ref_axis',(-0.781200482846105,0.,-0.624280230025758));
#51129=DIRECTION('center_axis',(0.988679578606276,0.,0.150042296859641));
#51130=DIRECTION('ref_axis',(0.150042296859641,0.,-0.988679578606276));
#51131=DIRECTION('',(0.,1.,0.));
#51132=DIRECTION('',(0.,1.,0.));
#51133=DIRECTION('center_axis',(0.364399348580517,0.,0.931242779705752));
#51134=DIRECTION('ref_axis',(0.931242779705752,0.,-0.364399348580517));
#51135=DIRECTION('',(0.,1.,0.));
#51136=DIRECTION('center_axis',(-0.624280230025758,0.,0.781200482846104));
#51137=DIRECTION('ref_axis',(0.781200482846104,0.,0.624280230025758));
#51138=DIRECTION('',(0.,1.,0.));
#51139=DIRECTION('center_axis',(-0.988679578606275,0.,-0.150042296859647));
#51140=DIRECTION('ref_axis',(-0.150042296859647,0.,0.988679578606275));
#51141=DIRECTION('',(0.,1.,0.));
#51142=DIRECTION('center_axis',(-0.364399348580519,0.,-0.931242779705751));
#51143=DIRECTION('ref_axis',(-0.931242779705751,0.,0.364399348580519));
#51144=DIRECTION('',(0.,1.,0.));
#51145=DIRECTION('center_axis',(0.624280230025758,0.,-0.781200482846105));
#51146=DIRECTION('ref_axis',(-0.781200482846105,0.,-0.624280230025758));
#51147=DIRECTION('center_axis',(0.988679578606276,0.,0.150042296859641));
#51148=DIRECTION('ref_axis',(0.150042296859641,0.,-0.988679578606276));
#51149=DIRECTION('',(0.,1.,0.));
#51150=DIRECTION('',(0.,1.,0.));
#51151=DIRECTION('center_axis',(0.364399348580517,0.,0.931242779705752));
#51152=DIRECTION('ref_axis',(0.931242779705752,0.,-0.364399348580517));
#51153=DIRECTION('',(0.,1.,0.));
#51154=DIRECTION('center_axis',(-0.624280230025758,0.,0.781200482846104));
#51155=DIRECTION('ref_axis',(0.781200482846104,0.,0.624280230025758));
#51156=DIRECTION('',(0.,1.,0.));
#51157=DIRECTION('center_axis',(-0.988679578606275,0.,-0.150042296859647));
#51158=DIRECTION('ref_axis',(-0.150042296859647,0.,0.988679578606275));
#51159=DIRECTION('',(0.,1.,0.));
#51160=DIRECTION('center_axis',(-0.364399348580519,0.,-0.931242779705751));
#51161=DIRECTION('ref_axis',(-0.931242779705751,0.,0.364399348580519));
#51162=DIRECTION('',(0.,1.,0.));
#51163=DIRECTION('center_axis',(0.624280230025758,0.,-0.781200482846105));
#51164=DIRECTION('ref_axis',(-0.781200482846105,0.,-0.624280230025758));
#51165=DIRECTION('center_axis',(0.988679578606276,0.,0.150042296859641));
#51166=DIRECTION('ref_axis',(0.150042296859641,0.,-0.988679578606276));
#51167=DIRECTION('',(0.,1.,0.));
#51168=DIRECTION('',(0.,1.,0.));
#51169=DIRECTION('center_axis',(0.364399348580517,0.,0.931242779705752));
#51170=DIRECTION('ref_axis',(0.931242779705752,0.,-0.364399348580517));
#51171=DIRECTION('',(0.,1.,0.));
#51172=DIRECTION('center_axis',(-0.624280230025758,0.,0.781200482846104));
#51173=DIRECTION('ref_axis',(0.781200482846104,0.,0.624280230025758));
#51174=DIRECTION('',(0.,1.,0.));
#51175=DIRECTION('center_axis',(-0.988679578606275,0.,-0.150042296859647));
#51176=DIRECTION('ref_axis',(-0.150042296859647,0.,0.988679578606275));
#51177=DIRECTION('',(0.,1.,0.));
#51178=DIRECTION('center_axis',(-0.364399348580519,0.,-0.931242779705751));
#51179=DIRECTION('ref_axis',(-0.931242779705751,0.,0.364399348580519));
#51180=DIRECTION('',(0.,1.,0.));
#51181=DIRECTION('center_axis',(0.624280230025758,0.,-0.781200482846105));
#51182=DIRECTION('ref_axis',(-0.781200482846105,0.,-0.624280230025758));
#51183=DIRECTION('center_axis',(0.988679578606276,0.,0.150042296859641));
#51184=DIRECTION('ref_axis',(0.150042296859641,0.,-0.988679578606276));
#51185=DIRECTION('',(0.,1.,0.));
#51186=DIRECTION('',(0.,1.,0.));
#51187=DIRECTION('center_axis',(0.364399348580517,0.,0.931242779705752));
#51188=DIRECTION('ref_axis',(0.931242779705752,0.,-0.364399348580517));
#51189=DIRECTION('',(0.,1.,0.));
#51190=DIRECTION('center_axis',(-0.624280230025758,0.,0.781200482846104));
#51191=DIRECTION('ref_axis',(0.781200482846104,0.,0.624280230025758));
#51192=DIRECTION('',(0.,1.,0.));
#51193=DIRECTION('center_axis',(-0.988679578606275,0.,-0.150042296859647));
#51194=DIRECTION('ref_axis',(-0.150042296859647,0.,0.988679578606275));
#51195=DIRECTION('',(0.,1.,0.));
#51196=DIRECTION('center_axis',(-0.364399348580519,0.,-0.931242779705751));
#51197=DIRECTION('ref_axis',(-0.931242779705751,0.,0.364399348580519));
#51198=DIRECTION('',(0.,1.,0.));
#51199=DIRECTION('center_axis',(0.624280230025758,0.,-0.781200482846105));
#51200=DIRECTION('ref_axis',(-0.781200482846105,0.,-0.624280230025758));
#51201=DIRECTION('center_axis',(0.988679578606276,0.,0.150042296859641));
#51202=DIRECTION('ref_axis',(0.150042296859641,0.,-0.988679578606276));
#51203=DIRECTION('',(0.,1.,0.));
#51204=DIRECTION('',(0.,1.,0.));
#51205=DIRECTION('center_axis',(0.364399348580517,0.,0.931242779705752));
#51206=DIRECTION('ref_axis',(0.931242779705752,0.,-0.364399348580517));
#51207=DIRECTION('',(0.,1.,0.));
#51208=DIRECTION('center_axis',(-0.624280230025758,0.,0.781200482846104));
#51209=DIRECTION('ref_axis',(0.781200482846104,0.,0.624280230025758));
#51210=DIRECTION('',(0.,1.,0.));
#51211=DIRECTION('center_axis',(-0.988679578606275,0.,-0.150042296859647));
#51212=DIRECTION('ref_axis',(-0.150042296859647,0.,0.988679578606275));
#51213=DIRECTION('',(0.,1.,0.));
#51214=DIRECTION('center_axis',(-0.364399348580519,0.,-0.931242779705751));
#51215=DIRECTION('ref_axis',(-0.931242779705751,0.,0.364399348580519));
#51216=DIRECTION('',(0.,1.,0.));
#51217=DIRECTION('center_axis',(0.624280230025758,0.,-0.781200482846105));
#51218=DIRECTION('ref_axis',(-0.781200482846105,0.,-0.624280230025758));
#51219=DIRECTION('center_axis',(0.988679578606276,0.,0.150042296859641));
#51220=DIRECTION('ref_axis',(0.150042296859641,0.,-0.988679578606276));
#51221=DIRECTION('',(0.,1.,0.));
#51222=DIRECTION('',(0.,1.,0.));
#51223=DIRECTION('center_axis',(0.364399348580517,0.,0.931242779705752));
#51224=DIRECTION('ref_axis',(0.931242779705752,0.,-0.364399348580517));
#51225=DIRECTION('',(0.,1.,0.));
#51226=DIRECTION('center_axis',(-0.624280230025758,0.,0.781200482846104));
#51227=DIRECTION('ref_axis',(0.781200482846104,0.,0.624280230025758));
#51228=DIRECTION('',(0.,1.,0.));
#51229=DIRECTION('center_axis',(-0.988679578606275,0.,-0.150042296859647));
#51230=DIRECTION('ref_axis',(-0.150042296859647,0.,0.988679578606275));
#51231=DIRECTION('',(0.,1.,0.));
#51232=DIRECTION('center_axis',(-0.364399348580519,0.,-0.931242779705751));
#51233=DIRECTION('ref_axis',(-0.931242779705751,0.,0.364399348580519));
#51234=DIRECTION('',(0.,1.,0.));
#51235=DIRECTION('center_axis',(0.624280230025758,0.,-0.781200482846105));
#51236=DIRECTION('ref_axis',(-0.781200482846105,0.,-0.624280230025758));
#51237=DIRECTION('center_axis',(0.988679578606276,0.,0.150042296859641));
#51238=DIRECTION('ref_axis',(0.150042296859641,0.,-0.988679578606276));
#51239=DIRECTION('',(0.,1.,0.));
#51240=DIRECTION('',(0.,1.,0.));
#51241=DIRECTION('center_axis',(0.364399348580517,0.,0.931242779705752));
#51242=DIRECTION('ref_axis',(0.931242779705752,0.,-0.364399348580517));
#51243=DIRECTION('',(0.,1.,0.));
#51244=DIRECTION('center_axis',(-0.624280230025758,0.,0.781200482846104));
#51245=DIRECTION('ref_axis',(0.781200482846104,0.,0.624280230025758));
#51246=DIRECTION('',(0.,1.,0.));
#51247=DIRECTION('center_axis',(-0.988679578606275,0.,-0.150042296859647));
#51248=DIRECTION('ref_axis',(-0.150042296859647,0.,0.988679578606275));
#51249=DIRECTION('',(0.,1.,0.));
#51250=DIRECTION('center_axis',(-0.364399348580519,0.,-0.931242779705751));
#51251=DIRECTION('ref_axis',(-0.931242779705751,0.,0.364399348580519));
#51252=DIRECTION('',(0.,1.,0.));
#51253=DIRECTION('center_axis',(0.624280230025758,0.,-0.781200482846105));
#51254=DIRECTION('ref_axis',(-0.781200482846105,0.,-0.624280230025758));
#51255=DIRECTION('center_axis',(0.988679578606276,0.,0.150042296859641));
#51256=DIRECTION('ref_axis',(0.150042296859641,0.,-0.988679578606276));
#51257=DIRECTION('',(0.,1.,0.));
#51258=DIRECTION('',(0.,1.,0.));
#51259=DIRECTION('center_axis',(0.364399348580517,0.,0.931242779705752));
#51260=DIRECTION('ref_axis',(0.931242779705752,0.,-0.364399348580517));
#51261=DIRECTION('',(0.,1.,0.));
#51262=DIRECTION('center_axis',(-0.624280230025758,0.,0.781200482846104));
#51263=DIRECTION('ref_axis',(0.781200482846104,0.,0.624280230025758));
#51264=DIRECTION('',(0.,1.,0.));
#51265=DIRECTION('center_axis',(-0.988679578606275,0.,-0.150042296859647));
#51266=DIRECTION('ref_axis',(-0.150042296859647,0.,0.988679578606275));
#51267=DIRECTION('',(0.,1.,0.));
#51268=DIRECTION('center_axis',(-0.364399348580519,0.,-0.931242779705751));
#51269=DIRECTION('ref_axis',(-0.931242779705751,0.,0.364399348580519));
#51270=DIRECTION('',(0.,1.,0.));
#51271=DIRECTION('center_axis',(0.624280230025758,0.,-0.781200482846105));
#51272=DIRECTION('ref_axis',(-0.781200482846105,0.,-0.624280230025758));
#51273=DIRECTION('center_axis',(0.988679578606276,0.,0.150042296859641));
#51274=DIRECTION('ref_axis',(0.150042296859641,0.,-0.988679578606276));
#51275=DIRECTION('',(0.,1.,0.));
#51276=DIRECTION('',(0.,1.,0.));
#51277=DIRECTION('center_axis',(0.364399348580517,0.,0.931242779705752));
#51278=DIRECTION('ref_axis',(0.931242779705752,0.,-0.364399348580517));
#51279=DIRECTION('',(0.,1.,0.));
#51280=DIRECTION('center_axis',(-0.624280230025758,0.,0.781200482846104));
#51281=DIRECTION('ref_axis',(0.781200482846104,0.,0.624280230025758));
#51282=DIRECTION('',(0.,1.,0.));
#51283=DIRECTION('center_axis',(-0.988679578606275,0.,-0.150042296859647));
#51284=DIRECTION('ref_axis',(-0.150042296859647,0.,0.988679578606275));
#51285=DIRECTION('',(0.,1.,0.));
#51286=DIRECTION('center_axis',(-0.364399348580519,0.,-0.931242779705751));
#51287=DIRECTION('ref_axis',(-0.931242779705751,0.,0.364399348580519));
#51288=DIRECTION('',(0.,1.,0.));
#51289=DIRECTION('center_axis',(0.624280230025758,0.,-0.781200482846105));
#51290=DIRECTION('ref_axis',(-0.781200482846105,0.,-0.624280230025758));
#51291=DIRECTION('center_axis',(0.988679578606276,0.,0.150042296859641));
#51292=DIRECTION('ref_axis',(0.150042296859641,0.,-0.988679578606276));
#51293=DIRECTION('',(0.,1.,0.));
#51294=DIRECTION('',(0.,1.,0.));
#51295=DIRECTION('center_axis',(0.364399348580517,0.,0.931242779705752));
#51296=DIRECTION('ref_axis',(0.931242779705752,0.,-0.364399348580517));
#51297=DIRECTION('',(0.,1.,0.));
#51298=DIRECTION('center_axis',(-0.624280230025758,0.,0.781200482846104));
#51299=DIRECTION('ref_axis',(0.781200482846104,0.,0.624280230025758));
#51300=DIRECTION('',(0.,1.,0.));
#51301=DIRECTION('center_axis',(-0.988679578606275,0.,-0.150042296859647));
#51302=DIRECTION('ref_axis',(-0.150042296859647,0.,0.988679578606275));
#51303=DIRECTION('',(0.,1.,0.));
#51304=DIRECTION('center_axis',(-0.364399348580519,0.,-0.931242779705751));
#51305=DIRECTION('ref_axis',(-0.931242779705751,0.,0.364399348580519));
#51306=DIRECTION('',(0.,1.,0.));
#51307=DIRECTION('center_axis',(0.624280230025758,0.,-0.781200482846105));
#51308=DIRECTION('ref_axis',(-0.781200482846105,0.,-0.624280230025758));
#51309=DIRECTION('center_axis',(0.988679578606276,0.,0.150042296859641));
#51310=DIRECTION('ref_axis',(0.150042296859641,0.,-0.988679578606276));
#51311=DIRECTION('',(0.,1.,0.));
#51312=DIRECTION('',(0.,1.,0.));
#51313=DIRECTION('center_axis',(0.364399348580517,0.,0.931242779705752));
#51314=DIRECTION('ref_axis',(0.931242779705752,0.,-0.364399348580517));
#51315=DIRECTION('',(0.,1.,0.));
#51316=DIRECTION('center_axis',(-0.624280230025758,0.,0.781200482846104));
#51317=DIRECTION('ref_axis',(0.781200482846104,0.,0.624280230025758));
#51318=DIRECTION('',(0.,1.,0.));
#51319=DIRECTION('center_axis',(-0.988679578606275,0.,-0.150042296859647));
#51320=DIRECTION('ref_axis',(-0.150042296859647,0.,0.988679578606275));
#51321=DIRECTION('',(0.,1.,0.));
#51322=DIRECTION('center_axis',(-0.364399348580519,0.,-0.931242779705751));
#51323=DIRECTION('ref_axis',(-0.931242779705751,0.,0.364399348580519));
#51324=DIRECTION('',(0.,1.,0.));
#51325=DIRECTION('center_axis',(0.624280230025758,0.,-0.781200482846105));
#51326=DIRECTION('ref_axis',(-0.781200482846105,0.,-0.624280230025758));
#51327=DIRECTION('center_axis',(0.988679578606276,0.,0.150042296859641));
#51328=DIRECTION('ref_axis',(0.150042296859641,0.,-0.988679578606276));
#51329=DIRECTION('',(0.,1.,0.));
#51330=DIRECTION('',(0.,1.,0.));
#51331=DIRECTION('center_axis',(0.364399348580517,0.,0.931242779705752));
#51332=DIRECTION('ref_axis',(0.931242779705752,0.,-0.364399348580517));
#51333=DIRECTION('',(0.,1.,0.));
#51334=DIRECTION('center_axis',(-0.624280230025758,0.,0.781200482846104));
#51335=DIRECTION('ref_axis',(0.781200482846104,0.,0.624280230025758));
#51336=DIRECTION('',(0.,1.,0.));
#51337=DIRECTION('center_axis',(-0.988679578606275,0.,-0.150042296859647));
#51338=DIRECTION('ref_axis',(-0.150042296859647,0.,0.988679578606275));
#51339=DIRECTION('',(0.,1.,0.));
#51340=DIRECTION('center_axis',(-0.364399348580519,0.,-0.931242779705751));
#51341=DIRECTION('ref_axis',(-0.931242779705751,0.,0.364399348580519));
#51342=DIRECTION('',(0.,1.,0.));
#51343=DIRECTION('center_axis',(0.624280230025758,0.,-0.781200482846105));
#51344=DIRECTION('ref_axis',(-0.781200482846105,0.,-0.624280230025758));
#51345=DIRECTION('center_axis',(0.988679578606276,0.,0.150042296859641));
#51346=DIRECTION('ref_axis',(0.150042296859641,0.,-0.988679578606276));
#51347=DIRECTION('',(0.,1.,0.));
#51348=DIRECTION('',(0.,1.,0.));
#51349=DIRECTION('center_axis',(0.364399348580517,0.,0.931242779705752));
#51350=DIRECTION('ref_axis',(0.931242779705752,0.,-0.364399348580517));
#51351=DIRECTION('',(0.,1.,0.));
#51352=DIRECTION('center_axis',(-0.624280230025758,0.,0.781200482846104));
#51353=DIRECTION('ref_axis',(0.781200482846104,0.,0.624280230025758));
#51354=DIRECTION('',(0.,1.,0.));
#51355=DIRECTION('center_axis',(-0.988679578606275,0.,-0.150042296859647));
#51356=DIRECTION('ref_axis',(-0.150042296859647,0.,0.988679578606275));
#51357=DIRECTION('',(0.,1.,0.));
#51358=DIRECTION('center_axis',(-0.364399348580519,0.,-0.931242779705751));
#51359=DIRECTION('ref_axis',(-0.931242779705751,0.,0.364399348580519));
#51360=DIRECTION('',(0.,1.,0.));
#51361=DIRECTION('center_axis',(0.624280230025758,0.,-0.781200482846105));
#51362=DIRECTION('ref_axis',(-0.781200482846105,0.,-0.624280230025758));
#51363=DIRECTION('center_axis',(0.988679578606276,0.,0.150042296859641));
#51364=DIRECTION('ref_axis',(0.150042296859641,0.,-0.988679578606276));
#51365=DIRECTION('',(0.,1.,0.));
#51366=DIRECTION('',(0.,1.,0.));
#51367=DIRECTION('center_axis',(0.364399348580517,0.,0.931242779705752));
#51368=DIRECTION('ref_axis',(0.931242779705752,0.,-0.364399348580517));
#51369=DIRECTION('',(0.,1.,0.));
#51370=DIRECTION('center_axis',(-0.624280230025758,0.,0.781200482846104));
#51371=DIRECTION('ref_axis',(0.781200482846104,0.,0.624280230025758));
#51372=DIRECTION('',(0.,1.,0.));
#51373=DIRECTION('center_axis',(-0.988679578606275,0.,-0.150042296859647));
#51374=DIRECTION('ref_axis',(-0.150042296859647,0.,0.988679578606275));
#51375=DIRECTION('',(0.,1.,0.));
#51376=DIRECTION('center_axis',(-0.364399348580519,0.,-0.931242779705751));
#51377=DIRECTION('ref_axis',(-0.931242779705751,0.,0.364399348580519));
#51378=DIRECTION('',(0.,1.,0.));
#51379=DIRECTION('center_axis',(0.624280230025758,0.,-0.781200482846105));
#51380=DIRECTION('ref_axis',(-0.781200482846105,0.,-0.624280230025758));
#51381=DIRECTION('center_axis',(0.988679578606276,0.,0.150042296859641));
#51382=DIRECTION('ref_axis',(0.150042296859641,0.,-0.988679578606276));
#51383=DIRECTION('',(0.,1.,0.));
#51384=DIRECTION('',(0.,1.,0.));
#51385=DIRECTION('center_axis',(0.364399348580517,0.,0.931242779705752));
#51386=DIRECTION('ref_axis',(0.931242779705752,0.,-0.364399348580517));
#51387=DIRECTION('',(0.,1.,0.));
#51388=DIRECTION('center_axis',(-0.624280230025758,0.,0.781200482846104));
#51389=DIRECTION('ref_axis',(0.781200482846104,0.,0.624280230025758));
#51390=DIRECTION('',(0.,1.,0.));
#51391=DIRECTION('center_axis',(-0.988679578606275,0.,-0.150042296859647));
#51392=DIRECTION('ref_axis',(-0.150042296859647,0.,0.988679578606275));
#51393=DIRECTION('',(0.,1.,0.));
#51394=DIRECTION('center_axis',(-0.364399348580519,0.,-0.931242779705751));
#51395=DIRECTION('ref_axis',(-0.931242779705751,0.,0.364399348580519));
#51396=DIRECTION('',(0.,1.,0.));
#51397=DIRECTION('center_axis',(0.624280230025758,0.,-0.781200482846105));
#51398=DIRECTION('ref_axis',(-0.781200482846105,0.,-0.624280230025758));
#51399=DIRECTION('center_axis',(0.988679578606276,0.,0.150042296859641));
#51400=DIRECTION('ref_axis',(0.150042296859641,0.,-0.988679578606276));
#51401=DIRECTION('',(0.,1.,0.));
#51402=DIRECTION('',(0.,1.,0.));
#51403=DIRECTION('center_axis',(0.364399348580517,0.,0.931242779705752));
#51404=DIRECTION('ref_axis',(0.931242779705752,0.,-0.364399348580517));
#51405=DIRECTION('',(0.,1.,0.));
#51406=DIRECTION('center_axis',(-0.624280230025758,0.,0.781200482846104));
#51407=DIRECTION('ref_axis',(0.781200482846104,0.,0.624280230025758));
#51408=DIRECTION('',(0.,1.,0.));
#51409=DIRECTION('center_axis',(-0.988679578606275,0.,-0.150042296859647));
#51410=DIRECTION('ref_axis',(-0.150042296859647,0.,0.988679578606275));
#51411=DIRECTION('',(0.,1.,0.));
#51412=DIRECTION('center_axis',(-0.364399348580519,0.,-0.931242779705751));
#51413=DIRECTION('ref_axis',(-0.931242779705751,0.,0.364399348580519));
#51414=DIRECTION('',(0.,1.,0.));
#51415=DIRECTION('center_axis',(0.624280230025758,0.,-0.781200482846105));
#51416=DIRECTION('ref_axis',(-0.781200482846105,0.,-0.624280230025758));
#51417=DIRECTION('center_axis',(0.988679578606276,0.,0.150042296859641));
#51418=DIRECTION('ref_axis',(0.150042296859641,0.,-0.988679578606276));
#51419=DIRECTION('',(0.,1.,0.));
#51420=DIRECTION('',(0.,1.,0.));
#51421=DIRECTION('center_axis',(0.364399348580517,0.,0.931242779705752));
#51422=DIRECTION('ref_axis',(0.931242779705752,0.,-0.364399348580517));
#51423=DIRECTION('',(0.,1.,0.));
#51424=DIRECTION('center_axis',(-0.624280230025758,0.,0.781200482846104));
#51425=DIRECTION('ref_axis',(0.781200482846104,0.,0.624280230025758));
#51426=DIRECTION('',(0.,1.,0.));
#51427=DIRECTION('center_axis',(-0.988679578606275,0.,-0.150042296859647));
#51428=DIRECTION('ref_axis',(-0.150042296859647,0.,0.988679578606275));
#51429=DIRECTION('',(0.,1.,0.));
#51430=DIRECTION('center_axis',(-0.364399348580519,0.,-0.931242779705751));
#51431=DIRECTION('ref_axis',(-0.931242779705751,0.,0.364399348580519));
#51432=DIRECTION('',(0.,1.,0.));
#51433=DIRECTION('center_axis',(0.624280230025758,0.,-0.781200482846105));
#51434=DIRECTION('ref_axis',(-0.781200482846105,0.,-0.624280230025758));
#51435=DIRECTION('center_axis',(0.988679578606276,0.,0.150042296859641));
#51436=DIRECTION('ref_axis',(0.150042296859641,0.,-0.988679578606276));
#51437=DIRECTION('',(0.,1.,0.));
#51438=DIRECTION('',(0.,1.,0.));
#51439=DIRECTION('center_axis',(0.364399348580517,0.,0.931242779705752));
#51440=DIRECTION('ref_axis',(0.931242779705752,0.,-0.364399348580517));
#51441=DIRECTION('',(0.,1.,0.));
#51442=DIRECTION('center_axis',(-0.624280230025758,0.,0.781200482846104));
#51443=DIRECTION('ref_axis',(0.781200482846104,0.,0.624280230025758));
#51444=DIRECTION('',(0.,1.,0.));
#51445=DIRECTION('center_axis',(-0.988679578606275,0.,-0.150042296859647));
#51446=DIRECTION('ref_axis',(-0.150042296859647,0.,0.988679578606275));
#51447=DIRECTION('',(0.,1.,0.));
#51448=DIRECTION('center_axis',(-0.364399348580519,0.,-0.931242779705751));
#51449=DIRECTION('ref_axis',(-0.931242779705751,0.,0.364399348580519));
#51450=DIRECTION('',(0.,1.,0.));
#51451=DIRECTION('center_axis',(0.624280230025758,0.,-0.781200482846105));
#51452=DIRECTION('ref_axis',(-0.781200482846105,0.,-0.624280230025758));
#51453=DIRECTION('center_axis',(0.988679578606276,0.,0.150042296859641));
#51454=DIRECTION('ref_axis',(0.150042296859641,0.,-0.988679578606276));
#51455=DIRECTION('',(0.,1.,0.));
#51456=DIRECTION('',(0.,1.,0.));
#51457=DIRECTION('center_axis',(0.364399348580517,0.,0.931242779705752));
#51458=DIRECTION('ref_axis',(0.931242779705752,0.,-0.364399348580517));
#51459=DIRECTION('',(0.,1.,0.));
#51460=DIRECTION('center_axis',(-0.624280230025758,0.,0.781200482846104));
#51461=DIRECTION('ref_axis',(0.781200482846104,0.,0.624280230025758));
#51462=DIRECTION('',(0.,1.,0.));
#51463=DIRECTION('center_axis',(-0.988679578606275,0.,-0.150042296859647));
#51464=DIRECTION('ref_axis',(-0.150042296859647,0.,0.988679578606275));
#51465=DIRECTION('',(0.,1.,0.));
#51466=DIRECTION('center_axis',(-0.364399348580519,0.,-0.931242779705751));
#51467=DIRECTION('ref_axis',(-0.931242779705751,0.,0.364399348580519));
#51468=DIRECTION('',(0.,1.,0.));
#51469=DIRECTION('center_axis',(0.624280230025758,0.,-0.781200482846105));
#51470=DIRECTION('ref_axis',(-0.781200482846105,0.,-0.624280230025758));
#51471=DIRECTION('center_axis',(0.988679578606276,0.,0.150042296859641));
#51472=DIRECTION('ref_axis',(0.150042296859641,0.,-0.988679578606276));
#51473=DIRECTION('',(0.,1.,0.));
#51474=DIRECTION('',(0.,1.,0.));
#51475=DIRECTION('center_axis',(0.364399348580517,0.,0.931242779705752));
#51476=DIRECTION('ref_axis',(0.931242779705752,0.,-0.364399348580517));
#51477=DIRECTION('',(0.,1.,0.));
#51478=DIRECTION('center_axis',(-0.624280230025758,0.,0.781200482846104));
#51479=DIRECTION('ref_axis',(0.781200482846104,0.,0.624280230025758));
#51480=DIRECTION('',(0.,1.,0.));
#51481=DIRECTION('center_axis',(-0.988679578606275,0.,-0.150042296859647));
#51482=DIRECTION('ref_axis',(-0.150042296859647,0.,0.988679578606275));
#51483=DIRECTION('',(0.,1.,0.));
#51484=DIRECTION('center_axis',(-0.364399348580519,0.,-0.931242779705751));
#51485=DIRECTION('ref_axis',(-0.931242779705751,0.,0.364399348580519));
#51486=DIRECTION('',(0.,1.,0.));
#51487=DIRECTION('center_axis',(0.624280230025758,0.,-0.781200482846105));
#51488=DIRECTION('ref_axis',(-0.781200482846105,0.,-0.624280230025758));
#51489=DIRECTION('center_axis',(0.988679578606276,0.,0.150042296859641));
#51490=DIRECTION('ref_axis',(0.150042296859641,0.,-0.988679578606276));
#51491=DIRECTION('',(0.,1.,0.));
#51492=DIRECTION('',(0.,1.,0.));
#51493=DIRECTION('center_axis',(0.364399348580517,0.,0.931242779705752));
#51494=DIRECTION('ref_axis',(0.931242779705752,0.,-0.364399348580517));
#51495=DIRECTION('',(0.,1.,0.));
#51496=DIRECTION('center_axis',(-0.624280230025758,0.,0.781200482846104));
#51497=DIRECTION('ref_axis',(0.781200482846104,0.,0.624280230025758));
#51498=DIRECTION('',(0.,1.,0.));
#51499=DIRECTION('center_axis',(-0.988679578606275,0.,-0.150042296859647));
#51500=DIRECTION('ref_axis',(-0.150042296859647,0.,0.988679578606275));
#51501=DIRECTION('',(0.,1.,0.));
#51502=DIRECTION('center_axis',(-0.364399348580519,0.,-0.931242779705751));
#51503=DIRECTION('ref_axis',(-0.931242779705751,0.,0.364399348580519));
#51504=DIRECTION('',(0.,1.,0.));
#51505=DIRECTION('center_axis',(0.624280230025758,0.,-0.781200482846105));
#51506=DIRECTION('ref_axis',(-0.781200482846105,0.,-0.624280230025758));
#51507=DIRECTION('center_axis',(0.988679578606276,0.,0.150042296859641));
#51508=DIRECTION('ref_axis',(0.150042296859641,0.,-0.988679578606276));
#51509=DIRECTION('',(0.,1.,0.));
#51510=DIRECTION('',(0.,1.,0.));
#51511=DIRECTION('center_axis',(0.364399348580517,0.,0.931242779705752));
#51512=DIRECTION('ref_axis',(0.931242779705752,0.,-0.364399348580517));
#51513=DIRECTION('',(0.,1.,0.));
#51514=DIRECTION('center_axis',(-0.624280230025758,0.,0.781200482846104));
#51515=DIRECTION('ref_axis',(0.781200482846104,0.,0.624280230025758));
#51516=DIRECTION('',(0.,1.,0.));
#51517=DIRECTION('center_axis',(-0.988679578606275,0.,-0.150042296859647));
#51518=DIRECTION('ref_axis',(-0.150042296859647,0.,0.988679578606275));
#51519=DIRECTION('',(0.,1.,0.));
#51520=DIRECTION('center_axis',(-0.364399348580519,0.,-0.931242779705751));
#51521=DIRECTION('ref_axis',(-0.931242779705751,0.,0.364399348580519));
#51522=DIRECTION('',(0.,1.,0.));
#51523=DIRECTION('center_axis',(0.624280230025758,0.,-0.781200482846105));
#51524=DIRECTION('ref_axis',(-0.781200482846105,0.,-0.624280230025758));
#51525=DIRECTION('center_axis',(0.988679578606276,0.,0.150042296859641));
#51526=DIRECTION('ref_axis',(0.150042296859641,0.,-0.988679578606276));
#51527=DIRECTION('',(0.,1.,0.));
#51528=DIRECTION('',(0.,1.,0.));
#51529=DIRECTION('center_axis',(0.364399348580517,0.,0.931242779705752));
#51530=DIRECTION('ref_axis',(0.931242779705752,0.,-0.364399348580517));
#51531=DIRECTION('',(0.,1.,0.));
#51532=DIRECTION('center_axis',(-0.624280230025758,0.,0.781200482846104));
#51533=DIRECTION('ref_axis',(0.781200482846104,0.,0.624280230025758));
#51534=DIRECTION('',(0.,1.,0.));
#51535=DIRECTION('center_axis',(-0.988679578606275,0.,-0.150042296859647));
#51536=DIRECTION('ref_axis',(-0.150042296859647,0.,0.988679578606275));
#51537=DIRECTION('',(0.,1.,0.));
#51538=DIRECTION('center_axis',(-0.364399348580519,0.,-0.931242779705751));
#51539=DIRECTION('ref_axis',(-0.931242779705751,0.,0.364399348580519));
#51540=DIRECTION('',(0.,1.,0.));
#51541=DIRECTION('center_axis',(0.624280230025758,0.,-0.781200482846105));
#51542=DIRECTION('ref_axis',(-0.781200482846105,0.,-0.624280230025758));
#51543=DIRECTION('center_axis',(0.988679578606276,0.,0.150042296859641));
#51544=DIRECTION('ref_axis',(0.150042296859641,0.,-0.988679578606276));
#51545=DIRECTION('',(0.,1.,0.));
#51546=DIRECTION('',(0.,1.,0.));
#51547=DIRECTION('center_axis',(0.364399348580517,0.,0.931242779705752));
#51548=DIRECTION('ref_axis',(0.931242779705752,0.,-0.364399348580517));
#51549=DIRECTION('',(0.,1.,0.));
#51550=DIRECTION('center_axis',(-0.624280230025758,0.,0.781200482846104));
#51551=DIRECTION('ref_axis',(0.781200482846104,0.,0.624280230025758));
#51552=DIRECTION('',(0.,1.,0.));
#51553=DIRECTION('center_axis',(-0.988679578606275,0.,-0.150042296859647));
#51554=DIRECTION('ref_axis',(-0.150042296859647,0.,0.988679578606275));
#51555=DIRECTION('',(0.,1.,0.));
#51556=DIRECTION('center_axis',(-0.364399348580519,0.,-0.931242779705751));
#51557=DIRECTION('ref_axis',(-0.931242779705751,0.,0.364399348580519));
#51558=DIRECTION('',(0.,1.,0.));
#51559=DIRECTION('center_axis',(0.624280230025758,0.,-0.781200482846105));
#51560=DIRECTION('ref_axis',(-0.781200482846105,0.,-0.624280230025758));
#51561=DIRECTION('center_axis',(0.988679578606276,0.,0.150042296859641));
#51562=DIRECTION('ref_axis',(0.150042296859641,0.,-0.988679578606276));
#51563=DIRECTION('',(0.,1.,0.));
#51564=DIRECTION('',(0.,1.,0.));
#51565=DIRECTION('center_axis',(0.364399348580517,0.,0.931242779705752));
#51566=DIRECTION('ref_axis',(0.931242779705752,0.,-0.364399348580517));
#51567=DIRECTION('',(0.,1.,0.));
#51568=DIRECTION('center_axis',(-0.624280230025758,0.,0.781200482846104));
#51569=DIRECTION('ref_axis',(0.781200482846104,0.,0.624280230025758));
#51570=DIRECTION('',(0.,1.,0.));
#51571=DIRECTION('center_axis',(-0.988679578606275,0.,-0.150042296859647));
#51572=DIRECTION('ref_axis',(-0.150042296859647,0.,0.988679578606275));
#51573=DIRECTION('',(0.,1.,0.));
#51574=DIRECTION('center_axis',(-0.364399348580519,0.,-0.931242779705751));
#51575=DIRECTION('ref_axis',(-0.931242779705751,0.,0.364399348580519));
#51576=DIRECTION('',(0.,1.,0.));
#51577=DIRECTION('center_axis',(0.624280230025758,0.,-0.781200482846105));
#51578=DIRECTION('ref_axis',(-0.781200482846105,0.,-0.624280230025758));
#51579=DIRECTION('center_axis',(0.988679578606276,0.,0.150042296859641));
#51580=DIRECTION('ref_axis',(0.150042296859641,0.,-0.988679578606276));
#51581=DIRECTION('',(0.,1.,0.));
#51582=DIRECTION('',(0.,1.,0.));
#51583=DIRECTION('center_axis',(0.364399348580517,0.,0.931242779705752));
#51584=DIRECTION('ref_axis',(0.931242779705752,0.,-0.364399348580517));
#51585=DIRECTION('',(0.,1.,0.));
#51586=DIRECTION('center_axis',(-0.624280230025758,0.,0.781200482846104));
#51587=DIRECTION('ref_axis',(0.781200482846104,0.,0.624280230025758));
#51588=DIRECTION('',(0.,1.,0.));
#51589=DIRECTION('center_axis',(-0.988679578606275,0.,-0.150042296859647));
#51590=DIRECTION('ref_axis',(-0.150042296859647,0.,0.988679578606275));
#51591=DIRECTION('',(0.,1.,0.));
#51592=DIRECTION('center_axis',(-0.364399348580519,0.,-0.931242779705751));
#51593=DIRECTION('ref_axis',(-0.931242779705751,0.,0.364399348580519));
#51594=DIRECTION('',(0.,1.,0.));
#51595=DIRECTION('center_axis',(0.624280230025758,0.,-0.781200482846105));
#51596=DIRECTION('ref_axis',(-0.781200482846105,0.,-0.624280230025758));
#51597=DIRECTION('center_axis',(0.988679578606276,0.,0.150042296859641));
#51598=DIRECTION('ref_axis',(0.150042296859641,0.,-0.988679578606276));
#51599=DIRECTION('',(0.,1.,0.));
#51600=DIRECTION('',(0.,1.,0.));
#51601=DIRECTION('center_axis',(0.364399348580517,0.,0.931242779705752));
#51602=DIRECTION('ref_axis',(0.931242779705752,0.,-0.364399348580517));
#51603=DIRECTION('',(0.,1.,0.));
#51604=DIRECTION('center_axis',(-0.624280230025758,0.,0.781200482846104));
#51605=DIRECTION('ref_axis',(0.781200482846104,0.,0.624280230025758));
#51606=DIRECTION('',(0.,1.,0.));
#51607=DIRECTION('center_axis',(-0.988679578606275,0.,-0.150042296859647));
#51608=DIRECTION('ref_axis',(-0.150042296859647,0.,0.988679578606275));
#51609=DIRECTION('',(0.,1.,0.));
#51610=DIRECTION('center_axis',(-0.364399348580519,0.,-0.931242779705751));
#51611=DIRECTION('ref_axis',(-0.931242779705751,0.,0.364399348580519));
#51612=DIRECTION('',(0.,1.,0.));
#51613=DIRECTION('center_axis',(0.624280230025758,0.,-0.781200482846105));
#51614=DIRECTION('ref_axis',(-0.781200482846105,0.,-0.624280230025758));
#51615=DIRECTION('center_axis',(0.988679578606276,0.,0.150042296859641));
#51616=DIRECTION('ref_axis',(0.150042296859641,0.,-0.988679578606276));
#51617=DIRECTION('',(0.,1.,0.));
#51618=DIRECTION('',(0.,1.,0.));
#51619=DIRECTION('center_axis',(0.364399348580517,0.,0.931242779705752));
#51620=DIRECTION('ref_axis',(0.931242779705752,0.,-0.364399348580517));
#51621=DIRECTION('',(0.,1.,0.));
#51622=DIRECTION('center_axis',(-0.624280230025758,0.,0.781200482846104));
#51623=DIRECTION('ref_axis',(0.781200482846104,0.,0.624280230025758));
#51624=DIRECTION('',(0.,1.,0.));
#51625=DIRECTION('center_axis',(-0.988679578606275,0.,-0.150042296859647));
#51626=DIRECTION('ref_axis',(-0.150042296859647,0.,0.988679578606275));
#51627=DIRECTION('',(0.,1.,0.));
#51628=DIRECTION('center_axis',(-0.364399348580519,0.,-0.931242779705751));
#51629=DIRECTION('ref_axis',(-0.931242779705751,0.,0.364399348580519));
#51630=DIRECTION('',(0.,1.,0.));
#51631=DIRECTION('center_axis',(0.624280230025758,0.,-0.781200482846105));
#51632=DIRECTION('ref_axis',(-0.781200482846105,0.,-0.624280230025758));
#51633=DIRECTION('center_axis',(0.988679578606276,0.,0.150042296859641));
#51634=DIRECTION('ref_axis',(0.150042296859641,0.,-0.988679578606276));
#51635=DIRECTION('',(0.,1.,0.));
#51636=DIRECTION('',(0.,1.,0.));
#51637=DIRECTION('center_axis',(0.364399348580517,0.,0.931242779705752));
#51638=DIRECTION('ref_axis',(0.931242779705752,0.,-0.364399348580517));
#51639=DIRECTION('',(0.,1.,0.));
#51640=DIRECTION('center_axis',(-0.624280230025758,0.,0.781200482846104));
#51641=DIRECTION('ref_axis',(0.781200482846104,0.,0.624280230025758));
#51642=DIRECTION('',(0.,1.,0.));
#51643=DIRECTION('center_axis',(-0.988679578606275,0.,-0.150042296859647));
#51644=DIRECTION('ref_axis',(-0.150042296859647,0.,0.988679578606275));
#51645=DIRECTION('',(0.,1.,0.));
#51646=DIRECTION('center_axis',(-0.364399348580519,0.,-0.931242779705751));
#51647=DIRECTION('ref_axis',(-0.931242779705751,0.,0.364399348580519));
#51648=DIRECTION('',(0.,1.,0.));
#51649=DIRECTION('center_axis',(0.624280230025758,0.,-0.781200482846105));
#51650=DIRECTION('ref_axis',(-0.781200482846105,0.,-0.624280230025758));
#51651=DIRECTION('center_axis',(0.988679578606276,0.,0.150042296859641));
#51652=DIRECTION('ref_axis',(0.150042296859641,0.,-0.988679578606276));
#51653=DIRECTION('',(0.,1.,0.));
#51654=DIRECTION('',(0.,1.,0.));
#51655=DIRECTION('center_axis',(0.364399348580517,0.,0.931242779705752));
#51656=DIRECTION('ref_axis',(0.931242779705752,0.,-0.364399348580517));
#51657=DIRECTION('',(0.,1.,0.));
#51658=DIRECTION('center_axis',(-0.624280230025758,0.,0.781200482846104));
#51659=DIRECTION('ref_axis',(0.781200482846104,0.,0.624280230025758));
#51660=DIRECTION('',(0.,1.,0.));
#51661=DIRECTION('center_axis',(-0.988679578606275,0.,-0.150042296859647));
#51662=DIRECTION('ref_axis',(-0.150042296859647,0.,0.988679578606275));
#51663=DIRECTION('',(0.,1.,0.));
#51664=DIRECTION('center_axis',(-0.364399348580519,0.,-0.931242779705751));
#51665=DIRECTION('ref_axis',(-0.931242779705751,0.,0.364399348580519));
#51666=DIRECTION('',(0.,1.,0.));
#51667=DIRECTION('center_axis',(0.624280230025758,0.,-0.781200482846105));
#51668=DIRECTION('ref_axis',(-0.781200482846105,0.,-0.624280230025758));
#51669=DIRECTION('center_axis',(0.988679578606276,0.,0.150042296859641));
#51670=DIRECTION('ref_axis',(0.150042296859641,0.,-0.988679578606276));
#51671=DIRECTION('',(0.,1.,0.));
#51672=DIRECTION('',(0.,1.,0.));
#51673=DIRECTION('center_axis',(0.364399348580517,0.,0.931242779705752));
#51674=DIRECTION('ref_axis',(0.931242779705752,0.,-0.364399348580517));
#51675=DIRECTION('',(0.,1.,0.));
#51676=DIRECTION('center_axis',(-0.624280230025758,0.,0.781200482846104));
#51677=DIRECTION('ref_axis',(0.781200482846104,0.,0.624280230025758));
#51678=DIRECTION('',(0.,1.,0.));
#51679=DIRECTION('center_axis',(-0.988679578606275,0.,-0.150042296859647));
#51680=DIRECTION('ref_axis',(-0.150042296859647,0.,0.988679578606275));
#51681=DIRECTION('',(0.,1.,0.));
#51682=DIRECTION('center_axis',(-0.364399348580519,0.,-0.931242779705751));
#51683=DIRECTION('ref_axis',(-0.931242779705751,0.,0.364399348580519));
#51684=DIRECTION('',(0.,1.,0.));
#51685=DIRECTION('center_axis',(0.624280230025758,0.,-0.781200482846105));
#51686=DIRECTION('ref_axis',(-0.781200482846105,0.,-0.624280230025758));
#51687=DIRECTION('center_axis',(0.988679578606276,0.,0.150042296859641));
#51688=DIRECTION('ref_axis',(0.150042296859641,0.,-0.988679578606276));
#51689=DIRECTION('',(0.,1.,0.));
#51690=DIRECTION('',(0.,1.,0.));
#51691=DIRECTION('center_axis',(0.364399348580517,0.,0.931242779705752));
#51692=DIRECTION('ref_axis',(0.931242779705752,0.,-0.364399348580517));
#51693=DIRECTION('',(0.,1.,0.));
#51694=DIRECTION('center_axis',(-0.624280230025758,0.,0.781200482846104));
#51695=DIRECTION('ref_axis',(0.781200482846104,0.,0.624280230025758));
#51696=DIRECTION('',(0.,1.,0.));
#51697=DIRECTION('center_axis',(-0.988679578606275,0.,-0.150042296859647));
#51698=DIRECTION('ref_axis',(-0.150042296859647,0.,0.988679578606275));
#51699=DIRECTION('',(0.,1.,0.));
#51700=DIRECTION('center_axis',(-0.364399348580519,0.,-0.931242779705751));
#51701=DIRECTION('ref_axis',(-0.931242779705751,0.,0.364399348580519));
#51702=DIRECTION('',(0.,1.,0.));
#51703=DIRECTION('center_axis',(0.624280230025758,0.,-0.781200482846105));
#51704=DIRECTION('ref_axis',(-0.781200482846105,0.,-0.624280230025758));
#51705=DIRECTION('center_axis',(0.988679578606276,0.,0.150042296859641));
#51706=DIRECTION('ref_axis',(0.150042296859641,0.,-0.988679578606276));
#51707=DIRECTION('',(0.,1.,0.));
#51708=DIRECTION('',(0.,1.,0.));
#51709=DIRECTION('center_axis',(0.364399348580517,0.,0.931242779705752));
#51710=DIRECTION('ref_axis',(0.931242779705752,0.,-0.364399348580517));
#51711=DIRECTION('',(0.,1.,0.));
#51712=DIRECTION('center_axis',(-0.624280230025758,0.,0.781200482846104));
#51713=DIRECTION('ref_axis',(0.781200482846104,0.,0.624280230025758));
#51714=DIRECTION('',(0.,1.,0.));
#51715=DIRECTION('center_axis',(-0.988679578606275,0.,-0.150042296859647));
#51716=DIRECTION('ref_axis',(-0.150042296859647,0.,0.988679578606275));
#51717=DIRECTION('',(0.,1.,0.));
#51718=DIRECTION('center_axis',(-0.364399348580519,0.,-0.931242779705751));
#51719=DIRECTION('ref_axis',(-0.931242779705751,0.,0.364399348580519));
#51720=DIRECTION('',(0.,1.,0.));
#51721=DIRECTION('center_axis',(0.624280230025758,0.,-0.781200482846105));
#51722=DIRECTION('ref_axis',(-0.781200482846105,0.,-0.624280230025758));
#51723=DIRECTION('center_axis',(0.988679578606276,0.,0.150042296859641));
#51724=DIRECTION('ref_axis',(0.150042296859641,0.,-0.988679578606276));
#51725=DIRECTION('',(0.,1.,0.));
#51726=DIRECTION('',(0.,1.,0.));
#51727=DIRECTION('center_axis',(0.364399348580517,0.,0.931242779705752));
#51728=DIRECTION('ref_axis',(0.931242779705752,0.,-0.364399348580517));
#51729=DIRECTION('',(0.,1.,0.));
#51730=DIRECTION('center_axis',(-0.624280230025758,0.,0.781200482846104));
#51731=DIRECTION('ref_axis',(0.781200482846104,0.,0.624280230025758));
#51732=DIRECTION('',(0.,1.,0.));
#51733=DIRECTION('center_axis',(-0.988679578606275,0.,-0.150042296859647));
#51734=DIRECTION('ref_axis',(-0.150042296859647,0.,0.988679578606275));
#51735=DIRECTION('',(0.,1.,0.));
#51736=DIRECTION('center_axis',(-0.364399348580519,0.,-0.931242779705751));
#51737=DIRECTION('ref_axis',(-0.931242779705751,0.,0.364399348580519));
#51738=DIRECTION('',(0.,1.,0.));
#51739=DIRECTION('center_axis',(0.624280230025758,0.,-0.781200482846105));
#51740=DIRECTION('ref_axis',(-0.781200482846105,0.,-0.624280230025758));
#51741=DIRECTION('center_axis',(0.988679578606276,0.,0.150042296859641));
#51742=DIRECTION('ref_axis',(0.150042296859641,0.,-0.988679578606276));
#51743=DIRECTION('',(0.,1.,0.));
#51744=DIRECTION('',(0.,1.,0.));
#51745=DIRECTION('center_axis',(0.364399348580517,0.,0.931242779705752));
#51746=DIRECTION('ref_axis',(0.931242779705752,0.,-0.364399348580517));
#51747=DIRECTION('',(0.,1.,0.));
#51748=DIRECTION('center_axis',(-0.624280230025758,0.,0.781200482846104));
#51749=DIRECTION('ref_axis',(0.781200482846104,0.,0.624280230025758));
#51750=DIRECTION('',(0.,1.,0.));
#51751=DIRECTION('center_axis',(-0.988679578606275,0.,-0.150042296859647));
#51752=DIRECTION('ref_axis',(-0.150042296859647,0.,0.988679578606275));
#51753=DIRECTION('',(0.,1.,0.));
#51754=DIRECTION('center_axis',(-0.364399348580519,0.,-0.931242779705751));
#51755=DIRECTION('ref_axis',(-0.931242779705751,0.,0.364399348580519));
#51756=DIRECTION('',(0.,1.,0.));
#51757=DIRECTION('center_axis',(0.624280230025758,0.,-0.781200482846105));
#51758=DIRECTION('ref_axis',(-0.781200482846105,0.,-0.624280230025758));
#51759=DIRECTION('center_axis',(0.988679578606276,0.,0.150042296859641));
#51760=DIRECTION('ref_axis',(0.150042296859641,0.,-0.988679578606276));
#51761=DIRECTION('',(0.,1.,0.));
#51762=DIRECTION('',(0.,1.,0.));
#51763=DIRECTION('center_axis',(0.364399348580517,0.,0.931242779705752));
#51764=DIRECTION('ref_axis',(0.931242779705752,0.,-0.364399348580517));
#51765=DIRECTION('',(0.,1.,0.));
#51766=DIRECTION('center_axis',(-0.624280230025758,0.,0.781200482846104));
#51767=DIRECTION('ref_axis',(0.781200482846104,0.,0.624280230025758));
#51768=DIRECTION('',(0.,1.,0.));
#51769=DIRECTION('center_axis',(-0.988679578606275,0.,-0.150042296859647));
#51770=DIRECTION('ref_axis',(-0.150042296859647,0.,0.988679578606275));
#51771=DIRECTION('',(0.,1.,0.));
#51772=DIRECTION('center_axis',(-0.364399348580519,0.,-0.931242779705751));
#51773=DIRECTION('ref_axis',(-0.931242779705751,0.,0.364399348580519));
#51774=DIRECTION('',(0.,1.,0.));
#51775=DIRECTION('center_axis',(0.624280230025758,0.,-0.781200482846105));
#51776=DIRECTION('ref_axis',(-0.781200482846105,0.,-0.624280230025758));
#51777=DIRECTION('center_axis',(0.988679578606276,0.,0.150042296859641));
#51778=DIRECTION('ref_axis',(0.150042296859641,0.,-0.988679578606276));
#51779=DIRECTION('',(0.,1.,0.));
#51780=DIRECTION('',(0.,1.,0.));
#51781=DIRECTION('center_axis',(0.364399348580517,0.,0.931242779705752));
#51782=DIRECTION('ref_axis',(0.931242779705752,0.,-0.364399348580517));
#51783=DIRECTION('',(0.,1.,0.));
#51784=DIRECTION('center_axis',(-0.624280230025758,0.,0.781200482846104));
#51785=DIRECTION('ref_axis',(0.781200482846104,0.,0.624280230025758));
#51786=DIRECTION('',(0.,1.,0.));
#51787=DIRECTION('center_axis',(-0.988679578606275,0.,-0.150042296859647));
#51788=DIRECTION('ref_axis',(-0.150042296859647,0.,0.988679578606275));
#51789=DIRECTION('',(0.,1.,0.));
#51790=DIRECTION('center_axis',(-0.364399348580519,0.,-0.931242779705751));
#51791=DIRECTION('ref_axis',(-0.931242779705751,0.,0.364399348580519));
#51792=DIRECTION('',(0.,1.,0.));
#51793=DIRECTION('center_axis',(0.624280230025758,0.,-0.781200482846105));
#51794=DIRECTION('ref_axis',(-0.781200482846105,0.,-0.624280230025758));
#51795=DIRECTION('center_axis',(0.988679578606276,0.,0.150042296859641));
#51796=DIRECTION('ref_axis',(0.150042296859641,0.,-0.988679578606276));
#51797=DIRECTION('',(0.,1.,0.));
#51798=DIRECTION('',(0.,1.,0.));
#51799=DIRECTION('center_axis',(0.364399348580517,0.,0.931242779705752));
#51800=DIRECTION('ref_axis',(0.931242779705752,0.,-0.364399348580517));
#51801=DIRECTION('',(0.,1.,0.));
#51802=DIRECTION('center_axis',(-0.624280230025758,0.,0.781200482846104));
#51803=DIRECTION('ref_axis',(0.781200482846104,0.,0.624280230025758));
#51804=DIRECTION('',(0.,1.,0.));
#51805=DIRECTION('center_axis',(-0.988679578606275,0.,-0.150042296859647));
#51806=DIRECTION('ref_axis',(-0.150042296859647,0.,0.988679578606275));
#51807=DIRECTION('',(0.,1.,0.));
#51808=DIRECTION('center_axis',(-0.364399348580519,0.,-0.931242779705751));
#51809=DIRECTION('ref_axis',(-0.931242779705751,0.,0.364399348580519));
#51810=DIRECTION('',(0.,1.,0.));
#51811=DIRECTION('center_axis',(0.624280230025758,0.,-0.781200482846105));
#51812=DIRECTION('ref_axis',(-0.781200482846105,0.,-0.624280230025758));
#51813=DIRECTION('center_axis',(0.988679578606276,0.,0.150042296859641));
#51814=DIRECTION('ref_axis',(0.150042296859641,0.,-0.988679578606276));
#51815=DIRECTION('',(0.,1.,0.));
#51816=DIRECTION('',(0.,1.,0.));
#51817=DIRECTION('center_axis',(0.364399348580517,0.,0.931242779705752));
#51818=DIRECTION('ref_axis',(0.931242779705752,0.,-0.364399348580517));
#51819=DIRECTION('',(0.,1.,0.));
#51820=DIRECTION('center_axis',(-0.624280230025758,0.,0.781200482846104));
#51821=DIRECTION('ref_axis',(0.781200482846104,0.,0.624280230025758));
#51822=DIRECTION('',(0.,1.,0.));
#51823=DIRECTION('center_axis',(-0.988679578606275,0.,-0.150042296859647));
#51824=DIRECTION('ref_axis',(-0.150042296859647,0.,0.988679578606275));
#51825=DIRECTION('',(0.,1.,0.));
#51826=DIRECTION('center_axis',(-0.364399348580519,0.,-0.931242779705751));
#51827=DIRECTION('ref_axis',(-0.931242779705751,0.,0.364399348580519));
#51828=DIRECTION('',(0.,1.,0.));
#51829=DIRECTION('center_axis',(0.624280230025758,0.,-0.781200482846105));
#51830=DIRECTION('ref_axis',(-0.781200482846105,0.,-0.624280230025758));
#51831=DIRECTION('center_axis',(0.988679578606276,0.,0.150042296859641));
#51832=DIRECTION('ref_axis',(0.150042296859641,0.,-0.988679578606276));
#51833=DIRECTION('',(0.,1.,0.));
#51834=DIRECTION('',(0.,1.,0.));
#51835=DIRECTION('center_axis',(0.364399348580517,0.,0.931242779705752));
#51836=DIRECTION('ref_axis',(0.931242779705752,0.,-0.364399348580517));
#51837=DIRECTION('',(0.,1.,0.));
#51838=DIRECTION('center_axis',(-0.624280230025758,0.,0.781200482846104));
#51839=DIRECTION('ref_axis',(0.781200482846104,0.,0.624280230025758));
#51840=DIRECTION('',(0.,1.,0.));
#51841=DIRECTION('center_axis',(-0.988679578606275,0.,-0.150042296859647));
#51842=DIRECTION('ref_axis',(-0.150042296859647,0.,0.988679578606275));
#51843=DIRECTION('',(0.,1.,0.));
#51844=DIRECTION('center_axis',(-0.364399348580519,0.,-0.931242779705751));
#51845=DIRECTION('ref_axis',(-0.931242779705751,0.,0.364399348580519));
#51846=DIRECTION('',(0.,1.,0.));
#51847=DIRECTION('center_axis',(0.624280230025758,0.,-0.781200482846105));
#51848=DIRECTION('ref_axis',(-0.781200482846105,0.,-0.624280230025758));
#51849=DIRECTION('center_axis',(0.988679578606276,0.,0.150042296859641));
#51850=DIRECTION('ref_axis',(0.150042296859641,0.,-0.988679578606276));
#51851=DIRECTION('',(0.,1.,0.));
#51852=DIRECTION('',(0.,1.,0.));
#51853=DIRECTION('center_axis',(0.364399348580517,0.,0.931242779705752));
#51854=DIRECTION('ref_axis',(0.931242779705752,0.,-0.364399348580517));
#51855=DIRECTION('',(0.,1.,0.));
#51856=DIRECTION('center_axis',(-0.624280230025758,0.,0.781200482846104));
#51857=DIRECTION('ref_axis',(0.781200482846104,0.,0.624280230025758));
#51858=DIRECTION('',(0.,1.,0.));
#51859=DIRECTION('center_axis',(-0.988679578606275,0.,-0.150042296859647));
#51860=DIRECTION('ref_axis',(-0.150042296859647,0.,0.988679578606275));
#51861=DIRECTION('',(0.,1.,0.));
#51862=DIRECTION('center_axis',(-0.364399348580519,0.,-0.931242779705751));
#51863=DIRECTION('ref_axis',(-0.931242779705751,0.,0.364399348580519));
#51864=DIRECTION('',(0.,1.,0.));
#51865=DIRECTION('center_axis',(0.624280230025758,0.,-0.781200482846105));
#51866=DIRECTION('ref_axis',(-0.781200482846105,0.,-0.624280230025758));
#51867=DIRECTION('center_axis',(0.988679578606276,0.,0.150042296859641));
#51868=DIRECTION('ref_axis',(0.150042296859641,0.,-0.988679578606276));
#51869=DIRECTION('',(0.,1.,0.));
#51870=DIRECTION('',(0.,1.,0.));
#51871=DIRECTION('center_axis',(0.364399348580517,0.,0.931242779705752));
#51872=DIRECTION('ref_axis',(0.931242779705752,0.,-0.364399348580517));
#51873=DIRECTION('',(0.,1.,0.));
#51874=DIRECTION('center_axis',(-0.624280230025758,0.,0.781200482846104));
#51875=DIRECTION('ref_axis',(0.781200482846104,0.,0.624280230025758));
#51876=DIRECTION('',(0.,1.,0.));
#51877=DIRECTION('center_axis',(-0.988679578606275,0.,-0.150042296859647));
#51878=DIRECTION('ref_axis',(-0.150042296859647,0.,0.988679578606275));
#51879=DIRECTION('',(0.,1.,0.));
#51880=DIRECTION('center_axis',(-0.364399348580519,0.,-0.931242779705751));
#51881=DIRECTION('ref_axis',(-0.931242779705751,0.,0.364399348580519));
#51882=DIRECTION('',(0.,1.,0.));
#51883=DIRECTION('center_axis',(0.624280230025758,0.,-0.781200482846105));
#51884=DIRECTION('ref_axis',(-0.781200482846105,0.,-0.624280230025758));
#51885=DIRECTION('center_axis',(0.988679578606276,0.,0.150042296859641));
#51886=DIRECTION('ref_axis',(0.150042296859641,0.,-0.988679578606276));
#51887=DIRECTION('',(0.,1.,0.));
#51888=DIRECTION('',(0.,1.,0.));
#51889=DIRECTION('center_axis',(0.364399348580517,0.,0.931242779705752));
#51890=DIRECTION('ref_axis',(0.931242779705752,0.,-0.364399348580517));
#51891=DIRECTION('',(0.,1.,0.));
#51892=DIRECTION('center_axis',(-0.624280230025758,0.,0.781200482846104));
#51893=DIRECTION('ref_axis',(0.781200482846104,0.,0.624280230025758));
#51894=DIRECTION('',(0.,1.,0.));
#51895=DIRECTION('center_axis',(-0.988679578606275,0.,-0.150042296859647));
#51896=DIRECTION('ref_axis',(-0.150042296859647,0.,0.988679578606275));
#51897=DIRECTION('',(0.,1.,0.));
#51898=DIRECTION('center_axis',(-0.364399348580519,0.,-0.931242779705751));
#51899=DIRECTION('ref_axis',(-0.931242779705751,0.,0.364399348580519));
#51900=DIRECTION('',(0.,1.,0.));
#51901=DIRECTION('center_axis',(0.624280230025758,0.,-0.781200482846105));
#51902=DIRECTION('ref_axis',(-0.781200482846105,0.,-0.624280230025758));
#51903=DIRECTION('center_axis',(0.988679578606276,0.,0.150042296859641));
#51904=DIRECTION('ref_axis',(0.150042296859641,0.,-0.988679578606276));
#51905=DIRECTION('',(0.,1.,0.));
#51906=DIRECTION('',(0.,1.,0.));
#51907=DIRECTION('center_axis',(0.364399348580517,0.,0.931242779705752));
#51908=DIRECTION('ref_axis',(0.931242779705752,0.,-0.364399348580517));
#51909=DIRECTION('',(0.,1.,0.));
#51910=DIRECTION('center_axis',(-0.624280230025758,0.,0.781200482846104));
#51911=DIRECTION('ref_axis',(0.781200482846104,0.,0.624280230025758));
#51912=DIRECTION('',(0.,1.,0.));
#51913=DIRECTION('center_axis',(-0.988679578606275,0.,-0.150042296859647));
#51914=DIRECTION('ref_axis',(-0.150042296859647,0.,0.988679578606275));
#51915=DIRECTION('',(0.,1.,0.));
#51916=DIRECTION('center_axis',(-0.364399348580519,0.,-0.931242779705751));
#51917=DIRECTION('ref_axis',(-0.931242779705751,0.,0.364399348580519));
#51918=DIRECTION('',(0.,1.,0.));
#51919=DIRECTION('center_axis',(0.624280230025758,0.,-0.781200482846105));
#51920=DIRECTION('ref_axis',(-0.781200482846105,0.,-0.624280230025758));
#51921=DIRECTION('center_axis',(0.988679578606276,0.,0.150042296859641));
#51922=DIRECTION('ref_axis',(0.150042296859641,0.,-0.988679578606276));
#51923=DIRECTION('',(0.,1.,0.));
#51924=DIRECTION('',(0.,1.,0.));
#51925=DIRECTION('center_axis',(0.364399348580517,0.,0.931242779705752));
#51926=DIRECTION('ref_axis',(0.931242779705752,0.,-0.364399348580517));
#51927=DIRECTION('',(0.,1.,0.));
#51928=DIRECTION('center_axis',(-0.624280230025758,0.,0.781200482846104));
#51929=DIRECTION('ref_axis',(0.781200482846104,0.,0.624280230025758));
#51930=DIRECTION('',(0.,1.,0.));
#51931=DIRECTION('center_axis',(-0.988679578606275,0.,-0.150042296859647));
#51932=DIRECTION('ref_axis',(-0.150042296859647,0.,0.988679578606275));
#51933=DIRECTION('',(0.,1.,0.));
#51934=DIRECTION('center_axis',(-0.364399348580519,0.,-0.931242779705751));
#51935=DIRECTION('ref_axis',(-0.931242779705751,0.,0.364399348580519));
#51936=DIRECTION('',(0.,1.,0.));
#51937=DIRECTION('center_axis',(0.624280230025758,0.,-0.781200482846105));
#51938=DIRECTION('ref_axis',(-0.781200482846105,0.,-0.624280230025758));
#51939=DIRECTION('center_axis',(0.988679578606276,0.,0.150042296859641));
#51940=DIRECTION('ref_axis',(0.150042296859641,0.,-0.988679578606276));
#51941=DIRECTION('',(0.,1.,0.));
#51942=DIRECTION('',(0.,1.,0.));
#51943=DIRECTION('center_axis',(0.364399348580517,0.,0.931242779705752));
#51944=DIRECTION('ref_axis',(0.931242779705752,0.,-0.364399348580517));
#51945=DIRECTION('',(0.,1.,0.));
#51946=DIRECTION('center_axis',(-0.624280230025758,0.,0.781200482846104));
#51947=DIRECTION('ref_axis',(0.781200482846104,0.,0.624280230025758));
#51948=DIRECTION('',(0.,1.,0.));
#51949=DIRECTION('center_axis',(-0.988679578606275,0.,-0.150042296859647));
#51950=DIRECTION('ref_axis',(-0.150042296859647,0.,0.988679578606275));
#51951=DIRECTION('',(0.,1.,0.));
#51952=DIRECTION('center_axis',(-0.364399348580519,0.,-0.931242779705751));
#51953=DIRECTION('ref_axis',(-0.931242779705751,0.,0.364399348580519));
#51954=DIRECTION('',(0.,1.,0.));
#51955=DIRECTION('center_axis',(0.624280230025758,0.,-0.781200482846105));
#51956=DIRECTION('ref_axis',(-0.781200482846105,0.,-0.624280230025758));
#51957=DIRECTION('center_axis',(0.988679578606276,0.,0.150042296859641));
#51958=DIRECTION('ref_axis',(0.150042296859641,0.,-0.988679578606276));
#51959=DIRECTION('',(0.,1.,0.));
#51960=DIRECTION('',(0.,1.,0.));
#51961=DIRECTION('center_axis',(0.364399348580517,0.,0.931242779705752));
#51962=DIRECTION('ref_axis',(0.931242779705752,0.,-0.364399348580517));
#51963=DIRECTION('',(0.,1.,0.));
#51964=DIRECTION('center_axis',(-0.624280230025758,0.,0.781200482846104));
#51965=DIRECTION('ref_axis',(0.781200482846104,0.,0.624280230025758));
#51966=DIRECTION('',(0.,1.,0.));
#51967=DIRECTION('center_axis',(-0.988679578606275,0.,-0.150042296859647));
#51968=DIRECTION('ref_axis',(-0.150042296859647,0.,0.988679578606275));
#51969=DIRECTION('',(0.,1.,0.));
#51970=DIRECTION('center_axis',(-0.364399348580519,0.,-0.931242779705751));
#51971=DIRECTION('ref_axis',(-0.931242779705751,0.,0.364399348580519));
#51972=DIRECTION('',(0.,1.,0.));
#51973=DIRECTION('center_axis',(0.624280230025758,0.,-0.781200482846105));
#51974=DIRECTION('ref_axis',(-0.781200482846105,0.,-0.624280230025758));
#51975=DIRECTION('center_axis',(0.988679578606276,0.,0.150042296859641));
#51976=DIRECTION('ref_axis',(0.150042296859641,0.,-0.988679578606276));
#51977=DIRECTION('',(0.,1.,0.));
#51978=DIRECTION('',(0.,1.,0.));
#51979=DIRECTION('center_axis',(0.364399348580517,0.,0.931242779705752));
#51980=DIRECTION('ref_axis',(0.931242779705752,0.,-0.364399348580517));
#51981=DIRECTION('',(0.,1.,0.));
#51982=DIRECTION('center_axis',(-0.624280230025758,0.,0.781200482846104));
#51983=DIRECTION('ref_axis',(0.781200482846104,0.,0.624280230025758));
#51984=DIRECTION('',(0.,1.,0.));
#51985=DIRECTION('center_axis',(-0.988679578606275,0.,-0.150042296859647));
#51986=DIRECTION('ref_axis',(-0.150042296859647,0.,0.988679578606275));
#51987=DIRECTION('',(0.,1.,0.));
#51988=DIRECTION('center_axis',(-0.364399348580519,0.,-0.931242779705751));
#51989=DIRECTION('ref_axis',(-0.931242779705751,0.,0.364399348580519));
#51990=DIRECTION('',(0.,1.,0.));
#51991=DIRECTION('center_axis',(0.624280230025758,0.,-0.781200482846105));
#51992=DIRECTION('ref_axis',(-0.781200482846105,0.,-0.624280230025758));
#51993=DIRECTION('center_axis',(0.988679578606276,0.,0.150042296859641));
#51994=DIRECTION('ref_axis',(0.150042296859641,0.,-0.988679578606276));
#51995=DIRECTION('',(0.,1.,0.));
#51996=DIRECTION('',(0.,1.,0.));
#51997=DIRECTION('center_axis',(0.364399348580517,0.,0.931242779705752));
#51998=DIRECTION('ref_axis',(0.931242779705752,0.,-0.364399348580517));
#51999=DIRECTION('',(0.,1.,0.));
#52000=DIRECTION('center_axis',(-0.624280230025758,0.,0.781200482846104));
#52001=DIRECTION('ref_axis',(0.781200482846104,0.,0.624280230025758));
#52002=DIRECTION('',(0.,1.,0.));
#52003=DIRECTION('center_axis',(-0.988679578606275,0.,-0.150042296859647));
#52004=DIRECTION('ref_axis',(-0.150042296859647,0.,0.988679578606275));
#52005=DIRECTION('',(0.,1.,0.));
#52006=DIRECTION('center_axis',(-0.364399348580519,0.,-0.931242779705751));
#52007=DIRECTION('ref_axis',(-0.931242779705751,0.,0.364399348580519));
#52008=DIRECTION('',(0.,1.,0.));
#52009=DIRECTION('center_axis',(0.624280230025758,0.,-0.781200482846105));
#52010=DIRECTION('ref_axis',(-0.781200482846105,0.,-0.624280230025758));
#52011=DIRECTION('center_axis',(0.988679578606276,0.,0.150042296859641));
#52012=DIRECTION('ref_axis',(0.150042296859641,0.,-0.988679578606276));
#52013=DIRECTION('',(0.,1.,0.));
#52014=DIRECTION('',(0.,1.,0.));
#52015=DIRECTION('center_axis',(0.364399348580517,0.,0.931242779705752));
#52016=DIRECTION('ref_axis',(0.931242779705752,0.,-0.364399348580517));
#52017=DIRECTION('',(0.,1.,0.));
#52018=DIRECTION('center_axis',(-0.624280230025758,0.,0.781200482846104));
#52019=DIRECTION('ref_axis',(0.781200482846104,0.,0.624280230025758));
#52020=DIRECTION('',(0.,1.,0.));
#52021=DIRECTION('center_axis',(-0.988679578606275,0.,-0.150042296859647));
#52022=DIRECTION('ref_axis',(-0.150042296859647,0.,0.988679578606275));
#52023=DIRECTION('',(0.,1.,0.));
#52024=DIRECTION('center_axis',(-0.364399348580519,0.,-0.931242779705751));
#52025=DIRECTION('ref_axis',(-0.931242779705751,0.,0.364399348580519));
#52026=DIRECTION('',(0.,1.,0.));
#52027=DIRECTION('center_axis',(0.624280230025758,0.,-0.781200482846105));
#52028=DIRECTION('ref_axis',(-0.781200482846105,0.,-0.624280230025758));
#52029=DIRECTION('center_axis',(0.988679578606276,0.,0.150042296859641));
#52030=DIRECTION('ref_axis',(0.150042296859641,0.,-0.988679578606276));
#52031=DIRECTION('',(0.,1.,0.));
#52032=DIRECTION('',(0.,1.,0.));
#52033=DIRECTION('center_axis',(0.364399348580517,0.,0.931242779705752));
#52034=DIRECTION('ref_axis',(0.931242779705752,0.,-0.364399348580517));
#52035=DIRECTION('',(0.,1.,0.));
#52036=DIRECTION('center_axis',(-0.624280230025758,0.,0.781200482846104));
#52037=DIRECTION('ref_axis',(0.781200482846104,0.,0.624280230025758));
#52038=DIRECTION('',(0.,1.,0.));
#52039=DIRECTION('center_axis',(-0.988679578606275,0.,-0.150042296859647));
#52040=DIRECTION('ref_axis',(-0.150042296859647,0.,0.988679578606275));
#52041=DIRECTION('',(0.,1.,0.));
#52042=DIRECTION('center_axis',(-0.364399348580519,0.,-0.931242779705751));
#52043=DIRECTION('ref_axis',(-0.931242779705751,0.,0.364399348580519));
#52044=DIRECTION('',(0.,1.,0.));
#52045=DIRECTION('center_axis',(0.624280230025758,0.,-0.781200482846105));
#52046=DIRECTION('ref_axis',(-0.781200482846105,0.,-0.624280230025758));
#52047=DIRECTION('center_axis',(0.988679578606276,0.,0.150042296859641));
#52048=DIRECTION('ref_axis',(0.150042296859641,0.,-0.988679578606276));
#52049=DIRECTION('',(0.,1.,0.));
#52050=DIRECTION('',(0.,1.,0.));
#52051=DIRECTION('center_axis',(0.364399348580517,0.,0.931242779705752));
#52052=DIRECTION('ref_axis',(0.931242779705752,0.,-0.364399348580517));
#52053=DIRECTION('',(0.,1.,0.));
#52054=DIRECTION('center_axis',(-0.624280230025758,0.,0.781200482846104));
#52055=DIRECTION('ref_axis',(0.781200482846104,0.,0.624280230025758));
#52056=DIRECTION('',(0.,1.,0.));
#52057=DIRECTION('center_axis',(-0.988679578606275,0.,-0.150042296859647));
#52058=DIRECTION('ref_axis',(-0.150042296859647,0.,0.988679578606275));
#52059=DIRECTION('',(0.,1.,0.));
#52060=DIRECTION('center_axis',(-0.364399348580519,0.,-0.931242779705751));
#52061=DIRECTION('ref_axis',(-0.931242779705751,0.,0.364399348580519));
#52062=DIRECTION('',(0.,1.,0.));
#52063=DIRECTION('center_axis',(0.624280230025758,0.,-0.781200482846105));
#52064=DIRECTION('ref_axis',(-0.781200482846105,0.,-0.624280230025758));
#52065=DIRECTION('center_axis',(0.988679578606276,0.,0.150042296859641));
#52066=DIRECTION('ref_axis',(0.150042296859641,0.,-0.988679578606276));
#52067=DIRECTION('',(0.,1.,0.));
#52068=DIRECTION('',(0.,1.,0.));
#52069=DIRECTION('center_axis',(0.364399348580517,0.,0.931242779705752));
#52070=DIRECTION('ref_axis',(0.931242779705752,0.,-0.364399348580517));
#52071=DIRECTION('',(0.,1.,0.));
#52072=DIRECTION('center_axis',(-0.624280230025758,0.,0.781200482846104));
#52073=DIRECTION('ref_axis',(0.781200482846104,0.,0.624280230025758));
#52074=DIRECTION('',(0.,1.,0.));
#52075=DIRECTION('center_axis',(-0.988679578606275,0.,-0.150042296859647));
#52076=DIRECTION('ref_axis',(-0.150042296859647,0.,0.988679578606275));
#52077=DIRECTION('',(0.,1.,0.));
#52078=DIRECTION('center_axis',(-0.364399348580519,0.,-0.931242779705751));
#52079=DIRECTION('ref_axis',(-0.931242779705751,0.,0.364399348580519));
#52080=DIRECTION('',(0.,1.,0.));
#52081=DIRECTION('center_axis',(0.624280230025758,0.,-0.781200482846105));
#52082=DIRECTION('ref_axis',(-0.781200482846105,0.,-0.624280230025758));
#52083=DIRECTION('center_axis',(0.988679578606276,0.,0.150042296859641));
#52084=DIRECTION('ref_axis',(0.150042296859641,0.,-0.988679578606276));
#52085=DIRECTION('',(0.,1.,0.));
#52086=DIRECTION('',(0.,1.,0.));
#52087=DIRECTION('center_axis',(0.364399348580517,0.,0.931242779705752));
#52088=DIRECTION('ref_axis',(0.931242779705752,0.,-0.364399348580517));
#52089=DIRECTION('',(0.,1.,0.));
#52090=DIRECTION('center_axis',(-0.624280230025758,0.,0.781200482846104));
#52091=DIRECTION('ref_axis',(0.781200482846104,0.,0.624280230025758));
#52092=DIRECTION('',(0.,1.,0.));
#52093=DIRECTION('center_axis',(-0.988679578606275,0.,-0.150042296859647));
#52094=DIRECTION('ref_axis',(-0.150042296859647,0.,0.988679578606275));
#52095=DIRECTION('',(0.,1.,0.));
#52096=DIRECTION('center_axis',(-0.364399348580519,0.,-0.931242779705751));
#52097=DIRECTION('ref_axis',(-0.931242779705751,0.,0.364399348580519));
#52098=DIRECTION('',(0.,1.,0.));
#52099=DIRECTION('center_axis',(0.624280230025758,0.,-0.781200482846105));
#52100=DIRECTION('ref_axis',(-0.781200482846105,0.,-0.624280230025758));
#52101=DIRECTION('center_axis',(0.988679578606276,0.,0.150042296859641));
#52102=DIRECTION('ref_axis',(0.150042296859641,0.,-0.988679578606276));
#52103=DIRECTION('',(0.,1.,0.));
#52104=DIRECTION('',(0.,1.,0.));
#52105=DIRECTION('center_axis',(0.364399348580517,0.,0.931242779705752));
#52106=DIRECTION('ref_axis',(0.931242779705752,0.,-0.364399348580517));
#52107=DIRECTION('',(0.,1.,0.));
#52108=DIRECTION('center_axis',(-0.624280230025758,0.,0.781200482846104));
#52109=DIRECTION('ref_axis',(0.781200482846104,0.,0.624280230025758));
#52110=DIRECTION('',(0.,1.,0.));
#52111=DIRECTION('center_axis',(-0.988679578606275,0.,-0.150042296859647));
#52112=DIRECTION('ref_axis',(-0.150042296859647,0.,0.988679578606275));
#52113=DIRECTION('',(0.,1.,0.));
#52114=DIRECTION('center_axis',(-0.364399348580519,0.,-0.931242779705751));
#52115=DIRECTION('ref_axis',(-0.931242779705751,0.,0.364399348580519));
#52116=DIRECTION('',(0.,1.,0.));
#52117=DIRECTION('center_axis',(0.624280230025758,0.,-0.781200482846105));
#52118=DIRECTION('ref_axis',(-0.781200482846105,0.,-0.624280230025758));
#52119=DIRECTION('center_axis',(0.988679578606276,0.,0.150042296859641));
#52120=DIRECTION('ref_axis',(0.150042296859641,0.,-0.988679578606276));
#52121=DIRECTION('',(0.,1.,0.));
#52122=DIRECTION('',(0.,1.,0.));
#52123=DIRECTION('center_axis',(0.364399348580517,0.,0.931242779705752));
#52124=DIRECTION('ref_axis',(0.931242779705752,0.,-0.364399348580517));
#52125=DIRECTION('',(0.,1.,0.));
#52126=DIRECTION('center_axis',(-0.624280230025758,0.,0.781200482846104));
#52127=DIRECTION('ref_axis',(0.781200482846104,0.,0.624280230025758));
#52128=DIRECTION('',(0.,1.,0.));
#52129=DIRECTION('center_axis',(-0.988679578606275,0.,-0.150042296859647));
#52130=DIRECTION('ref_axis',(-0.150042296859647,0.,0.988679578606275));
#52131=DIRECTION('',(0.,1.,0.));
#52132=DIRECTION('center_axis',(-0.364399348580519,0.,-0.931242779705751));
#52133=DIRECTION('ref_axis',(-0.931242779705751,0.,0.364399348580519));
#52134=DIRECTION('',(0.,1.,0.));
#52135=DIRECTION('center_axis',(0.624280230025758,0.,-0.781200482846105));
#52136=DIRECTION('ref_axis',(-0.781200482846105,0.,-0.624280230025758));
#52137=DIRECTION('center_axis',(0.988679578606276,0.,0.150042296859641));
#52138=DIRECTION('ref_axis',(0.150042296859641,0.,-0.988679578606276));
#52139=DIRECTION('',(0.,1.,0.));
#52140=DIRECTION('',(0.,1.,0.));
#52141=DIRECTION('center_axis',(0.364399348580517,0.,0.931242779705752));
#52142=DIRECTION('ref_axis',(0.931242779705752,0.,-0.364399348580517));
#52143=DIRECTION('',(0.,1.,0.));
#52144=DIRECTION('center_axis',(-0.624280230025758,0.,0.781200482846104));
#52145=DIRECTION('ref_axis',(0.781200482846104,0.,0.624280230025758));
#52146=DIRECTION('',(0.,1.,0.));
#52147=DIRECTION('center_axis',(-0.988679578606275,0.,-0.150042296859647));
#52148=DIRECTION('ref_axis',(-0.150042296859647,0.,0.988679578606275));
#52149=DIRECTION('',(0.,1.,0.));
#52150=DIRECTION('center_axis',(-0.364399348580519,0.,-0.931242779705751));
#52151=DIRECTION('ref_axis',(-0.931242779705751,0.,0.364399348580519));
#52152=DIRECTION('',(0.,1.,0.));
#52153=DIRECTION('center_axis',(0.624280230025758,0.,-0.781200482846105));
#52154=DIRECTION('ref_axis',(-0.781200482846105,0.,-0.624280230025758));
#52155=DIRECTION('center_axis',(0.988679578606276,0.,0.150042296859641));
#52156=DIRECTION('ref_axis',(0.150042296859641,0.,-0.988679578606276));
#52157=DIRECTION('',(0.,1.,0.));
#52158=DIRECTION('',(0.,1.,0.));
#52159=DIRECTION('center_axis',(0.364399348580517,0.,0.931242779705752));
#52160=DIRECTION('ref_axis',(0.931242779705752,0.,-0.364399348580517));
#52161=DIRECTION('',(0.,1.,0.));
#52162=DIRECTION('center_axis',(-0.624280230025758,0.,0.781200482846104));
#52163=DIRECTION('ref_axis',(0.781200482846104,0.,0.624280230025758));
#52164=DIRECTION('',(0.,1.,0.));
#52165=DIRECTION('center_axis',(-0.988679578606275,0.,-0.150042296859647));
#52166=DIRECTION('ref_axis',(-0.150042296859647,0.,0.988679578606275));
#52167=DIRECTION('',(0.,1.,0.));
#52168=DIRECTION('center_axis',(-0.364399348580519,0.,-0.931242779705751));
#52169=DIRECTION('ref_axis',(-0.931242779705751,0.,0.364399348580519));
#52170=DIRECTION('',(0.,1.,0.));
#52171=DIRECTION('center_axis',(0.624280230025758,0.,-0.781200482846105));
#52172=DIRECTION('ref_axis',(-0.781200482846105,0.,-0.624280230025758));
#52173=DIRECTION('center_axis',(0.988679578606276,0.,0.150042296859641));
#52174=DIRECTION('ref_axis',(0.150042296859641,0.,-0.988679578606276));
#52175=DIRECTION('',(0.,1.,0.));
#52176=DIRECTION('',(0.,1.,0.));
#52177=DIRECTION('center_axis',(0.364399348580517,0.,0.931242779705752));
#52178=DIRECTION('ref_axis',(0.931242779705752,0.,-0.364399348580517));
#52179=DIRECTION('',(0.,1.,0.));
#52180=DIRECTION('center_axis',(-0.624280230025758,0.,0.781200482846104));
#52181=DIRECTION('ref_axis',(0.781200482846104,0.,0.624280230025758));
#52182=DIRECTION('',(0.,1.,0.));
#52183=DIRECTION('center_axis',(-0.988679578606275,0.,-0.150042296859647));
#52184=DIRECTION('ref_axis',(-0.150042296859647,0.,0.988679578606275));
#52185=DIRECTION('',(0.,1.,0.));
#52186=DIRECTION('center_axis',(-0.364399348580519,0.,-0.931242779705751));
#52187=DIRECTION('ref_axis',(-0.931242779705751,0.,0.364399348580519));
#52188=DIRECTION('',(0.,1.,0.));
#52189=DIRECTION('center_axis',(0.624280230025758,0.,-0.781200482846105));
#52190=DIRECTION('ref_axis',(-0.781200482846105,0.,-0.624280230025758));
#52191=DIRECTION('center_axis',(0.988679578606276,0.,0.150042296859641));
#52192=DIRECTION('ref_axis',(0.150042296859641,0.,-0.988679578606276));
#52193=DIRECTION('',(0.,1.,0.));
#52194=DIRECTION('',(0.,1.,0.));
#52195=DIRECTION('center_axis',(0.364399348580517,0.,0.931242779705752));
#52196=DIRECTION('ref_axis',(0.931242779705752,0.,-0.364399348580517));
#52197=DIRECTION('',(0.,1.,0.));
#52198=DIRECTION('center_axis',(-0.624280230025758,0.,0.781200482846104));
#52199=DIRECTION('ref_axis',(0.781200482846104,0.,0.624280230025758));
#52200=DIRECTION('',(0.,1.,0.));
#52201=DIRECTION('center_axis',(-0.988679578606275,0.,-0.150042296859647));
#52202=DIRECTION('ref_axis',(-0.150042296859647,0.,0.988679578606275));
#52203=DIRECTION('',(0.,1.,0.));
#52204=DIRECTION('center_axis',(-0.364399348580519,0.,-0.931242779705751));
#52205=DIRECTION('ref_axis',(-0.931242779705751,0.,0.364399348580519));
#52206=DIRECTION('',(0.,1.,0.));
#52207=DIRECTION('center_axis',(0.624280230025758,0.,-0.781200482846105));
#52208=DIRECTION('ref_axis',(-0.781200482846105,0.,-0.624280230025758));
#52209=DIRECTION('center_axis',(0.988679578606276,0.,0.150042296859641));
#52210=DIRECTION('ref_axis',(0.150042296859641,0.,-0.988679578606276));
#52211=DIRECTION('',(0.,1.,0.));
#52212=DIRECTION('',(0.,1.,0.));
#52213=DIRECTION('center_axis',(0.364399348580517,0.,0.931242779705752));
#52214=DIRECTION('ref_axis',(0.931242779705752,0.,-0.364399348580517));
#52215=DIRECTION('',(0.,1.,0.));
#52216=DIRECTION('center_axis',(-0.624280230025758,0.,0.781200482846104));
#52217=DIRECTION('ref_axis',(0.781200482846104,0.,0.624280230025758));
#52218=DIRECTION('',(0.,1.,0.));
#52219=DIRECTION('center_axis',(-0.988679578606275,0.,-0.150042296859647));
#52220=DIRECTION('ref_axis',(-0.150042296859647,0.,0.988679578606275));
#52221=DIRECTION('',(0.,1.,0.));
#52222=DIRECTION('center_axis',(-0.364399348580519,0.,-0.931242779705751));
#52223=DIRECTION('ref_axis',(-0.931242779705751,0.,0.364399348580519));
#52224=DIRECTION('',(0.,1.,0.));
#52225=DIRECTION('center_axis',(0.624280230025758,0.,-0.781200482846105));
#52226=DIRECTION('ref_axis',(-0.781200482846105,0.,-0.624280230025758));
#52227=DIRECTION('center_axis',(0.988679578606276,0.,0.150042296859641));
#52228=DIRECTION('ref_axis',(0.150042296859641,0.,-0.988679578606276));
#52229=DIRECTION('',(0.,1.,0.));
#52230=DIRECTION('',(0.,1.,0.));
#52231=DIRECTION('center_axis',(0.364399348580517,0.,0.931242779705752));
#52232=DIRECTION('ref_axis',(0.931242779705752,0.,-0.364399348580517));
#52233=DIRECTION('',(0.,1.,0.));
#52234=DIRECTION('center_axis',(-0.624280230025758,0.,0.781200482846104));
#52235=DIRECTION('ref_axis',(0.781200482846104,0.,0.624280230025758));
#52236=DIRECTION('',(0.,1.,0.));
#52237=DIRECTION('center_axis',(-0.988679578606275,0.,-0.150042296859647));
#52238=DIRECTION('ref_axis',(-0.150042296859647,0.,0.988679578606275));
#52239=DIRECTION('',(0.,1.,0.));
#52240=DIRECTION('center_axis',(-0.364399348580519,0.,-0.931242779705751));
#52241=DIRECTION('ref_axis',(-0.931242779705751,0.,0.364399348580519));
#52242=DIRECTION('',(0.,1.,0.));
#52243=DIRECTION('center_axis',(0.624280230025758,0.,-0.781200482846105));
#52244=DIRECTION('ref_axis',(-0.781200482846105,0.,-0.624280230025758));
#52245=DIRECTION('center_axis',(0.988679578606276,0.,0.150042296859641));
#52246=DIRECTION('ref_axis',(0.150042296859641,0.,-0.988679578606276));
#52247=DIRECTION('',(0.,1.,0.));
#52248=DIRECTION('',(0.,1.,0.));
#52249=DIRECTION('center_axis',(0.364399348580517,0.,0.931242779705752));
#52250=DIRECTION('ref_axis',(0.931242779705752,0.,-0.364399348580517));
#52251=DIRECTION('',(0.,1.,0.));
#52252=DIRECTION('center_axis',(-0.624280230025758,0.,0.781200482846104));
#52253=DIRECTION('ref_axis',(0.781200482846104,0.,0.624280230025758));
#52254=DIRECTION('',(0.,1.,0.));
#52255=DIRECTION('center_axis',(-0.988679578606275,0.,-0.150042296859647));
#52256=DIRECTION('ref_axis',(-0.150042296859647,0.,0.988679578606275));
#52257=DIRECTION('',(0.,1.,0.));
#52258=DIRECTION('center_axis',(-0.364399348580519,0.,-0.931242779705751));
#52259=DIRECTION('ref_axis',(-0.931242779705751,0.,0.364399348580519));
#52260=DIRECTION('',(0.,1.,0.));
#52261=DIRECTION('center_axis',(0.624280230025758,0.,-0.781200482846105));
#52262=DIRECTION('ref_axis',(-0.781200482846105,0.,-0.624280230025758));
#52263=DIRECTION('center_axis',(0.988679578606276,0.,0.150042296859641));
#52264=DIRECTION('ref_axis',(0.150042296859641,0.,-0.988679578606276));
#52265=DIRECTION('',(0.,1.,0.));
#52266=DIRECTION('',(0.,1.,0.));
#52267=DIRECTION('center_axis',(0.364399348580517,0.,0.931242779705752));
#52268=DIRECTION('ref_axis',(0.931242779705752,0.,-0.364399348580517));
#52269=DIRECTION('',(0.,1.,0.));
#52270=DIRECTION('center_axis',(-0.624280230025758,0.,0.781200482846104));
#52271=DIRECTION('ref_axis',(0.781200482846104,0.,0.624280230025758));
#52272=DIRECTION('',(0.,1.,0.));
#52273=DIRECTION('center_axis',(-0.988679578606275,0.,-0.150042296859647));
#52274=DIRECTION('ref_axis',(-0.150042296859647,0.,0.988679578606275));
#52275=DIRECTION('',(0.,1.,0.));
#52276=DIRECTION('center_axis',(-0.364399348580519,0.,-0.931242779705751));
#52277=DIRECTION('ref_axis',(-0.931242779705751,0.,0.364399348580519));
#52278=DIRECTION('',(0.,1.,0.));
#52279=DIRECTION('center_axis',(0.624280230025758,0.,-0.781200482846105));
#52280=DIRECTION('ref_axis',(-0.781200482846105,0.,-0.624280230025758));
#52281=DIRECTION('center_axis',(0.988679578606276,0.,0.150042296859641));
#52282=DIRECTION('ref_axis',(0.150042296859641,0.,-0.988679578606276));
#52283=DIRECTION('',(0.,1.,0.));
#52284=DIRECTION('',(0.,1.,0.));
#52285=DIRECTION('center_axis',(0.364399348580517,0.,0.931242779705752));
#52286=DIRECTION('ref_axis',(0.931242779705752,0.,-0.364399348580517));
#52287=DIRECTION('',(0.,1.,0.));
#52288=DIRECTION('center_axis',(-0.624280230025758,0.,0.781200482846104));
#52289=DIRECTION('ref_axis',(0.781200482846104,0.,0.624280230025758));
#52290=DIRECTION('',(0.,1.,0.));
#52291=DIRECTION('center_axis',(-0.988679578606275,0.,-0.150042296859647));
#52292=DIRECTION('ref_axis',(-0.150042296859647,0.,0.988679578606275));
#52293=DIRECTION('',(0.,1.,0.));
#52294=DIRECTION('center_axis',(-0.364399348580519,0.,-0.931242779705751));
#52295=DIRECTION('ref_axis',(-0.931242779705751,0.,0.364399348580519));
#52296=DIRECTION('',(0.,1.,0.));
#52297=DIRECTION('center_axis',(0.624280230025758,0.,-0.781200482846105));
#52298=DIRECTION('ref_axis',(-0.781200482846105,0.,-0.624280230025758));
#52299=DIRECTION('center_axis',(0.988679578606276,0.,0.150042296859641));
#52300=DIRECTION('ref_axis',(0.150042296859641,0.,-0.988679578606276));
#52301=DIRECTION('',(0.,1.,0.));
#52302=DIRECTION('',(0.,1.,0.));
#52303=DIRECTION('center_axis',(0.364399348580517,0.,0.931242779705752));
#52304=DIRECTION('ref_axis',(0.931242779705752,0.,-0.364399348580517));
#52305=DIRECTION('',(0.,1.,0.));
#52306=DIRECTION('center_axis',(-0.624280230025758,0.,0.781200482846104));
#52307=DIRECTION('ref_axis',(0.781200482846104,0.,0.624280230025758));
#52308=DIRECTION('',(0.,1.,0.));
#52309=DIRECTION('center_axis',(-0.988679578606275,0.,-0.150042296859647));
#52310=DIRECTION('ref_axis',(-0.150042296859647,0.,0.988679578606275));
#52311=DIRECTION('',(0.,1.,0.));
#52312=DIRECTION('center_axis',(-0.364399348580519,0.,-0.931242779705751));
#52313=DIRECTION('ref_axis',(-0.931242779705751,0.,0.364399348580519));
#52314=DIRECTION('',(0.,1.,0.));
#52315=DIRECTION('center_axis',(0.624280230025758,0.,-0.781200482846105));
#52316=DIRECTION('ref_axis',(-0.781200482846105,0.,-0.624280230025758));
#52317=DIRECTION('center_axis',(0.988679578606276,0.,0.150042296859641));
#52318=DIRECTION('ref_axis',(0.150042296859641,0.,-0.988679578606276));
#52319=DIRECTION('',(0.,1.,0.));
#52320=DIRECTION('',(0.,1.,0.));
#52321=DIRECTION('center_axis',(0.364399348580517,0.,0.931242779705752));
#52322=DIRECTION('ref_axis',(0.931242779705752,0.,-0.364399348580517));
#52323=DIRECTION('',(0.,1.,0.));
#52324=DIRECTION('center_axis',(-0.624280230025758,0.,0.781200482846104));
#52325=DIRECTION('ref_axis',(0.781200482846104,0.,0.624280230025758));
#52326=DIRECTION('',(0.,1.,0.));
#52327=DIRECTION('center_axis',(-0.988679578606275,0.,-0.150042296859647));
#52328=DIRECTION('ref_axis',(-0.150042296859647,0.,0.988679578606275));
#52329=DIRECTION('',(0.,1.,0.));
#52330=DIRECTION('center_axis',(-0.364399348580519,0.,-0.931242779705751));
#52331=DIRECTION('ref_axis',(-0.931242779705751,0.,0.364399348580519));
#52332=DIRECTION('',(0.,1.,0.));
#52333=DIRECTION('center_axis',(0.624280230025758,0.,-0.781200482846105));
#52334=DIRECTION('ref_axis',(-0.781200482846105,0.,-0.624280230025758));
#52335=DIRECTION('center_axis',(0.988679578606276,0.,0.150042296859641));
#52336=DIRECTION('ref_axis',(0.150042296859641,0.,-0.988679578606276));
#52337=DIRECTION('',(0.,1.,0.));
#52338=DIRECTION('',(0.,1.,0.));
#52339=DIRECTION('center_axis',(0.364399348580517,0.,0.931242779705752));
#52340=DIRECTION('ref_axis',(0.931242779705752,0.,-0.364399348580517));
#52341=DIRECTION('',(0.,1.,0.));
#52342=DIRECTION('center_axis',(-0.624280230025758,0.,0.781200482846104));
#52343=DIRECTION('ref_axis',(0.781200482846104,0.,0.624280230025758));
#52344=DIRECTION('',(0.,1.,0.));
#52345=DIRECTION('center_axis',(-0.988679578606275,0.,-0.150042296859647));
#52346=DIRECTION('ref_axis',(-0.150042296859647,0.,0.988679578606275));
#52347=DIRECTION('',(0.,1.,0.));
#52348=DIRECTION('center_axis',(-0.364399348580519,0.,-0.931242779705751));
#52349=DIRECTION('ref_axis',(-0.931242779705751,0.,0.364399348580519));
#52350=DIRECTION('',(0.,1.,0.));
#52351=DIRECTION('center_axis',(0.624280230025758,0.,-0.781200482846105));
#52352=DIRECTION('ref_axis',(-0.781200482846105,0.,-0.624280230025758));
#52353=DIRECTION('center_axis',(0.988679578606276,0.,0.150042296859641));
#52354=DIRECTION('ref_axis',(0.150042296859641,0.,-0.988679578606276));
#52355=DIRECTION('',(0.,1.,0.));
#52356=DIRECTION('',(0.,1.,0.));
#52357=DIRECTION('center_axis',(0.364399348580517,0.,0.931242779705752));
#52358=DIRECTION('ref_axis',(0.931242779705752,0.,-0.364399348580517));
#52359=DIRECTION('',(0.,1.,0.));
#52360=DIRECTION('center_axis',(-0.624280230025758,0.,0.781200482846104));
#52361=DIRECTION('ref_axis',(0.781200482846104,0.,0.624280230025758));
#52362=DIRECTION('',(0.,1.,0.));
#52363=DIRECTION('center_axis',(-0.988679578606275,0.,-0.150042296859647));
#52364=DIRECTION('ref_axis',(-0.150042296859647,0.,0.988679578606275));
#52365=DIRECTION('',(0.,1.,0.));
#52366=DIRECTION('center_axis',(-0.364399348580519,0.,-0.931242779705751));
#52367=DIRECTION('ref_axis',(-0.931242779705751,0.,0.364399348580519));
#52368=DIRECTION('',(0.,1.,0.));
#52369=DIRECTION('center_axis',(0.624280230025758,0.,-0.781200482846105));
#52370=DIRECTION('ref_axis',(-0.781200482846105,0.,-0.624280230025758));
#52371=DIRECTION('center_axis',(0.988679578606276,0.,0.150042296859641));
#52372=DIRECTION('ref_axis',(0.150042296859641,0.,-0.988679578606276));
#52373=DIRECTION('',(0.,1.,0.));
#52374=DIRECTION('',(0.,1.,0.));
#52375=DIRECTION('center_axis',(0.364399348580517,0.,0.931242779705752));
#52376=DIRECTION('ref_axis',(0.931242779705752,0.,-0.364399348580517));
#52377=DIRECTION('',(0.,1.,0.));
#52378=DIRECTION('center_axis',(-0.624280230025758,0.,0.781200482846104));
#52379=DIRECTION('ref_axis',(0.781200482846104,0.,0.624280230025758));
#52380=DIRECTION('',(0.,1.,0.));
#52381=DIRECTION('center_axis',(-0.988679578606275,0.,-0.150042296859647));
#52382=DIRECTION('ref_axis',(-0.150042296859647,0.,0.988679578606275));
#52383=DIRECTION('',(0.,1.,0.));
#52384=DIRECTION('center_axis',(-0.364399348580519,0.,-0.931242779705751));
#52385=DIRECTION('ref_axis',(-0.931242779705751,0.,0.364399348580519));
#52386=DIRECTION('',(0.,1.,0.));
#52387=DIRECTION('center_axis',(0.624280230025758,0.,-0.781200482846105));
#52388=DIRECTION('ref_axis',(-0.781200482846105,0.,-0.624280230025758));
#52389=DIRECTION('center_axis',(0.988679578606276,0.,0.150042296859641));
#52390=DIRECTION('ref_axis',(0.150042296859641,0.,-0.988679578606276));
#52391=DIRECTION('',(0.,1.,0.));
#52392=DIRECTION('',(0.,1.,0.));
#52393=DIRECTION('center_axis',(0.364399348580517,0.,0.931242779705752));
#52394=DIRECTION('ref_axis',(0.931242779705752,0.,-0.364399348580517));
#52395=DIRECTION('',(0.,1.,0.));
#52396=DIRECTION('center_axis',(-0.624280230025758,0.,0.781200482846104));
#52397=DIRECTION('ref_axis',(0.781200482846104,0.,0.624280230025758));
#52398=DIRECTION('',(0.,1.,0.));
#52399=DIRECTION('center_axis',(-0.988679578606275,0.,-0.150042296859647));
#52400=DIRECTION('ref_axis',(-0.150042296859647,0.,0.988679578606275));
#52401=DIRECTION('',(0.,1.,0.));
#52402=DIRECTION('center_axis',(-0.364399348580519,0.,-0.931242779705751));
#52403=DIRECTION('ref_axis',(-0.931242779705751,0.,0.364399348580519));
#52404=DIRECTION('',(0.,1.,0.));
#52405=DIRECTION('center_axis',(0.624280230025758,0.,-0.781200482846105));
#52406=DIRECTION('ref_axis',(-0.781200482846105,0.,-0.624280230025758));
#52407=DIRECTION('center_axis',(0.988679578606276,0.,0.150042296859641));
#52408=DIRECTION('ref_axis',(0.150042296859641,0.,-0.988679578606276));
#52409=DIRECTION('',(0.,1.,0.));
#52410=DIRECTION('',(0.,1.,0.));
#52411=DIRECTION('center_axis',(0.364399348580517,0.,0.931242779705752));
#52412=DIRECTION('ref_axis',(0.931242779705752,0.,-0.364399348580517));
#52413=DIRECTION('',(0.,1.,0.));
#52414=DIRECTION('center_axis',(-0.624280230025758,0.,0.781200482846104));
#52415=DIRECTION('ref_axis',(0.781200482846104,0.,0.624280230025758));
#52416=DIRECTION('',(0.,1.,0.));
#52417=DIRECTION('center_axis',(-0.988679578606275,0.,-0.150042296859647));
#52418=DIRECTION('ref_axis',(-0.150042296859647,0.,0.988679578606275));
#52419=DIRECTION('',(0.,1.,0.));
#52420=DIRECTION('center_axis',(-0.364399348580519,0.,-0.931242779705751));
#52421=DIRECTION('ref_axis',(-0.931242779705751,0.,0.364399348580519));
#52422=DIRECTION('',(0.,1.,0.));
#52423=DIRECTION('center_axis',(0.624280230025758,0.,-0.781200482846105));
#52424=DIRECTION('ref_axis',(-0.781200482846105,0.,-0.624280230025758));
#52425=DIRECTION('center_axis',(0.988679578606276,0.,0.150042296859641));
#52426=DIRECTION('ref_axis',(0.150042296859641,0.,-0.988679578606276));
#52427=DIRECTION('',(0.,1.,0.));
#52428=DIRECTION('',(0.,1.,0.));
#52429=DIRECTION('center_axis',(0.364399348580517,0.,0.931242779705752));
#52430=DIRECTION('ref_axis',(0.931242779705752,0.,-0.364399348580517));
#52431=DIRECTION('',(0.,1.,0.));
#52432=DIRECTION('center_axis',(-0.624280230025758,0.,0.781200482846104));
#52433=DIRECTION('ref_axis',(0.781200482846104,0.,0.624280230025758));
#52434=DIRECTION('',(0.,1.,0.));
#52435=DIRECTION('center_axis',(-0.988679578606275,0.,-0.150042296859647));
#52436=DIRECTION('ref_axis',(-0.150042296859647,0.,0.988679578606275));
#52437=DIRECTION('',(0.,1.,0.));
#52438=DIRECTION('center_axis',(-0.364399348580519,0.,-0.931242779705751));
#52439=DIRECTION('ref_axis',(-0.931242779705751,0.,0.364399348580519));
#52440=DIRECTION('',(0.,1.,0.));
#52441=DIRECTION('center_axis',(0.624280230025758,0.,-0.781200482846105));
#52442=DIRECTION('ref_axis',(-0.781200482846105,0.,-0.624280230025758));
#58348=CARTESIAN_POINT('',(0.,0.,0.));
#58349=CARTESIAN_POINT('Origin',(0.,92.5000000000001,-77.5000000000001));
#58350=CARTESIAN_POINT('',(-59.9898979485574,92.6000000000002,-77.5000000000001));
#58351=CARTESIAN_POINT('Origin',(0.,92.6000000000002,-77.5000000000001));
#58352=CARTESIAN_POINT('',(-59.5,93.,-77.5000000000001));
#58353=CARTESIAN_POINT('Origin',(-59.5,92.5000000000001,-77.5000000000001));
#58354=CARTESIAN_POINT('Origin',(0.,93.,-77.5000000000001));
#58355=CARTESIAN_POINT('Origin',(0.,93.,-77.5000000000001));
#58356=CARTESIAN_POINT('',(-60.7737346662472,92.76,-77.5000000000001));
#58357=CARTESIAN_POINT('Origin',(0.,92.76,-77.5000000000001));
#58358=CARTESIAN_POINT('',(-61.9494897427832,91.8000000000001,-77.5000000000001));
#58359=CARTESIAN_POINT('Origin',(-61.9494897427832,93.,-77.5000000000001));
#58360=CARTESIAN_POINT('Origin',(0.,91.8000000000001,-77.5000000000001));
#58361=CARTESIAN_POINT('Origin',(0.,92.5000000000001,-77.5000000000001));
#58362=CARTESIAN_POINT('',(-59.5,93.8,-77.5000000000001));
#58363=CARTESIAN_POINT('Origin',(0.,93.8,-77.5000000000001));
#58364=CARTESIAN_POINT('Origin',(-59.5,92.5000000000001,-77.5000000000001));
#58365=CARTESIAN_POINT('Origin',(0.,93.,-77.5000000000001));
#58366=CARTESIAN_POINT('',(-61.9494897427832,91.0000000000001,-77.5000000000001));
#58367=CARTESIAN_POINT('Origin',(0.,91.0000000000001,-77.5000000000001));
#58368=CARTESIAN_POINT('Origin',(-61.9494897427832,93.,-77.5000000000001));
#58369=CARTESIAN_POINT('Origin',(80.,91.0000000000001,-155.));
#58370=CARTESIAN_POINT('',(-77.6424777960769,91.0000000000001,-57.5));
#58371=CARTESIAN_POINT('',(-79.2,91.,-57.5));
#58372=CARTESIAN_POINT('',(80.,91.0000000000001,-57.5));
#58373=CARTESIAN_POINT('',(-77.6424777960769,91.0000000000001,-97.5));
#58374=CARTESIAN_POINT('',(-77.6424777960769,91.0000000000001,-155.));
#58375=CARTESIAN_POINT('',(-79.2,91.0000000000001,-97.5));
#58376=CARTESIAN_POINT('',(80.,91.0000000000001,-97.5));
#58377=CARTESIAN_POINT('',(-79.2,91.0000000000001,-155.));
#58378=CARTESIAN_POINT('',(-79.2,91.0000000000001,-155.));
#58379=CARTESIAN_POINT('',(79.2,91.0000000000001,-155.));
#58380=CARTESIAN_POINT('',(80.,91.0000000000001,-155.));
#58381=CARTESIAN_POINT('',(79.2,91.0000000000001,-97.5000000000001));
#58382=CARTESIAN_POINT('',(79.2,91.0000000000001,-155.));
#58383=CARTESIAN_POINT('',(77.642477796077,91.0000000000001,-97.5000000000001));
#58384=CARTESIAN_POINT('',(80.,91.0000000000001,-97.5000000000001));
#58385=CARTESIAN_POINT('',(77.642477796077,91.0000000000001,-57.5000000000001));
#58386=CARTESIAN_POINT('',(77.6424777960769,91.0000000000001,-155.));
#58387=CARTESIAN_POINT('',(79.2,91.0000000000001,-57.5000000000001));
#58388=CARTESIAN_POINT('',(80.,91.0000000000001,-57.5000000000001));
#58389=CARTESIAN_POINT('',(79.2,91.0000000000001,0.));
#58390=CARTESIAN_POINT('',(79.2,91.0000000000001,-155.));
#58391=CARTESIAN_POINT('',(-79.2,91.0000000000001,0.));
#58392=CARTESIAN_POINT('',(80.,91.0000000000001,0.));
#58393=CARTESIAN_POINT('',(-79.2,91.0000000000001,-155.));
#58394=CARTESIAN_POINT('Origin',(80.,91.8000000000001,-155.));
#58395=CARTESIAN_POINT('',(-77.6424777960769,91.8000000000001,-57.5));
#58396=CARTESIAN_POINT('',(-77.6424777960769,91.8000000000001,-97.5));
#58397=CARTESIAN_POINT('',(-77.6424777960769,91.8000000000001,-57.5));
#58398=CARTESIAN_POINT('',(-79.2,91.8000000000001,-57.5));
#58399=CARTESIAN_POINT('',(-82.6424777960769,91.8000000000001,-57.5));
#58400=CARTESIAN_POINT('',(-79.2,91.8000000000001,0.));
#58401=CARTESIAN_POINT('',(-79.2,91.8000000000001,-155.));
#58402=CARTESIAN_POINT('',(79.2,91.8000000000001,0.));
#58403=CARTESIAN_POINT('',(80.,91.8000000000001,0.));
#58404=CARTESIAN_POINT('',(79.2,91.8000000000001,-57.5000000000001));
#58405=CARTESIAN_POINT('',(79.2,91.8000000000001,-155.));
#58406=CARTESIAN_POINT('',(77.642477796077,91.8000000000001,-57.5000000000001));
#58407=CARTESIAN_POINT('',(82.642477796077,91.8000000000001,-57.5000000000001));
#58408=CARTESIAN_POINT('',(77.642477796077,91.8000000000001,-97.5000000000001));
#58409=CARTESIAN_POINT('',(77.642477796077,91.8000000000001,-57.5000000000001));
#58410=CARTESIAN_POINT('',(79.2,91.8000000000001,-97.5000000000001));
#58411=CARTESIAN_POINT('',(82.642477796077,91.8000000000001,-97.5000000000001));
#58412=CARTESIAN_POINT('',(79.2,91.8000000000001,-155.));
#58413=CARTESIAN_POINT('',(79.2,91.8000000000001,-155.));
#58414=CARTESIAN_POINT('',(-79.2,91.8000000000001,-155.));
#58415=CARTESIAN_POINT('',(80.,91.8000000000001,-155.));
#58416=CARTESIAN_POINT('',(-79.2,91.8000000000001,-97.5));
#58417=CARTESIAN_POINT('',(-79.2,91.8000000000001,-155.));
#58418=CARTESIAN_POINT('',(-82.6424777960769,91.8000000000001,-97.5));
#58419=CARTESIAN_POINT('Origin',(80.8,90.2,0.));
#58420=CARTESIAN_POINT('',(79.2,91.0000000000001,0.));
#58421=CARTESIAN_POINT('',(-79.2,91.8000000000001,0.));
#58422=CARTESIAN_POINT('Origin',(-80.8,90.2,-155.));
#58423=CARTESIAN_POINT('',(-79.2,91.0000000000001,-155.));
#58424=CARTESIAN_POINT('',(79.2,91.8000000000001,-155.));
#58425=CARTESIAN_POINT('Origin',(-82.6424777960769,81.8000000000001,-57.5));
#58426=CARTESIAN_POINT('',(-79.2,91.8000000000001,-57.5));
#58427=CARTESIAN_POINT('',(-77.6424777960769,81.8000000000001,-57.5));
#58428=CARTESIAN_POINT('Origin',(-82.6424777960769,81.8000000000001,-97.5));
#58429=CARTESIAN_POINT('',(-79.2,91.0000000000001,-97.5));
#58430=CARTESIAN_POINT('',(-77.6424777960769,81.8000000000001,-97.5));
#58431=CARTESIAN_POINT('Origin',(-77.6424777960769,81.8000000000001,-57.5));
#58432=CARTESIAN_POINT('Origin',(82.642477796077,81.8000000000001,-57.5000000000001));
#58433=CARTESIAN_POINT('',(79.2,91.0000000000001,-57.5000000000001));
#58434=CARTESIAN_POINT('',(77.642477796077,81.8000000000001,-57.5000000000001));
#58435=CARTESIAN_POINT('Origin',(77.642477796077,81.8000000000001,-57.5000000000001));
#58436=CARTESIAN_POINT('',(77.642477796077,81.8000000000001,-97.5000000000001));
#58437=CARTESIAN_POINT('Origin',(82.642477796077,81.8000000000001,-97.5000000000001));
#58438=CARTESIAN_POINT('',(79.2,91.8000000000001,-97.5000000000001));
#58439=CARTESIAN_POINT('Origin',(79.2,90.2,-57.5000000000001));
#58440=CARTESIAN_POINT('',(80.8,90.2,-57.5000000000001));
#58441=CARTESIAN_POINT('',(80.0000000000001,90.2,-57.5000000000001));
#58442=CARTESIAN_POINT('',(80.8,90.2,-57.5000000000001));
#58443=CARTESIAN_POINT('Origin',(79.2,90.2,-57.5000000000001));
#58444=CARTESIAN_POINT('Origin',(79.2,90.2,-57.5000000000001));
#58445=CARTESIAN_POINT('Origin',(79.2,90.2,0.));
#58446=CARTESIAN_POINT('',(80.0000000000001,90.2,0.));
#58447=CARTESIAN_POINT('Origin',(79.2,90.2,0.));
#58448=CARTESIAN_POINT('',(80.8000000000001,90.2,0.));
#58449=CARTESIAN_POINT('',(80.8000000000001,90.2,0.));
#58450=CARTESIAN_POINT('Origin',(79.2,90.2,0.));
#58451=CARTESIAN_POINT('Origin',(79.2,90.2,28.7864498173497));
#58452=CARTESIAN_POINT('',(80.8000000000001,90.2,-155.));
#58453=CARTESIAN_POINT('Origin',(79.2,90.2,28.7864498173497));
#58454=CARTESIAN_POINT('',(80.0000000000001,90.2,-155.));
#58455=CARTESIAN_POINT('Origin',(79.2,90.2,-97.5000000000001));
#58456=CARTESIAN_POINT('',(80.0000000000001,90.2,-97.5000000000001));
#58457=CARTESIAN_POINT('Origin',(79.2,90.2,-97.5000000000001));
#58458=CARTESIAN_POINT('',(80.8,90.2,-97.5000000000001));
#58459=CARTESIAN_POINT('',(80.0000000000001,90.2,-97.5000000000001));
#58460=CARTESIAN_POINT('Origin',(79.2,90.2,-97.5000000000001));
#58461=CARTESIAN_POINT('Origin',(79.2,90.2,-155.));
#58462=CARTESIAN_POINT('',(80.0000000000001,90.2,-155.));
#58463=CARTESIAN_POINT('',(80.8,90.2,-155.));
#58464=CARTESIAN_POINT('',(80.0000000000001,90.2,-155.));
#58465=CARTESIAN_POINT('Origin',(79.2,90.2,-155.));
#58466=CARTESIAN_POINT('Origin',(79.2,90.2,-155.));
#58467=CARTESIAN_POINT('Origin',(79.2,90.2,-68.7135501826506));
#58468=CARTESIAN_POINT('',(80.8000000000001,90.2,-155.));
#58469=CARTESIAN_POINT('Origin',(79.2,90.2,-68.7135501826506));
#58470=CARTESIAN_POINT('',(80.0000000000001,90.2,-155.));
#58471=CARTESIAN_POINT('Origin',(80.8000000000001,3.1575222039231,-5.));
#58472=CARTESIAN_POINT('',(80.8000000000001,3.1575222039231,0.));
#58473=CARTESIAN_POINT('',(80.8000000000001,-1.84247779607691,-5.));
#58474=CARTESIAN_POINT('Origin',(80.8000000000001,3.1575222039231,-5.));
#58475=CARTESIAN_POINT('',(80.0000000000001,3.1575222039231,0.));
#58476=CARTESIAN_POINT('',(80.8000000000001,3.1575222039231,0.));
#58477=CARTESIAN_POINT('',(80.0000000000001,-1.84247779607691,-5.));
#58478=CARTESIAN_POINT('Origin',(80.0000000000001,3.1575222039231,-5.));
#58479=CARTESIAN_POINT('',(80.0000000000001,-1.84247779607691,-5.));
#58480=CARTESIAN_POINT('Origin',(70.8,88.6424777960769,-57.5000000000001));
#58481=CARTESIAN_POINT('',(80.0000000000001,88.642477796077,-97.5000000000001));
#58482=CARTESIAN_POINT('',(80.0000000000001,88.6424777960769,-57.5000000000001));
#58483=CARTESIAN_POINT('',(80.0000000000001,88.6424777960771,-155.));
#58484=CARTESIAN_POINT('',(80.8000000000001,88.6424777960769,-57.5000000000001));
#58485=CARTESIAN_POINT('',(70.8,88.6424777960769,-57.5000000000001));
#58486=CARTESIAN_POINT('',(80.8,88.642477796077,-97.5000000000001));
#58487=CARTESIAN_POINT('',(80.8,88.6424777960769,-57.5000000000001));
#58488=CARTESIAN_POINT('',(70.8,88.642477796077,-97.5000000000001));
#58489=CARTESIAN_POINT('Origin',(79.2000000000001,3.1575222039231,-150.));
#58490=CARTESIAN_POINT('',(80.8000000000001,-1.84247779607691,-150.));
#58491=CARTESIAN_POINT('',(80.8000000000001,3.1575222039231,-155.));
#58492=CARTESIAN_POINT('Origin',(80.8000000000001,3.1575222039231,-150.));
#58493=CARTESIAN_POINT('',(80.0000000000001,-1.84247779607691,-150.));
#58494=CARTESIAN_POINT('',(80.8000000000001,-1.84247779607691,-150.));
#58495=CARTESIAN_POINT('',(80.0000000000001,3.1575222039231,-155.));
#58496=CARTESIAN_POINT('Origin',(80.0000000000001,3.1575222039231,-150.));
#58497=CARTESIAN_POINT('',(80.0000000000001,3.1575222039231,-155.));
#58498=CARTESIAN_POINT('Origin',(80.8000000000001,-1.84247779607691,-155.));
#58499=CARTESIAN_POINT('',(80.0000000000001,-1.84247779607691,-155.));
#58500=CARTESIAN_POINT('',(80.8000000000001,-1.84247779607691,-155.));
#58501=CARTESIAN_POINT('Origin',(80.8000000000001,-1.84247779607691,-155.));
#58502=CARTESIAN_POINT('',(80.8000000000001,-1.84247779607691,-155.));
#58503=CARTESIAN_POINT('',(80.8,88.642477796077,-97.5000000000001));
#58504=CARTESIAN_POINT('',(80.8,88.6424777960769,-57.5000000000001));
#58505=CARTESIAN_POINT('',(80.8000000000001,-1.84247779607691,0.));
#58506=CARTESIAN_POINT('Origin',(70.8,88.642477796077,-97.5000000000001));
#58507=CARTESIAN_POINT('',(80.0000000000001,-1.84247779607691,-97.5000000000001));
#58508=CARTESIAN_POINT('Origin',(80.0000000000001,-1.84247779607691,-155.));
#58509=CARTESIAN_POINT('',(80.0000000000001,-1.84247779607691,-155.));
#58510=CARTESIAN_POINT('',(80.0000000000001,-1.84247779607691,0.));
#58511=CARTESIAN_POINT('',(80.0000000000001,-1.84247779607691,-57.5000000000001));
#58512=CARTESIAN_POINT('Origin',(79.2000000000001,91.8000000000001,-155.));
#58513=CARTESIAN_POINT('Origin',(79.2000000000001,90.2,0.));
#58514=CARTESIAN_POINT('Origin',(70.8,88.6424777960769,-57.5000000000001));
#58515=CARTESIAN_POINT('Origin',(-79.2,90.2,-97.5));
#58516=CARTESIAN_POINT('',(-80.8,90.2000000000001,-97.5));
#58517=CARTESIAN_POINT('',(-80.,90.2,-97.5));
#58518=CARTESIAN_POINT('',(-80.8,90.2,-97.5));
#58519=CARTESIAN_POINT('Origin',(-79.2,90.2,-97.5));
#58520=CARTESIAN_POINT('Origin',(-79.2,90.2,-97.5));
#58521=CARTESIAN_POINT('Origin',(-79.2,90.2,-155.));
#58522=CARTESIAN_POINT('',(-80.,90.2,-155.));
#58523=CARTESIAN_POINT('Origin',(-79.2,90.2,-155.));
#58524=CARTESIAN_POINT('',(-80.8,90.2,-155.));
#58525=CARTESIAN_POINT('',(-80.8,90.2,-155.));
#58526=CARTESIAN_POINT('Origin',(-79.2,90.2,-155.));
#58527=CARTESIAN_POINT('Origin',(-79.2,90.2,-183.78644981735));
#58528=CARTESIAN_POINT('',(-80.8,90.2,-155.));
#58529=CARTESIAN_POINT('Origin',(-79.2,90.2,-183.78644981735));
#58530=CARTESIAN_POINT('',(-80.,90.2,-155.));
#58531=CARTESIAN_POINT('Origin',(-79.2,90.2,-57.5));
#58532=CARTESIAN_POINT('',(-80.,90.2,-57.5));
#58533=CARTESIAN_POINT('Origin',(-79.2,90.2,-57.5));
#58534=CARTESIAN_POINT('',(-80.8,90.2,-57.5));
#58535=CARTESIAN_POINT('',(-80.,90.2,-57.5));
#58536=CARTESIAN_POINT('Origin',(-79.2,90.2,-57.5));
#58537=CARTESIAN_POINT('Origin',(-79.2,90.2,0.));
#58538=CARTESIAN_POINT('',(-80.,90.2,0.));
#58539=CARTESIAN_POINT('',(-80.8,90.2000000000001,0.));
#58540=CARTESIAN_POINT('',(-80.,90.2,0.));
#58541=CARTESIAN_POINT('Origin',(-79.2,90.2,0.));
#58542=CARTESIAN_POINT('Origin',(-79.2,90.2,0.));
#58543=CARTESIAN_POINT('Origin',(-79.2,90.2,-86.2864498173496));
#58544=CARTESIAN_POINT('',(-80.8,90.2,-155.));
#58545=CARTESIAN_POINT('Origin',(-79.2,90.2,-86.2864498173496));
#58546=CARTESIAN_POINT('',(-80.,90.2,-155.));
#58547=CARTESIAN_POINT('Origin',(79.2,3.15752220392312,-150.));
#58548=CARTESIAN_POINT('',(-80.,-1.84247779607691,-150.));
#58549=CARTESIAN_POINT('',(-80.,3.15752220392312,-155.));
#58550=CARTESIAN_POINT('Origin',(-80.,3.15752220392312,-150.));
#58551=CARTESIAN_POINT('',(-80.8,-1.84247779607691,-150.));
#58552=CARTESIAN_POINT('',(-80.,-1.84247779607691,-150.));
#58553=CARTESIAN_POINT('',(-80.8,3.15752220392312,-155.));
#58554=CARTESIAN_POINT('Origin',(-80.8,3.15752220392312,-150.));
#58555=CARTESIAN_POINT('',(79.2,3.15752220392312,-155.));
#58556=CARTESIAN_POINT('Origin',(-70.8,88.642477796077,-57.5));
#58557=CARTESIAN_POINT('',(-80.,88.642477796077,-97.5));
#58558=CARTESIAN_POINT('',(-80.8,88.642477796077,-97.5));
#58559=CARTESIAN_POINT('',(-70.8,88.642477796077,-97.5));
#58560=CARTESIAN_POINT('',(-80.8,88.642477796077,-57.5));
#58561=CARTESIAN_POINT('',(-80.8,88.642477796077,-57.5));
#58562=CARTESIAN_POINT('',(-80.,88.642477796077,-57.5));
#58563=CARTESIAN_POINT('',(-70.8,88.642477796077,-57.5));
#58564=CARTESIAN_POINT('',(-80.,88.642477796077,-155.));
#58565=CARTESIAN_POINT('Origin',(-80.,3.1575222039231,-5.));
#58566=CARTESIAN_POINT('',(-80.,3.1575222039231,0.));
#58567=CARTESIAN_POINT('',(-80.,-1.84247779607691,-5.));
#58568=CARTESIAN_POINT('Origin',(-80.,3.1575222039231,-5.));
#58569=CARTESIAN_POINT('',(-80.8,3.1575222039231,0.));
#58570=CARTESIAN_POINT('',(-80.,3.1575222039231,0.));
#58571=CARTESIAN_POINT('',(-80.8,-1.84247779607691,-5.));
#58572=CARTESIAN_POINT('Origin',(-80.8,3.1575222039231,-5.));
#58573=CARTESIAN_POINT('',(-80.8,-1.84247779607691,-5.));
#58574=CARTESIAN_POINT('Origin',(-80.,-1.84247779607691,-155.));
#58575=CARTESIAN_POINT('',(-80.,-1.84247779607691,-155.));
#58576=CARTESIAN_POINT('',(-80.8,-1.84247779607691,-155.));
#58577=CARTESIAN_POINT('Origin',(-80.8,-1.84247779607691,-155.));
#58578=CARTESIAN_POINT('',(-80.8,-1.84247779607691,0.));
#58579=CARTESIAN_POINT('',(-80.8,88.642477796077,-57.5));
#58580=CARTESIAN_POINT('',(-80.8,88.642477796077,-97.5));
#58581=CARTESIAN_POINT('',(-80.8,-1.84247779607691,-155.));
#58582=CARTESIAN_POINT('Origin',(-70.8,88.642477796077,-57.5));
#58583=CARTESIAN_POINT('',(-80.,-1.84247779607691,-57.5));
#58584=CARTESIAN_POINT('Origin',(-80.,-1.84247779607691,-155.));
#58585=CARTESIAN_POINT('',(-80.,-1.84247779607691,0.));
#58586=CARTESIAN_POINT('',(-80.,-1.84247779607691,-155.));
#58587=CARTESIAN_POINT('',(-80.,-1.84247779607691,-97.5));
#58588=CARTESIAN_POINT('Origin',(-79.2,91.8000000000001,0.));
#58589=CARTESIAN_POINT('Origin',(79.2,90.2,-155.));
#58590=CARTESIAN_POINT('Origin',(-70.8,88.642477796077,-97.5));
#58591=CARTESIAN_POINT('Origin',(0.,93.8,-77.5000000000001));
#58592=CARTESIAN_POINT('',(-21.8868869275414,93.8,-69.9335415751337));
#58593=CARTESIAN_POINT('',(-21.4537521251327,93.8,-72.7876136793868));
#58594=CARTESIAN_POINT('',(-21.8868869275414,93.8,-69.9335415751337));
#58595=CARTESIAN_POINT('',(-24.5751532752614,93.8,-68.8816112651563));
#58596=CARTESIAN_POINT('',(-24.5751532752614,93.8,-68.8816112651563));
#58597=CARTESIAN_POINT('',(-26.8302848205727,93.8,-70.683753059432));
#58598=CARTESIAN_POINT('',(-26.8302848205727,93.8,-70.683753059432));
#58599=CARTESIAN_POINT('',(-26.397150018164,93.8,-73.537825163685));
#58600=CARTESIAN_POINT('',(-26.397150018164,93.8,-73.537825163685));
#58601=CARTESIAN_POINT('',(-23.708883670444,93.8,-74.5897554736624));
#58602=CARTESIAN_POINT('',(-23.708883670444,93.8,-74.5897554736624));
#58603=CARTESIAN_POINT('',(-21.4537521251327,93.8,-72.7876136793868));
#58604=CARTESIAN_POINT('',(-14.9025660797482,93.8,-72.6665366894876));
#58605=CARTESIAN_POINT('',(-14.4694312773395,93.8,-75.5206087937407));
#58606=CARTESIAN_POINT('',(-14.9025660797482,93.8,-72.6665366894876));
#58607=CARTESIAN_POINT('',(-17.5908324274683,93.8,-71.6146063795101));
#58608=CARTESIAN_POINT('',(-17.5908324274683,93.8,-71.6146063795101));
#58609=CARTESIAN_POINT('',(-19.8459639727796,93.8,-73.4167481737858));
#58610=CARTESIAN_POINT('',(-19.8459639727796,93.8,-73.4167481737858));
#58611=CARTESIAN_POINT('',(-19.4128291703709,93.8,-76.2708202780389));
#58612=CARTESIAN_POINT('',(-19.4128291703709,93.8,-76.2708202780389));
#58613=CARTESIAN_POINT('',(-16.7245628226509,93.8,-77.3227505880163));
#58614=CARTESIAN_POINT('',(-16.7245628226509,93.8,-77.3227505880163));
#58615=CARTESIAN_POINT('',(-14.4694312773395,93.8,-75.5206087937407));
#58616=CARTESIAN_POINT('',(-7.91824523195512,93.8,-75.3995318038414));
#58617=CARTESIAN_POINT('',(-7.4851104295464,93.8,-78.2536039080945));
#58618=CARTESIAN_POINT('',(-7.91824523195512,93.8,-75.3995318038414));
#58619=CARTESIAN_POINT('',(-10.6065115796751,93.8,-74.347601493864));
#58620=CARTESIAN_POINT('',(-10.6065115796751,93.8,-74.347601493864));
#58621=CARTESIAN_POINT('',(-12.8616431249865,93.8,-76.1497432881397));
#58622=CARTESIAN_POINT('',(-12.8616431249865,93.8,-76.1497432881397));
#58623=CARTESIAN_POINT('',(-12.4285083225778,93.8,-79.0038153923928));
#58624=CARTESIAN_POINT('',(-12.4285083225778,93.8,-79.0038153923928));
#58625=CARTESIAN_POINT('',(-9.74024197485773,93.8,-80.0557457023702));
#58626=CARTESIAN_POINT('',(-9.74024197485773,93.8,-80.0557457023702));
#58627=CARTESIAN_POINT('',(-7.4851104295464,93.8,-78.2536039080945));
#58628=CARTESIAN_POINT('',(-0.933924384161986,93.8,-78.1325269181953));
#58629=CARTESIAN_POINT('',(-0.500789581753268,93.8,-80.9865990224485));
#58630=CARTESIAN_POINT('',(-0.933924384161986,93.8,-78.1325269181953));
#58631=CARTESIAN_POINT('',(-3.622190731882,93.8,-77.0805966082179));
#58632=CARTESIAN_POINT('',(-3.622190731882,93.8,-77.0805966082179));
#58633=CARTESIAN_POINT('',(-5.87732227719335,93.8,-78.8827384024936));
#58634=CARTESIAN_POINT('',(-5.87732227719335,93.8,-78.8827384024936));
#58635=CARTESIAN_POINT('',(-5.44418747478462,93.8,-81.7368105067467));
#58636=CARTESIAN_POINT('',(-5.44418747478462,93.8,-81.7368105067467));
#58637=CARTESIAN_POINT('',(-2.75592112706459,93.8,-82.7887408167241));
#58638=CARTESIAN_POINT('',(-2.75592112706459,93.8,-82.7887408167241));
#58639=CARTESIAN_POINT('',(-0.500789581753269,93.8,-80.9865990224485));
#58640=CARTESIAN_POINT('',(6.05039646363115,93.8,-80.8655220325492));
#58641=CARTESIAN_POINT('',(6.48353126603986,93.8,-83.7195941368023));
#58642=CARTESIAN_POINT('',(6.05039646363115,93.8,-80.8655220325492));
#58643=CARTESIAN_POINT('',(3.36213011591114,93.8,-79.8135917225718));
#58644=CARTESIAN_POINT('',(3.36213011591114,93.8,-79.8135917225718));
#58645=CARTESIAN_POINT('',(1.10699857059978,93.8,-81.6157335168475));
#58646=CARTESIAN_POINT('',(1.10699857059978,93.8,-81.6157335168475));
#58647=CARTESIAN_POINT('',(1.54013337300851,93.8,-84.4698056211006));
#58648=CARTESIAN_POINT('',(1.54013337300851,93.8,-84.4698056211006));
#58649=CARTESIAN_POINT('',(4.22839972072854,93.8,-85.521735931078));
#58650=CARTESIAN_POINT('',(4.22839972072854,93.8,-85.521735931078));
#58651=CARTESIAN_POINT('',(6.48353126603986,93.8,-83.7195941368023));
#58652=CARTESIAN_POINT('',(13.0347173114243,93.8,-83.5985171469031));
#58653=CARTESIAN_POINT('',(13.467852113833,93.8,-86.4525892511562));
#58654=CARTESIAN_POINT('',(13.0347173114243,93.8,-83.5985171469031));
#58655=CARTESIAN_POINT('',(10.3464509637043,93.8,-82.5465868369257));
#58656=CARTESIAN_POINT('',(10.3464509637043,93.8,-82.5465868369257));
#58657=CARTESIAN_POINT('',(8.09131941839291,93.8,-84.3487286312014));
#58658=CARTESIAN_POINT('',(8.09131941839291,93.8,-84.3487286312014));
#58659=CARTESIAN_POINT('',(8.52445422080164,93.8,-87.2028007354545));
#58660=CARTESIAN_POINT('',(8.52445422080164,93.8,-87.2028007354545));
#58661=CARTESIAN_POINT('',(11.2127205685217,93.8,-88.2547310454319));
#58662=CARTESIAN_POINT('',(11.2127205685217,93.8,-88.2547310454319));
#58663=CARTESIAN_POINT('',(13.467852113833,93.8,-86.4525892511562));
#58664=CARTESIAN_POINT('',(20.0190381592174,93.8,-86.331512261257));
#58665=CARTESIAN_POINT('',(20.4521729616261,93.8,-89.1855843655101));
#58666=CARTESIAN_POINT('',(20.0190381592174,93.8,-86.331512261257));
#58667=CARTESIAN_POINT('',(17.3307718114974,93.8,-85.2795819512796));
#58668=CARTESIAN_POINT('',(17.3307718114974,93.8,-85.2795819512796));
#58669=CARTESIAN_POINT('',(15.075640266186,93.8,-87.0817237455553));
#58670=CARTESIAN_POINT('',(15.075640266186,93.8,-87.0817237455553));
#58671=CARTESIAN_POINT('',(15.5087750685948,93.8,-89.9357958498083));
#58672=CARTESIAN_POINT('',(15.5087750685948,93.8,-89.9357958498083));
#58673=CARTESIAN_POINT('',(18.1970414163148,93.8,-90.9877261597858));
#58674=CARTESIAN_POINT('',(18.1970414163148,93.8,-90.9877261597858));
#58675=CARTESIAN_POINT('',(20.4521729616261,93.8,-89.1855843655101));
#58676=CARTESIAN_POINT('',(27.0033590070105,93.8,-89.0645073756109));
#58677=CARTESIAN_POINT('',(27.4364938094193,93.8,-91.918579479864));
#58678=CARTESIAN_POINT('',(27.0033590070105,93.8,-89.0645073756109));
#58679=CARTESIAN_POINT('',(24.3150926592905,93.8,-88.0125770656335));
#58680=CARTESIAN_POINT('',(24.3150926592905,93.8,-88.0125770656335));
#58681=CARTESIAN_POINT('',(22.0599611139792,93.8,-89.8147188599092));
#58682=CARTESIAN_POINT('',(22.0599611139792,93.8,-89.8147188599092));
#58683=CARTESIAN_POINT('',(22.4930959163879,93.8,-92.6687909641622));
#58684=CARTESIAN_POINT('',(22.4930959163879,93.8,-92.6687909641622));
#58685=CARTESIAN_POINT('',(25.1813622641079,93.8,-93.7207212741397));
#58686=CARTESIAN_POINT('',(25.1813622641079,93.8,-93.7207212741397));
#58687=CARTESIAN_POINT('',(27.4364938094193,93.8,-91.918579479864));
#58688=CARTESIAN_POINT('',(-16.0278833061956,93.8,-65.2514398499405));
#58689=CARTESIAN_POINT('',(-15.5947485037869,93.8,-68.1055119541936));
#58690=CARTESIAN_POINT('',(-16.0278833061956,93.8,-65.2514398499405));
#58691=CARTESIAN_POINT('',(-18.7161496539156,93.8,-64.1995095399631));
#58692=CARTESIAN_POINT('',(-18.7161496539156,93.8,-64.1995095399631));
#58693=CARTESIAN_POINT('',(-20.971281199227,93.8,-66.0016513342388));
#58694=CARTESIAN_POINT('',(-20.971281199227,93.8,-66.0016513342388));
#58695=CARTESIAN_POINT('',(-20.5381463968183,93.8,-68.8557234384919));
#58696=CARTESIAN_POINT('',(-20.5381463968183,93.8,-68.8557234384919));
#58697=CARTESIAN_POINT('',(-17.8498800490982,93.8,-69.9076537484693));
#58698=CARTESIAN_POINT('',(-17.8498800490982,93.8,-69.9076537484693));
#58699=CARTESIAN_POINT('',(-15.5947485037869,93.8,-68.1055119541936));
#58700=CARTESIAN_POINT('',(-23.0122041539888,93.8,-62.5184447355866));
#58701=CARTESIAN_POINT('',(-22.57906935158,93.8,-65.3725168398397));
#58702=CARTESIAN_POINT('',(-23.0122041539888,93.8,-62.5184447355866));
#58703=CARTESIAN_POINT('',(-25.7004705017088,93.8,-61.4665144256092));
#58704=CARTESIAN_POINT('',(-25.7004705017088,93.8,-61.4665144256092));
#58705=CARTESIAN_POINT('',(-27.9556020470201,93.8,-63.2686562198849));
#58706=CARTESIAN_POINT('',(-27.9556020470201,93.8,-63.2686562198849));
#58707=CARTESIAN_POINT('',(-27.5224672446114,93.8,-66.122728324138));
#58708=CARTESIAN_POINT('',(-27.5224672446114,93.8,-66.122728324138));
#58709=CARTESIAN_POINT('',(-24.8342008968914,93.8,-67.1746586341154));
#58710=CARTESIAN_POINT('',(-24.8342008968914,93.8,-67.1746586341154));
#58711=CARTESIAN_POINT('',(-22.57906935158,93.8,-65.3725168398397));
#58712=CARTESIAN_POINT('',(-29.9965250017819,93.8,-59.7854496212327));
#58713=CARTESIAN_POINT('',(-29.5633901993732,93.8,-62.6395217254858));
#58714=CARTESIAN_POINT('',(-29.9965250017819,93.8,-59.7854496212327));
#58715=CARTESIAN_POINT('',(-32.6847913495019,93.8,-58.7335193112553));
#58716=CARTESIAN_POINT('',(-32.6847913495019,93.8,-58.7335193112553));
#58717=CARTESIAN_POINT('',(-34.9399228948133,93.8,-60.535661105531));
#58718=CARTESIAN_POINT('',(-34.9399228948133,93.8,-60.535661105531));
#58719=CARTESIAN_POINT('',(-34.5067880924045,93.8,-63.3897332097841));
#58720=CARTESIAN_POINT('',(-34.5067880924045,93.8,-63.3897332097841));
#58721=CARTESIAN_POINT('',(-31.8185217446845,93.8,-64.4416635197615));
#58722=CARTESIAN_POINT('',(-31.8185217446845,93.8,-64.4416635197615));
#58723=CARTESIAN_POINT('',(-29.5633901993732,93.8,-62.6395217254858));
#58724=CARTESIAN_POINT('',(-36.980845849575,93.8,-57.0524545068788));
#58725=CARTESIAN_POINT('',(-36.5477110471663,93.8,-59.9065266111319));
#58726=CARTESIAN_POINT('',(-36.980845849575,93.8,-57.0524545068788));
#58727=CARTESIAN_POINT('',(-39.669112197295,93.8,-56.0005241969014));
#58728=CARTESIAN_POINT('',(-39.669112197295,93.8,-56.0005241969014));
#58729=CARTESIAN_POINT('',(-41.9242437426064,93.8,-57.8026659911771));
#58730=CARTESIAN_POINT('',(-41.9242437426064,93.8,-57.8026659911771));
#58731=CARTESIAN_POINT('',(-41.4911089401976,93.8,-60.6567380954302));
#58732=CARTESIAN_POINT('',(-41.4911089401976,93.8,-60.6567380954302));
#58733=CARTESIAN_POINT('',(-38.8028425924776,93.8,-61.7086684054076));
#58734=CARTESIAN_POINT('',(-38.8028425924776,93.8,-61.7086684054076));
#58735=CARTESIAN_POINT('',(-36.5477110471663,93.8,-59.9065266111319));
#58736=CARTESIAN_POINT('',(33.9876798548037,93.8,-91.7975024899648));
#58737=CARTESIAN_POINT('',(34.4208146572124,93.8,-94.6515745942179));
#58738=CARTESIAN_POINT('',(33.9876798548037,93.8,-91.7975024899648));
#58739=CARTESIAN_POINT('',(31.2994135070836,93.8,-90.7455721799874));
#58740=CARTESIAN_POINT('',(31.2994135070836,93.8,-90.7455721799874));
#58741=CARTESIAN_POINT('',(29.0442819617723,93.8,-92.5477139742631));
#58742=CARTESIAN_POINT('',(29.0442819617723,93.8,-92.5477139742631));
#58743=CARTESIAN_POINT('',(29.477416764181,93.8,-95.4017860785161));
#58744=CARTESIAN_POINT('',(29.477416764181,93.8,-95.4017860785161));
#58745=CARTESIAN_POINT('',(32.1656831119011,93.8,-96.4537163884935));
#58746=CARTESIAN_POINT('',(32.1656831119011,93.8,-96.4537163884935));
#58747=CARTESIAN_POINT('',(34.4208146572124,93.8,-94.6515745942179));
#58748=CARTESIAN_POINT('',(40.9720007025968,93.8,-94.5304976043187));
#58749=CARTESIAN_POINT('',(41.4051355050055,93.8,-97.3845697085718));
#58750=CARTESIAN_POINT('',(40.9720007025968,93.8,-94.5304976043187));
#58751=CARTESIAN_POINT('',(38.2837343548768,93.8,-93.4785672943413));
#58752=CARTESIAN_POINT('',(38.2837343548768,93.8,-93.4785672943413));
#58753=CARTESIAN_POINT('',(36.0286028095654,93.8,-95.280709088617));
#58754=CARTESIAN_POINT('',(36.0286028095654,93.8,-95.280709088617));
#58755=CARTESIAN_POINT('',(36.4617376119742,93.8,-98.13478119287));
#58756=CARTESIAN_POINT('',(36.4617376119742,93.8,-98.13478119287));
#58757=CARTESIAN_POINT('',(39.1500039596942,93.8,-99.1867115028474));
#58758=CARTESIAN_POINT('',(39.1500039596942,93.8,-99.1867115028474));
#58759=CARTESIAN_POINT('',(41.4051355050055,93.8,-97.3845697085718));
#58760=CARTESIAN_POINT('',(47.9563215503899,93.8,-97.2634927186726));
#58761=CARTESIAN_POINT('',(48.3894563527986,93.8,-100.117564822926));
#58762=CARTESIAN_POINT('',(47.9563215503899,93.8,-97.2634927186726));
#58763=CARTESIAN_POINT('',(45.2680552026699,93.8,-96.2115624086952));
#58764=CARTESIAN_POINT('',(45.2680552026699,93.8,-96.2115624086952));
#58765=CARTESIAN_POINT('',(43.0129236573585,93.8,-98.0137042029708));
#58766=CARTESIAN_POINT('',(43.0129236573585,93.8,-98.0137042029708));
#58767=CARTESIAN_POINT('',(43.4460584597673,93.8,-100.867776307224));
#58768=CARTESIAN_POINT('',(43.4460584597673,93.8,-100.867776307224));
#58769=CARTESIAN_POINT('',(46.1343248074873,93.8,-101.919706617201));
#58770=CARTESIAN_POINT('',(46.1343248074873,93.8,-101.919706617201));
#58771=CARTESIAN_POINT('',(48.3894563527986,93.8,-100.117564822926));
#58772=CARTESIAN_POINT('',(-43.9651666973681,93.8,-54.3194593925249));
#58773=CARTESIAN_POINT('',(-43.5320318949594,93.8,-57.1735314967781));
#58774=CARTESIAN_POINT('',(-43.9651666973681,93.8,-54.3194593925249));
#58775=CARTESIAN_POINT('',(-46.6534330450882,93.8,-53.2675290825475));
#58776=CARTESIAN_POINT('',(-46.6534330450882,93.8,-53.2675290825475));
#58777=CARTESIAN_POINT('',(-48.9085645903995,93.8,-55.0696708768232));
#58778=CARTESIAN_POINT('',(-48.9085645903995,93.8,-55.0696708768232));
#58779=CARTESIAN_POINT('',(-48.4754297879908,93.8,-57.9237429810763));
#58780=CARTESIAN_POINT('',(-48.4754297879908,93.8,-57.9237429810763));
#58781=CARTESIAN_POINT('',(-45.7871634402707,93.8,-58.9756732910537));
#58782=CARTESIAN_POINT('',(-45.7871634402707,93.8,-58.9756732910537));
#58783=CARTESIAN_POINT('',(-43.5320318949594,93.8,-57.1735314967781));
#58784=CARTESIAN_POINT('',(-41.7145322444734,93.8,-69.1496530716191));
#58785=CARTESIAN_POINT('',(-41.2813974420647,93.8,-72.0037251758721));
#58786=CARTESIAN_POINT('',(-41.7145322444734,93.8,-69.1496530716191));
#58787=CARTESIAN_POINT('',(-44.4027985921934,93.8,-68.0977227616416));
#58788=CARTESIAN_POINT('',(-44.4027985921934,93.8,-68.0977227616416));
#58789=CARTESIAN_POINT('',(-46.6579301375048,93.8,-69.8998645559173));
#58790=CARTESIAN_POINT('',(-46.6579301375048,93.8,-69.8998645559173));
#58791=CARTESIAN_POINT('',(-46.224795335096,93.8,-72.7539366601704));
#58792=CARTESIAN_POINT('',(-46.224795335096,93.8,-72.7539366601704));
#58793=CARTESIAN_POINT('',(-43.536528987376,93.8,-73.8058669701478));
#58794=CARTESIAN_POINT('',(-43.536528987376,93.8,-73.8058669701478));
#58795=CARTESIAN_POINT('',(-41.2813974420647,93.8,-72.0037251758721));
#58796=CARTESIAN_POINT('',(-34.7302113966803,93.8,-71.8826481859729));
#58797=CARTESIAN_POINT('',(-34.2970765942716,93.8,-74.7367202902261));
#58798=CARTESIAN_POINT('',(-34.7302113966803,93.8,-71.8826481859729));
#58799=CARTESIAN_POINT('',(-37.4184777444003,93.8,-70.8307178759955));
#58800=CARTESIAN_POINT('',(-37.4184777444003,93.8,-70.8307178759955));
#58801=CARTESIAN_POINT('',(-39.6736092897116,93.8,-72.6328596702712));
#58802=CARTESIAN_POINT('',(-39.6736092897116,93.8,-72.6328596702712));
#58803=CARTESIAN_POINT('',(-39.2404744873029,93.8,-75.4869317745243));
#58804=CARTESIAN_POINT('',(-39.2404744873029,93.8,-75.4869317745243));
#58805=CARTESIAN_POINT('',(-36.5522081395829,93.8,-76.5388620845017));
#58806=CARTESIAN_POINT('',(-36.5522081395829,93.8,-76.5388620845017));
#58807=CARTESIAN_POINT('',(-34.2970765942716,93.8,-74.7367202902261));
#58808=CARTESIAN_POINT('',(-27.7458905488871,93.8,-74.6156433003268));
#58809=CARTESIAN_POINT('',(-27.3127557464784,93.8,-77.4697154045799));
#58810=CARTESIAN_POINT('',(-27.7458905488871,93.8,-74.6156433003268));
#58811=CARTESIAN_POINT('',(-30.4341568966072,93.8,-73.5637129903494));
#58812=CARTESIAN_POINT('',(-30.4341568966072,93.8,-73.5637129903494));
#58813=CARTESIAN_POINT('',(-32.6892884419185,93.8,-75.3658547846251));
#58814=CARTESIAN_POINT('',(-32.6892884419185,93.8,-75.3658547846251));
#58815=CARTESIAN_POINT('',(-32.2561536395098,93.8,-78.2199268888782));
#58816=CARTESIAN_POINT('',(-32.2561536395098,93.8,-78.2199268888782));
#58817=CARTESIAN_POINT('',(-29.5678872917897,93.8,-79.2718571988556));
#58818=CARTESIAN_POINT('',(-29.5678872917897,93.8,-79.2718571988556));
#58819=CARTESIAN_POINT('',(-27.3127557464784,93.8,-77.4697154045799));
#58820=CARTESIAN_POINT('',(-20.761569701094,93.8,-77.3486384146807));
#58821=CARTESIAN_POINT('',(-20.3284348986853,93.8,-80.2027105189338));
#58822=CARTESIAN_POINT('',(-20.761569701094,93.8,-77.3486384146807));
#58823=CARTESIAN_POINT('',(-23.449836048814,93.8,-76.2967081047033));
#58824=CARTESIAN_POINT('',(-23.449836048814,93.8,-76.2967081047033));
#58825=CARTESIAN_POINT('',(-25.7049675941254,93.8,-78.098849898979));
#58826=CARTESIAN_POINT('',(-25.7049675941254,93.8,-78.098849898979));
#58827=CARTESIAN_POINT('',(-25.2718327917166,93.8,-80.9529220032321));
#58828=CARTESIAN_POINT('',(-25.2718327917166,93.8,-80.9529220032321));
#58829=CARTESIAN_POINT('',(-22.5835664439966,93.8,-82.0048523132095));
#58830=CARTESIAN_POINT('',(-22.5835664439966,93.8,-82.0048523132095));
#58831=CARTESIAN_POINT('',(-20.3284348986853,93.8,-80.2027105189338));
#58832=CARTESIAN_POINT('',(-13.7772488533009,93.8,-80.0816335290346));
#58833=CARTESIAN_POINT('',(-13.3441140508922,93.8,-82.9357056332877));
#58834=CARTESIAN_POINT('',(-13.7772488533009,93.8,-80.0816335290346));
#58835=CARTESIAN_POINT('',(-16.4655152010209,93.8,-79.0297032190572));
#58836=CARTESIAN_POINT('',(-16.4655152010209,93.8,-79.0297032190572));
#58837=CARTESIAN_POINT('',(-18.7206467463322,93.8,-80.8318450133329));
#58838=CARTESIAN_POINT('',(-18.7206467463322,93.8,-80.8318450133329));
#58839=CARTESIAN_POINT('',(-18.2875119439235,93.8,-83.685917117586));
#58840=CARTESIAN_POINT('',(-18.2875119439235,93.8,-83.685917117586));
#58841=CARTESIAN_POINT('',(-15.5992455962035,93.8,-84.7378474275634));
#58842=CARTESIAN_POINT('',(-15.5992455962035,93.8,-84.7378474275634));
#58843=CARTESIAN_POINT('',(-13.3441140508922,93.8,-82.9357056332877));
#58844=CARTESIAN_POINT('',(-6.79292800550775,93.8,-82.8146286433885));
#58845=CARTESIAN_POINT('',(-6.35979320309903,93.8,-85.6687007476416));
#58846=CARTESIAN_POINT('',(-6.79292800550775,93.8,-82.8146286433885));
#58847=CARTESIAN_POINT('',(-9.48119435322776,93.8,-81.7626983334111));
#58848=CARTESIAN_POINT('',(-9.48119435322776,93.8,-81.7626983334111));
#58849=CARTESIAN_POINT('',(-11.7363258985391,93.8,-83.5648401276868));
#58850=CARTESIAN_POINT('',(-11.7363258985391,93.8,-83.5648401276868));
#58851=CARTESIAN_POINT('',(-11.3031910961304,93.8,-86.4189122319399));
#58852=CARTESIAN_POINT('',(-11.3031910961304,93.8,-86.4189122319399));
#58853=CARTESIAN_POINT('',(-8.61492474841036,93.8,-87.4708425419173));
#58854=CARTESIAN_POINT('',(-8.61492474841036,93.8,-87.4708425419173));
#58855=CARTESIAN_POINT('',(-6.35979320309903,93.8,-85.6687007476416));
#58856=CARTESIAN_POINT('',(0.191392842285382,93.8,-85.5476237577424));
#58857=CARTESIAN_POINT('',(0.6245276446941,93.8,-88.4016958619955));
#58858=CARTESIAN_POINT('',(0.191392842285382,93.8,-85.5476237577424));
#58859=CARTESIAN_POINT('',(-2.49687350543463,93.8,-84.495693447765));
#58860=CARTESIAN_POINT('',(-2.49687350543463,93.8,-84.495693447765));
#58861=CARTESIAN_POINT('',(-4.75200505074598,93.8,-86.2978352420407));
#58862=CARTESIAN_POINT('',(-4.75200505074598,93.8,-86.2978352420407));
#58863=CARTESIAN_POINT('',(-4.31887024833725,93.8,-89.1519073462937));
#58864=CARTESIAN_POINT('',(-4.31887024833725,93.8,-89.1519073462937));
#58865=CARTESIAN_POINT('',(-1.63060390061722,93.8,-90.2038376562712));
#58866=CARTESIAN_POINT('',(-1.63060390061722,93.8,-90.2038376562712));
#58867=CARTESIAN_POINT('',(0.6245276446941,93.8,-88.4016958619955));
#58868=CARTESIAN_POINT('',(7.17571369007852,93.8,-88.2806188720963));
#58869=CARTESIAN_POINT('',(7.60884849248723,93.8,-91.1346909763494));
#58870=CARTESIAN_POINT('',(7.17571369007852,93.8,-88.2806188720963));
#58871=CARTESIAN_POINT('',(4.4874473423585,93.8,-87.2286885621189));
#58872=CARTESIAN_POINT('',(4.4874473423585,93.8,-87.2286885621189));
#58873=CARTESIAN_POINT('',(2.23231579704715,93.8,-89.0308303563946));
#58874=CARTESIAN_POINT('',(2.23231579704715,93.8,-89.0308303563946));
#58875=CARTESIAN_POINT('',(2.66545059945588,93.8,-91.8849024606476));
#58876=CARTESIAN_POINT('',(2.66545059945588,93.8,-91.8849024606476));
#58877=CARTESIAN_POINT('',(5.35371694717591,93.8,-92.936832770625));
#58878=CARTESIAN_POINT('',(5.35371694717591,93.8,-92.936832770625));
#58879=CARTESIAN_POINT('',(7.60884849248723,93.8,-91.1346909763494));
#58880=CARTESIAN_POINT('',(42.0973179290442,93.8,-101.945594443866));
#58881=CARTESIAN_POINT('',(42.5304527314529,93.8,-104.799666548119));
#58882=CARTESIAN_POINT('',(42.0973179290442,93.8,-101.945594443866));
#58883=CARTESIAN_POINT('',(39.4090515813242,93.8,-100.893664133888));
#58884=CARTESIAN_POINT('',(39.4090515813242,93.8,-100.893664133888));
#58885=CARTESIAN_POINT('',(37.1539200360128,93.8,-102.695805928164));
#58886=CARTESIAN_POINT('',(37.1539200360128,93.8,-102.695805928164));
#58887=CARTESIAN_POINT('',(37.5870548384215,93.8,-105.549878032417));
#58888=CARTESIAN_POINT('',(37.5870548384215,93.8,-105.549878032417));
#58889=CARTESIAN_POINT('',(40.2753211861416,93.8,-106.601808342394));
#58890=CARTESIAN_POINT('',(40.2753211861416,93.8,-106.601808342394));
#58891=CARTESIAN_POINT('',(42.5304527314529,93.8,-104.799666548119));
#58892=CARTESIAN_POINT('',(-42.8398494709208,93.8,-61.734556232072));
#58893=CARTESIAN_POINT('',(-42.4067146685121,93.8,-64.5886283363251));
#58894=CARTESIAN_POINT('',(-42.8398494709208,93.8,-61.734556232072));
#58895=CARTESIAN_POINT('',(-45.5281158186408,93.8,-60.6826259220946));
#58896=CARTESIAN_POINT('',(-45.5281158186408,93.8,-60.6826259220946));
#58897=CARTESIAN_POINT('',(-47.7832473639521,93.8,-62.4847677163703));
#58898=CARTESIAN_POINT('',(-47.7832473639521,93.8,-62.4847677163703));
#58899=CARTESIAN_POINT('',(-47.3501125615434,93.8,-65.3388398206233));
#58900=CARTESIAN_POINT('',(-47.3501125615434,93.8,-65.3388398206233));
#58901=CARTESIAN_POINT('',(-44.6618462138234,93.8,-66.3907701306008));
#58902=CARTESIAN_POINT('',(-44.6618462138234,93.8,-66.3907701306008));
#58903=CARTESIAN_POINT('',(-42.4067146685121,93.8,-64.5886283363251));
#58904=CARTESIAN_POINT('',(-35.8555286231276,93.8,-64.4675513464259));
#58905=CARTESIAN_POINT('',(-35.4223938207189,93.8,-67.321623450679));
#58906=CARTESIAN_POINT('',(-35.8555286231276,93.8,-64.4675513464259));
#58907=CARTESIAN_POINT('',(-38.5437949708476,93.8,-63.4156210364485));
#58908=CARTESIAN_POINT('',(-38.5437949708476,93.8,-63.4156210364485));
#58909=CARTESIAN_POINT('',(-40.798926516159,93.8,-65.2177628307242));
#58910=CARTESIAN_POINT('',(-40.798926516159,93.8,-65.2177628307242));
#58911=CARTESIAN_POINT('',(-40.3657917137503,93.8,-68.0718349349772));
#58912=CARTESIAN_POINT('',(-40.3657917137503,93.8,-68.0718349349772));
#58913=CARTESIAN_POINT('',(-37.6775253660303,93.8,-69.1237652449547));
#58914=CARTESIAN_POINT('',(-37.6775253660303,93.8,-69.1237652449547));
#58915=CARTESIAN_POINT('',(-35.4223938207189,93.8,-67.321623450679));
#58916=CARTESIAN_POINT('',(-28.8712077753345,93.8,-67.2005464607798));
#58917=CARTESIAN_POINT('',(-28.4380729729258,93.8,-70.0546185650329));
#58918=CARTESIAN_POINT('',(-28.8712077753345,93.8,-67.2005464607798));
#58919=CARTESIAN_POINT('',(-31.5594741230545,93.8,-66.1486161508024));
#58920=CARTESIAN_POINT('',(-31.5594741230545,93.8,-66.1486161508024));
#58921=CARTESIAN_POINT('',(-33.8146056683659,93.8,-67.9507579450781));
#58922=CARTESIAN_POINT('',(-33.8146056683659,93.8,-67.9507579450781));
#58923=CARTESIAN_POINT('',(-33.3814708659571,93.8,-70.8048300493311));
#58924=CARTESIAN_POINT('',(-33.3814708659571,93.8,-70.8048300493311));
#58925=CARTESIAN_POINT('',(-30.6932045182371,93.8,-71.8567603593086));
#58926=CARTESIAN_POINT('',(-30.6932045182371,93.8,-71.8567603593086));
#58927=CARTESIAN_POINT('',(-28.4380729729258,93.8,-70.0546185650329));
#58928=CARTESIAN_POINT('',(35.112997081251,93.8,-99.2125993295118));
#58929=CARTESIAN_POINT('',(35.5461318836598,93.8,-102.066671433765));
#58930=CARTESIAN_POINT('',(35.112997081251,93.8,-99.2125993295118));
#58931=CARTESIAN_POINT('',(32.424730733531,93.8,-98.1606690195344));
#58932=CARTESIAN_POINT('',(32.424730733531,93.8,-98.1606690195344));
#58933=CARTESIAN_POINT('',(30.1695991882197,93.8,-99.9628108138101));
#58934=CARTESIAN_POINT('',(30.1695991882197,93.8,-99.9628108138101));
#58935=CARTESIAN_POINT('',(30.6027339906284,93.8,-102.816882918063));
#58936=CARTESIAN_POINT('',(30.6027339906284,93.8,-102.816882918063));
#58937=CARTESIAN_POINT('',(33.2910003383484,93.8,-103.868813228041));
#58938=CARTESIAN_POINT('',(33.2910003383484,93.8,-103.868813228041));
#58939=CARTESIAN_POINT('',(35.5461318836598,93.8,-102.066671433765));
#58940=CARTESIAN_POINT('',(28.1286762334579,93.8,-96.479604215158));
#58941=CARTESIAN_POINT('',(28.5618110358666,93.8,-99.333676319411));
#58942=CARTESIAN_POINT('',(28.1286762334579,93.8,-96.479604215158));
#58943=CARTESIAN_POINT('',(25.4404098857379,93.8,-95.4276739051805));
#58944=CARTESIAN_POINT('',(25.4404098857379,93.8,-95.4276739051805));
#58945=CARTESIAN_POINT('',(23.1852783404265,93.8,-97.2298156994562));
#58946=CARTESIAN_POINT('',(23.1852783404265,93.8,-97.2298156994562));
#58947=CARTESIAN_POINT('',(23.6184131428353,93.8,-100.083887803709));
#58948=CARTESIAN_POINT('',(23.6184131428353,93.8,-100.083887803709));
#58949=CARTESIAN_POINT('',(26.3066794905553,93.8,-101.135818113687));
#58950=CARTESIAN_POINT('',(26.3066794905553,93.8,-101.135818113687));
#58951=CARTESIAN_POINT('',(28.5618110358666,93.8,-99.3336763194111));
#58952=CARTESIAN_POINT('',(21.1443553856648,93.8,-93.7466091008041));
#58953=CARTESIAN_POINT('',(21.5774901880735,93.8,-96.6006812050572));
#58954=CARTESIAN_POINT('',(21.1443553856648,93.8,-93.7466091008041));
#58955=CARTESIAN_POINT('',(18.4560890379448,93.8,-92.6946787908267));
#58956=CARTESIAN_POINT('',(18.4560890379448,93.8,-92.6946787908267));
#58957=CARTESIAN_POINT('',(16.2009574926334,93.8,-94.4968205851023));
#58958=CARTESIAN_POINT('',(16.2009574926334,93.8,-94.4968205851023));
#58959=CARTESIAN_POINT('',(16.6340922950421,93.8,-97.3508926893554));
#58960=CARTESIAN_POINT('',(16.6340922950421,93.8,-97.3508926893554));
#58961=CARTESIAN_POINT('',(19.3223586427622,93.8,-98.4028229993328));
#58962=CARTESIAN_POINT('',(19.3223586427622,93.8,-98.4028229993328));
#58963=CARTESIAN_POINT('',(21.5774901880735,93.8,-96.6006812050572));
#58964=CARTESIAN_POINT('',(14.1600345378716,93.8,-91.0136139864502));
#58965=CARTESIAN_POINT('',(14.5931693402804,93.8,-93.8676860907033));
#58966=CARTESIAN_POINT('',(14.1600345378716,93.8,-91.0136139864502));
#58967=CARTESIAN_POINT('',(11.4717681901516,93.8,-89.9616836764728));
#58968=CARTESIAN_POINT('',(11.4717681901516,93.8,-89.9616836764728));
#58969=CARTESIAN_POINT('',(9.21663664484028,93.8,-91.7638254707484));
#58970=CARTESIAN_POINT('',(9.21663664484028,93.8,-91.7638254707484));
#58971=CARTESIAN_POINT('',(9.64977144724901,93.8,-94.6178975750015));
#58972=CARTESIAN_POINT('',(9.64977144724901,93.8,-94.6178975750015));
#58973=CARTESIAN_POINT('',(12.338037794969,93.8,-95.6698278849789));
#58974=CARTESIAN_POINT('',(12.338037794969,93.8,-95.6698278849789));
#58975=CARTESIAN_POINT('',(14.5931693402804,93.8,-93.8676860907033));
#58976=CARTESIAN_POINT('',(38.721366249702,93.8,-79.7003039252246));
#58977=CARTESIAN_POINT('',(39.1545010521108,93.8,-82.5543760294777));
#58978=CARTESIAN_POINT('',(38.721366249702,93.8,-79.7003039252246));
#58979=CARTESIAN_POINT('',(36.033099901982,93.8,-78.6483736152472));
#58980=CARTESIAN_POINT('',(36.033099901982,93.8,-78.6483736152472));
#58981=CARTESIAN_POINT('',(33.7779683566707,93.8,-80.4505154095229));
#58982=CARTESIAN_POINT('',(33.7779683566707,93.8,-80.4505154095229));
#58983=CARTESIAN_POINT('',(34.2111031590794,93.8,-83.3045875137759));
#58984=CARTESIAN_POINT('',(34.2111031590794,93.8,-83.3045875137759));
#58985=CARTESIAN_POINT('',(36.8993695067994,93.8,-84.3565178237533));
#58986=CARTESIAN_POINT('',(36.8993695067994,93.8,-84.3565178237533));
#58987=CARTESIAN_POINT('',(39.1545010521108,93.8,-82.5543760294777));
#58988=CARTESIAN_POINT('',(45.7056870974952,93.8,-82.4332990395785));
#58989=CARTESIAN_POINT('',(46.1388218999039,93.8,-85.2873711438316));
#58990=CARTESIAN_POINT('',(45.7056870974952,93.8,-82.4332990395785));
#58991=CARTESIAN_POINT('',(43.0174207497752,93.8,-81.381368729601));
#58992=CARTESIAN_POINT('',(43.0174207497752,93.8,-81.381368729601));
#58993=CARTESIAN_POINT('',(40.7622892044638,93.8,-83.1835105238767));
#58994=CARTESIAN_POINT('',(40.7622892044638,93.8,-83.1835105238767));
#58995=CARTESIAN_POINT('',(41.1954240068725,93.8,-86.0375826281298));
#58996=CARTESIAN_POINT('',(41.1954240068725,93.8,-86.0375826281298));
#58997=CARTESIAN_POINT('',(43.8836903545926,93.8,-87.0895129381072));
#58998=CARTESIAN_POINT('',(43.8836903545926,93.8,-87.0895129381072));
#58999=CARTESIAN_POINT('',(46.1388218999039,93.8,-85.2873711438316));
#59000=CARTESIAN_POINT('',(52.6900079452883,93.8,-85.1662941539323));
#59001=CARTESIAN_POINT('',(53.123142747697,93.8,-88.0203662581854));
#59002=CARTESIAN_POINT('',(52.6900079452883,93.8,-85.1662941539323));
#59003=CARTESIAN_POINT('',(50.0017415975683,93.8,-84.1143638439549));
#59004=CARTESIAN_POINT('',(50.0017415975683,93.8,-84.1143638439549));
#59005=CARTESIAN_POINT('',(47.7466100522569,93.8,-85.9165056382306));
#59006=CARTESIAN_POINT('',(47.7466100522569,93.8,-85.9165056382306));
#59007=CARTESIAN_POINT('',(48.1797448546657,93.8,-88.7705777424837));
#59008=CARTESIAN_POINT('',(48.1797448546657,93.8,-88.7705777424837));
#59009=CARTESIAN_POINT('',(50.8680112023857,93.8,-89.8225080524611));
#59010=CARTESIAN_POINT('',(50.8680112023857,93.8,-89.8225080524611));
#59011=CARTESIAN_POINT('',(53.123142747697,93.8,-88.0203662581854));
#59012=CARTESIAN_POINT('',(-39.2314803024698,93.8,-42.2222608277847));
#59013=CARTESIAN_POINT('',(-38.798345500061,93.8,-45.0763329320378));
#59014=CARTESIAN_POINT('',(-39.2314803024698,93.8,-42.2222608277847));
#59015=CARTESIAN_POINT('',(-41.9197466501898,93.8,-41.1703305178073));
#59016=CARTESIAN_POINT('',(-41.9197466501898,93.8,-41.1703305178073));
#59017=CARTESIAN_POINT('',(-44.1748781955011,93.8,-42.972472312083));
#59018=CARTESIAN_POINT('',(-44.1748781955011,93.8,-42.972472312083));
#59019=CARTESIAN_POINT('',(-43.7417433930924,93.8,-45.8265444163361));
#59020=CARTESIAN_POINT('',(-43.7417433930924,93.8,-45.8265444163361));
#59021=CARTESIAN_POINT('',(-41.0534770453724,93.8,-46.8784747263135));
#59022=CARTESIAN_POINT('',(-41.0534770453724,93.8,-46.8784747263135));
#59023=CARTESIAN_POINT('',(-38.798345500061,93.8,-45.0763329320378));
#59024=CARTESIAN_POINT('',(31.7370454019089,93.8,-76.9673088108707));
#59025=CARTESIAN_POINT('',(32.1701802043176,93.8,-79.8213809151238));
#59026=CARTESIAN_POINT('',(31.7370454019089,93.8,-76.9673088108707));
#59027=CARTESIAN_POINT('',(29.0487790541889,93.8,-75.9153785008933));
#59028=CARTESIAN_POINT('',(29.0487790541889,93.8,-75.9153785008933));
#59029=CARTESIAN_POINT('',(26.7936475088776,93.8,-77.717520295169));
#59030=CARTESIAN_POINT('',(26.7936475088776,93.8,-77.717520295169));
#59031=CARTESIAN_POINT('',(27.2267823112863,93.8,-80.571592399422));
#59032=CARTESIAN_POINT('',(27.2267823112863,93.8,-80.571592399422));
#59033=CARTESIAN_POINT('',(29.9150486590063,93.8,-81.6235227093995));
#59034=CARTESIAN_POINT('',(29.9150486590063,93.8,-81.6235227093995));
#59035=CARTESIAN_POINT('',(32.1701802043176,93.8,-79.8213809151238));
#59036=CARTESIAN_POINT('',(24.7527245541158,93.8,-74.2343136965168));
#59037=CARTESIAN_POINT('',(25.1858593565245,93.8,-77.0883858007699));
#59038=CARTESIAN_POINT('',(24.7527245541158,93.8,-74.2343136965168));
#59039=CARTESIAN_POINT('',(22.0644582063958,93.8,-73.1823833865394));
#59040=CARTESIAN_POINT('',(22.0644582063958,93.8,-73.1823833865394));
#59041=CARTESIAN_POINT('',(19.8093266610844,93.8,-74.9845251808151));
#59042=CARTESIAN_POINT('',(19.8093266610844,93.8,-74.9845251808151));
#59043=CARTESIAN_POINT('',(20.2424614634932,93.8,-77.8385972850681));
#59044=CARTESIAN_POINT('',(20.2424614634932,93.8,-77.8385972850681));
#59045=CARTESIAN_POINT('',(22.9307278112132,93.8,-78.8905275950456));
#59046=CARTESIAN_POINT('',(22.9307278112132,93.8,-78.8905275950456));
#59047=CARTESIAN_POINT('',(25.1858593565245,93.8,-77.0883858007699));
#59048=CARTESIAN_POINT('',(17.7684037063227,93.8,-71.5013185821629));
#59049=CARTESIAN_POINT('',(18.2015385087314,93.8,-74.355390686416));
#59050=CARTESIAN_POINT('',(17.7684037063227,93.8,-71.5013185821629));
#59051=CARTESIAN_POINT('',(15.0801373586026,93.8,-70.4493882721855));
#59052=CARTESIAN_POINT('',(15.0801373586026,93.8,-70.4493882721855));
#59053=CARTESIAN_POINT('',(12.8250058132913,93.8,-72.2515300664612));
#59054=CARTESIAN_POINT('',(12.8250058132913,93.8,-72.2515300664612));
#59055=CARTESIAN_POINT('',(13.2581406157,93.8,-75.1056021707142));
#59056=CARTESIAN_POINT('',(13.2581406157,93.8,-75.1056021707142));
#59057=CARTESIAN_POINT('',(15.94640696342,93.8,-76.1575324806917));
#59058=CARTESIAN_POINT('',(15.94640696342,93.8,-76.1575324806917));
#59059=CARTESIAN_POINT('',(18.2015385087314,93.8,-74.355390686416));
#59060=CARTESIAN_POINT('',(10.7840828585295,93.8,-68.768323467809));
#59061=CARTESIAN_POINT('',(11.2172176609382,93.8,-71.6223955720621));
#59062=CARTESIAN_POINT('',(10.7840828585295,93.8,-68.768323467809));
#59063=CARTESIAN_POINT('',(8.09581651080951,93.8,-67.7163931578316));
#59064=CARTESIAN_POINT('',(8.09581651080951,93.8,-67.7163931578316));
#59065=CARTESIAN_POINT('',(5.84068496549816,93.8,-69.5185349521073));
#59066=CARTESIAN_POINT('',(5.84068496549816,93.8,-69.5185349521073));
#59067=CARTESIAN_POINT('',(6.27381976790689,93.8,-72.3726070563604));
#59068=CARTESIAN_POINT('',(6.27381976790689,93.8,-72.3726070563604));
#59069=CARTESIAN_POINT('',(8.96208611562692,93.8,-73.4245373663378));
#59070=CARTESIAN_POINT('',(8.96208611562692,93.8,-73.4245373663378));
#59071=CARTESIAN_POINT('',(11.2172176609382,93.8,-71.6223955720621));
#59072=CARTESIAN_POINT('',(-32.2471594546766,93.8,-44.9552559421386));
#59073=CARTESIAN_POINT('',(-31.8140246522679,93.8,-47.8093280463917));
#59074=CARTESIAN_POINT('',(-32.2471594546766,93.8,-44.9552559421386));
#59075=CARTESIAN_POINT('',(-34.9354258023966,93.8,-43.9033256321612));
#59076=CARTESIAN_POINT('',(-34.9354258023966,93.8,-43.9033256321612));
#59077=CARTESIAN_POINT('',(-37.190557347708,93.8,-45.7054674264369));
#59078=CARTESIAN_POINT('',(-37.190557347708,93.8,-45.7054674264369));
#59079=CARTESIAN_POINT('',(-36.7574225452993,93.8,-48.55953953069));
#59080=CARTESIAN_POINT('',(-36.7574225452993,93.8,-48.55953953069));
#59081=CARTESIAN_POINT('',(-34.0691561975792,93.8,-49.6114698406674));
#59082=CARTESIAN_POINT('',(-34.0691561975792,93.8,-49.6114698406674));
#59083=CARTESIAN_POINT('',(-31.8140246522679,93.8,-47.8093280463917));
#59084=CARTESIAN_POINT('',(-25.2628386068835,93.8,-47.6882510564925));
#59085=CARTESIAN_POINT('',(-24.8297038044748,93.8,-50.5423231607456));
#59086=CARTESIAN_POINT('',(-25.2628386068835,93.8,-47.6882510564925));
#59087=CARTESIAN_POINT('',(-27.9511049546035,93.8,-46.6363207465151));
#59088=CARTESIAN_POINT('',(-27.9511049546035,93.8,-46.6363207465151));
#59089=CARTESIAN_POINT('',(-30.2062364999149,93.8,-48.4384625407908));
#59090=CARTESIAN_POINT('',(-30.2062364999149,93.8,-48.4384625407908));
#59091=CARTESIAN_POINT('',(-29.7731016975061,93.8,-51.2925346450439));
#59092=CARTESIAN_POINT('',(-29.7731016975061,93.8,-51.2925346450439));
#59093=CARTESIAN_POINT('',(-27.0848353497861,93.8,-52.3444649550213));
#59094=CARTESIAN_POINT('',(-27.0848353497861,93.8,-52.3444649550213));
#59095=CARTESIAN_POINT('',(-24.8297038044748,93.8,-50.5423231607456));
#59096=CARTESIAN_POINT('',(-18.2785177590904,93.8,-50.4212461708464));
#59097=CARTESIAN_POINT('',(-17.8453829566817,93.8,-53.2753182750995));
#59098=CARTESIAN_POINT('',(-18.2785177590904,93.8,-50.4212461708464));
#59099=CARTESIAN_POINT('',(-20.9667841068104,93.8,-49.369315860869));
#59100=CARTESIAN_POINT('',(-20.9667841068104,93.8,-49.369315860869));
#59101=CARTESIAN_POINT('',(-23.2219156521217,93.8,-51.1714576551447));
#59102=CARTESIAN_POINT('',(-23.2219156521217,93.8,-51.1714576551447));
#59103=CARTESIAN_POINT('',(-22.788780849713,93.8,-54.0255297593977));
#59104=CARTESIAN_POINT('',(-22.788780849713,93.8,-54.0255297593977));
#59105=CARTESIAN_POINT('',(-20.100514501993,93.8,-55.0774600693752));
#59106=CARTESIAN_POINT('',(-20.100514501993,93.8,-55.0774600693752));
#59107=CARTESIAN_POINT('',(-17.8453829566817,93.8,-53.2753182750995));
#59108=CARTESIAN_POINT('',(-11.2941969112972,93.8,-53.1542412852003));
#59109=CARTESIAN_POINT('',(-10.8610621088885,93.8,-56.0083133894534));
#59110=CARTESIAN_POINT('',(-11.2941969112972,93.8,-53.1542412852003));
#59111=CARTESIAN_POINT('',(-13.9824632590173,93.8,-52.1023109752229));
#59112=CARTESIAN_POINT('',(-13.9824632590173,93.8,-52.1023109752229));
#59113=CARTESIAN_POINT('',(-16.2375948043286,93.8,-53.9044527694986));
#59114=CARTESIAN_POINT('',(-16.2375948043286,93.8,-53.9044527694986));
#59115=CARTESIAN_POINT('',(-15.8044600019199,93.8,-56.7585248737516));
#59116=CARTESIAN_POINT('',(-15.8044600019199,93.8,-56.7585248737516));
#59117=CARTESIAN_POINT('',(-13.1161936541999,93.8,-57.8104551837291));
#59118=CARTESIAN_POINT('',(-13.1161936541999,93.8,-57.8104551837291));
#59119=CARTESIAN_POINT('',(-10.8610621088885,93.8,-56.0083133894534));
#59120=CARTESIAN_POINT('',(-4.30987606350412,93.8,-55.8872363995542));
#59121=CARTESIAN_POINT('',(-3.8767412610954,93.8,-58.7413085038073));
#59122=CARTESIAN_POINT('',(-4.30987606350412,93.8,-55.8872363995542));
#59123=CARTESIAN_POINT('',(-6.99814241122413,93.8,-54.8353060895768));
#59124=CARTESIAN_POINT('',(-6.99814241122413,93.8,-54.8353060895768));
#59125=CARTESIAN_POINT('',(-9.25327395653548,93.8,-56.6374478838525));
#59126=CARTESIAN_POINT('',(-9.25327395653548,93.8,-56.6374478838525));
#59127=CARTESIAN_POINT('',(-8.82013915412675,93.8,-59.4915199881055));
#59128=CARTESIAN_POINT('',(-8.82013915412675,93.8,-59.4915199881055));
#59129=CARTESIAN_POINT('',(-6.13187280640672,93.8,-60.543450298083));
#59130=CARTESIAN_POINT('',(-6.13187280640672,93.8,-60.543450298083));
#59131=CARTESIAN_POINT('',(-3.8767412610954,93.8,-58.7413085038073));
#59132=CARTESIAN_POINT('',(2.67444478428902,93.8,-58.6202315139081));
#59133=CARTESIAN_POINT('',(3.10757958669774,93.8,-61.4743036181612));
#59134=CARTESIAN_POINT('',(2.67444478428902,93.8,-58.6202315139081));
#59135=CARTESIAN_POINT('',(-0.0138215634309935,93.8,-57.5683012039307));
#59136=CARTESIAN_POINT('',(-0.0138215634309935,93.8,-57.5683012039307));
#59137=CARTESIAN_POINT('',(-2.26895310874235,93.8,-59.3704429982063));
#59138=CARTESIAN_POINT('',(-2.26895310874235,93.8,-59.3704429982063));
#59139=CARTESIAN_POINT('',(-1.83581830633362,93.8,-62.2245151024594));
#59140=CARTESIAN_POINT('',(-1.83581830633362,93.8,-62.2245151024594));
#59141=CARTESIAN_POINT('',(0.852448041386411,93.8,-63.2764454124368));
#59142=CARTESIAN_POINT('',(0.852448041386411,93.8,-63.2764454124368));
#59143=CARTESIAN_POINT('',(3.10757958669774,93.8,-61.4743036181612));
#59144=CARTESIAN_POINT('',(9.65876563208215,93.8,-61.353226628262));
#59145=CARTESIAN_POINT('',(10.0919004344909,93.8,-64.2072987325151));
#59146=CARTESIAN_POINT('',(9.65876563208215,93.8,-61.353226628262));
#59147=CARTESIAN_POINT('',(6.97049928436214,93.8,-60.3012963182845));
#59148=CARTESIAN_POINT('',(6.97049928436214,93.8,-60.3012963182845));
#59149=CARTESIAN_POINT('',(4.71536773905078,93.8,-62.1034381125602));
#59150=CARTESIAN_POINT('',(4.71536773905078,93.8,-62.1034381125602));
#59151=CARTESIAN_POINT('',(5.14850254145952,93.8,-64.9575102168133));
#59152=CARTESIAN_POINT('',(5.14850254145952,93.8,-64.9575102168133));
#59153=CARTESIAN_POINT('',(7.83676888917954,93.8,-66.0094405267907));
#59154=CARTESIAN_POINT('',(7.83676888917954,93.8,-66.0094405267907));
#59155=CARTESIAN_POINT('',(10.0919004344909,93.8,-64.2072987325151));
#59156=CARTESIAN_POINT('',(16.6430864798753,93.8,-64.0862217426158));
#59157=CARTESIAN_POINT('',(17.076221282284,93.8,-66.940293846869));
#59158=CARTESIAN_POINT('',(16.6430864798753,93.8,-64.0862217426158));
#59159=CARTESIAN_POINT('',(13.9548201321553,93.8,-63.0342914326384));
#59160=CARTESIAN_POINT('',(13.9548201321553,93.8,-63.0342914326384));
#59161=CARTESIAN_POINT('',(11.6996885868439,93.8,-64.8364332269141));
#59162=CARTESIAN_POINT('',(11.6996885868439,93.8,-64.8364332269141));
#59163=CARTESIAN_POINT('',(12.1328233892526,93.8,-67.6905053311672));
#59164=CARTESIAN_POINT('',(12.1328233892526,93.8,-67.6905053311672));
#59165=CARTESIAN_POINT('',(14.8210897369727,93.8,-68.7424356411446));
#59166=CARTESIAN_POINT('',(14.8210897369727,93.8,-68.7424356411446));
#59167=CARTESIAN_POINT('',(17.076221282284,93.8,-66.940293846869));
#59168=CARTESIAN_POINT('',(-9.04356245840249,93.8,-67.9844349642944));
#59169=CARTESIAN_POINT('',(-8.61042765599378,93.8,-70.8385070685475));
#59170=CARTESIAN_POINT('',(-9.04356245840249,93.8,-67.9844349642944));
#59171=CARTESIAN_POINT('',(-11.7318288061225,93.8,-66.932504654317));
#59172=CARTESIAN_POINT('',(-11.7318288061225,93.8,-66.932504654317));
#59173=CARTESIAN_POINT('',(-13.9869603514339,93.8,-68.7346464485927));
#59174=CARTESIAN_POINT('',(-13.9869603514339,93.8,-68.7346464485927));
#59175=CARTESIAN_POINT('',(-13.5538255490251,93.8,-71.5887185528457));
#59176=CARTESIAN_POINT('',(-13.5538255490251,93.8,-71.5887185528457));
#59177=CARTESIAN_POINT('',(-10.8655592013051,93.8,-72.6406488628232));
#59178=CARTESIAN_POINT('',(-10.8655592013051,93.8,-72.6406488628232));
#59179=CARTESIAN_POINT('',(-8.61042765599378,93.8,-70.8385070685475));
#59180=CARTESIAN_POINT('',(-2.05924161060936,93.8,-70.7174300786483));
#59181=CARTESIAN_POINT('',(-1.62610680820064,93.8,-73.5715021829014));
#59182=CARTESIAN_POINT('',(-2.05924161060936,93.8,-70.7174300786483));
#59183=CARTESIAN_POINT('',(-4.74750795832937,93.8,-69.6654997686709));
#59184=CARTESIAN_POINT('',(-4.74750795832937,93.8,-69.6654997686709));
#59185=CARTESIAN_POINT('',(-7.00263950364073,93.8,-71.4676415629466));
#59186=CARTESIAN_POINT('',(-7.00263950364073,93.8,-71.4676415629466));
#59187=CARTESIAN_POINT('',(-6.569504701232,93.8,-74.3217136671996));
#59188=CARTESIAN_POINT('',(-6.569504701232,93.8,-74.3217136671996));
#59189=CARTESIAN_POINT('',(-3.88123835351197,93.8,-75.3736439771771));
#59190=CARTESIAN_POINT('',(-3.88123835351197,93.8,-75.3736439771771));
#59191=CARTESIAN_POINT('',(-1.62610680820064,93.8,-73.5715021829014));
#59192=CARTESIAN_POINT('',(4.92507923718377,93.8,-73.4504251930022));
#59193=CARTESIAN_POINT('',(5.35821403959249,93.8,-76.3044972972553));
#59194=CARTESIAN_POINT('',(4.92507923718377,93.8,-73.4504251930022));
#59195=CARTESIAN_POINT('',(2.23681288946376,93.8,-72.3984948830248));
#59196=CARTESIAN_POINT('',(2.23681288946376,93.8,-72.3984948830248));
#59197=CARTESIAN_POINT('',(-0.0183186558475948,93.8,-74.2006366773005));
#59198=CARTESIAN_POINT('',(-0.0183186558475948,93.8,-74.2006366773005));
#59199=CARTESIAN_POINT('',(0.414816146561137,93.8,-77.0547087815535));
#59200=CARTESIAN_POINT('',(0.414816146561137,93.8,-77.0547087815535));
#59201=CARTESIAN_POINT('',(3.10308249428116,93.8,-78.1066390915309));
#59202=CARTESIAN_POINT('',(3.10308249428116,93.8,-78.1066390915309));
#59203=CARTESIAN_POINT('',(5.35821403959249,93.8,-76.3044972972553));
#59204=CARTESIAN_POINT('',(11.9094000849769,93.8,-76.1834203073561));
#59205=CARTESIAN_POINT('',(12.3425348873856,93.8,-79.0374924116092));
#59206=CARTESIAN_POINT('',(11.9094000849769,93.8,-76.1834203073561));
#59207=CARTESIAN_POINT('',(9.22113373725689,93.8,-75.1314899973787));
#59208=CARTESIAN_POINT('',(9.22113373725689,93.8,-75.1314899973787));
#59209=CARTESIAN_POINT('',(6.96600219194553,93.8,-76.9336317916543));
#59210=CARTESIAN_POINT('',(6.96600219194553,93.8,-76.9336317916543));
#59211=CARTESIAN_POINT('',(7.39913699435427,93.8,-79.7877038959074));
#59212=CARTESIAN_POINT('',(7.39913699435427,93.8,-79.7877038959074));
#59213=CARTESIAN_POINT('',(10.0874033420743,93.8,-80.8396342058848));
#59214=CARTESIAN_POINT('',(10.0874033420743,93.8,-80.8396342058848));
#59215=CARTESIAN_POINT('',(12.3425348873856,93.8,-79.0374924116092));
#59216=CARTESIAN_POINT('',(18.89372093277,93.8,-78.9164154217099));
#59217=CARTESIAN_POINT('',(19.3268557351787,93.8,-81.770487525963));
#59218=CARTESIAN_POINT('',(18.89372093277,93.8,-78.9164154217099));
#59219=CARTESIAN_POINT('',(16.20545458505,93.8,-77.8644851117325));
#59220=CARTESIAN_POINT('',(16.20545458505,93.8,-77.8644851117325));
#59221=CARTESIAN_POINT('',(13.9503230397387,93.8,-79.6666269060082));
#59222=CARTESIAN_POINT('',(13.9503230397387,93.8,-79.6666269060082));
#59223=CARTESIAN_POINT('',(14.3834578421474,93.8,-82.5206990102613));
#59224=CARTESIAN_POINT('',(14.3834578421474,93.8,-82.5206990102613));
#59225=CARTESIAN_POINT('',(17.0717241898674,93.8,-83.5726293202387));
#59226=CARTESIAN_POINT('',(17.0717241898674,93.8,-83.5726293202387));
#59227=CARTESIAN_POINT('',(19.3268557351787,93.8,-81.770487525963));
#59228=CARTESIAN_POINT('',(25.8780417805632,93.8,-81.6494105360638));
#59229=CARTESIAN_POINT('',(26.3111765829719,93.8,-84.5034826403169));
#59230=CARTESIAN_POINT('',(25.8780417805632,93.8,-81.6494105360638));
#59231=CARTESIAN_POINT('',(23.1897754328432,93.8,-80.5974802260864));
#59232=CARTESIAN_POINT('',(23.1897754328432,93.8,-80.5974802260864));
#59233=CARTESIAN_POINT('',(20.9346438875318,93.8,-82.3996220203621));
#59234=CARTESIAN_POINT('',(20.9346438875318,93.8,-82.3996220203621));
#59235=CARTESIAN_POINT('',(21.3677786899405,93.8,-85.2536941246152));
#59236=CARTESIAN_POINT('',(21.3677786899405,93.8,-85.2536941246152));
#59237=CARTESIAN_POINT('',(24.0560450376606,93.8,-86.3056244345926));
#59238=CARTESIAN_POINT('',(24.0560450376606,93.8,-86.3056244345926));
#59239=CARTESIAN_POINT('',(26.3111765829719,93.8,-84.5034826403169));
#59240=CARTESIAN_POINT('',(32.8623626283563,93.8,-84.3824056504177));
#59241=CARTESIAN_POINT('',(33.295497430765,93.8,-87.2364777546708));
#59242=CARTESIAN_POINT('',(32.8623626283563,93.8,-84.3824056504177));
#59243=CARTESIAN_POINT('',(30.1740962806363,93.8,-83.3304753404403));
#59244=CARTESIAN_POINT('',(30.1740962806363,93.8,-83.3304753404403));
#59245=CARTESIAN_POINT('',(27.9189647353249,93.8,-85.132617134716));
#59246=CARTESIAN_POINT('',(27.9189647353249,93.8,-85.132617134716));
#59247=CARTESIAN_POINT('',(28.3520995377337,93.8,-87.9866892389691));
#59248=CARTESIAN_POINT('',(28.3520995377337,93.8,-87.9866892389691));
#59249=CARTESIAN_POINT('',(31.0403658854537,93.8,-89.0386195489465));
#59250=CARTESIAN_POINT('',(31.0403658854537,93.8,-89.0386195489465));
#59251=CARTESIAN_POINT('',(33.295497430765,93.8,-87.2364777546708));
#59252=CARTESIAN_POINT('',(39.8466834761494,93.8,-87.1154007647716));
#59253=CARTESIAN_POINT('',(40.2798182785581,93.8,-89.9694728690247));
#59254=CARTESIAN_POINT('',(39.8466834761494,93.8,-87.1154007647716));
#59255=CARTESIAN_POINT('',(37.1584171284294,93.8,-86.0634704547942));
#59256=CARTESIAN_POINT('',(37.1584171284294,93.8,-86.0634704547942));
#59257=CARTESIAN_POINT('',(34.903285583118,93.8,-87.8656122490699));
#59258=CARTESIAN_POINT('',(34.903285583118,93.8,-87.8656122490699));
#59259=CARTESIAN_POINT('',(35.3364203855268,93.8,-90.719684353323));
#59260=CARTESIAN_POINT('',(35.3364203855268,93.8,-90.719684353323));
#59261=CARTESIAN_POINT('',(38.0246867332468,93.8,-91.7716146633004));
#59262=CARTESIAN_POINT('',(38.0246867332468,93.8,-91.7716146633004));
#59263=CARTESIAN_POINT('',(40.2798182785581,93.8,-89.9694728690247));
#59264=CARTESIAN_POINT('',(3.7997620107364,93.8,-66.0353283534551));
#59265=CARTESIAN_POINT('',(4.23289681314511,93.8,-68.8894004577082));
#59266=CARTESIAN_POINT('',(3.7997620107364,93.8,-66.0353283534551));
#59267=CARTESIAN_POINT('',(1.11149566301639,93.8,-64.9833980434777));
#59268=CARTESIAN_POINT('',(1.11149566301639,93.8,-64.9833980434777));
#59269=CARTESIAN_POINT('',(-1.14363588229497,93.8,-66.7855398377534));
#59270=CARTESIAN_POINT('',(-1.14363588229497,93.8,-66.7855398377534));
#59271=CARTESIAN_POINT('',(-0.710501079886239,93.8,-69.6396119420065));
#59272=CARTESIAN_POINT('',(-0.710501079886239,93.8,-69.6396119420065));
#59273=CARTESIAN_POINT('',(1.97776526783379,93.8,-70.6915422519839));
#59274=CARTESIAN_POINT('',(1.97776526783379,93.8,-70.6915422519839));
#59275=CARTESIAN_POINT('',(4.23289681314511,93.8,-68.8894004577082));
#59276=CARTESIAN_POINT('',(-3.18455883705674,93.8,-63.3023332391012));
#59277=CARTESIAN_POINT('',(-2.75142403464802,93.8,-66.1564053433543));
#59278=CARTESIAN_POINT('',(-3.18455883705674,93.8,-63.3023332391012));
#59279=CARTESIAN_POINT('',(-5.87282518477675,93.8,-62.2504029291238));
#59280=CARTESIAN_POINT('',(-5.87282518477675,93.8,-62.2504029291238));
#59281=CARTESIAN_POINT('',(-8.1279567300881,93.8,-64.0525447233995));
#59282=CARTESIAN_POINT('',(-8.1279567300881,93.8,-64.0525447233995));
#59283=CARTESIAN_POINT('',(-7.69482192767937,93.8,-66.9066168276526));
#59284=CARTESIAN_POINT('',(-7.69482192767937,93.8,-66.9066168276526));
#59285=CARTESIAN_POINT('',(-5.00655557995934,93.8,-67.95854713763));
#59286=CARTESIAN_POINT('',(-5.00655557995934,93.8,-67.95854713763));
#59287=CARTESIAN_POINT('',(-2.75142403464802,93.8,-66.1564053433543));
#59288=CARTESIAN_POINT('',(-10.1688796848499,93.8,-60.5693381247473));
#59289=CARTESIAN_POINT('',(-9.73574488244115,93.8,-63.4234102290004));
#59290=CARTESIAN_POINT('',(-10.1688796848499,93.8,-60.5693381247473));
#59291=CARTESIAN_POINT('',(-12.8571460325699,93.8,-59.5174078147699));
#59292=CARTESIAN_POINT('',(-12.8571460325699,93.8,-59.5174078147699));
#59293=CARTESIAN_POINT('',(-15.1122775778812,93.8,-61.3195496090456));
#59294=CARTESIAN_POINT('',(-15.1122775778812,93.8,-61.3195496090456));
#59295=CARTESIAN_POINT('',(-14.6791427754725,93.8,-64.1736217132987));
#59296=CARTESIAN_POINT('',(-14.6791427754725,93.8,-64.1736217132987));
#59297=CARTESIAN_POINT('',(-11.9908764277525,93.8,-65.2255520232761));
#59298=CARTESIAN_POINT('',(-11.9908764277525,93.8,-65.2255520232761));
#59299=CARTESIAN_POINT('',(-9.73574488244115,93.8,-63.4234102290004));
#59300=CARTESIAN_POINT('',(-17.153200532643,93.8,-57.8363430103935));
#59301=CARTESIAN_POINT('',(-16.7200657302343,93.8,-60.6904151146466));
#59302=CARTESIAN_POINT('',(-17.153200532643,93.8,-57.8363430103935));
#59303=CARTESIAN_POINT('',(-19.841466880363,93.8,-56.784412700416));
#59304=CARTESIAN_POINT('',(-19.841466880363,93.8,-56.784412700416));
#59305=CARTESIAN_POINT('',(-22.0965984256744,93.8,-58.5865544946917));
#59306=CARTESIAN_POINT('',(-22.0965984256744,93.8,-58.5865544946917));
#59307=CARTESIAN_POINT('',(-21.6634636232656,93.8,-61.4406265989448));
#59308=CARTESIAN_POINT('',(-21.6634636232656,93.8,-61.4406265989448));
#59309=CARTESIAN_POINT('',(-18.9751972755456,93.8,-62.4925569089222));
#59310=CARTESIAN_POINT('',(-18.9751972755456,93.8,-62.4925569089222));
#59311=CARTESIAN_POINT('',(-16.7200657302343,93.8,-60.6904151146466));
#59312=CARTESIAN_POINT('',(46.8310043239425,93.8,-89.8483958791255));
#59313=CARTESIAN_POINT('',(47.2641391263513,93.8,-92.7024679833786));
#59314=CARTESIAN_POINT('',(46.8310043239425,93.8,-89.8483958791255));
#59315=CARTESIAN_POINT('',(44.1427379762225,93.8,-88.7964655691481));
#59316=CARTESIAN_POINT('',(44.1427379762225,93.8,-88.7964655691481));
#59317=CARTESIAN_POINT('',(41.8876064309112,93.8,-90.5986073634238));
#59318=CARTESIAN_POINT('',(41.8876064309112,93.8,-90.5986073634238));
#59319=CARTESIAN_POINT('',(42.3207412333199,93.8,-93.4526794676769));
#59320=CARTESIAN_POINT('',(42.3207412333199,93.8,-93.4526794676769));
#59321=CARTESIAN_POINT('',(45.0090075810399,93.8,-94.5046097776543));
#59322=CARTESIAN_POINT('',(45.0090075810399,93.8,-94.5046097776543));
#59323=CARTESIAN_POINT('',(47.2641391263513,93.8,-92.7024679833786));
#59324=CARTESIAN_POINT('',(-38.1061630760224,93.8,-49.6373576673318));
#59325=CARTESIAN_POINT('',(-37.6730282736137,93.8,-52.4914297715849));
#59326=CARTESIAN_POINT('',(-38.1061630760224,93.8,-49.6373576673318));
#59327=CARTESIAN_POINT('',(-40.7944294237424,93.8,-48.5854273573544));
#59328=CARTESIAN_POINT('',(-40.7944294237424,93.8,-48.5854273573544));
#59329=CARTESIAN_POINT('',(-43.0495609690538,93.8,-50.3875691516301));
#59330=CARTESIAN_POINT('',(-43.0495609690538,93.8,-50.3875691516301));
#59331=CARTESIAN_POINT('',(-42.616426166645,93.8,-53.2416412558831));
#59332=CARTESIAN_POINT('',(-42.616426166645,93.8,-53.2416412558831));
#59333=CARTESIAN_POINT('',(-39.928159818925,93.8,-54.2935715658606));
#59334=CARTESIAN_POINT('',(-39.928159818925,93.8,-54.2935715658606));
#59335=CARTESIAN_POINT('',(-37.6730282736137,93.8,-52.4914297715849));
#59336=CARTESIAN_POINT('',(-31.1218422282293,93.8,-52.3703527816857));
#59337=CARTESIAN_POINT('',(-30.6887074258205,93.8,-55.2244248859388));
#59338=CARTESIAN_POINT('',(-31.1218422282293,93.8,-52.3703527816857));
#59339=CARTESIAN_POINT('',(-33.8101085759493,93.8,-51.3184224717083));
#59340=CARTESIAN_POINT('',(-33.8101085759493,93.8,-51.3184224717083));
#59341=CARTESIAN_POINT('',(-36.0652401212606,93.8,-53.120564265984));
#59342=CARTESIAN_POINT('',(-36.0652401212606,93.8,-53.120564265984));
#59343=CARTESIAN_POINT('',(-35.6321053188519,93.8,-55.974636370237));
#59344=CARTESIAN_POINT('',(-35.6321053188519,93.8,-55.974636370237));
#59345=CARTESIAN_POINT('',(-32.9438389711319,93.8,-57.0265666802144));
#59346=CARTESIAN_POINT('',(-32.9438389711319,93.8,-57.0265666802144));
#59347=CARTESIAN_POINT('',(-30.6887074258205,93.8,-55.2244248859388));
#59348=CARTESIAN_POINT('',(-24.1375213804361,93.8,-55.1033478960396));
#59349=CARTESIAN_POINT('',(-23.7043865780274,93.8,-57.9574200002927));
#59350=CARTESIAN_POINT('',(-24.1375213804361,93.8,-55.1033478960396));
#59351=CARTESIAN_POINT('',(-26.8257877281561,93.8,-54.0514175860622));
#59352=CARTESIAN_POINT('',(-26.8257877281561,93.8,-54.0514175860622));
#59353=CARTESIAN_POINT('',(-29.0809192734675,93.8,-55.8535593803378));
#59354=CARTESIAN_POINT('',(-29.0809192734675,93.8,-55.8535593803378));
#59355=CARTESIAN_POINT('',(-28.6477844710588,93.8,-58.7076314845909));
#59356=CARTESIAN_POINT('',(-28.6477844710588,93.8,-58.7076314845909));
#59357=CARTESIAN_POINT('',(-25.9595181233387,93.8,-59.7595617945683));
#59358=CARTESIAN_POINT('',(-25.9595181233387,93.8,-59.7595617945683));
#59359=CARTESIAN_POINT('',(-23.7043865780274,93.8,-57.9574200002927));
#59360=CARTESIAN_POINT('',(-23.2446216430976,93.8,-104.276030658515));
#59361=CARTESIAN_POINT('',(-22.8114868406889,93.8,-107.130102762768));
#59362=CARTESIAN_POINT('',(-23.2446216430976,93.8,-104.276030658515));
#59363=CARTESIAN_POINT('',(-25.9328879908176,93.8,-103.224100348538));
#59364=CARTESIAN_POINT('',(-25.9328879908176,93.8,-103.224100348538));
#59365=CARTESIAN_POINT('',(-28.188019536129,93.8,-105.026242142813));
#59366=CARTESIAN_POINT('',(-28.188019536129,93.8,-105.026242142813));
#59367=CARTESIAN_POINT('',(-27.7548847337203,93.8,-107.880314247066));
#59368=CARTESIAN_POINT('',(-27.7548847337203,93.8,-107.880314247066));
#59369=CARTESIAN_POINT('',(-25.0666183860002,93.8,-108.932244557044));
#59370=CARTESIAN_POINT('',(-25.0666183860002,93.8,-108.932244557044));
#59371=CARTESIAN_POINT('',(-22.8114868406889,93.8,-107.130102762768));
#59372=CARTESIAN_POINT('',(-16.2603007953045,93.8,-107.009025772869));
#59373=CARTESIAN_POINT('',(-15.8271659928958,93.8,-109.863097877122));
#59374=CARTESIAN_POINT('',(-16.2603007953045,93.8,-107.009025772869));
#59375=CARTESIAN_POINT('',(-18.9485671430245,93.8,-105.957095462892));
#59376=CARTESIAN_POINT('',(-18.9485671430245,93.8,-105.957095462892));
#59377=CARTESIAN_POINT('',(-21.2036986883359,93.8,-107.759237257167));
#59378=CARTESIAN_POINT('',(-21.2036986883359,93.8,-107.759237257167));
#59379=CARTESIAN_POINT('',(-20.7705638859271,93.8,-110.61330936142));
#59380=CARTESIAN_POINT('',(-20.7705638859271,93.8,-110.61330936142));
#59381=CARTESIAN_POINT('',(-18.0822975382071,93.8,-111.665239671398));
#59382=CARTESIAN_POINT('',(-18.0822975382071,93.8,-111.665239671398));
#59383=CARTESIAN_POINT('',(-15.8271659928958,93.8,-109.863097877122));
#59384=CARTESIAN_POINT('',(-9.27597994751136,93.8,-109.742020887223));
#59385=CARTESIAN_POINT('',(-8.84284514510264,93.8,-112.596092991476));
#59386=CARTESIAN_POINT('',(-9.27597994751136,93.8,-109.742020887223));
#59387=CARTESIAN_POINT('',(-11.9642462952314,93.8,-108.690090577245));
#59388=CARTESIAN_POINT('',(-11.9642462952314,93.8,-108.690090577245));
#59389=CARTESIAN_POINT('',(-14.2193778405427,93.8,-110.492232371521));
#59390=CARTESIAN_POINT('',(-14.2193778405427,93.8,-110.492232371521));
#59391=CARTESIAN_POINT('',(-13.786243038134,93.8,-113.346304475774));
#59392=CARTESIAN_POINT('',(-13.786243038134,93.8,-113.346304475774));
#59393=CARTESIAN_POINT('',(-11.097976690414,93.8,-114.398234785752));
#59394=CARTESIAN_POINT('',(-11.097976690414,93.8,-114.398234785752));
#59395=CARTESIAN_POINT('',(-8.84284514510264,93.8,-112.596092991476));
#59396=CARTESIAN_POINT('',(-2.29165909971822,93.8,-112.475016001577));
#59397=CARTESIAN_POINT('',(-1.85852429730951,93.8,-115.32908810583));
#59398=CARTESIAN_POINT('',(-2.29165909971822,93.8,-112.475016001577));
#59399=CARTESIAN_POINT('',(-4.97992544743824,93.8,-111.423085691599));
#59400=CARTESIAN_POINT('',(-4.97992544743824,93.8,-111.423085691599));
#59401=CARTESIAN_POINT('',(-7.23505699274959,93.8,-113.225227485875));
#59402=CARTESIAN_POINT('',(-7.23505699274959,93.8,-113.225227485875));
#59403=CARTESIAN_POINT('',(-6.80192219034086,93.8,-116.079299590128));
#59404=CARTESIAN_POINT('',(-6.80192219034086,93.8,-116.079299590128));
#59405=CARTESIAN_POINT('',(-4.11365584262083,93.8,-117.131229900105));
#59406=CARTESIAN_POINT('',(-4.11365584262083,93.8,-117.131229900105));
#59407=CARTESIAN_POINT('',(-1.85852429730951,93.8,-115.32908810583));
#59408=CARTESIAN_POINT('',(4.69266174807491,93.8,-115.208011115931));
#59409=CARTESIAN_POINT('',(5.12579655048363,93.8,-118.062083220184));
#59410=CARTESIAN_POINT('',(4.69266174807491,93.8,-115.208011115931));
#59411=CARTESIAN_POINT('',(2.0043954003549,93.8,-114.156080805953));
#59412=CARTESIAN_POINT('',(2.0043954003549,93.8,-114.156080805953));
#59413=CARTESIAN_POINT('',(-0.250736144956458,93.8,-115.958222600229));
#59414=CARTESIAN_POINT('',(-0.250736144956458,93.8,-115.958222600229));
#59415=CARTESIAN_POINT('',(0.182398657452273,93.8,-118.812294704482));
#59416=CARTESIAN_POINT('',(0.182398657452273,93.8,-118.812294704482));
#59417=CARTESIAN_POINT('',(2.8706650051723,93.8,-119.864225014459));
#59418=CARTESIAN_POINT('',(2.8706650051723,93.8,-119.864225014459));
#59419=CARTESIAN_POINT('',(5.12579655048363,93.8,-118.062083220184));
#59420=CARTESIAN_POINT('',(11.676982595868,93.8,-117.941006230285));
#59421=CARTESIAN_POINT('',(12.1101173982768,93.8,-120.795078334538));
#59422=CARTESIAN_POINT('',(11.676982595868,93.8,-117.941006230285));
#59423=CARTESIAN_POINT('',(8.98871624814803,93.8,-116.889075920307));
#59424=CARTESIAN_POINT('',(8.98871624814803,93.8,-116.889075920307));
#59425=CARTESIAN_POINT('',(6.73358470283667,93.8,-118.691217714583));
#59426=CARTESIAN_POINT('',(6.73358470283667,93.8,-118.691217714583));
#59427=CARTESIAN_POINT('',(7.1667195052454,93.8,-121.545289818836));
#59428=CARTESIAN_POINT('',(7.1667195052454,93.8,-121.545289818836));
#59429=CARTESIAN_POINT('',(9.85498585296543,93.8,-122.597220128813));
#59430=CARTESIAN_POINT('',(9.85498585296543,93.8,-122.597220128813));
#59431=CARTESIAN_POINT('',(12.1101173982768,93.8,-120.795078334538));
#59432=CARTESIAN_POINT('',(18.6613034436612,93.8,-120.674001344638));
#59433=CARTESIAN_POINT('',(19.0944382460699,93.8,-123.528073448892));
#59434=CARTESIAN_POINT('',(18.6613034436612,93.8,-120.674001344638));
#59435=CARTESIAN_POINT('',(15.9730370959412,93.8,-119.622071034661));
#59436=CARTESIAN_POINT('',(15.9730370959412,93.8,-119.622071034661));
#59437=CARTESIAN_POINT('',(13.7179055506298,93.8,-121.424212828937));
#59438=CARTESIAN_POINT('',(13.7179055506298,93.8,-121.424212828937));
#59439=CARTESIAN_POINT('',(14.1510403530385,93.8,-124.27828493319));
#59440=CARTESIAN_POINT('',(14.1510403530385,93.8,-124.27828493319));
#59441=CARTESIAN_POINT('',(16.8393067007586,93.8,-125.330215243167));
#59442=CARTESIAN_POINT('',(16.8393067007586,93.8,-125.330215243167));
#59443=CARTESIAN_POINT('',(19.0944382460699,93.8,-123.528073448892));
#59444=CARTESIAN_POINT('',(25.6456242914543,93.8,-123.406996458992));
#59445=CARTESIAN_POINT('',(26.078759093863,93.8,-126.261068563245));
#59446=CARTESIAN_POINT('',(25.6456242914543,93.8,-123.406996458992));
#59447=CARTESIAN_POINT('',(22.9573579437343,93.8,-122.355066149015));
#59448=CARTESIAN_POINT('',(22.9573579437343,93.8,-122.355066149015));
#59449=CARTESIAN_POINT('',(20.7022263984229,93.8,-124.157207943291));
#59450=CARTESIAN_POINT('',(20.7022263984229,93.8,-124.157207943291));
#59451=CARTESIAN_POINT('',(21.1353612008317,93.8,-127.011280047544));
#59452=CARTESIAN_POINT('',(21.1353612008317,93.8,-127.011280047544));
#59453=CARTESIAN_POINT('',(23.8236275485517,93.8,-128.063210357521));
#59454=CARTESIAN_POINT('',(23.8236275485517,93.8,-128.063210357521));
#59455=CARTESIAN_POINT('',(26.078759093863,93.8,-126.261068563245));
#59456=CARTESIAN_POINT('',(-45.3229014129244,93.8,-88.6619484759063));
#59457=CARTESIAN_POINT('',(-44.8897666105157,93.8,-91.5160205801594));
#59458=CARTESIAN_POINT('',(-45.3229014129244,93.8,-88.6619484759063));
#59459=CARTESIAN_POINT('',(-48.0111677606444,93.8,-87.6100181659289));
#59460=CARTESIAN_POINT('',(-48.0111677606444,93.8,-87.6100181659289));
#59461=CARTESIAN_POINT('',(-50.2662993059558,93.8,-89.4121599602046));
#59462=CARTESIAN_POINT('',(-50.2662993059558,93.8,-89.4121599602046));
#59463=CARTESIAN_POINT('',(-49.833164503547,93.8,-92.2662320644577));
#59464=CARTESIAN_POINT('',(-49.833164503547,93.8,-92.2662320644577));
#59465=CARTESIAN_POINT('',(-47.144898155827,93.8,-93.3181623744351));
#59466=CARTESIAN_POINT('',(-47.144898155827,93.8,-93.3181623744351));
#59467=CARTESIAN_POINT('',(-44.8897666105157,93.8,-91.5160205801594));
#59468=CARTESIAN_POINT('',(-38.3385805651313,93.8,-91.3949435902602));
#59469=CARTESIAN_POINT('',(-37.9054457627226,93.8,-94.2490156945133));
#59470=CARTESIAN_POINT('',(-38.3385805651313,93.8,-91.3949435902602));
#59471=CARTESIAN_POINT('',(-41.0268469128513,93.8,-90.3430132802828));
#59472=CARTESIAN_POINT('',(-41.0268469128513,93.8,-90.3430132802828));
#59473=CARTESIAN_POINT('',(-43.2819784581626,93.8,-92.1451550745585));
#59474=CARTESIAN_POINT('',(-43.2819784581626,93.8,-92.1451550745585));
#59475=CARTESIAN_POINT('',(-42.8488436557539,93.8,-94.9992271788116));
#59476=CARTESIAN_POINT('',(-42.8488436557539,93.8,-94.9992271788116));
#59477=CARTESIAN_POINT('',(-40.1605773080339,93.8,-96.051157488789));
#59478=CARTESIAN_POINT('',(-40.1605773080339,93.8,-96.051157488789));
#59479=CARTESIAN_POINT('',(-37.9054457627226,93.8,-94.2490156945133));
#59480=CARTESIAN_POINT('',(-31.3542597173381,93.8,-94.1279387046141));
#59481=CARTESIAN_POINT('',(-30.9211249149294,93.8,-96.9820108088672));
#59482=CARTESIAN_POINT('',(-31.3542597173381,93.8,-94.1279387046141));
#59483=CARTESIAN_POINT('',(-34.0425260650581,93.8,-93.0760083946367));
#59484=CARTESIAN_POINT('',(-34.0425260650581,93.8,-93.0760083946367));
#59485=CARTESIAN_POINT('',(-36.2976576103695,93.8,-94.8781501889124));
#59486=CARTESIAN_POINT('',(-36.2976576103695,93.8,-94.8781501889124));
#59487=CARTESIAN_POINT('',(-35.8645228079608,93.8,-97.7322222931655));
#59488=CARTESIAN_POINT('',(-35.8645228079608,93.8,-97.7322222931655));
#59489=CARTESIAN_POINT('',(-33.1762564602408,93.8,-98.7841526031429));
#59490=CARTESIAN_POINT('',(-33.1762564602408,93.8,-98.7841526031429));
#59491=CARTESIAN_POINT('',(-30.9211249149294,93.8,-96.9820108088672));
#59492=CARTESIAN_POINT('',(-24.369938869545,93.8,-96.860933818968));
#59493=CARTESIAN_POINT('',(-23.9368040671363,93.8,-99.7150059232211));
#59494=CARTESIAN_POINT('',(-24.369938869545,93.8,-96.860933818968));
#59495=CARTESIAN_POINT('',(-27.058205217265,93.8,-95.8090035089906));
#59496=CARTESIAN_POINT('',(-27.058205217265,93.8,-95.8090035089906));
#59497=CARTESIAN_POINT('',(-29.3133367625764,93.8,-97.6111453032663));
#59498=CARTESIAN_POINT('',(-29.3133367625764,93.8,-97.6111453032663));
#59499=CARTESIAN_POINT('',(-28.8802019601676,93.8,-100.465217407519));
#59500=CARTESIAN_POINT('',(-28.8802019601676,93.8,-100.465217407519));
#59501=CARTESIAN_POINT('',(-26.1919356124476,93.8,-101.517147717497));
#59502=CARTESIAN_POINT('',(-26.1919356124476,93.8,-101.517147717497));
#59503=CARTESIAN_POINT('',(-23.9368040671363,93.8,-99.7150059232211));
#59504=CARTESIAN_POINT('',(-17.3856180217519,93.8,-99.5939289333219));
#59505=CARTESIAN_POINT('',(-16.9524832193432,93.8,-102.448001037575));
#59506=CARTESIAN_POINT('',(-17.3856180217519,93.8,-99.5939289333219));
#59507=CARTESIAN_POINT('',(-20.0738843694719,93.8,-98.5419986233445));
#59508=CARTESIAN_POINT('',(-20.0738843694719,93.8,-98.5419986233445));
#59509=CARTESIAN_POINT('',(-22.3290159147832,93.8,-100.34414041762));
#59510=CARTESIAN_POINT('',(-22.3290159147832,93.8,-100.34414041762));
#59511=CARTESIAN_POINT('',(-21.8958811123745,93.8,-103.198212521873));
#59512=CARTESIAN_POINT('',(-21.8958811123745,93.8,-103.198212521873));
#59513=CARTESIAN_POINT('',(-19.2076147646545,93.8,-104.250142831851));
#59514=CARTESIAN_POINT('',(-19.2076147646545,93.8,-104.250142831851));
#59515=CARTESIAN_POINT('',(-16.9524832193432,93.8,-102.448001037575));
#59516=CARTESIAN_POINT('',(-10.4012971739587,93.8,-102.326924047676));
#59517=CARTESIAN_POINT('',(-9.96816237155003,93.8,-105.180996151929));
#59518=CARTESIAN_POINT('',(-10.4012971739587,93.8,-102.326924047676));
#59519=CARTESIAN_POINT('',(-13.0895635216788,93.8,-101.274993737698));
#59520=CARTESIAN_POINT('',(-13.0895635216788,93.8,-101.274993737698));
#59521=CARTESIAN_POINT('',(-15.3446950669901,93.8,-103.077135531974));
#59522=CARTESIAN_POINT('',(-15.3446950669901,93.8,-103.077135531974));
#59523=CARTESIAN_POINT('',(-14.9115602645814,93.8,-105.931207636227));
#59524=CARTESIAN_POINT('',(-14.9115602645814,93.8,-105.931207636227));
#59525=CARTESIAN_POINT('',(-12.2232939168614,93.8,-106.983137946205));
#59526=CARTESIAN_POINT('',(-12.2232939168614,93.8,-106.983137946205));
#59527=CARTESIAN_POINT('',(-9.96816237155003,93.8,-105.180996151929));
#59528=CARTESIAN_POINT('',(-3.41697632616561,93.8,-105.05991916203));
#59529=CARTESIAN_POINT('',(-2.9838415237569,93.8,-107.913991266283));
#59530=CARTESIAN_POINT('',(-3.41697632616561,93.8,-105.05991916203));
#59531=CARTESIAN_POINT('',(-6.10524267388563,93.8,-104.007988852052));
#59532=CARTESIAN_POINT('',(-6.10524267388563,93.8,-104.007988852052));
#59533=CARTESIAN_POINT('',(-8.36037421919698,93.8,-105.810130646328));
#59534=CARTESIAN_POINT('',(-8.36037421919698,93.8,-105.810130646328));
#59535=CARTESIAN_POINT('',(-7.92723941678825,93.8,-108.664202750581));
#59536=CARTESIAN_POINT('',(-7.92723941678825,93.8,-108.664202750581));
#59537=CARTESIAN_POINT('',(-5.23897306906822,93.8,-109.716133060558));
#59538=CARTESIAN_POINT('',(-5.23897306906822,93.8,-109.716133060558));
#59539=CARTESIAN_POINT('',(-2.9838415237569,93.8,-107.913991266283));
#59540=CARTESIAN_POINT('',(3.56734452162752,93.8,-107.792914276384));
#59541=CARTESIAN_POINT('',(4.00047932403623,93.8,-110.646986380637));
#59542=CARTESIAN_POINT('',(3.56734452162752,93.8,-107.792914276384));
#59543=CARTESIAN_POINT('',(0.879078173907508,93.8,-106.740983966406));
#59544=CARTESIAN_POINT('',(0.879078173907508,93.8,-106.740983966406));
#59545=CARTESIAN_POINT('',(-1.37605337140385,93.8,-108.543125760682));
#59546=CARTESIAN_POINT('',(-1.37605337140385,93.8,-108.543125760682));
#59547=CARTESIAN_POINT('',(-0.942918568995116,93.8,-111.397197864935));
#59548=CARTESIAN_POINT('',(-0.942918568995116,93.8,-111.397197864935));
#59549=CARTESIAN_POINT('',(1.74534777872491,93.8,-112.449128174912));
#59550=CARTESIAN_POINT('',(1.74534777872491,93.8,-112.449128174912));
#59551=CARTESIAN_POINT('',(4.00047932403624,93.8,-110.646986380637));
#59552=CARTESIAN_POINT('',(-20.9939871902029,93.8,-119.106224337609));
#59553=CARTESIAN_POINT('',(-20.5608523877941,93.8,-121.960296441862));
#59554=CARTESIAN_POINT('',(-20.9939871902029,93.8,-119.106224337609));
#59555=CARTESIAN_POINT('',(-23.6822535379229,93.8,-118.054294027632));
#59556=CARTESIAN_POINT('',(-23.6822535379229,93.8,-118.054294027632));
#59557=CARTESIAN_POINT('',(-25.9373850832342,93.8,-119.856435821907));
#59558=CARTESIAN_POINT('',(-25.9373850832342,93.8,-119.856435821907));
#59559=CARTESIAN_POINT('',(-25.5042502808255,93.8,-122.710507926161));
#59560=CARTESIAN_POINT('',(-25.5042502808255,93.8,-122.710507926161));
#59561=CARTESIAN_POINT('',(-22.8159839331055,93.8,-123.762438236138));
#59562=CARTESIAN_POINT('',(-22.8159839331055,93.8,-123.762438236138));
#59563=CARTESIAN_POINT('',(-20.5608523877941,93.8,-121.960296441862));
#59564=CARTESIAN_POINT('',(-14.0096663424097,93.8,-121.839219451963));
#59565=CARTESIAN_POINT('',(-13.576531540001,93.8,-124.693291556216));
#59566=CARTESIAN_POINT('',(-14.0096663424097,93.8,-121.839219451963));
#59567=CARTESIAN_POINT('',(-16.6979326901297,93.8,-120.787289141986));
#59568=CARTESIAN_POINT('',(-16.6979326901297,93.8,-120.787289141986));
#59569=CARTESIAN_POINT('',(-18.9530642354411,93.8,-122.589430936261));
#59570=CARTESIAN_POINT('',(-18.9530642354411,93.8,-122.589430936261));
#59571=CARTESIAN_POINT('',(-18.5199294330324,93.8,-125.443503040514));
#59572=CARTESIAN_POINT('',(-18.5199294330324,93.8,-125.443503040514));
#59573=CARTESIAN_POINT('',(-15.8316630853123,93.8,-126.495433350492));
#59574=CARTESIAN_POINT('',(-15.8316630853123,93.8,-126.495433350492));
#59575=CARTESIAN_POINT('',(-13.576531540001,93.8,-124.693291556216));
#59576=CARTESIAN_POINT('',(-7.02534549461661,93.8,-124.572214566317));
#59577=CARTESIAN_POINT('',(-6.59221069220789,93.8,-127.42628667057));
#59578=CARTESIAN_POINT('',(-7.02534549461661,93.8,-124.572214566317));
#59579=CARTESIAN_POINT('',(-9.71361184233662,93.8,-123.52028425634));
#59580=CARTESIAN_POINT('',(-9.71361184233662,93.8,-123.52028425634));
#59581=CARTESIAN_POINT('',(-11.968743387648,93.8,-125.322426050615));
#59582=CARTESIAN_POINT('',(-11.968743387648,93.8,-125.322426050615));
#59583=CARTESIAN_POINT('',(-11.5356085852392,93.8,-128.176498154868));
#59584=CARTESIAN_POINT('',(-11.5356085852392,93.8,-128.176498154868));
#59585=CARTESIAN_POINT('',(-8.84734223751921,93.8,-129.228428464846));
#59586=CARTESIAN_POINT('',(-8.84734223751921,93.8,-129.228428464846));
#59587=CARTESIAN_POINT('',(-6.59221069220789,93.8,-127.42628667057));
#59588=CARTESIAN_POINT('',(-0.0410246468234739,93.8,-127.305209680671));
#59589=CARTESIAN_POINT('',(0.392110155585244,93.8,-130.159281784924));
#59590=CARTESIAN_POINT('',(-0.0410246468234739,93.8,-127.305209680671));
#59591=CARTESIAN_POINT('',(-2.72929099454348,93.8,-126.253279370693));
#59592=CARTESIAN_POINT('',(-2.72929099454348,93.8,-126.253279370693));
#59593=CARTESIAN_POINT('',(-4.98442253985484,93.8,-128.055421164969));
#59594=CARTESIAN_POINT('',(-4.98442253985484,93.8,-128.055421164969));
#59595=CARTESIAN_POINT('',(-4.55128773744611,93.8,-130.909493269222));
#59596=CARTESIAN_POINT('',(-4.55128773744611,93.8,-130.909493269222));
#59597=CARTESIAN_POINT('',(-1.86302138972608,93.8,-131.9614235792));
#59598=CARTESIAN_POINT('',(-1.86302138972608,93.8,-131.9614235792));
#59599=CARTESIAN_POINT('',(0.392110155585244,93.8,-130.159281784924));
#59600=CARTESIAN_POINT('',(-43.0722669600296,93.8,-103.492142155));
#59601=CARTESIAN_POINT('',(-42.6391321576209,93.8,-106.346214259254));
#59602=CARTESIAN_POINT('',(-43.0722669600296,93.8,-103.492142155));
#59603=CARTESIAN_POINT('',(-45.7605333077496,93.8,-102.440211845023));
#59604=CARTESIAN_POINT('',(-45.7605333077496,93.8,-102.440211845023));
#59605=CARTESIAN_POINT('',(-48.015664853061,93.8,-104.242353639299));
#59606=CARTESIAN_POINT('',(-48.015664853061,93.8,-104.242353639299));
#59607=CARTESIAN_POINT('',(-47.5825300506523,93.8,-107.096425743552));
#59608=CARTESIAN_POINT('',(-47.5825300506523,93.8,-107.096425743552));
#59609=CARTESIAN_POINT('',(-44.8942637029322,93.8,-108.148356053529));
#59610=CARTESIAN_POINT('',(-44.8942637029322,93.8,-108.148356053529));
#59611=CARTESIAN_POINT('',(-42.6391321576209,93.8,-106.346214259254));
#59612=CARTESIAN_POINT('',(-36.0879461122365,93.8,-106.225137269354));
#59613=CARTESIAN_POINT('',(-35.6548113098278,93.8,-109.079209373607));
#59614=CARTESIAN_POINT('',(-36.0879461122365,93.8,-106.225137269354));
#59615=CARTESIAN_POINT('',(-38.7762124599565,93.8,-105.173206959377));
#59616=CARTESIAN_POINT('',(-38.7762124599565,93.8,-105.173206959377));
#59617=CARTESIAN_POINT('',(-41.0313440052679,93.8,-106.975348753653));
#59618=CARTESIAN_POINT('',(-41.0313440052679,93.8,-106.975348753653));
#59619=CARTESIAN_POINT('',(-40.5982092028591,93.8,-109.829420857906));
#59620=CARTESIAN_POINT('',(-40.5982092028591,93.8,-109.829420857906));
#59621=CARTESIAN_POINT('',(-37.9099428551391,93.8,-110.881351167883));
#59622=CARTESIAN_POINT('',(-37.9099428551391,93.8,-110.881351167883));
#59623=CARTESIAN_POINT('',(-35.6548113098278,93.8,-109.079209373607));
#59624=CARTESIAN_POINT('',(-29.1036252644434,93.8,-108.958132383708));
#59625=CARTESIAN_POINT('',(-28.6704904620346,93.8,-111.812204487961));
#59626=CARTESIAN_POINT('',(-29.1036252644434,93.8,-108.958132383708));
#59627=CARTESIAN_POINT('',(-31.7918916121634,93.8,-107.906202073731));
#59628=CARTESIAN_POINT('',(-31.7918916121634,93.8,-107.906202073731));
#59629=CARTESIAN_POINT('',(-34.0470231574747,93.8,-109.708343868006));
#59630=CARTESIAN_POINT('',(-34.0470231574747,93.8,-109.708343868006));
#59631=CARTESIAN_POINT('',(-33.613888355066,93.8,-112.56241597226));
#59632=CARTESIAN_POINT('',(-33.613888355066,93.8,-112.56241597226));
#59633=CARTESIAN_POINT('',(-30.925622007346,93.8,-113.614346282237));
#59634=CARTESIAN_POINT('',(-30.925622007346,93.8,-113.614346282237));
#59635=CARTESIAN_POINT('',(-28.6704904620347,93.8,-111.812204487961));
#59636=CARTESIAN_POINT('',(-22.1193044166502,93.8,-111.691127498062));
#59637=CARTESIAN_POINT('',(-21.6861696142415,93.8,-114.545199602315));
#59638=CARTESIAN_POINT('',(-22.1193044166502,93.8,-111.691127498062));
#59639=CARTESIAN_POINT('',(-24.8075707643703,93.8,-110.639197188085));
#59640=CARTESIAN_POINT('',(-24.8075707643703,93.8,-110.639197188085));
#59641=CARTESIAN_POINT('',(-27.0627023096816,93.8,-112.44133898236));
#59642=CARTESIAN_POINT('',(-27.0627023096816,93.8,-112.44133898236));
#59643=CARTESIAN_POINT('',(-26.6295675072729,93.8,-115.295411086613));
#59644=CARTESIAN_POINT('',(-26.6295675072729,93.8,-115.295411086613));
#59645=CARTESIAN_POINT('',(-23.9413011595528,93.8,-116.347341396591));
#59646=CARTESIAN_POINT('',(-23.9413011595528,93.8,-116.347341396591));
#59647=CARTESIAN_POINT('',(-21.6861696142415,93.8,-114.545199602315));
#59648=CARTESIAN_POINT('',(12.8022998223154,93.8,-125.356103069832));
#59649=CARTESIAN_POINT('',(13.2354346247241,93.8,-128.210175174085));
#59650=CARTESIAN_POINT('',(12.8022998223154,93.8,-125.356103069832));
#59651=CARTESIAN_POINT('',(10.1140334745954,93.8,-124.304172759854));
#59652=CARTESIAN_POINT('',(10.1140334745954,93.8,-124.304172759854));
#59653=CARTESIAN_POINT('',(7.85890192928405,93.8,-126.10631455413));
#59654=CARTESIAN_POINT('',(7.85890192928405,93.8,-126.10631455413));
#59655=CARTESIAN_POINT('',(8.29203673169278,93.8,-128.960386658383));
#59656=CARTESIAN_POINT('',(8.29203673169278,93.8,-128.960386658383));
#59657=CARTESIAN_POINT('',(10.9803030794128,93.8,-130.01231696836));
#59658=CARTESIAN_POINT('',(10.9803030794128,93.8,-130.01231696836));
#59659=CARTESIAN_POINT('',(13.2354346247241,93.8,-128.210175174085));
#59660=CARTESIAN_POINT('',(-44.197584186477,93.8,-96.0770453154534));
#59661=CARTESIAN_POINT('',(-43.7644493840683,93.8,-98.9311174197065));
#59662=CARTESIAN_POINT('',(-44.197584186477,93.8,-96.0770453154534));
#59663=CARTESIAN_POINT('',(-46.885850534197,93.8,-95.025115005476));
#59664=CARTESIAN_POINT('',(-46.885850534197,93.8,-95.025115005476));
#59665=CARTESIAN_POINT('',(-49.1409820795084,93.8,-96.8272567997517));
#59666=CARTESIAN_POINT('',(-49.1409820795084,93.8,-96.8272567997517));
#59667=CARTESIAN_POINT('',(-48.7078472770996,93.8,-99.6813289040047));
#59668=CARTESIAN_POINT('',(-48.7078472770996,93.8,-99.6813289040047));
#59669=CARTESIAN_POINT('',(-46.0195809293796,93.8,-100.733259213982));
#59670=CARTESIAN_POINT('',(-46.0195809293796,93.8,-100.733259213982));
#59671=CARTESIAN_POINT('',(-43.7644493840683,93.8,-98.9311174197065));
#59672=CARTESIAN_POINT('',(-37.2132633386839,93.8,-98.8100404298073));
#59673=CARTESIAN_POINT('',(-36.7801285362752,93.8,-101.66411253406));
#59674=CARTESIAN_POINT('',(-37.2132633386839,93.8,-98.8100404298073));
#59675=CARTESIAN_POINT('',(-39.9015296864039,93.8,-97.7581101198299));
#59676=CARTESIAN_POINT('',(-39.9015296864039,93.8,-97.7581101198299));
#59677=CARTESIAN_POINT('',(-42.1566612317152,93.8,-99.5602519141056));
#59678=CARTESIAN_POINT('',(-42.1566612317152,93.8,-99.5602519141056));
#59679=CARTESIAN_POINT('',(-41.7235264293065,93.8,-102.414324018359));
#59680=CARTESIAN_POINT('',(-41.7235264293065,93.8,-102.414324018359));
#59681=CARTESIAN_POINT('',(-39.0352600815865,93.8,-103.466254328336));
#59682=CARTESIAN_POINT('',(-39.0352600815865,93.8,-103.466254328336));
#59683=CARTESIAN_POINT('',(-36.7801285362752,93.8,-101.66411253406));
#59684=CARTESIAN_POINT('',(-30.2289424908907,93.8,-101.543035544161));
#59685=CARTESIAN_POINT('',(-29.795807688482,93.8,-104.397107648414));
#59686=CARTESIAN_POINT('',(-30.2289424908907,93.8,-101.543035544161));
#59687=CARTESIAN_POINT('',(-32.9172088386108,93.8,-100.491105234184));
#59688=CARTESIAN_POINT('',(-32.9172088386108,93.8,-100.491105234184));
#59689=CARTESIAN_POINT('',(-35.1723403839221,93.8,-102.293247028459));
#59690=CARTESIAN_POINT('',(-35.1723403839221,93.8,-102.293247028459));
#59691=CARTESIAN_POINT('',(-34.7392055815134,93.8,-105.147319132713));
#59692=CARTESIAN_POINT('',(-34.7392055815134,93.8,-105.147319132713));
#59693=CARTESIAN_POINT('',(-32.0509392337934,93.8,-106.19924944269));
#59694=CARTESIAN_POINT('',(-32.0509392337934,93.8,-106.19924944269));
#59695=CARTESIAN_POINT('',(-29.795807688482,93.8,-104.397107648414));
#59696=CARTESIAN_POINT('',(5.81797897452228,93.8,-122.623107955478));
#59697=CARTESIAN_POINT('',(6.251113776931,93.8,-125.477180059731));
#59698=CARTESIAN_POINT('',(5.81797897452228,93.8,-122.623107955478));
#59699=CARTESIAN_POINT('',(3.12971262680227,93.8,-121.5711776455));
#59700=CARTESIAN_POINT('',(3.12971262680227,93.8,-121.5711776455));
#59701=CARTESIAN_POINT('',(0.874581081490917,93.8,-123.373319439776));
#59702=CARTESIAN_POINT('',(0.874581081490917,93.8,-123.373319439776));
#59703=CARTESIAN_POINT('',(1.30771588389965,93.8,-126.227391544029));
#59704=CARTESIAN_POINT('',(1.30771588389965,93.8,-126.227391544029));
#59705=CARTESIAN_POINT('',(3.99598223161968,93.8,-127.279321854006));
#59706=CARTESIAN_POINT('',(3.99598223161968,93.8,-127.279321854006));
#59707=CARTESIAN_POINT('',(6.251113776931,93.8,-125.477180059731));
#59708=CARTESIAN_POINT('',(-1.16634187327085,93.8,-119.890112841124));
#59709=CARTESIAN_POINT('',(-0.733207070862132,93.8,-122.744184945377));
#59710=CARTESIAN_POINT('',(-1.16634187327085,93.8,-119.890112841124));
#59711=CARTESIAN_POINT('',(-3.85460822099086,93.8,-118.838182531146));
#59712=CARTESIAN_POINT('',(-3.85460822099086,93.8,-118.838182531146));
#59713=CARTESIAN_POINT('',(-6.10973976630222,93.8,-120.640324325422));
#59714=CARTESIAN_POINT('',(-6.10973976630222,93.8,-120.640324325422));
#59715=CARTESIAN_POINT('',(-5.67660496389348,93.8,-123.494396429675));
#59716=CARTESIAN_POINT('',(-5.67660496389348,93.8,-123.494396429675));
#59717=CARTESIAN_POINT('',(-2.98833861617346,93.8,-124.546326739653));
#59718=CARTESIAN_POINT('',(-2.98833861617346,93.8,-124.546326739653));
#59719=CARTESIAN_POINT('',(-0.733207070862132,93.8,-122.744184945377));
#59720=CARTESIAN_POINT('',(-8.15066272106398,93.8,-117.15711772677));
#59721=CARTESIAN_POINT('',(-7.71752791865526,93.8,-120.011189831023));
#59722=CARTESIAN_POINT('',(-8.15066272106398,93.8,-117.15711772677));
#59723=CARTESIAN_POINT('',(-10.838929068784,93.8,-116.105187416792));
#59724=CARTESIAN_POINT('',(-10.838929068784,93.8,-116.105187416792));
#59725=CARTESIAN_POINT('',(-13.0940606140953,93.8,-117.907329211068));
#59726=CARTESIAN_POINT('',(-13.0940606140953,93.8,-117.907329211068));
#59727=CARTESIAN_POINT('',(-12.6609258116866,93.8,-120.761401315321));
#59728=CARTESIAN_POINT('',(-12.6609258116866,93.8,-120.761401315321));
#59729=CARTESIAN_POINT('',(-9.97265946396659,93.8,-121.813331625299));
#59730=CARTESIAN_POINT('',(-9.97265946396659,93.8,-121.813331625299));
#59731=CARTESIAN_POINT('',(-7.71752791865526,93.8,-120.011189831023));
#59732=CARTESIAN_POINT('',(-15.1349835688571,93.8,-114.424122612416));
#59733=CARTESIAN_POINT('',(-14.7018487664484,93.8,-117.278194716669));
#59734=CARTESIAN_POINT('',(-15.1349835688571,93.8,-114.424122612416));
#59735=CARTESIAN_POINT('',(-17.8232499165771,93.8,-113.372192302439));
#59736=CARTESIAN_POINT('',(-17.8232499165771,93.8,-113.372192302439));
#59737=CARTESIAN_POINT('',(-20.0783814618885,93.8,-115.174334096714));
#59738=CARTESIAN_POINT('',(-20.0783814618885,93.8,-115.174334096714));
#59739=CARTESIAN_POINT('',(-19.6452466594797,93.8,-118.028406200967));
#59740=CARTESIAN_POINT('',(-19.6452466594797,93.8,-118.028406200967));
#59741=CARTESIAN_POINT('',(-16.9569803117597,93.8,-119.080336510945));
#59742=CARTESIAN_POINT('',(-16.9569803117597,93.8,-119.080336510945));
#59743=CARTESIAN_POINT('',(-14.7018487664484,93.8,-117.278194716669));
#59744=CARTESIAN_POINT('',(-5.66761077906036,93.8,-90.2297254829355));
#59745=CARTESIAN_POINT('',(-5.23447597665164,93.8,-93.0837975871887));
#59746=CARTESIAN_POINT('',(-5.66761077906036,93.8,-90.2297254829355));
#59747=CARTESIAN_POINT('',(-8.35587712678037,93.8,-89.1777951729581));
#59748=CARTESIAN_POINT('',(-8.35587712678037,93.8,-89.1777951729581));
#59749=CARTESIAN_POINT('',(-10.6110086720917,93.8,-90.9799369672338));
#59750=CARTESIAN_POINT('',(-10.6110086720917,93.8,-90.9799369672338));
#59751=CARTESIAN_POINT('',(-10.177873869683,93.8,-93.8340090714869));
#59752=CARTESIAN_POINT('',(-10.177873869683,93.8,-93.8340090714869));
#59753=CARTESIAN_POINT('',(-7.48960752196297,93.8,-94.8859393814643));
#59754=CARTESIAN_POINT('',(-7.48960752196297,93.8,-94.8859393814643));
#59755=CARTESIAN_POINT('',(-5.23447597665164,93.8,-93.0837975871887));
#59756=CARTESIAN_POINT('',(-12.6519316268535,93.8,-87.4967303685817));
#59757=CARTESIAN_POINT('',(-12.2187968244448,93.8,-90.3508024728348));
#59758=CARTESIAN_POINT('',(-12.6519316268535,93.8,-87.4967303685817));
#59759=CARTESIAN_POINT('',(-15.3401979745735,93.8,-86.4448000586042));
#59760=CARTESIAN_POINT('',(-15.3401979745735,93.8,-86.4448000586042));
#59761=CARTESIAN_POINT('',(-17.5953295198849,93.8,-88.2469418528799));
#59762=CARTESIAN_POINT('',(-17.5953295198849,93.8,-88.2469418528799));
#59763=CARTESIAN_POINT('',(-17.1621947174761,93.8,-91.101013957133));
#59764=CARTESIAN_POINT('',(-17.1621947174761,93.8,-91.101013957133));
#59765=CARTESIAN_POINT('',(-14.4739283697561,93.8,-92.1529442671104));
#59766=CARTESIAN_POINT('',(-14.4739283697561,93.8,-92.1529442671104));
#59767=CARTESIAN_POINT('',(-12.2187968244448,93.8,-90.3508024728348));
#59768=CARTESIAN_POINT('',(-19.6362524746466,93.8,-84.7637352542278));
#59769=CARTESIAN_POINT('',(-19.2031176722379,93.8,-87.6178073584809));
#59770=CARTESIAN_POINT('',(-19.6362524746466,93.8,-84.7637352542278));
#59771=CARTESIAN_POINT('',(-22.3245188223666,93.8,-83.7118049442504));
#59772=CARTESIAN_POINT('',(-22.3245188223666,93.8,-83.7118049442504));
#59773=CARTESIAN_POINT('',(-24.579650367678,93.8,-85.5139467385261));
#59774=CARTESIAN_POINT('',(-24.579650367678,93.8,-85.5139467385261));
#59775=CARTESIAN_POINT('',(-24.1465155652693,93.8,-88.3680188427791));
#59776=CARTESIAN_POINT('',(-24.1465155652693,93.8,-88.3680188427791));
#59777=CARTESIAN_POINT('',(-21.4582492175492,93.8,-89.4199491527566));
#59778=CARTESIAN_POINT('',(-21.4582492175492,93.8,-89.4199491527566));
#59779=CARTESIAN_POINT('',(-19.2031176722379,93.8,-87.6178073584809));
#59780=CARTESIAN_POINT('',(-26.6205733224398,93.8,-82.0307401398739));
#59781=CARTESIAN_POINT('',(-26.187438520031,93.8,-84.884812244127));
#59782=CARTESIAN_POINT('',(-26.6205733224398,93.8,-82.0307401398739));
#59783=CARTESIAN_POINT('',(-29.3088396701598,93.8,-80.9788098298965));
#59784=CARTESIAN_POINT('',(-29.3088396701598,93.8,-80.9788098298965));
#59785=CARTESIAN_POINT('',(-31.5639712154711,93.8,-82.7809516241722));
#59786=CARTESIAN_POINT('',(-31.5639712154711,93.8,-82.7809516241722));
#59787=CARTESIAN_POINT('',(-31.1308364130624,93.8,-85.6350237284252));
#59788=CARTESIAN_POINT('',(-31.1308364130624,93.8,-85.6350237284252));
#59789=CARTESIAN_POINT('',(-28.4425700653424,93.8,-86.6869540384027));
#59790=CARTESIAN_POINT('',(-28.4425700653424,93.8,-86.6869540384027));
#59791=CARTESIAN_POINT('',(-26.187438520031,93.8,-84.884812244127));
#59792=CARTESIAN_POINT('',(37.3636315341458,93.8,-114.042793008606));
#59793=CARTESIAN_POINT('',(37.7967663365545,93.8,-116.896865112859));
#59794=CARTESIAN_POINT('',(37.3636315341458,93.8,-114.042793008606));
#59795=CARTESIAN_POINT('',(34.6753651864258,93.8,-112.990862698629));
#59796=CARTESIAN_POINT('',(34.6753651864258,93.8,-112.990862698629));
#59797=CARTESIAN_POINT('',(32.4202336411144,93.8,-114.793004492904));
#59798=CARTESIAN_POINT('',(32.4202336411144,93.8,-114.793004492904));
#59799=CARTESIAN_POINT('',(32.8533684435232,93.8,-117.647076597157));
#59800=CARTESIAN_POINT('',(32.8533684435232,93.8,-117.647076597157));
#59801=CARTESIAN_POINT('',(35.5416347912432,93.8,-118.699006907135));
#59802=CARTESIAN_POINT('',(35.5416347912432,93.8,-118.699006907135));
#59803=CARTESIAN_POINT('',(37.7967663365545,93.8,-116.896865112859));
#59804=CARTESIAN_POINT('',(-47.5735358658191,93.8,-73.8317547968122));
#59805=CARTESIAN_POINT('',(-47.1404010634104,93.8,-76.6858269010653));
#59806=CARTESIAN_POINT('',(-47.5735358658191,93.8,-73.8317547968122));
#59807=CARTESIAN_POINT('',(-50.2618022135392,93.8,-72.7798244868348));
#59808=CARTESIAN_POINT('',(-50.2618022135392,93.8,-72.7798244868348));
#59809=CARTESIAN_POINT('',(-52.5169337588505,93.8,-74.5819662811105));
#59810=CARTESIAN_POINT('',(-52.5169337588505,93.8,-74.5819662811105));
#59811=CARTESIAN_POINT('',(-52.0837989564418,93.8,-77.4360383853636));
#59812=CARTESIAN_POINT('',(-52.0837989564418,93.8,-77.4360383853636));
#59813=CARTESIAN_POINT('',(-49.3955326087217,93.8,-78.487968695341));
#59814=CARTESIAN_POINT('',(-49.3955326087217,93.8,-78.487968695341));
#59815=CARTESIAN_POINT('',(-47.1404010634104,93.8,-76.6858269010653));
#59816=CARTESIAN_POINT('',(-40.589215018026,93.8,-76.5647499111661));
#59817=CARTESIAN_POINT('',(-40.1560802156173,93.8,-79.4188220154192));
#59818=CARTESIAN_POINT('',(-40.589215018026,93.8,-76.5647499111661));
#59819=CARTESIAN_POINT('',(-43.277481365746,93.8,-75.5128196011887));
#59820=CARTESIAN_POINT('',(-43.277481365746,93.8,-75.5128196011887));
#59821=CARTESIAN_POINT('',(-45.5326129110574,93.8,-77.3149613954644));
#59822=CARTESIAN_POINT('',(-45.5326129110574,93.8,-77.3149613954644));
#59823=CARTESIAN_POINT('',(-45.0994781086486,93.8,-80.1690334997174));
#59824=CARTESIAN_POINT('',(-45.0994781086486,93.8,-80.1690334997174));
#59825=CARTESIAN_POINT('',(-42.4112117609286,93.8,-81.2209638096949));
#59826=CARTESIAN_POINT('',(-42.4112117609286,93.8,-81.2209638096949));
#59827=CARTESIAN_POINT('',(-40.1560802156173,93.8,-79.4188220154192));
#59828=CARTESIAN_POINT('',(-33.6048941702329,93.8,-79.29774502552));
#59829=CARTESIAN_POINT('',(-33.1717593678242,93.8,-82.1518171297731));
#59830=CARTESIAN_POINT('',(-33.6048941702329,93.8,-79.29774502552));
#59831=CARTESIAN_POINT('',(-36.2931605179529,93.8,-78.2458147155426));
#59832=CARTESIAN_POINT('',(-36.2931605179529,93.8,-78.2458147155426));
#59833=CARTESIAN_POINT('',(-38.5482920632642,93.8,-80.0479565098183));
#59834=CARTESIAN_POINT('',(-38.5482920632642,93.8,-80.0479565098183));
#59835=CARTESIAN_POINT('',(-38.1151572608555,93.8,-82.9020286140714));
#59836=CARTESIAN_POINT('',(-38.1151572608555,93.8,-82.9020286140714));
#59837=CARTESIAN_POINT('',(-35.4268909131355,93.8,-83.9539589240488));
#59838=CARTESIAN_POINT('',(-35.4268909131355,93.8,-83.9539589240488));
#59839=CARTESIAN_POINT('',(-33.1717593678242,93.8,-82.1518171297731));
#59840=CARTESIAN_POINT('',(29.2539934599053,93.8,-103.894701054705));
#59841=CARTESIAN_POINT('',(29.687128262314,93.8,-106.748773158958));
#59842=CARTESIAN_POINT('',(29.2539934599053,93.8,-103.894701054705));
#59843=CARTESIAN_POINT('',(26.5657271121853,93.8,-102.842770744728));
#59844=CARTESIAN_POINT('',(26.5657271121853,93.8,-102.842770744728));
#59845=CARTESIAN_POINT('',(24.3105955668739,93.8,-104.644912539003));
#59846=CARTESIAN_POINT('',(24.3105955668739,93.8,-104.644912539003));
#59847=CARTESIAN_POINT('',(24.7437303692827,93.8,-107.498984643256));
#59848=CARTESIAN_POINT('',(24.7437303692827,93.8,-107.498984643256));
#59849=CARTESIAN_POINT('',(27.4319967170027,93.8,-108.550914953234));
#59850=CARTESIAN_POINT('',(27.4319967170027,93.8,-108.550914953234));
#59851=CARTESIAN_POINT('',(29.687128262314,93.8,-106.748773158958));
#59852=CARTESIAN_POINT('',(36.2383143076984,93.8,-106.627696169059));
#59853=CARTESIAN_POINT('',(36.6714491101071,93.8,-109.481768273312));
#59854=CARTESIAN_POINT('',(36.2383143076984,93.8,-106.627696169059));
#59855=CARTESIAN_POINT('',(33.5500479599784,93.8,-105.575765859081));
#59856=CARTESIAN_POINT('',(33.5500479599784,93.8,-105.575765859081));
#59857=CARTESIAN_POINT('',(31.2949164146671,93.8,-107.377907653357));
#59858=CARTESIAN_POINT('',(31.2949164146671,93.8,-107.377907653357));
#59859=CARTESIAN_POINT('',(31.7280512170758,93.8,-110.23197975761));
#59860=CARTESIAN_POINT('',(31.7280512170758,93.8,-110.23197975761));
#59861=CARTESIAN_POINT('',(34.4163175647958,93.8,-111.283910067588));
#59862=CARTESIAN_POINT('',(34.4163175647958,93.8,-111.283910067588));
#59863=CARTESIAN_POINT('',(36.6714491101071,93.8,-109.481768273312));
#59864=CARTESIAN_POINT('',(43.2226351554916,93.8,-109.360691283413));
#59865=CARTESIAN_POINT('',(43.6557699579003,93.8,-112.214763387666));
#59866=CARTESIAN_POINT('',(43.2226351554916,93.8,-109.360691283413));
#59867=CARTESIAN_POINT('',(40.5343688077715,93.8,-108.308760973435));
#59868=CARTESIAN_POINT('',(40.5343688077715,93.8,-108.308760973435));
#59869=CARTESIAN_POINT('',(38.2792372624602,93.8,-110.110902767711));
#59870=CARTESIAN_POINT('',(38.2792372624602,93.8,-110.110902767711));
#59871=CARTESIAN_POINT('',(38.7123720648689,93.8,-112.964974871964));
#59872=CARTESIAN_POINT('',(38.7123720648689,93.8,-112.964974871964));
#59873=CARTESIAN_POINT('',(41.4006384125889,93.8,-114.016905181942));
#59874=CARTESIAN_POINT('',(41.4006384125889,93.8,-114.016905181942));
#59875=CARTESIAN_POINT('',(43.6557699579003,93.8,-112.214763387666));
#59876=CARTESIAN_POINT('',(-48.6988530922665,93.8,-66.4166579572652));
#59877=CARTESIAN_POINT('',(-48.2657182898578,93.8,-69.2707300615183));
#59878=CARTESIAN_POINT('',(-48.6988530922665,93.8,-66.4166579572652));
#59879=CARTESIAN_POINT('',(-51.3871194399865,93.8,-65.3647276472878));
#59880=CARTESIAN_POINT('',(-51.3871194399865,93.8,-65.3647276472878));
#59881=CARTESIAN_POINT('',(-53.6422509852979,93.8,-67.1668694415634));
#59882=CARTESIAN_POINT('',(-53.6422509852979,93.8,-67.1668694415634));
#59883=CARTESIAN_POINT('',(-53.2091161828892,93.8,-70.0209415458165));
#59884=CARTESIAN_POINT('',(-53.2091161828892,93.8,-70.0209415458165));
#59885=CARTESIAN_POINT('',(-50.5208498351691,93.8,-71.0728718557939));
#59886=CARTESIAN_POINT('',(-50.5208498351691,93.8,-71.0728718557939));
#59887=CARTESIAN_POINT('',(-48.2657182898578,93.8,-69.2707300615183));
#59888=CARTESIAN_POINT('',(22.2696726121122,93.8,-101.161705940351));
#59889=CARTESIAN_POINT('',(22.7028074145209,93.8,-104.015778044604));
#59890=CARTESIAN_POINT('',(22.2696726121122,93.8,-101.161705940351));
#59891=CARTESIAN_POINT('',(19.5814062643922,93.8,-100.109775630374));
#59892=CARTESIAN_POINT('',(19.5814062643922,93.8,-100.109775630374));
#59893=CARTESIAN_POINT('',(17.3262747190808,93.8,-101.911917424649));
#59894=CARTESIAN_POINT('',(17.3262747190808,93.8,-101.911917424649));
#59895=CARTESIAN_POINT('',(17.7594095214895,93.8,-104.765989528902));
#59896=CARTESIAN_POINT('',(17.7594095214895,93.8,-104.765989528902));
#59897=CARTESIAN_POINT('',(20.4476758692096,93.8,-105.81791983888));
#59898=CARTESIAN_POINT('',(20.4476758692096,93.8,-105.81791983888));
#59899=CARTESIAN_POINT('',(22.7028074145209,93.8,-104.015778044604));
#59900=CARTESIAN_POINT('',(15.285351764319,93.8,-98.4287108259972));
#59901=CARTESIAN_POINT('',(15.7184865667278,93.8,-101.28278293025));
#59902=CARTESIAN_POINT('',(15.285351764319,93.8,-98.4287108259972));
#59903=CARTESIAN_POINT('',(12.597085416599,93.8,-97.3767805160198));
#59904=CARTESIAN_POINT('',(12.597085416599,93.8,-97.3767805160198));
#59905=CARTESIAN_POINT('',(10.3419538712877,93.8,-99.1789223102955));
#59906=CARTESIAN_POINT('',(10.3419538712877,93.8,-99.1789223102955));
#59907=CARTESIAN_POINT('',(10.7750886736964,93.8,-102.032994414549));
#59908=CARTESIAN_POINT('',(10.7750886736964,93.8,-102.032994414549));
#59909=CARTESIAN_POINT('',(13.4633550214164,93.8,-103.084924724526));
#59910=CARTESIAN_POINT('',(13.4633550214164,93.8,-103.084924724526));
#59911=CARTESIAN_POINT('',(15.7184865667278,93.8,-101.28278293025));
#59912=CARTESIAN_POINT('',(8.3010309165259,93.8,-95.6957157116433));
#59913=CARTESIAN_POINT('',(8.73416571893462,93.8,-98.5497878158964));
#59914=CARTESIAN_POINT('',(8.3010309165259,93.8,-95.6957157116433));
#59915=CARTESIAN_POINT('',(5.6127645688059,93.8,-94.6437854016659));
#59916=CARTESIAN_POINT('',(5.6127645688059,93.8,-94.6437854016659));
#59917=CARTESIAN_POINT('',(3.35763302349454,93.8,-96.4459271959416));
#59918=CARTESIAN_POINT('',(3.35763302349454,93.8,-96.4459271959416));
#59919=CARTESIAN_POINT('',(3.79076782590327,93.8,-99.2999993001947));
#59920=CARTESIAN_POINT('',(3.79076782590327,93.8,-99.2999993001947));
#59921=CARTESIAN_POINT('',(6.4790341736233,93.8,-100.351929610172));
#59922=CARTESIAN_POINT('',(6.4790341736233,93.8,-100.351929610172));
#59923=CARTESIAN_POINT('',(8.73416571893462,93.8,-98.5497878158964));
#59924=CARTESIAN_POINT('',(1.31671006873277,93.8,-92.9627205972894));
#59925=CARTESIAN_POINT('',(1.74984487114149,93.8,-95.8167927015425));
#59926=CARTESIAN_POINT('',(1.31671006873277,93.8,-92.9627205972894));
#59927=CARTESIAN_POINT('',(-1.37155627898724,93.8,-91.910790287312));
#59928=CARTESIAN_POINT('',(-1.37155627898724,93.8,-91.910790287312));
#59929=CARTESIAN_POINT('',(-3.6266878242986,93.8,-93.7129320815877));
#59930=CARTESIAN_POINT('',(-3.6266878242986,93.8,-93.7129320815877));
#59931=CARTESIAN_POINT('',(-3.19355302188986,93.8,-96.5670041858408));
#59932=CARTESIAN_POINT('',(-3.19355302188986,93.8,-96.5670041858408));
#59933=CARTESIAN_POINT('',(-0.505286674169835,93.8,-97.6189344958182));
#59934=CARTESIAN_POINT('',(-0.505286674169835,93.8,-97.6189344958182));
#59935=CARTESIAN_POINT('',(1.74984487114149,93.8,-95.8167927015425));
#59936=CARTESIAN_POINT('',(10.5516653694206,93.8,-110.525909390737));
#59937=CARTESIAN_POINT('',(10.9848001718294,93.8,-113.379981494991));
#59938=CARTESIAN_POINT('',(10.5516653694206,93.8,-110.525909390737));
#59939=CARTESIAN_POINT('',(7.86339902170064,93.8,-109.47397908076));
#59940=CARTESIAN_POINT('',(7.86339902170064,93.8,-109.47397908076));
#59941=CARTESIAN_POINT('',(5.60826747638928,93.8,-111.276120875036));
#59942=CARTESIAN_POINT('',(5.60826747638928,93.8,-111.276120875036));
#59943=CARTESIAN_POINT('',(6.04140227879801,93.8,-114.130192979289));
#59944=CARTESIAN_POINT('',(6.04140227879801,93.8,-114.130192979289));
#59945=CARTESIAN_POINT('',(8.72966862651804,93.8,-115.182123289266));
#59946=CARTESIAN_POINT('',(8.72966862651804,93.8,-115.182123289266));
#59947=CARTESIAN_POINT('',(10.9848001718294,93.8,-113.379981494991));
#59948=CARTESIAN_POINT('',(17.5359862172138,93.8,-113.258904505091));
#59949=CARTESIAN_POINT('',(17.9691210196225,93.8,-116.112976609344));
#59950=CARTESIAN_POINT('',(17.5359862172138,93.8,-113.258904505091));
#59951=CARTESIAN_POINT('',(14.8477198694938,93.8,-112.206974195114));
#59952=CARTESIAN_POINT('',(14.8477198694938,93.8,-112.206974195114));
#59953=CARTESIAN_POINT('',(12.5925883241824,93.8,-114.00911598939));
#59954=CARTESIAN_POINT('',(12.5925883241824,93.8,-114.00911598939));
#59955=CARTESIAN_POINT('',(13.0257231265911,93.8,-116.863188093643));
#59956=CARTESIAN_POINT('',(13.0257231265911,93.8,-116.863188093643));
#59957=CARTESIAN_POINT('',(15.7139894743112,93.8,-117.91511840362));
#59958=CARTESIAN_POINT('',(15.7139894743112,93.8,-117.91511840362));
#59959=CARTESIAN_POINT('',(17.9691210196225,93.8,-116.112976609344));
#59960=CARTESIAN_POINT('',(24.5203070650069,93.8,-115.991899619445));
#59961=CARTESIAN_POINT('',(24.9534418674156,93.8,-118.845971723698));
#59962=CARTESIAN_POINT('',(24.5203070650069,93.8,-115.991899619445));
#59963=CARTESIAN_POINT('',(21.8320407172869,93.8,-114.939969309468));
#59964=CARTESIAN_POINT('',(21.8320407172869,93.8,-114.939969309468));
#59965=CARTESIAN_POINT('',(19.5769091719755,93.8,-116.742111103744));
#59966=CARTESIAN_POINT('',(19.5769091719755,93.8,-116.742111103744));
#59967=CARTESIAN_POINT('',(20.0100439743843,93.8,-119.596183207997));
#59968=CARTESIAN_POINT('',(20.0100439743843,93.8,-119.596183207997));
#59969=CARTESIAN_POINT('',(22.6983103221043,93.8,-120.648113517974));
#59970=CARTESIAN_POINT('',(22.6983103221043,93.8,-120.648113517974));
#59971=CARTESIAN_POINT('',(24.9534418674156,93.8,-118.845971723698));
#59972=CARTESIAN_POINT('',(31.5046279128,93.8,-118.724894733799));
#59973=CARTESIAN_POINT('',(31.9377627152088,93.8,-121.578966838052));
#59974=CARTESIAN_POINT('',(31.5046279128,93.8,-118.724894733799));
#59975=CARTESIAN_POINT('',(28.81636156508,93.8,-117.672964423822));
#59976=CARTESIAN_POINT('',(28.81636156508,93.8,-117.672964423822));
#59977=CARTESIAN_POINT('',(26.5612300197687,93.8,-119.475106218097));
#59978=CARTESIAN_POINT('',(26.5612300197687,93.8,-119.475106218097));
#59979=CARTESIAN_POINT('',(26.9943648221774,93.8,-122.32917832235));
#59980=CARTESIAN_POINT('',(26.9943648221774,93.8,-122.32917832235));
#59981=CARTESIAN_POINT('',(29.6826311698974,93.8,-123.381108632328));
#59982=CARTESIAN_POINT('',(29.6826311698974,93.8,-123.381108632328));
#59983=CARTESIAN_POINT('',(31.9377627152088,93.8,-121.578966838052));
#59984=CARTESIAN_POINT('',(-46.4482186393718,93.8,-81.2468516363593));
#59985=CARTESIAN_POINT('',(-46.0150838369631,93.8,-84.1009237406124));
#59986=CARTESIAN_POINT('',(-46.4482186393718,93.8,-81.2468516363593));
#59987=CARTESIAN_POINT('',(-49.1364849870918,93.8,-80.1949213263819));
#59988=CARTESIAN_POINT('',(-49.1364849870918,93.8,-80.1949213263819));
#59989=CARTESIAN_POINT('',(-51.3916165324031,93.8,-81.9970631206576));
#59990=CARTESIAN_POINT('',(-51.3916165324031,93.8,-81.9970631206576));
#59991=CARTESIAN_POINT('',(-50.9584817299944,93.8,-84.8511352249106));
#59992=CARTESIAN_POINT('',(-50.9584817299944,93.8,-84.8511352249106));
#59993=CARTESIAN_POINT('',(-48.2702153822744,93.8,-85.9030655348881));
#59994=CARTESIAN_POINT('',(-48.2702153822744,93.8,-85.9030655348881));
#59995=CARTESIAN_POINT('',(-46.0150838369631,93.8,-84.1009237406124));
#59996=CARTESIAN_POINT('',(-39.4638977915786,93.8,-83.9798467507132));
#59997=CARTESIAN_POINT('',(-39.0307629891699,93.8,-86.8339188549663));
#59998=CARTESIAN_POINT('',(-39.4638977915786,93.8,-83.9798467507132));
#59999=CARTESIAN_POINT('',(-42.1521641392987,93.8,-82.9279164407358));
#60000=CARTESIAN_POINT('',(-42.1521641392987,93.8,-82.9279164407358));
#60001=CARTESIAN_POINT('',(-44.40729568461,93.8,-84.7300582350115));
#60002=CARTESIAN_POINT('',(-44.40729568461,93.8,-84.7300582350115));
#60003=CARTESIAN_POINT('',(-43.9741608822013,93.8,-87.5841303392645));
#60004=CARTESIAN_POINT('',(-43.9741608822013,93.8,-87.5841303392645));
#60005=CARTESIAN_POINT('',(-41.2858945344812,93.8,-88.636060649242));
#60006=CARTESIAN_POINT('',(-41.2858945344812,93.8,-88.636060649242));
#60007=CARTESIAN_POINT('',(-39.0307629891699,93.8,-86.8339188549663));
#60008=CARTESIAN_POINT('',(-32.4795769437855,93.8,-86.7128418650671));
#60009=CARTESIAN_POINT('',(-32.0464421413768,93.8,-89.5669139693202));
#60010=CARTESIAN_POINT('',(-32.4795769437855,93.8,-86.7128418650671));
#60011=CARTESIAN_POINT('',(-35.1678432915055,93.8,-85.6609115550896));
#60012=CARTESIAN_POINT('',(-35.1678432915055,93.8,-85.6609115550896));
#60013=CARTESIAN_POINT('',(-37.4229748368169,93.8,-87.4630533493654));
#60014=CARTESIAN_POINT('',(-37.4229748368169,93.8,-87.4630533493654));
#60015=CARTESIAN_POINT('',(-36.9898400344081,93.8,-90.3171254536184));
#60016=CARTESIAN_POINT('',(-36.9898400344081,93.8,-90.3171254536184));
#60017=CARTESIAN_POINT('',(-34.3015736866881,93.8,-91.3690557635958));
#60018=CARTESIAN_POINT('',(-34.3015736866881,93.8,-91.3690557635958));
#60019=CARTESIAN_POINT('',(-32.0464421413768,93.8,-89.5669139693202));
#60020=CARTESIAN_POINT('',(-25.4952560959924,93.8,-89.4458369794209));
#60021=CARTESIAN_POINT('',(-25.0621212935837,93.8,-92.2999090836741));
#60022=CARTESIAN_POINT('',(-25.4952560959924,93.8,-89.4458369794209));
#60023=CARTESIAN_POINT('',(-28.1835224437124,93.8,-88.3939066694435));
#60024=CARTESIAN_POINT('',(-28.1835224437124,93.8,-88.3939066694435));
#60025=CARTESIAN_POINT('',(-30.4386539890237,93.8,-90.1960484637193));
#60026=CARTESIAN_POINT('',(-30.4386539890237,93.8,-90.1960484637193));
#60027=CARTESIAN_POINT('',(-30.005519186615,93.8,-93.0501205679723));
#60028=CARTESIAN_POINT('',(-30.005519186615,93.8,-93.0501205679723));
#60029=CARTESIAN_POINT('',(-27.317252838895,93.8,-94.1020508779497));
#60030=CARTESIAN_POINT('',(-27.317252838895,93.8,-94.1020508779497));
#60031=CARTESIAN_POINT('',(-25.0621212935837,93.8,-92.2999090836741));
#60032=CARTESIAN_POINT('',(-18.5109352481993,93.8,-92.1788320937748));
#60033=CARTESIAN_POINT('',(-18.0778004457905,93.8,-95.0329041980279));
#60034=CARTESIAN_POINT('',(-18.5109352481993,93.8,-92.1788320937748));
#60035=CARTESIAN_POINT('',(-21.1992015959193,93.8,-91.1269017837974));
#60036=CARTESIAN_POINT('',(-21.1992015959193,93.8,-91.1269017837974));
#60037=CARTESIAN_POINT('',(-23.4543331412306,93.8,-92.9290435780731));
#60038=CARTESIAN_POINT('',(-23.4543331412306,93.8,-92.9290435780731));
#60039=CARTESIAN_POINT('',(-23.0211983388219,93.8,-95.7831156823262));
#60040=CARTESIAN_POINT('',(-23.0211983388219,93.8,-95.7831156823262));
#60041=CARTESIAN_POINT('',(-20.3329319911019,93.8,-96.8350459923036));
#60042=CARTESIAN_POINT('',(-20.3329319911019,93.8,-96.8350459923036));
#60043=CARTESIAN_POINT('',(-18.0778004457905,93.8,-95.0329041980279));
#60044=CARTESIAN_POINT('',(-11.5266144004061,93.8,-94.9118272081287));
#60045=CARTESIAN_POINT('',(-11.0934795979974,93.8,-97.7658993123818));
#60046=CARTESIAN_POINT('',(-11.5266144004061,93.8,-94.9118272081287));
#60047=CARTESIAN_POINT('',(-14.2148807481261,93.8,-93.8598968981513));
#60048=CARTESIAN_POINT('',(-14.2148807481261,93.8,-93.8598968981513));
#60049=CARTESIAN_POINT('',(-16.4700122934375,93.8,-95.662038692427));
#60050=CARTESIAN_POINT('',(-16.4700122934375,93.8,-95.662038692427));
#60051=CARTESIAN_POINT('',(-16.0368774910288,93.8,-98.5161107966801));
#60052=CARTESIAN_POINT('',(-16.0368774910288,93.8,-98.5161107966801));
#60053=CARTESIAN_POINT('',(-13.3486111433087,93.8,-99.5680411066575));
#60054=CARTESIAN_POINT('',(-13.3486111433087,93.8,-99.5680411066575));
#60055=CARTESIAN_POINT('',(-11.0934795979974,93.8,-97.7658993123818));
#60056=CARTESIAN_POINT('',(-4.54229355261299,93.8,-97.6448223224826));
#60057=CARTESIAN_POINT('',(-4.10915875020428,93.8,-100.498894426736));
#60058=CARTESIAN_POINT('',(-4.54229355261299,93.8,-97.6448223224826));
#60059=CARTESIAN_POINT('',(-7.230559900333,93.8,-96.5928920125052));
#60060=CARTESIAN_POINT('',(-7.230559900333,93.8,-96.5928920125052));
#60061=CARTESIAN_POINT('',(-9.48569144564436,93.8,-98.3950338067809));
#60062=CARTESIAN_POINT('',(-9.48569144564436,93.8,-98.3950338067809));
#60063=CARTESIAN_POINT('',(-9.05255664323563,93.8,-101.249105911034));
#60064=CARTESIAN_POINT('',(-9.05255664323563,93.8,-101.249105911034));
#60065=CARTESIAN_POINT('',(-6.3642902955156,93.8,-102.301036221011));
#60066=CARTESIAN_POINT('',(-6.3642902955156,93.8,-102.301036221011));
#60067=CARTESIAN_POINT('',(-4.10915875020428,93.8,-100.498894426736));
#60068=CARTESIAN_POINT('',(2.44202729518014,93.8,-100.377817436837));
#60069=CARTESIAN_POINT('',(2.87516209758886,93.8,-103.23188954109));
#60070=CARTESIAN_POINT('',(2.44202729518014,93.8,-100.377817436837));
#60071=CARTESIAN_POINT('',(-0.246239052539871,93.8,-99.3258871268591));
#60072=CARTESIAN_POINT('',(-0.246239052539871,93.8,-99.3258871268591));
#60073=CARTESIAN_POINT('',(-2.50137059785123,93.8,-101.128028921135));
#60074=CARTESIAN_POINT('',(-2.50137059785123,93.8,-101.128028921135));
#60075=CARTESIAN_POINT('',(-2.06823579544249,93.8,-103.982101025388));
#60076=CARTESIAN_POINT('',(-2.06823579544249,93.8,-103.982101025388));
#60077=CARTESIAN_POINT('',(0.620030552277533,93.8,-105.034031335365));
#60078=CARTESIAN_POINT('',(0.620030552277533,93.8,-105.034031335365));
#60079=CARTESIAN_POINT('',(2.87516209758886,93.8,-103.23188954109));
#60080=CARTESIAN_POINT('',(9.42634814297327,93.8,-103.11081255119));
#60081=CARTESIAN_POINT('',(9.85948294538199,93.8,-105.964884655444));
#60082=CARTESIAN_POINT('',(9.42634814297327,93.8,-103.11081255119));
#60083=CARTESIAN_POINT('',(6.73808179525326,93.8,-102.058882241213));
#60084=CARTESIAN_POINT('',(6.73808179525326,93.8,-102.058882241213));
#60085=CARTESIAN_POINT('',(4.48295024994191,93.8,-103.861024035489));
#60086=CARTESIAN_POINT('',(4.48295024994191,93.8,-103.861024035489));
#60087=CARTESIAN_POINT('',(4.91608505235064,93.8,-106.715096139742));
#60088=CARTESIAN_POINT('',(4.91608505235064,93.8,-106.715096139742));
#60089=CARTESIAN_POINT('',(7.60435140007067,93.8,-107.767026449719));
#60090=CARTESIAN_POINT('',(7.60435140007067,93.8,-107.767026449719));
#60091=CARTESIAN_POINT('',(9.85948294538199,93.8,-105.964884655444));
#60092=CARTESIAN_POINT('',(16.4106689907664,93.8,-105.843807665544));
#60093=CARTESIAN_POINT('',(16.8438037931751,93.8,-108.697879769797));
#60094=CARTESIAN_POINT('',(16.4106689907664,93.8,-105.843807665544));
#60095=CARTESIAN_POINT('',(13.7224026430464,93.8,-104.791877355567));
#60096=CARTESIAN_POINT('',(13.7224026430464,93.8,-104.791877355567));
#60097=CARTESIAN_POINT('',(11.467271097735,93.8,-106.594019149843));
#60098=CARTESIAN_POINT('',(11.467271097735,93.8,-106.594019149843));
#60099=CARTESIAN_POINT('',(11.9004059001438,93.8,-109.448091254096));
#60100=CARTESIAN_POINT('',(11.9004059001438,93.8,-109.448091254096));
#60101=CARTESIAN_POINT('',(14.5886722478638,93.8,-110.500021564073));
#60102=CARTESIAN_POINT('',(14.5886722478638,93.8,-110.500021564073));
#60103=CARTESIAN_POINT('',(16.8438037931751,93.8,-108.697879769797));
#60104=CARTESIAN_POINT('',(23.3949898385595,93.8,-108.576802779898));
#60105=CARTESIAN_POINT('',(23.8281246409682,93.8,-111.430874884151));
#60106=CARTESIAN_POINT('',(23.3949898385595,93.8,-108.576802779898));
#60107=CARTESIAN_POINT('',(20.7067234908395,93.8,-107.524872469921));
#60108=CARTESIAN_POINT('',(20.7067234908395,93.8,-107.524872469921));
#60109=CARTESIAN_POINT('',(18.4515919455282,93.8,-109.327014264196));
#60110=CARTESIAN_POINT('',(18.4515919455282,93.8,-109.327014264196));
#60111=CARTESIAN_POINT('',(18.8847267479369,93.8,-112.18108636845));
#60112=CARTESIAN_POINT('',(18.8847267479369,93.8,-112.18108636845));
#60113=CARTESIAN_POINT('',(21.5729930956569,93.8,-113.233016678427));
#60114=CARTESIAN_POINT('',(21.5729930956569,93.8,-113.233016678427));
#60115=CARTESIAN_POINT('',(23.8281246409682,93.8,-111.430874884151));
#60116=CARTESIAN_POINT('',(30.3793106863527,93.8,-111.309797894252));
#60117=CARTESIAN_POINT('',(30.8124454887614,93.8,-114.163869998505));
#60118=CARTESIAN_POINT('',(30.3793106863527,93.8,-111.309797894252));
#60119=CARTESIAN_POINT('',(27.6910443386327,93.8,-110.257867584275));
#60120=CARTESIAN_POINT('',(27.6910443386327,93.8,-110.257867584275));
#60121=CARTESIAN_POINT('',(25.4359127933213,93.8,-112.06000937855));
#60122=CARTESIAN_POINT('',(25.4359127933213,93.8,-112.06000937855));
#60123=CARTESIAN_POINT('',(25.86904759573,93.8,-114.914081482803));
#60124=CARTESIAN_POINT('',(25.86904759573,93.8,-114.914081482803));
#60125=CARTESIAN_POINT('',(28.5573139434501,93.8,-115.966011792781));
#60126=CARTESIAN_POINT('',(28.5573139434501,93.8,-115.966011792781));
#60127=CARTESIAN_POINT('',(30.8124454887614,93.8,-114.163869998505));
#60128=CARTESIAN_POINT('',(5.15749672629266,93.8,-31.6928392700737));
#60129=CARTESIAN_POINT('',(5.59063152870137,93.8,-34.5469113743268));
#60130=CARTESIAN_POINT('',(5.15749672629266,93.8,-31.6928392700737));
#60131=CARTESIAN_POINT('',(2.46923037857264,93.8,-30.6409089600963));
#60132=CARTESIAN_POINT('',(2.46923037857264,93.8,-30.6409089600963));
#60133=CARTESIAN_POINT('',(0.214098833261289,93.8,-32.443050754372));
#60134=CARTESIAN_POINT('',(0.214098833261289,93.8,-32.443050754372));
#60135=CARTESIAN_POINT('',(0.647233635670021,93.8,-35.2971228586251));
#60136=CARTESIAN_POINT('',(0.647233635670021,93.8,-35.2971228586251));
#60137=CARTESIAN_POINT('',(3.33549998339005,93.8,-36.3490531686025));
#60138=CARTESIAN_POINT('',(3.33549998339005,93.8,-36.3490531686025));
#60139=CARTESIAN_POINT('',(5.59063152870137,93.8,-34.5469113743268));
#60140=CARTESIAN_POINT('',(-1.82682412150048,93.8,-28.9598441557198));
#60141=CARTESIAN_POINT('',(-1.39368931909176,93.8,-31.8139162599729));
#60142=CARTESIAN_POINT('',(-1.82682412150048,93.8,-28.9598441557198));
#60143=CARTESIAN_POINT('',(-4.51509046922049,93.8,-27.9079138457424));
#60144=CARTESIAN_POINT('',(-4.51509046922049,93.8,-27.9079138457424));
#60145=CARTESIAN_POINT('',(-6.77022201453184,93.8,-29.7100556400181));
#60146=CARTESIAN_POINT('',(-6.77022201453184,93.8,-29.7100556400181));
#60147=CARTESIAN_POINT('',(-6.33708721212311,93.8,-32.5641277442712));
#60148=CARTESIAN_POINT('',(-6.33708721212311,93.8,-32.5641277442712));
#60149=CARTESIAN_POINT('',(-3.64882086440308,93.8,-33.6160580542486));
#60150=CARTESIAN_POINT('',(-3.64882086440308,93.8,-33.6160580542486));
#60151=CARTESIAN_POINT('',(-1.39368931909176,93.8,-31.8139162599729));
#60152=CARTESIAN_POINT('',(-8.81114496929361,93.8,-26.2268490413659));
#60153=CARTESIAN_POINT('',(-8.37801016688489,93.8,-29.080921145619));
#60154=CARTESIAN_POINT('',(-8.81114496929361,93.8,-26.2268490413659));
#60155=CARTESIAN_POINT('',(-11.4994113170136,93.8,-25.1749187313885));
#60156=CARTESIAN_POINT('',(-11.4994113170136,93.8,-25.1749187313885));
#60157=CARTESIAN_POINT('',(-13.754542862325,93.8,-26.9770605256642));
#60158=CARTESIAN_POINT('',(-13.754542862325,93.8,-26.9770605256642));
#60159=CARTESIAN_POINT('',(-13.3214080599162,93.8,-29.8311326299173));
#60160=CARTESIAN_POINT('',(-13.3214080599162,93.8,-29.8311326299173));
#60161=CARTESIAN_POINT('',(-10.6331417121962,93.8,-30.8830629398947));
#60162=CARTESIAN_POINT('',(-10.6331417121962,93.8,-30.8830629398947));
#60163=CARTESIAN_POINT('',(-8.37801016688489,93.8,-29.080921145619));
#60164=CARTESIAN_POINT('',(48.1887390394988,93.8,-55.5059067957441));
#60165=CARTESIAN_POINT('',(48.6218738419075,93.8,-58.3599788999972));
#60166=CARTESIAN_POINT('',(48.1887390394988,93.8,-55.5059067957441));
#60167=CARTESIAN_POINT('',(45.5004726917788,93.8,-54.4539764857667));
#60168=CARTESIAN_POINT('',(45.5004726917788,93.8,-54.4539764857667));
#60169=CARTESIAN_POINT('',(43.2453411464674,93.8,-56.2561182800424));
#60170=CARTESIAN_POINT('',(43.2453411464674,93.8,-56.2561182800424));
#60171=CARTESIAN_POINT('',(43.6784759488762,93.8,-59.1101903842955));
#60172=CARTESIAN_POINT('',(43.6784759488762,93.8,-59.1101903842955));
#60173=CARTESIAN_POINT('',(46.3667422965962,93.8,-60.1621206942729));
#60174=CARTESIAN_POINT('',(46.3667422965962,93.8,-60.1621206942729));
#60175=CARTESIAN_POINT('',(48.6218738419075,93.8,-58.3599788999972));
#60176=CARTESIAN_POINT('',(12.1418175740858,93.8,-34.4258343844276));
#60177=CARTESIAN_POINT('',(12.5749523764945,93.8,-37.2799064886807));
#60178=CARTESIAN_POINT('',(12.1418175740858,93.8,-34.4258343844276));
#60179=CARTESIAN_POINT('',(9.45355122636578,93.8,-33.3739040744502));
#60180=CARTESIAN_POINT('',(9.45355122636578,93.8,-33.3739040744502));
#60181=CARTESIAN_POINT('',(7.19841968105442,93.8,-35.1760458687259));
#60182=CARTESIAN_POINT('',(7.19841968105442,93.8,-35.1760458687259));
#60183=CARTESIAN_POINT('',(7.63155448346315,93.8,-38.030117972979));
#60184=CARTESIAN_POINT('',(7.63155448346315,93.8,-38.030117972979));
#60185=CARTESIAN_POINT('',(10.3198208311832,93.8,-39.0820482829564));
#60186=CARTESIAN_POINT('',(10.3198208311832,93.8,-39.0820482829564));
#60187=CARTESIAN_POINT('',(12.5749523764945,93.8,-37.2799064886807));
#60188=CARTESIAN_POINT('',(19.1261384218789,93.8,-37.1588294987815));
#60189=CARTESIAN_POINT('',(19.5592732242876,93.8,-40.0129016030346));
#60190=CARTESIAN_POINT('',(19.1261384218789,93.8,-37.1588294987815));
#60191=CARTESIAN_POINT('',(16.4378720741589,93.8,-36.1068991888041));
#60192=CARTESIAN_POINT('',(16.4378720741589,93.8,-36.1068991888041));
#60193=CARTESIAN_POINT('',(14.1827405288475,93.8,-37.9090409830798));
#60194=CARTESIAN_POINT('',(14.1827405288475,93.8,-37.9090409830798));
#60195=CARTESIAN_POINT('',(14.6158753312563,93.8,-40.7631130873329));
#60196=CARTESIAN_POINT('',(14.6158753312563,93.8,-40.7631130873329));
#60197=CARTESIAN_POINT('',(17.3041416789763,93.8,-41.8150433973103));
#60198=CARTESIAN_POINT('',(17.3041416789763,93.8,-41.8150433973103));
#60199=CARTESIAN_POINT('',(19.5592732242876,93.8,-40.0129016030346));
#60200=CARTESIAN_POINT('',(26.110459269672,93.8,-39.8918246131354));
#60201=CARTESIAN_POINT('',(26.5435940720808,93.8,-42.7458967173885));
#60202=CARTESIAN_POINT('',(26.110459269672,93.8,-39.8918246131354));
#60203=CARTESIAN_POINT('',(23.422192921952,93.8,-38.839894303158));
#60204=CARTESIAN_POINT('',(23.422192921952,93.8,-38.839894303158));
#60205=CARTESIAN_POINT('',(21.1670613766407,93.8,-40.6420360974337));
#60206=CARTESIAN_POINT('',(21.1670613766407,93.8,-40.6420360974337));
#60207=CARTESIAN_POINT('',(21.6001961790494,93.8,-43.4961082016867));
#60208=CARTESIAN_POINT('',(21.6001961790494,93.8,-43.4961082016867));
#60209=CARTESIAN_POINT('',(24.2884625267694,93.8,-44.5480385116642));
#60210=CARTESIAN_POINT('',(24.2884625267694,93.8,-44.5480385116642));
#60211=CARTESIAN_POINT('',(26.5435940720808,93.8,-42.7458967173885));
#60212=CARTESIAN_POINT('',(33.0947801174652,93.8,-42.6248197274893));
#60213=CARTESIAN_POINT('',(33.5279149198739,93.8,-45.4788918317424));
#60214=CARTESIAN_POINT('',(33.0947801174652,93.8,-42.6248197274893));
#60215=CARTESIAN_POINT('',(30.4065137697452,93.8,-41.5728894175119));
#60216=CARTESIAN_POINT('',(30.4065137697452,93.8,-41.5728894175119));
#60217=CARTESIAN_POINT('',(28.1513822244338,93.8,-43.3750312117876));
#60218=CARTESIAN_POINT('',(28.1513822244338,93.8,-43.3750312117876));
#60219=CARTESIAN_POINT('',(28.5845170268425,93.8,-46.2291033160406));
#60220=CARTESIAN_POINT('',(28.5845170268425,93.8,-46.2291033160406));
#60221=CARTESIAN_POINT('',(31.2727833745626,93.8,-47.2810336260181));
#60222=CARTESIAN_POINT('',(31.2727833745626,93.8,-47.2810336260181));
#60223=CARTESIAN_POINT('',(33.5279149198739,93.8,-45.4788918317424));
#60224=CARTESIAN_POINT('',(41.2044181917057,93.8,-52.7729116813902));
#60225=CARTESIAN_POINT('',(41.6375529941144,93.8,-55.6269837856433));
#60226=CARTESIAN_POINT('',(41.2044181917057,93.8,-52.7729116813902));
#60227=CARTESIAN_POINT('',(38.5161518439857,93.8,-51.7209813714128));
#60228=CARTESIAN_POINT('',(38.5161518439857,93.8,-51.7209813714128));
#60229=CARTESIAN_POINT('',(36.2610202986743,93.8,-53.5231231656885));
#60230=CARTESIAN_POINT('',(36.2610202986743,93.8,-53.5231231656885));
#60231=CARTESIAN_POINT('',(36.694155101083,93.8,-56.3771952699416));
#60232=CARTESIAN_POINT('',(36.694155101083,93.8,-56.3771952699416));
#60233=CARTESIAN_POINT('',(39.3824214488031,93.8,-57.429125579919));
#60234=CARTESIAN_POINT('',(39.3824214488031,93.8,-57.429125579919));
#60235=CARTESIAN_POINT('',(41.6375529941144,93.8,-55.6269837856433));
#60236=CARTESIAN_POINT('',(34.2200973439125,93.8,-50.0399165670363));
#60237=CARTESIAN_POINT('',(34.6532321463213,93.8,-52.8939886712894));
#60238=CARTESIAN_POINT('',(34.2200973439125,93.8,-50.0399165670363));
#60239=CARTESIAN_POINT('',(31.5318309961925,93.8,-48.9879862570589));
#60240=CARTESIAN_POINT('',(31.5318309961925,93.8,-48.9879862570589));
#60241=CARTESIAN_POINT('',(29.2766994508812,93.8,-50.7901280513346));
#60242=CARTESIAN_POINT('',(29.2766994508812,93.8,-50.7901280513346));
#60243=CARTESIAN_POINT('',(29.7098342532899,93.8,-53.6442001555877));
#60244=CARTESIAN_POINT('',(29.7098342532899,93.8,-53.6442001555877));
#60245=CARTESIAN_POINT('',(32.3981006010099,93.8,-54.6961304655651));
#60246=CARTESIAN_POINT('',(32.3981006010099,93.8,-54.6961304655651));
#60247=CARTESIAN_POINT('',(34.6532321463213,93.8,-52.8939886712894));
#60248=CARTESIAN_POINT('',(27.2357764961194,93.8,-47.3069214526824));
#60249=CARTESIAN_POINT('',(27.6689112985281,93.8,-50.1609935569356));
#60250=CARTESIAN_POINT('',(27.2357764961194,93.8,-47.3069214526824));
#60251=CARTESIAN_POINT('',(24.5475101483994,93.8,-46.254991142705));
#60252=CARTESIAN_POINT('',(24.5475101483994,93.8,-46.254991142705));
#60253=CARTESIAN_POINT('',(22.2923786030881,93.8,-48.0571329369807));
#60254=CARTESIAN_POINT('',(22.2923786030881,93.8,-48.0571329369807));
#60255=CARTESIAN_POINT('',(22.7255134054968,93.8,-50.9112050412338));
#60256=CARTESIAN_POINT('',(22.7255134054968,93.8,-50.9112050412338));
#60257=CARTESIAN_POINT('',(25.4137797532168,93.8,-51.9631353512112));
#60258=CARTESIAN_POINT('',(25.4137797532168,93.8,-51.9631353512112));
#60259=CARTESIAN_POINT('',(27.6689112985281,93.8,-50.1609935569356));
#60260=CARTESIAN_POINT('',(20.2514556483263,93.8,-44.5739263383286));
#60261=CARTESIAN_POINT('',(20.684590450735,93.8,-47.4279984425817));
#60262=CARTESIAN_POINT('',(20.2514556483263,93.8,-44.5739263383286));
#60263=CARTESIAN_POINT('',(17.5631893006063,93.8,-43.5219960283511));
#60264=CARTESIAN_POINT('',(17.5631893006063,93.8,-43.5219960283511));
#60265=CARTESIAN_POINT('',(15.3080577552949,93.8,-45.3241378226269));
#60266=CARTESIAN_POINT('',(15.3080577552949,93.8,-45.3241378226269));
#60267=CARTESIAN_POINT('',(15.7411925577037,93.8,-48.1782099268799));
#60268=CARTESIAN_POINT('',(15.7411925577037,93.8,-48.1782099268799));
#60269=CARTESIAN_POINT('',(18.4294589054237,93.8,-49.2301402368573));
#60270=CARTESIAN_POINT('',(18.4294589054237,93.8,-49.2301402368573));
#60271=CARTESIAN_POINT('',(20.684590450735,93.8,-47.4279984425817));
#60272=CARTESIAN_POINT('',(13.2671348005332,93.8,-41.8409312239747));
#60273=CARTESIAN_POINT('',(13.7002696029419,93.8,-44.6950033282278));
#60274=CARTESIAN_POINT('',(13.2671348005332,93.8,-41.8409312239747));
#60275=CARTESIAN_POINT('',(10.5788684528132,93.8,-40.7890009139973));
#60276=CARTESIAN_POINT('',(10.5788684528132,93.8,-40.7890009139973));
#60277=CARTESIAN_POINT('',(8.32373690750179,93.8,-42.591142708273));
#60278=CARTESIAN_POINT('',(8.32373690750179,93.8,-42.591142708273));
#60279=CARTESIAN_POINT('',(8.75687170991053,93.8,-45.445214812526));
#60280=CARTESIAN_POINT('',(8.75687170991053,93.8,-45.445214812526));
#60281=CARTESIAN_POINT('',(11.4451380576306,93.8,-46.4971451225034));
#60282=CARTESIAN_POINT('',(11.4451380576306,93.8,-46.4971451225034));
#60283=CARTESIAN_POINT('',(13.7002696029419,93.8,-44.6950033282278));
#60284=CARTESIAN_POINT('',(6.28281395274003,93.8,-39.1079361096208));
#60285=CARTESIAN_POINT('',(6.71594875514875,93.8,-41.9620082138739));
#60286=CARTESIAN_POINT('',(6.28281395274003,93.8,-39.1079361096208));
#60287=CARTESIAN_POINT('',(3.59454760502002,93.8,-38.0560057996434));
#60288=CARTESIAN_POINT('',(3.59454760502002,93.8,-38.0560057996434));
#60289=CARTESIAN_POINT('',(1.33941605970866,93.8,-39.8581475939191));
#60290=CARTESIAN_POINT('',(1.33941605970866,93.8,-39.8581475939191));
#60291=CARTESIAN_POINT('',(1.7725508621174,93.8,-42.7122196981721));
#60292=CARTESIAN_POINT('',(1.7725508621174,93.8,-42.7122196981721));
#60293=CARTESIAN_POINT('',(4.46081720983742,93.8,-43.7641500081495));
#60294=CARTESIAN_POINT('',(4.46081720983742,93.8,-43.7641500081495));
#60295=CARTESIAN_POINT('',(6.71594875514875,93.8,-41.9620082138739));
#60296=CARTESIAN_POINT('',(-0.701506895053102,93.8,-36.3749409952669));
#60297=CARTESIAN_POINT('',(-0.268372092644385,93.8,-39.22901309952));
#60298=CARTESIAN_POINT('',(-0.701506895053102,93.8,-36.3749409952669));
#60299=CARTESIAN_POINT('',(-3.38977324277311,93.8,-35.3230106852895));
#60300=CARTESIAN_POINT('',(-3.38977324277311,93.8,-35.3230106852895));
#60301=CARTESIAN_POINT('',(-5.64490478808447,93.8,-37.1251524795652));
#60302=CARTESIAN_POINT('',(-5.64490478808447,93.8,-37.1251524795652));
#60303=CARTESIAN_POINT('',(-5.21176998567574,93.8,-39.9792245838182));
#60304=CARTESIAN_POINT('',(-5.21176998567574,93.8,-39.9792245838182));
#60305=CARTESIAN_POINT('',(-2.52350363795571,93.8,-41.0311548937957));
#60306=CARTESIAN_POINT('',(-2.52350363795571,93.8,-41.0311548937957));
#60307=CARTESIAN_POINT('',(-0.268372092644385,93.8,-39.22901309952));
#60308=CARTESIAN_POINT('',(-7.68582774284623,93.8,-33.641945880913));
#60309=CARTESIAN_POINT('',(-7.25269294043752,93.8,-36.4960179851661));
#60310=CARTESIAN_POINT('',(-7.68582774284623,93.8,-33.641945880913));
#60311=CARTESIAN_POINT('',(-10.3740940905662,93.8,-32.5900155709356));
#60312=CARTESIAN_POINT('',(-10.3740940905662,93.8,-32.5900155709356));
#60313=CARTESIAN_POINT('',(-12.6292256358776,93.8,-34.3921573652113));
#60314=CARTESIAN_POINT('',(-12.6292256358776,93.8,-34.3921573652113));
#60315=CARTESIAN_POINT('',(-12.1960908334689,93.8,-37.2462294694643));
#60316=CARTESIAN_POINT('',(-12.1960908334689,93.8,-37.2462294694643));
#60317=CARTESIAN_POINT('',(-9.50782448574884,93.8,-38.2981597794418));
#60318=CARTESIAN_POINT('',(-9.50782448574884,93.8,-38.2981597794418));
#60319=CARTESIAN_POINT('',(-7.25269294043752,93.8,-36.4960179851661));
#60320=CARTESIAN_POINT('',(38.9537837388109,93.8,-37.9427180022961));
#60321=CARTESIAN_POINT('',(39.3869185412196,93.8,-40.7967901065492));
#60322=CARTESIAN_POINT('',(38.9537837388109,93.8,-37.9427180022961));
#60323=CARTESIAN_POINT('',(36.2655173910909,93.8,-36.8907876923187));
#60324=CARTESIAN_POINT('',(36.2655173910909,93.8,-36.8907876923187));
#60325=CARTESIAN_POINT('',(34.0103858457796,93.8,-38.6929294865944));
#60326=CARTESIAN_POINT('',(34.0103858457796,93.8,-38.6929294865944));
#60327=CARTESIAN_POINT('',(34.4435206481883,93.8,-41.5470015908475));
#60328=CARTESIAN_POINT('',(34.4435206481883,93.8,-41.5470015908475));
#60329=CARTESIAN_POINT('',(37.1317869959083,93.8,-42.5989319008249));
#60330=CARTESIAN_POINT('',(37.1317869959083,93.8,-42.5989319008249));
#60331=CARTESIAN_POINT('',(39.3869185412196,93.8,-40.7967901065492));
#60332=CARTESIAN_POINT('',(31.9694628910178,93.8,-35.2097228879422));
#60333=CARTESIAN_POINT('',(32.4025976934265,93.8,-38.0637949921953));
#60334=CARTESIAN_POINT('',(31.9694628910178,93.8,-35.2097228879422));
#60335=CARTESIAN_POINT('',(29.2811965432978,93.8,-34.1577925779648));
#60336=CARTESIAN_POINT('',(29.2811965432978,93.8,-34.1577925779648));
#60337=CARTESIAN_POINT('',(27.0260649979864,93.8,-35.9599343722405));
#60338=CARTESIAN_POINT('',(27.0260649979864,93.8,-35.9599343722405));
#60339=CARTESIAN_POINT('',(27.4591998003952,93.8,-38.8140064764936));
#60340=CARTESIAN_POINT('',(27.4591998003952,93.8,-38.8140064764936));
#60341=CARTESIAN_POINT('',(30.1474661481152,93.8,-39.865936786471));
#60342=CARTESIAN_POINT('',(30.1474661481152,93.8,-39.865936786471));
#60343=CARTESIAN_POINT('',(32.4025976934265,93.8,-38.0637949921953));
#60344=CARTESIAN_POINT('',(24.9851420432247,93.8,-32.4767277735883));
#60345=CARTESIAN_POINT('',(25.4182768456334,93.8,-35.3307998778415));
#60346=CARTESIAN_POINT('',(24.9851420432247,93.8,-32.4767277735883));
#60347=CARTESIAN_POINT('',(22.2968756955047,93.8,-31.4247974636109));
#60348=CARTESIAN_POINT('',(22.2968756955047,93.8,-31.4247974636109));
#60349=CARTESIAN_POINT('',(20.0417441501933,93.8,-33.2269392578866));
#60350=CARTESIAN_POINT('',(20.0417441501933,93.8,-33.2269392578866));
#60351=CARTESIAN_POINT('',(20.474878952602,93.8,-36.0810113621397));
#60352=CARTESIAN_POINT('',(20.474878952602,93.8,-36.0810113621397));
#60353=CARTESIAN_POINT('',(23.1631453003221,93.8,-37.1329416721171));
#60354=CARTESIAN_POINT('',(23.1631453003221,93.8,-37.1329416721171));
#60355=CARTESIAN_POINT('',(25.4182768456334,93.8,-35.3307998778414));
#60356=CARTESIAN_POINT('',(18.0008211954315,93.8,-29.7437326592344));
#60357=CARTESIAN_POINT('',(18.4339559978403,93.8,-32.5978047634876));
#60358=CARTESIAN_POINT('',(18.0008211954315,93.8,-29.7437326592344));
#60359=CARTESIAN_POINT('',(15.3125548477115,93.8,-28.691802349257));
#60360=CARTESIAN_POINT('',(15.3125548477115,93.8,-28.691802349257));
#60361=CARTESIAN_POINT('',(13.0574233024002,93.8,-30.4939441435327));
#60362=CARTESIAN_POINT('',(13.0574233024002,93.8,-30.4939441435327));
#60363=CARTESIAN_POINT('',(13.4905581048089,93.8,-33.3480162477858));
#60364=CARTESIAN_POINT('',(13.4905581048089,93.8,-33.3480162477858));
#60365=CARTESIAN_POINT('',(16.1788244525289,93.8,-34.3999465577632));
#60366=CARTESIAN_POINT('',(16.1788244525289,93.8,-34.3999465577632));
#60367=CARTESIAN_POINT('',(18.4339559978403,93.8,-32.5978047634875));
#60368=CARTESIAN_POINT('',(11.0165003476384,93.8,-27.0107375448806));
#60369=CARTESIAN_POINT('',(11.4496351500471,93.8,-29.8648096491337));
#60370=CARTESIAN_POINT('',(11.0165003476384,93.8,-27.0107375448806));
#60371=CARTESIAN_POINT('',(8.3282339999184,93.8,-25.9588072349031));
#60372=CARTESIAN_POINT('',(8.3282339999184,93.8,-25.9588072349031));
#60373=CARTESIAN_POINT('',(6.07310245460704,93.8,-27.7609490291788));
#60374=CARTESIAN_POINT('',(6.07310245460704,93.8,-27.7609490291788));
#60375=CARTESIAN_POINT('',(6.50623725701577,93.8,-30.6150211334319));
#60376=CARTESIAN_POINT('',(6.50623725701577,93.8,-30.6150211334319));
#60377=CARTESIAN_POINT('',(9.1945036047358,93.8,-31.6669514434093));
#60378=CARTESIAN_POINT('',(9.1945036047358,93.8,-31.6669514434093));
#60379=CARTESIAN_POINT('',(11.4496351500471,93.8,-29.8648096491337));
#60380=CARTESIAN_POINT('',(4.03217949984528,93.8,-24.2777424305267));
#60381=CARTESIAN_POINT('',(4.465314302254,93.8,-27.1318145347798));
#60382=CARTESIAN_POINT('',(4.03217949984528,93.8,-24.2777424305267));
#60383=CARTESIAN_POINT('',(1.34391315212527,93.8,-23.2258121205493));
#60384=CARTESIAN_POINT('',(1.34391315212527,93.8,-23.2258121205493));
#60385=CARTESIAN_POINT('',(-0.911218393186086,93.8,-25.0279539148249));
#60386=CARTESIAN_POINT('',(-0.911218393186086,93.8,-25.0279539148249));
#60387=CARTESIAN_POINT('',(-0.478083590777355,93.8,-27.882026019078));
#60388=CARTESIAN_POINT('',(-0.478083590777355,93.8,-27.882026019078));
#60389=CARTESIAN_POINT('',(2.21018275694267,93.8,-28.9339563290554));
#60390=CARTESIAN_POINT('',(2.21018275694267,93.8,-28.9339563290554));
#60391=CARTESIAN_POINT('',(4.465314302254,93.8,-27.1318145347798));
#60392=CARTESIAN_POINT('',(47.0634218130514,93.8,-48.0908099561971));
#60393=CARTESIAN_POINT('',(47.4965566154602,93.8,-50.9448820604502));
#60394=CARTESIAN_POINT('',(47.0634218130514,93.8,-48.0908099561971));
#60395=CARTESIAN_POINT('',(44.3751554653314,93.8,-47.0388796462197));
#60396=CARTESIAN_POINT('',(44.3751554653314,93.8,-47.0388796462197));
#60397=CARTESIAN_POINT('',(42.1200239200201,93.8,-48.8410214404954));
#60398=CARTESIAN_POINT('',(42.1200239200201,93.8,-48.8410214404954));
#60399=CARTESIAN_POINT('',(42.5531587224288,93.8,-51.6950935447484));
#60400=CARTESIAN_POINT('',(42.5531587224288,93.8,-51.6950935447484));
#60401=CARTESIAN_POINT('',(45.2414250701488,93.8,-52.7470238547258));
#60402=CARTESIAN_POINT('',(45.2414250701488,93.8,-52.7470238547258));
#60403=CARTESIAN_POINT('',(47.4965566154602,93.8,-50.9448820604502));
#60404=CARTESIAN_POINT('',(40.0791009652583,93.8,-45.3578148418432));
#60405=CARTESIAN_POINT('',(40.512235767667,93.8,-48.2118869460963));
#60406=CARTESIAN_POINT('',(40.0791009652583,93.8,-45.3578148418432));
#60407=CARTESIAN_POINT('',(37.3908346175383,93.8,-44.3058845318658));
#60408=CARTESIAN_POINT('',(37.3908346175383,93.8,-44.3058845318658));
#60409=CARTESIAN_POINT('',(35.1357030722269,93.8,-46.1080263261415));
#60410=CARTESIAN_POINT('',(35.1357030722269,93.8,-46.1080263261415));
#60411=CARTESIAN_POINT('',(35.5688378746357,93.8,-48.9620984303945));
#60412=CARTESIAN_POINT('',(35.5688378746357,93.8,-48.9620984303945));
#60413=CARTESIAN_POINT('',(38.2571042223557,93.8,-50.014028740372));
#60414=CARTESIAN_POINT('',(38.2571042223557,93.8,-50.014028740372));
#60415=CARTESIAN_POINT('',(40.512235767667,93.8,-48.2118869460963));
#60416=CARTESIAN_POINT('',(36.4707317968073,93.8,-64.8701102461305));
#60417=CARTESIAN_POINT('',(36.903866599216,93.8,-67.7241823503836));
#60418=CARTESIAN_POINT('',(36.4707317968073,93.8,-64.8701102461305));
#60419=CARTESIAN_POINT('',(33.7824654490873,93.8,-63.818179936153));
#60420=CARTESIAN_POINT('',(33.7824654490873,93.8,-63.818179936153));
#60421=CARTESIAN_POINT('',(31.5273339037759,93.8,-65.6203217304287));
#60422=CARTESIAN_POINT('',(31.5273339037759,93.8,-65.6203217304287));
#60423=CARTESIAN_POINT('',(31.9604687061847,93.8,-68.4743938346818));
#60424=CARTESIAN_POINT('',(31.9604687061847,93.8,-68.4743938346818));
#60425=CARTESIAN_POINT('',(34.6487350539047,93.8,-69.5263241446592));
#60426=CARTESIAN_POINT('',(34.6487350539047,93.8,-69.5263241446592));
#60427=CARTESIAN_POINT('',(36.903866599216,93.8,-67.7241823503836));
#60428=CARTESIAN_POINT('',(29.4864109490142,93.8,-62.1371151317766));
#60429=CARTESIAN_POINT('',(29.9195457514229,93.8,-64.9911872360297));
#60430=CARTESIAN_POINT('',(29.4864109490142,93.8,-62.1371151317766));
#60431=CARTESIAN_POINT('',(26.7981446012942,93.8,-61.0851848217992));
#60432=CARTESIAN_POINT('',(26.7981446012942,93.8,-61.0851848217992));
#60433=CARTESIAN_POINT('',(24.5430130559828,93.8,-62.8873266160749));
#60434=CARTESIAN_POINT('',(24.5430130559828,93.8,-62.8873266160749));
#60435=CARTESIAN_POINT('',(24.9761478583915,93.8,-65.7413987203279));
#60436=CARTESIAN_POINT('',(24.9761478583915,93.8,-65.7413987203279));
#60437=CARTESIAN_POINT('',(27.6644142061116,93.8,-66.7933290303053));
#60438=CARTESIAN_POINT('',(27.6644142061116,93.8,-66.7933290303053));
#60439=CARTESIAN_POINT('',(29.9195457514229,93.8,-64.9911872360297));
#60440=CARTESIAN_POINT('',(22.502090101221,93.8,-59.4041200174227));
#60441=CARTESIAN_POINT('',(22.9352249036298,93.8,-62.2581921216758));
#60442=CARTESIAN_POINT('',(22.502090101221,93.8,-59.4041200174227));
#60443=CARTESIAN_POINT('',(19.813823753501,93.8,-58.3521897074453));
#60444=CARTESIAN_POINT('',(19.813823753501,93.8,-58.3521897074453));
#60445=CARTESIAN_POINT('',(17.5586922081897,93.8,-60.154331501721));
#60446=CARTESIAN_POINT('',(17.5586922081897,93.8,-60.154331501721));
#60447=CARTESIAN_POINT('',(17.9918270105984,93.8,-63.008403605974));
#60448=CARTESIAN_POINT('',(17.9918270105984,93.8,-63.008403605974));
#60449=CARTESIAN_POINT('',(20.6800933583184,93.8,-64.0603339159514));
#60450=CARTESIAN_POINT('',(20.6800933583184,93.8,-64.0603339159514));
#60451=CARTESIAN_POINT('',(22.9352249036298,93.8,-62.2581921216758));
#60452=CARTESIAN_POINT('',(15.5177692534279,93.8,-56.6711249030688));
#60453=CARTESIAN_POINT('',(15.9509040558366,93.8,-59.5251970073219));
#60454=CARTESIAN_POINT('',(15.5177692534279,93.8,-56.6711249030688));
#60455=CARTESIAN_POINT('',(12.8295029057079,93.8,-55.6191945930914));
#60456=CARTESIAN_POINT('',(12.8295029057079,93.8,-55.6191945930914));
#60457=CARTESIAN_POINT('',(10.5743713603965,93.8,-57.4213363873671));
#60458=CARTESIAN_POINT('',(10.5743713603965,93.8,-57.4213363873671));
#60459=CARTESIAN_POINT('',(11.0075061628053,93.8,-60.2754084916201));
#60460=CARTESIAN_POINT('',(11.0075061628053,93.8,-60.2754084916201));
#60461=CARTESIAN_POINT('',(13.6957725105253,93.8,-61.3273388015976));
#60462=CARTESIAN_POINT('',(13.6957725105253,93.8,-61.3273388015976));
#60463=CARTESIAN_POINT('',(15.9509040558366,93.8,-59.5251970073219));
#60464=CARTESIAN_POINT('',(8.53344840563478,93.8,-53.9381297887149));
#60465=CARTESIAN_POINT('',(8.9665832080435,93.8,-56.792201892968));
#60466=CARTESIAN_POINT('',(8.53344840563478,93.8,-53.9381297887149));
#60467=CARTESIAN_POINT('',(5.84518205791477,93.8,-52.8861994787375));
#60468=CARTESIAN_POINT('',(5.84518205791477,93.8,-52.8861994787375));
#60469=CARTESIAN_POINT('',(3.59005051260342,93.8,-54.6883412730132));
#60470=CARTESIAN_POINT('',(3.59005051260342,93.8,-54.6883412730132));
#60471=CARTESIAN_POINT('',(4.02318531501215,93.8,-57.5424133772663));
#60472=CARTESIAN_POINT('',(4.02318531501215,93.8,-57.5424133772663));
#60473=CARTESIAN_POINT('',(6.71145166273218,93.8,-58.5943436872437));
#60474=CARTESIAN_POINT('',(6.71145166273218,93.8,-58.5943436872437));
#60475=CARTESIAN_POINT('',(8.9665832080435,93.8,-56.792201892968));
#60476=CARTESIAN_POINT('',(1.54912755784165,93.8,-51.205134674361));
#60477=CARTESIAN_POINT('',(1.98226236025037,93.8,-54.0592067786141));
#60478=CARTESIAN_POINT('',(1.54912755784165,93.8,-51.205134674361));
#60479=CARTESIAN_POINT('',(-1.13913878987836,93.8,-50.1532043643836));
#60480=CARTESIAN_POINT('',(-1.13913878987836,93.8,-50.1532043643836));
#60481=CARTESIAN_POINT('',(-3.39427033518972,93.8,-51.9553461586593));
#60482=CARTESIAN_POINT('',(-3.39427033518972,93.8,-51.9553461586593));
#60483=CARTESIAN_POINT('',(-2.96113553278099,93.8,-54.8094182629124));
#60484=CARTESIAN_POINT('',(-2.96113553278099,93.8,-54.8094182629124));
#60485=CARTESIAN_POINT('',(-0.272869185060958,93.8,-55.8613485728898));
#60486=CARTESIAN_POINT('',(-0.272869185060958,93.8,-55.8613485728898));
#60487=CARTESIAN_POINT('',(1.98226236025037,93.8,-54.0592067786141));
#60488=CARTESIAN_POINT('',(-5.43519328995148,93.8,-48.4721395600071));
#60489=CARTESIAN_POINT('',(-5.00205848754277,93.8,-51.3262116642602));
#60490=CARTESIAN_POINT('',(-5.43519328995148,93.8,-48.4721395600071));
#60491=CARTESIAN_POINT('',(-8.12345963767149,93.8,-47.4202092500297));
#60492=CARTESIAN_POINT('',(-8.12345963767149,93.8,-47.4202092500297));
#60493=CARTESIAN_POINT('',(-10.3785911829829,93.8,-49.2223510443054));
#60494=CARTESIAN_POINT('',(-10.3785911829829,93.8,-49.2223510443054));
#60495=CARTESIAN_POINT('',(-9.94545638057412,93.8,-52.0764231485585));
#60496=CARTESIAN_POINT('',(-9.94545638057412,93.8,-52.0764231485585));
#60497=CARTESIAN_POINT('',(-7.25719003285409,93.8,-53.1283534585359));
#60498=CARTESIAN_POINT('',(-7.25719003285409,93.8,-53.1283534585359));
#60499=CARTESIAN_POINT('',(-5.00205848754277,93.8,-51.3262116642602));
#60500=CARTESIAN_POINT('',(-12.4195141377446,93.8,-45.7391444456532));
#60501=CARTESIAN_POINT('',(-11.9863793353359,93.8,-48.5932165499063));
#60502=CARTESIAN_POINT('',(-12.4195141377446,93.8,-45.7391444456532));
#60503=CARTESIAN_POINT('',(-15.1077804854646,93.8,-44.6872141356758));
#60504=CARTESIAN_POINT('',(-15.1077804854646,93.8,-44.6872141356758));
#60505=CARTESIAN_POINT('',(-17.362912030776,93.8,-46.4893559299515));
#60506=CARTESIAN_POINT('',(-17.362912030776,93.8,-46.4893559299515));
#60507=CARTESIAN_POINT('',(-16.9297772283673,93.8,-49.3434280342046));
#60508=CARTESIAN_POINT('',(-16.9297772283673,93.8,-49.3434280342046));
#60509=CARTESIAN_POINT('',(-14.2415108806472,93.8,-50.395358344182));
#60510=CARTESIAN_POINT('',(-14.2415108806472,93.8,-50.395358344182));
#60511=CARTESIAN_POINT('',(-11.9863793353359,93.8,-48.5932165499063));
#60512=CARTESIAN_POINT('',(23.6274073276684,93.8,-66.8192168569697));
#60513=CARTESIAN_POINT('',(24.0605421300771,93.8,-69.6732889612228));
#60514=CARTESIAN_POINT('',(23.6274073276684,93.8,-66.8192168569697));
#60515=CARTESIAN_POINT('',(20.9391409799484,93.8,-65.7672865469923));
#60516=CARTESIAN_POINT('',(20.9391409799484,93.8,-65.7672865469923));
#60517=CARTESIAN_POINT('',(18.684009434637,93.8,-67.569428341268));
#60518=CARTESIAN_POINT('',(18.684009434637,93.8,-67.569428341268));
#60519=CARTESIAN_POINT('',(19.1171442370458,93.8,-70.4235004455211));
#60520=CARTESIAN_POINT('',(19.1171442370458,93.8,-70.4235004455211));
#60521=CARTESIAN_POINT('',(21.8054105847658,93.8,-71.4754307554985));
#60522=CARTESIAN_POINT('',(21.8054105847658,93.8,-71.4754307554985));
#60523=CARTESIAN_POINT('',(24.0605421300771,93.8,-69.6732889612228));
#60524=CARTESIAN_POINT('',(30.6117281754615,93.8,-69.5522119713236));
#60525=CARTESIAN_POINT('',(31.0448629778703,93.8,-72.4062840755767));
#60526=CARTESIAN_POINT('',(30.6117281754615,93.8,-69.5522119713236));
#60527=CARTESIAN_POINT('',(27.9234618277415,93.8,-68.5002816613462));
#60528=CARTESIAN_POINT('',(27.9234618277415,93.8,-68.5002816613462));
#60529=CARTESIAN_POINT('',(25.6683302824302,93.8,-70.3024234556219));
#60530=CARTESIAN_POINT('',(25.6683302824302,93.8,-70.3024234556219));
#60531=CARTESIAN_POINT('',(26.1014650848389,93.8,-73.156495559875));
#60532=CARTESIAN_POINT('',(26.1014650848389,93.8,-73.156495559875));
#60533=CARTESIAN_POINT('',(28.7897314325589,93.8,-74.2084258698524));
#60534=CARTESIAN_POINT('',(28.7897314325589,93.8,-74.2084258698524));
#60535=CARTESIAN_POINT('',(31.0448629778703,93.8,-72.4062840755767));
#60536=CARTESIAN_POINT('',(37.5960490232547,93.8,-72.2852070856775));
#60537=CARTESIAN_POINT('',(38.0291838256634,93.8,-75.1392791899306));
#60538=CARTESIAN_POINT('',(37.5960490232547,93.8,-72.2852070856775));
#60539=CARTESIAN_POINT('',(34.9077826755347,93.8,-71.2332767757001));
#60540=CARTESIAN_POINT('',(34.9077826755347,93.8,-71.2332767757001));
#60541=CARTESIAN_POINT('',(32.6526511302233,93.8,-73.0354185699758));
#60542=CARTESIAN_POINT('',(32.6526511302233,93.8,-73.0354185699758));
#60543=CARTESIAN_POINT('',(33.085785932632,93.8,-75.8894906742289));
#60544=CARTESIAN_POINT('',(33.085785932632,93.8,-75.8894906742289));
#60545=CARTESIAN_POINT('',(35.7740522803521,93.8,-76.9414209842063));
#60546=CARTESIAN_POINT('',(35.7740522803521,93.8,-76.9414209842063));
#60547=CARTESIAN_POINT('',(38.0291838256634,93.8,-75.1392791899306));
#60548=CARTESIAN_POINT('',(44.5803698710478,93.8,-75.0182022000314));
#60549=CARTESIAN_POINT('',(45.0135046734565,93.8,-77.8722743042845));
#60550=CARTESIAN_POINT('',(44.5803698710478,93.8,-75.0182022000314));
#60551=CARTESIAN_POINT('',(41.8921035233278,93.8,-73.966271890054));
#60552=CARTESIAN_POINT('',(41.8921035233278,93.8,-73.966271890054));
#60553=CARTESIAN_POINT('',(39.6369719780164,93.8,-75.7684136843297));
#60554=CARTESIAN_POINT('',(39.6369719780164,93.8,-75.7684136843297));
#60555=CARTESIAN_POINT('',(40.0701067804252,93.8,-78.6224857885828));
#60556=CARTESIAN_POINT('',(40.0701067804252,93.8,-78.6224857885828));
#60557=CARTESIAN_POINT('',(42.7583731281452,93.8,-79.6744160985602));
#60558=CARTESIAN_POINT('',(42.7583731281452,93.8,-79.6744160985602));
#60559=CARTESIAN_POINT('',(45.0135046734565,93.8,-77.8722743042845));
#60560=CARTESIAN_POINT('',(-19.4038349855377,93.8,-43.0061493312993));
#60561=CARTESIAN_POINT('',(-18.970700183129,93.8,-45.8602214355524));
#60562=CARTESIAN_POINT('',(-19.4038349855377,93.8,-43.0061493312993));
#60563=CARTESIAN_POINT('',(-22.0921013332578,93.8,-41.9542190213219));
#60564=CARTESIAN_POINT('',(-22.0921013332578,93.8,-41.9542190213219));
#60565=CARTESIAN_POINT('',(-24.3472328785691,93.8,-43.7563608155976));
#60566=CARTESIAN_POINT('',(-24.3472328785691,93.8,-43.7563608155976));
#60567=CARTESIAN_POINT('',(-23.9140980761604,93.8,-46.6104329198507));
#60568=CARTESIAN_POINT('',(-23.9140980761604,93.8,-46.6104329198507));
#60569=CARTESIAN_POINT('',(-21.2258317284404,93.8,-47.6623632298281));
#60570=CARTESIAN_POINT('',(-21.2258317284404,93.8,-47.6623632298281));
#60571=CARTESIAN_POINT('',(-18.970700183129,93.8,-45.8602214355524));
#60572=CARTESIAN_POINT('',(-26.3881558333309,93.8,-40.2731542169454));
#60573=CARTESIAN_POINT('',(-25.9550210309222,93.8,-43.1272263211985));
#60574=CARTESIAN_POINT('',(-26.3881558333309,93.8,-40.2731542169454));
#60575=CARTESIAN_POINT('',(-29.0764221810509,93.8,-39.221223906968));
#60576=CARTESIAN_POINT('',(-29.0764221810509,93.8,-39.221223906968));
#60577=CARTESIAN_POINT('',(-31.3315537263622,93.8,-41.0233657012437));
#60578=CARTESIAN_POINT('',(-31.3315537263622,93.8,-41.0233657012437));
#60579=CARTESIAN_POINT('',(-30.8984189239535,93.8,-43.8774378054968));
#60580=CARTESIAN_POINT('',(-30.8984189239535,93.8,-43.8774378054968));
#60581=CARTESIAN_POINT('',(-28.2101525762335,93.8,-44.9293681154742));
#60582=CARTESIAN_POINT('',(-28.2101525762335,93.8,-44.9293681154742));
#60583=CARTESIAN_POINT('',(-25.9550210309222,93.8,-43.1272263211986));
#60584=CARTESIAN_POINT('',(-33.372476681124,93.8,-37.5401591025916));
#60585=CARTESIAN_POINT('',(-32.9393418787153,93.8,-40.3942312068447));
#60586=CARTESIAN_POINT('',(-33.372476681124,93.8,-37.5401591025916));
#60587=CARTESIAN_POINT('',(-36.060743028844,93.8,-36.4882287926142));
#60588=CARTESIAN_POINT('',(-36.060743028844,93.8,-36.4882287926142));
#60589=CARTESIAN_POINT('',(-38.3158745741554,93.8,-38.2903705868898));
#60590=CARTESIAN_POINT('',(-38.3158745741554,93.8,-38.2903705868898));
#60591=CARTESIAN_POINT('',(-37.8827397717466,93.8,-41.1444426911429));
#60592=CARTESIAN_POINT('',(-37.8827397717466,93.8,-41.1444426911429));
#60593=CARTESIAN_POINT('',(-35.1944734240266,93.8,-42.1963730011203));
#60594=CARTESIAN_POINT('',(-35.1944734240266,93.8,-42.1963730011203));
#60595=CARTESIAN_POINT('',(-32.9393418787153,93.8,-40.3942312068447));
#60596=CARTESIAN_POINT('',(51.5646907188409,93.8,-77.7511973143853));
#60597=CARTESIAN_POINT('',(51.9978255212496,93.8,-80.6052694186384));
#60598=CARTESIAN_POINT('',(51.5646907188409,93.8,-77.7511973143853));
#60599=CARTESIAN_POINT('',(48.8764243711209,93.8,-76.6992670044079));
#60600=CARTESIAN_POINT('',(48.8764243711209,93.8,-76.6992670044079));
#60601=CARTESIAN_POINT('',(46.6212928258096,93.8,-78.5014087986836));
#60602=CARTESIAN_POINT('',(46.6212928258096,93.8,-78.5014087986836));
#60603=CARTESIAN_POINT('',(47.0544276282183,93.8,-81.3554809029366));
#60604=CARTESIAN_POINT('',(47.0544276282183,93.8,-81.3554809029366));
#60605=CARTESIAN_POINT('',(49.7426939759383,93.8,-82.4074112129141));
#60606=CARTESIAN_POINT('',(49.7426939759383,93.8,-82.4074112129141));
#60607=CARTESIAN_POINT('',(51.9978255212496,93.8,-80.6052694186384));
#60608=CARTESIAN_POINT('',(14.3924520269805,93.8,-49.2560280635217));
#60609=CARTESIAN_POINT('',(14.8255868293893,93.8,-52.1101001677748));
#60610=CARTESIAN_POINT('',(14.3924520269805,93.8,-49.2560280635217));
#60611=CARTESIAN_POINT('',(11.7041856792605,93.8,-48.2040977535443));
#60612=CARTESIAN_POINT('',(11.7041856792605,93.8,-48.2040977535443));
#60613=CARTESIAN_POINT('',(9.44905413394917,93.8,-50.00623954782));
#60614=CARTESIAN_POINT('',(9.44905413394917,93.8,-50.00623954782));
#60615=CARTESIAN_POINT('',(9.8821889363579,93.8,-52.8603116520731));
#60616=CARTESIAN_POINT('',(9.8821889363579,93.8,-52.8603116520731));
#60617=CARTESIAN_POINT('',(12.5704552840779,93.8,-53.9122419620505));
#60618=CARTESIAN_POINT('',(12.5704552840779,93.8,-53.9122419620505));
#60619=CARTESIAN_POINT('',(14.8255868293893,93.8,-52.1101001677748));
#60620=CARTESIAN_POINT('',(21.3767728747737,93.8,-51.9890231778756));
#60621=CARTESIAN_POINT('',(21.8099076771824,93.8,-54.8430952821287));
#60622=CARTESIAN_POINT('',(21.3767728747737,93.8,-51.9890231778756));
#60623=CARTESIAN_POINT('',(18.6885065270537,93.8,-50.9370928678982));
#60624=CARTESIAN_POINT('',(18.6885065270537,93.8,-50.9370928678982));
#60625=CARTESIAN_POINT('',(16.4333749817423,93.8,-52.7392346621739));
#60626=CARTESIAN_POINT('',(16.4333749817423,93.8,-52.7392346621739));
#60627=CARTESIAN_POINT('',(16.866509784151,93.8,-55.593306766427));
#60628=CARTESIAN_POINT('',(16.866509784151,93.8,-55.593306766427));
#60629=CARTESIAN_POINT('',(19.5547761318711,93.8,-56.6452370764044));
#60630=CARTESIAN_POINT('',(19.5547761318711,93.8,-56.6452370764044));
#60631=CARTESIAN_POINT('',(21.8099076771824,93.8,-54.8430952821287));
#60632=CARTESIAN_POINT('',(28.3610937225668,93.8,-54.7220182922295));
#60633=CARTESIAN_POINT('',(28.7942285249755,93.8,-57.5760903964826));
#60634=CARTESIAN_POINT('',(28.3610937225668,93.8,-54.7220182922295));
#60635=CARTESIAN_POINT('',(25.6728273748468,93.8,-53.6700879822521));
#60636=CARTESIAN_POINT('',(25.6728273748468,93.8,-53.6700879822521));
#60637=CARTESIAN_POINT('',(23.4176958295354,93.8,-55.4722297765278));
#60638=CARTESIAN_POINT('',(23.4176958295354,93.8,-55.4722297765278));
#60639=CARTESIAN_POINT('',(23.8508306319442,93.8,-58.3263018807808));
#60640=CARTESIAN_POINT('',(23.8508306319442,93.8,-58.3263018807808));
#60641=CARTESIAN_POINT('',(26.5390969796642,93.8,-59.3782321907583));
#60642=CARTESIAN_POINT('',(26.5390969796642,93.8,-59.3782321907583));
#60643=CARTESIAN_POINT('',(28.7942285249755,93.8,-57.5760903964826));
#60644=CARTESIAN_POINT('',(35.3454145703599,93.8,-57.4550134065834));
#60645=CARTESIAN_POINT('',(35.7785493727686,93.8,-60.3090855108365));
#60646=CARTESIAN_POINT('',(35.3454145703599,93.8,-57.4550134065834));
#60647=CARTESIAN_POINT('',(32.6571482226399,93.8,-56.403083096606));
#60648=CARTESIAN_POINT('',(32.6571482226399,93.8,-56.403083096606));
#60649=CARTESIAN_POINT('',(30.4020166773286,93.8,-58.2052248908817));
#60650=CARTESIAN_POINT('',(30.4020166773286,93.8,-58.2052248908817));
#60651=CARTESIAN_POINT('',(30.8351514797373,93.8,-61.0592969951347));
#60652=CARTESIAN_POINT('',(30.8351514797373,93.8,-61.0592969951347));
#60653=CARTESIAN_POINT('',(33.5234178274573,93.8,-62.1112273051122));
#60654=CARTESIAN_POINT('',(33.5234178274573,93.8,-62.1112273051122));
#60655=CARTESIAN_POINT('',(35.7785493727686,93.8,-60.3090855108365));
#60656=CARTESIAN_POINT('',(42.3297354181531,93.8,-60.1880085209373));
#60657=CARTESIAN_POINT('',(42.7628702205618,93.8,-63.0420806251904));
#60658=CARTESIAN_POINT('',(42.3297354181531,93.8,-60.1880085209373));
#60659=CARTESIAN_POINT('',(39.641469070433,93.8,-59.1360782109599));
#60660=CARTESIAN_POINT('',(39.641469070433,93.8,-59.1360782109599));
#60661=CARTESIAN_POINT('',(37.3863375251217,93.8,-60.9382200052356));
#60662=CARTESIAN_POINT('',(37.3863375251217,93.8,-60.9382200052356));
#60663=CARTESIAN_POINT('',(37.8194723275304,93.8,-63.7922921094886));
#60664=CARTESIAN_POINT('',(37.8194723275304,93.8,-63.7922921094886));
#60665=CARTESIAN_POINT('',(40.5077386752504,93.8,-64.844222419466));
#60666=CARTESIAN_POINT('',(40.5077386752504,93.8,-64.844222419466));
#60667=CARTESIAN_POINT('',(42.7628702205618,93.8,-63.0420806251904));
#60668=CARTESIAN_POINT('',(49.3140562659462,93.8,-62.9210036352912));
#60669=CARTESIAN_POINT('',(49.7471910683549,93.8,-65.7750757395443));
#60670=CARTESIAN_POINT('',(49.3140562659462,93.8,-62.9210036352912));
#60671=CARTESIAN_POINT('',(46.6257899182262,93.8,-61.8690733253138));
#60672=CARTESIAN_POINT('',(46.6257899182262,93.8,-61.8690733253138));
#60673=CARTESIAN_POINT('',(44.3706583729148,93.8,-63.6712151195895));
#60674=CARTESIAN_POINT('',(44.3706583729148,93.8,-63.6712151195895));
#60675=CARTESIAN_POINT('',(44.8037931753235,93.8,-66.5252872238425));
#60676=CARTESIAN_POINT('',(44.8037931753235,93.8,-66.5252872238425));
#60677=CARTESIAN_POINT('',(47.4920595230436,93.8,-67.5772175338199));
#60678=CARTESIAN_POINT('',(47.4920595230436,93.8,-67.5772175338199));
#60679=CARTESIAN_POINT('',(49.7471910683549,93.8,-65.7750757395443));
#60680=CARTESIAN_POINT('',(-21.6544694384325,93.8,-28.1759556522052));
#60681=CARTESIAN_POINT('',(-21.2213346360238,93.8,-31.0300277564583));
#60682=CARTESIAN_POINT('',(-21.6544694384325,93.8,-28.1759556522052));
#60683=CARTESIAN_POINT('',(-24.3427357861525,93.8,-27.1240253422278));
#60684=CARTESIAN_POINT('',(-24.3427357861525,93.8,-27.1240253422278));
#60685=CARTESIAN_POINT('',(-26.5978673314639,93.8,-28.9261671365035));
#60686=CARTESIAN_POINT('',(-26.5978673314639,93.8,-28.9261671365035));
#60687=CARTESIAN_POINT('',(-26.1647325290551,93.8,-31.7802392407566));
#60688=CARTESIAN_POINT('',(-26.1647325290551,93.8,-31.7802392407566));
#60689=CARTESIAN_POINT('',(-23.4764661813351,93.8,-32.832169550734));
#60690=CARTESIAN_POINT('',(-23.4764661813351,93.8,-32.832169550734));
#60691=CARTESIAN_POINT('',(-21.2213346360238,93.8,-31.0300277564583));
#60692=CARTESIAN_POINT('',(-14.6701485906394,93.8,-30.9089507665591));
#60693=CARTESIAN_POINT('',(-14.2370137882306,93.8,-33.7630228708122));
#60694=CARTESIAN_POINT('',(-14.6701485906394,93.8,-30.9089507665591));
#60695=CARTESIAN_POINT('',(-17.3584149383594,93.8,-29.8570204565817));
#60696=CARTESIAN_POINT('',(-17.3584149383594,93.8,-29.8570204565817));
#60697=CARTESIAN_POINT('',(-19.6135464836707,93.8,-31.6591622508574));
#60698=CARTESIAN_POINT('',(-19.6135464836707,93.8,-31.6591622508574));
#60699=CARTESIAN_POINT('',(-19.180411681262,93.8,-34.5132343551105));
#60700=CARTESIAN_POINT('',(-19.180411681262,93.8,-34.5132343551105));
#60701=CARTESIAN_POINT('',(-16.492145333542,93.8,-35.5651646650879));
#60702=CARTESIAN_POINT('',(-16.492145333542,93.8,-35.5651646650879));
#60703=CARTESIAN_POINT('',(-14.2370137882306,93.8,-33.7630228708122));
#60704=CARTESIAN_POINT('',(43.4550526446004,93.8,-67.6031053604843));
#60705=CARTESIAN_POINT('',(43.8881874470091,93.8,-70.4571774647375));
#60706=CARTESIAN_POINT('',(43.4550526446004,93.8,-67.6031053604843));
#60707=CARTESIAN_POINT('',(40.7667862968804,93.8,-66.5511750505069));
#60708=CARTESIAN_POINT('',(40.7667862968804,93.8,-66.5511750505069));
#60709=CARTESIAN_POINT('',(38.5116547515691,93.8,-68.3533168447826));
#60710=CARTESIAN_POINT('',(38.5116547515691,93.8,-68.3533168447826));
#60711=CARTESIAN_POINT('',(38.9447895539778,93.8,-71.2073889490357));
#60712=CARTESIAN_POINT('',(38.9447895539778,93.8,-71.2073889490357));
#60713=CARTESIAN_POINT('',(41.6330559016978,93.8,-72.2593192590131));
#60714=CARTESIAN_POINT('',(41.6330559016978,93.8,-72.2593192590131));
#60715=CARTESIAN_POINT('',(43.8881874470091,93.8,-70.4571774647375));
#60716=CARTESIAN_POINT('',(50.4393734923936,93.8,-70.3361004748382));
#60717=CARTESIAN_POINT('',(50.8725082948023,93.8,-73.1901725790914));
#60718=CARTESIAN_POINT('',(50.4393734923936,93.8,-70.3361004748382));
#60719=CARTESIAN_POINT('',(47.7511071446736,93.8,-69.2841701648608));
#60720=CARTESIAN_POINT('',(47.7511071446736,93.8,-69.2841701648608));
#60721=CARTESIAN_POINT('',(45.4959755993622,93.8,-71.0863119591365));
#60722=CARTESIAN_POINT('',(45.4959755993622,93.8,-71.0863119591365));
#60723=CARTESIAN_POINT('',(45.9291104017709,93.8,-73.9403840633896));
#60724=CARTESIAN_POINT('',(45.9291104017709,93.8,-73.9403840633896));
#60725=CARTESIAN_POINT('',(48.617376749491,93.8,-74.992314373367));
#60726=CARTESIAN_POINT('',(48.617376749491,93.8,-74.992314373367));
#60727=CARTESIAN_POINT('',(50.8725082948023,93.8,-73.1901725790914));
#60728=CARTESIAN_POINT('',(-27.5134730597783,93.8,-32.8580573773984));
#60729=CARTESIAN_POINT('',(-27.0803382573695,93.8,-35.7121294816515));
#60730=CARTESIAN_POINT('',(-27.5134730597783,93.8,-32.8580573773984));
#60731=CARTESIAN_POINT('',(-30.2017394074983,93.8,-31.806127067421));
#60732=CARTESIAN_POINT('',(-30.2017394074983,93.8,-31.806127067421));
#60733=CARTESIAN_POINT('',(-32.4568709528096,93.8,-33.6082688616967));
#60734=CARTESIAN_POINT('',(-32.4568709528096,93.8,-33.6082688616967));
#60735=CARTESIAN_POINT('',(-32.0237361504009,93.8,-36.4623409659497));
#60736=CARTESIAN_POINT('',(-32.0237361504009,93.8,-36.4623409659497));
#60737=CARTESIAN_POINT('',(-29.3354698026809,93.8,-37.5142712759272));
#60738=CARTESIAN_POINT('',(-29.3354698026809,93.8,-37.5142712759272));
#60739=CARTESIAN_POINT('',(-27.0803382573695,93.8,-35.7121294816515));
#60740=CARTESIAN_POINT('',(-20.5291522119851,93.8,-35.5910524917523));
#60741=CARTESIAN_POINT('',(-20.0960174095764,93.8,-38.4451245960054));
#60742=CARTESIAN_POINT('',(-20.5291522119851,93.8,-35.5910524917523));
#60743=CARTESIAN_POINT('',(-23.2174185597051,93.8,-34.5391221817749));
#60744=CARTESIAN_POINT('',(-23.2174185597051,93.8,-34.5391221817749));
#60745=CARTESIAN_POINT('',(-25.4725501050165,93.8,-36.3412639760506));
#60746=CARTESIAN_POINT('',(-25.4725501050165,93.8,-36.3412639760506));
#60747=CARTESIAN_POINT('',(-25.0394153026078,93.8,-39.1953360803036));
#60748=CARTESIAN_POINT('',(-25.0394153026078,93.8,-39.1953360803036));
#60749=CARTESIAN_POINT('',(-22.3511489548877,93.8,-40.2472663902811));
#60750=CARTESIAN_POINT('',(-22.3511489548877,93.8,-40.2472663902811));
#60751=CARTESIAN_POINT('',(-20.0960174095764,93.8,-38.4451245960054));
#60752=CARTESIAN_POINT('',(-13.544831364192,93.8,-38.3240476061062));
#60753=CARTESIAN_POINT('',(-13.1116965617833,93.8,-41.1781197103593));
#60754=CARTESIAN_POINT('',(-13.544831364192,93.8,-38.3240476061062));
#60755=CARTESIAN_POINT('',(-16.233097711912,93.8,-37.2721172961288));
#60756=CARTESIAN_POINT('',(-16.233097711912,93.8,-37.2721172961288));
#60757=CARTESIAN_POINT('',(-18.4882292572234,93.8,-39.0742590904044));
#60758=CARTESIAN_POINT('',(-18.4882292572234,93.8,-39.0742590904044));
#60759=CARTESIAN_POINT('',(-18.0550944548146,93.8,-41.9283311946575));
#60760=CARTESIAN_POINT('',(-18.0550944548146,93.8,-41.9283311946575));
#60761=CARTESIAN_POINT('',(-15.3668281070946,93.8,-42.9802615046349));
#60762=CARTESIAN_POINT('',(-15.3668281070946,93.8,-42.9802615046349));
#60763=CARTESIAN_POINT('',(-13.1116965617833,93.8,-41.1781197103593));
#60764=CARTESIAN_POINT('',(-6.56051051639886,93.8,-41.0570427204601));
#60765=CARTESIAN_POINT('',(-6.12737571399014,93.8,-43.9111148247132));
#60766=CARTESIAN_POINT('',(-6.56051051639886,93.8,-41.0570427204601));
#60767=CARTESIAN_POINT('',(-9.24877686411887,93.8,-40.0051124104826));
#60768=CARTESIAN_POINT('',(-9.24877686411887,93.8,-40.0051124104826));
#60769=CARTESIAN_POINT('',(-11.5039084094302,93.8,-41.8072542047583));
#60770=CARTESIAN_POINT('',(-11.5039084094302,93.8,-41.8072542047583));
#60771=CARTESIAN_POINT('',(-11.0707736070215,93.8,-44.6613263090114));
#60772=CARTESIAN_POINT('',(-11.0707736070215,93.8,-44.6613263090114));
#60773=CARTESIAN_POINT('',(-8.38250725930147,93.8,-45.7132566189888));
#60774=CARTESIAN_POINT('',(-8.38250725930147,93.8,-45.7132566189888));
#60775=CARTESIAN_POINT('',(-6.12737571399014,93.8,-43.9111148247132));
#60776=CARTESIAN_POINT('',(0.423810331394273,93.8,-43.7900378348139));
#60777=CARTESIAN_POINT('',(0.856945133802991,93.8,-46.6441099390671));
#60778=CARTESIAN_POINT('',(0.423810331394273,93.8,-43.7900378348139));
#60779=CARTESIAN_POINT('',(-2.26445601632574,93.8,-42.7381075248365));
#60780=CARTESIAN_POINT('',(-2.26445601632574,93.8,-42.7381075248365));
#60781=CARTESIAN_POINT('',(-4.51958756163709,93.8,-44.5402493191122));
#60782=CARTESIAN_POINT('',(-4.51958756163709,93.8,-44.5402493191122));
#60783=CARTESIAN_POINT('',(-4.08645275922836,93.8,-47.3943214233653));
#60784=CARTESIAN_POINT('',(-4.08645275922836,93.8,-47.3943214233653));
#60785=CARTESIAN_POINT('',(-1.39818641150833,93.8,-48.4462517333427));
#60786=CARTESIAN_POINT('',(-1.39818641150833,93.8,-48.4462517333427));
#60787=CARTESIAN_POINT('',(0.856945133802991,93.8,-46.6441099390671));
#60788=CARTESIAN_POINT('',(7.40813117918741,93.8,-46.5230329491678));
#60789=CARTESIAN_POINT('',(7.84126598159612,93.8,-49.3771050534209));
#60790=CARTESIAN_POINT('',(7.40813117918741,93.8,-46.5230329491678));
#60791=CARTESIAN_POINT('',(4.7198648314674,93.8,-45.4711026391904));
#60792=CARTESIAN_POINT('',(4.7198648314674,93.8,-45.4711026391904));
#60793=CARTESIAN_POINT('',(2.46473328615604,93.8,-47.2732444334661));
#60794=CARTESIAN_POINT('',(2.46473328615604,93.8,-47.2732444334661));
#60795=CARTESIAN_POINT('',(2.89786808856477,93.8,-50.1273165377192));
#60796=CARTESIAN_POINT('',(2.89786808856477,93.8,-50.1273165377192));
#60797=CARTESIAN_POINT('',(5.5861344362848,93.8,-51.1792468476966));
#60798=CARTESIAN_POINT('',(5.5861344362848,93.8,-51.1792468476966));
#60799=CARTESIAN_POINT('',(7.84126598159612,93.8,-49.3771050534209));
#60800=CARTESIAN_POINT('',(-34.9626288857891,93.8,-113.640234108901));
#60801=CARTESIAN_POINT('',(-34.5294940833804,93.8,-116.494306213155));
#60802=CARTESIAN_POINT('',(-34.9626288857891,93.8,-113.640234108901));
#60803=CARTESIAN_POINT('',(-37.6508952335091,93.8,-112.588303798924));
#60804=CARTESIAN_POINT('',(-37.6508952335091,93.8,-112.588303798924));
#60805=CARTESIAN_POINT('',(-39.9060267788205,93.8,-114.3904455932));
#60806=CARTESIAN_POINT('',(-39.9060267788205,93.8,-114.3904455932));
#60807=CARTESIAN_POINT('',(-39.4728919764118,93.8,-117.244517697453));
#60808=CARTESIAN_POINT('',(-39.4728919764118,93.8,-117.244517697453));
#60809=CARTESIAN_POINT('',(-36.7846256286917,93.8,-118.29644800743));
#60810=CARTESIAN_POINT('',(-36.7846256286917,93.8,-118.29644800743));
#60811=CARTESIAN_POINT('',(-34.5294940833804,93.8,-116.494306213155));
#60812=CARTESIAN_POINT('',(-27.978308037996,93.8,-116.373229223255));
#60813=CARTESIAN_POINT('',(-27.5451732355873,93.8,-119.227301327508));
#60814=CARTESIAN_POINT('',(-27.978308037996,93.8,-116.373229223255));
#60815=CARTESIAN_POINT('',(-30.666574385716,93.8,-115.321298913278));
#60816=CARTESIAN_POINT('',(-30.666574385716,93.8,-115.321298913278));
#60817=CARTESIAN_POINT('',(-32.9217059310274,93.8,-117.123440707554));
#60818=CARTESIAN_POINT('',(-32.9217059310274,93.8,-117.123440707554));
#60819=CARTESIAN_POINT('',(-32.4885711286186,93.8,-119.977512811807));
#60820=CARTESIAN_POINT('',(-32.4885711286186,93.8,-119.977512811807));
#60821=CARTESIAN_POINT('',(-29.8003047808986,93.8,-121.029443121784));
#60822=CARTESIAN_POINT('',(-29.8003047808986,93.8,-121.029443121784));
#60823=CARTESIAN_POINT('',(-27.5451732355873,93.8,-119.227301327508));
#60824=CARTESIAN_POINT('Origin',(0.,93.,-77.5000000000001));
#60825=CARTESIAN_POINT('',(-24.5751532752614,93.,-68.8816112651563));
#60826=CARTESIAN_POINT('',(-21.8868869275414,93.,-69.9335415751337));
#60827=CARTESIAN_POINT('',(-0.338657290464793,93.,-78.3654575200768));
#60828=CARTESIAN_POINT('',(-21.4537521251327,93.,-72.7876136793868));
#60829=CARTESIAN_POINT('',(-20.271717355013,93.,-80.5764416490967));
#60830=CARTESIAN_POINT('',(-23.708883670444,93.,-74.5897554736624));
#60831=CARTESIAN_POINT('',(-10.65925517077,93.,-64.1614144006423));
#60832=CARTESIAN_POINT('',(-26.397150018164,93.,-73.537825163685));
#60833=CARTESIAN_POINT('',(-2.16065403336742,93.,-83.0216714186056));
#60834=CARTESIAN_POINT('',(-26.8302848205727,93.,-70.683753059432));
#60835=CARTESIAN_POINT('',(-25.2151152480443,93.,-81.3266531333951));
#60836=CARTESIAN_POINT('',(-13.7806563208988,93.,-60.2554119864118));
#60837=CARTESIAN_POINT('',(-17.5908324274683,93.,-71.6146063795101));
#60838=CARTESIAN_POINT('',(-14.9025660797482,93.,-72.6665366894876));
#60839=CARTESIAN_POINT('',(-0.338657290464798,93.,-78.3654575200768));
#60840=CARTESIAN_POINT('',(-14.4694312773395,93.,-75.5206087937407));
#60841=CARTESIAN_POINT('',(-13.8500551204435,93.,-79.6018883436771));
#60842=CARTESIAN_POINT('',(-16.7245628226509,93.,-77.3227505880163));
#60843=CARTESIAN_POINT('',(-6.60443613364973,93.,-69.2354603775928));
#60844=CARTESIAN_POINT('',(-19.4128291703709,93.,-76.2708202780389));
#60845=CARTESIAN_POINT('',(-2.16065403336742,93.,-83.0216714186056));
#60846=CARTESIAN_POINT('',(-19.8459639727796,93.,-73.4167481737858));
#60847=CARTESIAN_POINT('',(-18.7934530134748,93.,-80.3520998279754));
#60848=CARTESIAN_POINT('',(-9.72583728377851,93.,-65.3294579633623));
#60849=CARTESIAN_POINT('',(-10.6065115796751,93.,-74.347601493864));
#60850=CARTESIAN_POINT('',(-7.91824523195512,93.,-75.3995318038414));
#60851=CARTESIAN_POINT('',(-0.338657290464803,93.,-78.3654575200768));
#60852=CARTESIAN_POINT('',(-7.4851104295464,93.,-78.2536039080945));
#60853=CARTESIAN_POINT('',(-7.42839288587402,93.,-78.6273350382575));
#60854=CARTESIAN_POINT('',(-9.74024197485773,93.,-80.0557457023702));
#60855=CARTESIAN_POINT('',(-2.54961709652949,93.,-74.3095063545433));
#60856=CARTESIAN_POINT('',(-12.4285083225778,93.,-79.0038153923928));
#60857=CARTESIAN_POINT('',(-2.16065403336741,93.,-83.0216714186056));
#60858=CARTESIAN_POINT('',(-12.8616431249865,93.,-76.1497432881397));
#60859=CARTESIAN_POINT('',(-12.3717907789054,93.,-79.3775465225557));
#60860=CARTESIAN_POINT('',(-5.67101824665826,93.,-70.4035039403128));
#60861=CARTESIAN_POINT('',(-3.622190731882,93.,-77.0805966082179));
#60862=CARTESIAN_POINT('',(-0.933924384161986,93.,-78.1325269181953));
#60863=CARTESIAN_POINT('',(-0.338657290464807,93.,-78.3654575200768));
#60864=CARTESIAN_POINT('',(-0.500789581753269,93.,-80.9865990224485));
#60865=CARTESIAN_POINT('',(-1.00673065130454,93.,-77.6527817328379));
#60866=CARTESIAN_POINT('',(-2.75592112706459,93.,-82.7887408167241));
#60867=CARTESIAN_POINT('',(1.50520194059076,93.,-79.3835523314938));
#60868=CARTESIAN_POINT('',(-5.44418747478462,93.,-81.7368105067467));
#60869=CARTESIAN_POINT('',(-2.16065403336741,93.,-83.0216714186056));
#60870=CARTESIAN_POINT('',(-5.87732227719335,93.,-78.8827384024936));
#60871=CARTESIAN_POINT('',(-5.95012854433591,93.,-78.4029932171361));
#60872=CARTESIAN_POINT('',(-1.61619920953801,93.,-75.4775499172633));
#60873=CARTESIAN_POINT('',(3.36213011591114,93.,-79.8135917225718));
#60874=CARTESIAN_POINT('',(6.05039646363115,93.,-80.8655220325492));
#60875=CARTESIAN_POINT('',(-0.338657290464812,93.,-78.3654575200769));
#60876=CARTESIAN_POINT('',(6.48353126603986,93.,-83.7195941368023));
#60877=CARTESIAN_POINT('',(5.41493158326495,93.,-76.6782284274182));
#60878=CARTESIAN_POINT('',(4.22839972072854,93.,-85.521735931078));
#60879=CARTESIAN_POINT('',(5.56002097771101,93.,-84.4575983084442));
#60880=CARTESIAN_POINT('',(1.54013337300851,93.,-84.4698056211006));
#60881=CARTESIAN_POINT('',(-2.16065403336741,93.,-83.0216714186056));
#60882=CARTESIAN_POINT('',(1.10699857059978,93.,-81.6157335168475));
#60883=CARTESIAN_POINT('',(0.471533690233543,93.,-77.4284399117164));
#60884=CARTESIAN_POINT('',(2.43861982758225,93.,-80.5515958942137));
#60885=CARTESIAN_POINT('',(10.3464509637043,93.,-82.5465868369257));
#60886=CARTESIAN_POINT('',(13.0347173114243,93.,-83.5985171469031));
#60887=CARTESIAN_POINT('',(-0.338657290464817,93.,-78.3654575200769));
#60888=CARTESIAN_POINT('',(13.467852113833,93.,-86.4525892511562));
#60889=CARTESIAN_POINT('',(11.8365938178344,93.,-75.7036751219986));
#60890=CARTESIAN_POINT('',(11.2127205685217,93.,-88.2547310454319));
#60891=CARTESIAN_POINT('',(9.61484001483125,93.,-89.5316442853947));
#60892=CARTESIAN_POINT('',(8.52445422080164,93.,-87.2028007354545));
#60893=CARTESIAN_POINT('',(-2.16065403336741,93.,-83.0216714186056));
#60894=CARTESIAN_POINT('',(8.09131941839291,93.,-84.3487286312014));
#60895=CARTESIAN_POINT('',(6.89319592480299,93.,-76.4538866062968));
#60896=CARTESIAN_POINT('',(6.4934388647025,93.,-85.6256418711642));
#60897=CARTESIAN_POINT('',(17.3307718114974,93.,-85.2795819512796));
#60898=CARTESIAN_POINT('',(20.0190381592174,93.,-86.331512261257));
#60899=CARTESIAN_POINT('',(-0.338657290464822,93.,-78.3654575200769));
#60900=CARTESIAN_POINT('',(20.4521729616261,93.,-89.1855843655101));
#60901=CARTESIAN_POINT('',(18.2582560524039,93.,-74.729121816579));
#60902=CARTESIAN_POINT('',(18.1970414163148,93.,-90.9877261597858));
#60903=CARTESIAN_POINT('',(13.6696590519515,93.,-94.6056902623452));
#60904=CARTESIAN_POINT('',(15.5087750685948,93.,-89.9357958498083));
#60905=CARTESIAN_POINT('',(-2.16065403336741,93.,-83.0216714186056));
#60906=CARTESIAN_POINT('',(15.075640266186,93.,-87.0817237455553));
#60907=CARTESIAN_POINT('',(13.3148581593724,93.,-75.4793333008771));
#60908=CARTESIAN_POINT('',(10.5482579018227,93.,-90.6996878481147));
#60909=CARTESIAN_POINT('',(24.3150926592905,93.,-88.0125770656335));
#60910=CARTESIAN_POINT('',(27.0033590070105,93.,-89.0645073756109));
#60911=CARTESIAN_POINT('',(-0.338657290464827,93.,-78.3654575200769));
#60912=CARTESIAN_POINT('',(27.4364938094193,93.,-91.918579479864));
#60913=CARTESIAN_POINT('',(24.6799182869734,93.,-73.7545685111594));
#60914=CARTESIAN_POINT('',(25.1813622641079,93.,-93.7207212741397));
#60915=CARTESIAN_POINT('',(17.7244780890717,93.,-99.6797362392957));
#60916=CARTESIAN_POINT('',(22.4930959163879,93.,-92.6687909641622));
#60917=CARTESIAN_POINT('',(-2.16065403336741,93.,-83.0216714186056));
#60918=CARTESIAN_POINT('',(22.0599611139792,93.,-89.8147188599092));
#60919=CARTESIAN_POINT('',(19.7365203939419,93.,-74.5047799954575));
#60920=CARTESIAN_POINT('',(14.603076938943,93.,-95.7737338250652));
#60921=CARTESIAN_POINT('',(-18.7161496539156,93.,-64.1995095399631));
#60922=CARTESIAN_POINT('',(-16.0278833061956,93.,-65.2514398499405));
#60923=CARTESIAN_POINT('',(2.02818590698441,93.,-72.3168582377067));
#60924=CARTESIAN_POINT('',(-15.5947485037869,93.,-68.1055119541936));
#60925=CARTESIAN_POINT('',(-13.8500551204436,93.,-79.6018883436771));
#60926=CARTESIAN_POINT('',(-17.8498800490982,93.,-69.9076537484693));
#60927=CARTESIAN_POINT('',(-10.65925517077,93.,-64.1614144006423));
#60928=CARTESIAN_POINT('',(-20.5381463968183,93.,-68.8557234384919));
#60929=CARTESIAN_POINT('',(0.206189164081804,93.,-76.9730721362355));
#60930=CARTESIAN_POINT('',(-20.971281199227,93.,-66.0016513342388));
#60931=CARTESIAN_POINT('',(-18.7934530134748,93.,-80.3520998279754));
#60932=CARTESIAN_POINT('',(-13.7806563208988,93.,-60.2554119864118));
#60933=CARTESIAN_POINT('',(-25.7004705017088,93.,-61.4665144256092));
#60934=CARTESIAN_POINT('',(-23.0122041539888,93.,-62.5184447355866));
#60935=CARTESIAN_POINT('',(2.02818590698442,93.,-72.3168582377067));
#60936=CARTESIAN_POINT('',(-22.57906935158,93.,-65.3725168398397));
#60937=CARTESIAN_POINT('',(-20.2717173550131,93.,-80.5764416490967));
#60938=CARTESIAN_POINT('',(-24.8342008968914,93.,-67.1746586341154));
#60939=CARTESIAN_POINT('',(-14.7140742078902,93.,-59.0873684236919));
#60940=CARTESIAN_POINT('',(-27.5224672446114,93.,-66.122728324138));
#60941=CARTESIAN_POINT('',(0.206189164081802,93.,-76.9730721362355));
#60942=CARTESIAN_POINT('',(-27.9556020470201,93.,-63.2686562198849));
#60943=CARTESIAN_POINT('',(-25.2151152480443,93.,-81.3266531333951));
#60944=CARTESIAN_POINT('',(-17.835475358019,93.,-55.1813660094614));
#60945=CARTESIAN_POINT('',(-32.6847913495019,93.,-58.7335193112553));
#60946=CARTESIAN_POINT('',(-29.9965250017819,93.,-59.7854496212327));
#60947=CARTESIAN_POINT('',(2.02818590698442,93.,-72.3168582377067));
#60948=CARTESIAN_POINT('',(-29.5633901993732,93.,-62.6395217254858));
#60949=CARTESIAN_POINT('',(-26.6933795895825,93.,-81.5509949545163));
#60950=CARTESIAN_POINT('',(-31.8185217446845,93.,-64.4416635197615));
#60951=CARTESIAN_POINT('',(-18.7688932450105,93.,-54.0133224467414));
#60952=CARTESIAN_POINT('',(-34.5067880924045,93.,-63.3897332097841));
#60953=CARTESIAN_POINT('',(0.206189164081802,93.,-76.9730721362355));
#60954=CARTESIAN_POINT('',(-34.9399228948133,93.,-60.535661105531));
#60955=CARTESIAN_POINT('',(-31.6367774826137,93.,-82.3012064388147));
#60956=CARTESIAN_POINT('',(-21.8902943951393,93.,-50.1073200325109));
#60957=CARTESIAN_POINT('',(-39.669112197295,93.,-56.0005241969014));
#60958=CARTESIAN_POINT('',(-36.980845849575,93.,-57.0524545068788));
#60959=CARTESIAN_POINT('',(2.02818590698443,93.,-72.3168582377067));
#60960=CARTESIAN_POINT('',(-36.5477110471663,93.,-59.9065266111319));
#60961=CARTESIAN_POINT('',(-33.115041824152,93.,-82.5255482599359));
#60962=CARTESIAN_POINT('',(-38.8028425924776,93.,-61.7086684054076));
#60963=CARTESIAN_POINT('',(-22.8237122821307,93.,-48.9392764697909));
#60964=CARTESIAN_POINT('',(-41.4911089401976,93.,-60.6567380954302));
#60965=CARTESIAN_POINT('',(0.2061891640818,93.,-76.9730721362355));
#60966=CARTESIAN_POINT('',(-41.9242437426064,93.,-57.8026659911771));
#60967=CARTESIAN_POINT('',(-38.0584397171832,93.,-83.2757597442344));
#60968=CARTESIAN_POINT('',(-25.9451134322595,93.,-45.0332740555604));
#60969=CARTESIAN_POINT('',(31.2994135070836,93.,-90.7455721799874));
#60970=CARTESIAN_POINT('',(33.9876798548037,93.,-91.7975024899648));
#60971=CARTESIAN_POINT('',(-0.338657290464832,93.,-78.3654575200769));
#60972=CARTESIAN_POINT('',(34.4208146572124,93.,-94.6515745942179));
#60973=CARTESIAN_POINT('',(31.1015805215429,93.,-72.7800152057398));
#60974=CARTESIAN_POINT('',(32.1656831119011,93.,-96.4537163884935));
#60975=CARTESIAN_POINT('',(21.779297126192,93.,-104.753782216246));
#60976=CARTESIAN_POINT('',(29.477416764181,93.,-95.4017860785161));
#60977=CARTESIAN_POINT('',(-2.16065403336741,93.,-83.0216714186056));
#60978=CARTESIAN_POINT('',(29.0442819617723,93.,-92.5477139742631));
#60979=CARTESIAN_POINT('',(26.1581826285113,93.,-73.5302266900378));
#60980=CARTESIAN_POINT('',(18.6578959760632,93.,-100.847779802016));
#60981=CARTESIAN_POINT('',(38.2837343548768,93.,-93.4785672943413));
#60982=CARTESIAN_POINT('',(40.9720007025968,93.,-94.5304976043187));
#60983=CARTESIAN_POINT('',(-0.338657290464837,93.,-78.3654575200769));
#60984=CARTESIAN_POINT('',(41.4051355050055,93.,-97.3845697085718));
#60985=CARTESIAN_POINT('',(37.5232427561124,93.,-71.8054619003202));
#60986=CARTESIAN_POINT('',(39.1500039596942,93.,-99.1867115028475));
#60987=CARTESIAN_POINT('',(25.8341161633122,93.,-109.827828193197));
#60988=CARTESIAN_POINT('',(36.4617376119742,93.,-98.13478119287));
#60989=CARTESIAN_POINT('',(-2.16065403336741,93.,-83.0216714186056));
#60990=CARTESIAN_POINT('',(36.0286028095654,93.,-95.280709088617));
#60991=CARTESIAN_POINT('',(32.5798448630808,93.,-72.5556733846182));
#60992=CARTESIAN_POINT('',(22.7127150131835,93.,-105.921825778966));
#60993=CARTESIAN_POINT('',(45.2680552026699,93.,-96.2115624086952));
#60994=CARTESIAN_POINT('',(47.9563215503899,93.,-97.2634927186726));
#60995=CARTESIAN_POINT('',(-0.338657290464843,93.,-78.3654575200769));
#60996=CARTESIAN_POINT('',(48.3894563527986,93.,-100.117564822926));
#60997=CARTESIAN_POINT('',(43.9449049906818,93.,-70.8309085949005));
#60998=CARTESIAN_POINT('',(46.1343248074873,93.,-101.919706617201));
#60999=CARTESIAN_POINT('',(29.8889352004325,93.,-114.901874170147));
#61000=CARTESIAN_POINT('',(43.4460584597673,93.,-100.867776307224));
#61001=CARTESIAN_POINT('',(-2.16065403336741,93.,-83.0216714186056));
#61002=CARTESIAN_POINT('',(43.0129236573585,93.,-98.0137042029708));
#61003=CARTESIAN_POINT('',(39.0015070976502,93.,-71.5811200791985));
#61004=CARTESIAN_POINT('',(26.7675340503037,93.,-110.995871755917));
#61005=CARTESIAN_POINT('',(-46.6534330450882,93.,-53.2675290825475));
#61006=CARTESIAN_POINT('',(-43.9651666973681,93.,-54.3194593925249));
#61007=CARTESIAN_POINT('',(2.02818590698443,93.,-72.3168582377067));
#61008=CARTESIAN_POINT('',(-43.5320318949594,93.,-57.1735314967781));
#61009=CARTESIAN_POINT('',(-39.5367040587215,93.,-83.5001015653555));
#61010=CARTESIAN_POINT('',(-45.7871634402707,93.,-58.9756732910537));
#61011=CARTESIAN_POINT('',(-26.878531319251,93.,-43.8652304928404));
#61012=CARTESIAN_POINT('',(-48.4754297879908,93.,-57.9237429810763));
#61013=CARTESIAN_POINT('',(0.206189164081799,93.,-76.9730721362355));
#61014=CARTESIAN_POINT('',(-48.9085645903995,93.,-55.0696708768232));
#61015=CARTESIAN_POINT('',(-44.4801019517526,93.,-84.250313049654));
#61016=CARTESIAN_POINT('',(-29.9999324693798,93.,-39.9592280786099));
#61017=CARTESIAN_POINT('',(-44.4027985921934,93.,-68.0977227616416));
#61018=CARTESIAN_POINT('',(-41.7145322444734,93.,-69.1496530716191));
#61019=CARTESIAN_POINT('',(-2.70550048791399,93.,-84.4140568024469));
#61020=CARTESIAN_POINT('',(-41.2813974420647,93.,-72.0037251758721));
#61021=CARTESIAN_POINT('',(-39.5367040587214,93.,-83.5001015653555));
#61022=CARTESIAN_POINT('',(-43.536528987376,93.,-73.8058669701478));
#61023=CARTESIAN_POINT('',(-18.7688932450105,93.,-54.0133224467414));
#61024=CARTESIAN_POINT('',(-46.224795335096,93.,-72.7539366601704));
#61025=CARTESIAN_POINT('',(-4.52749723081664,93.,-89.0702707009757));
#61026=CARTESIAN_POINT('',(-46.6579301375048,93.,-69.8998645559173));
#61027=CARTESIAN_POINT('',(-44.4801019517526,93.,-84.250313049654));
#61028=CARTESIAN_POINT('',(-21.8902943951393,93.,-50.1073200325109));
#61029=CARTESIAN_POINT('',(-37.4184777444003,93.,-70.8307178759955));
#61030=CARTESIAN_POINT('',(-34.7302113966803,93.,-71.8826481859729));
#61031=CARTESIAN_POINT('',(-2.70550048791399,93.,-84.4140568024469));
#61032=CARTESIAN_POINT('',(-34.2970765942716,93.,-74.7367202902261));
#61033=CARTESIAN_POINT('',(-33.1150418241519,93.,-82.5255482599359));
#61034=CARTESIAN_POINT('',(-36.5522081395829,93.,-76.5388620845017));
#61035=CARTESIAN_POINT('',(-14.7140742078902,93.,-59.0873684236919));
#61036=CARTESIAN_POINT('',(-39.2404744873029,93.,-75.4869317745243));
#61037=CARTESIAN_POINT('',(-4.52749723081664,93.,-89.0702707009757));
#61038=CARTESIAN_POINT('',(-39.6736092897116,93.,-72.6328596702712));
#61039=CARTESIAN_POINT('',(-38.0584397171832,93.,-83.2757597442344));
#61040=CARTESIAN_POINT('',(-17.835475358019,93.,-55.1813660094614));
#61041=CARTESIAN_POINT('',(-30.4341568966072,93.,-73.5637129903494));
#61042=CARTESIAN_POINT('',(-27.7458905488871,93.,-74.6156433003268));
#61043=CARTESIAN_POINT('',(-2.705500487914,93.,-84.4140568024469));
#61044=CARTESIAN_POINT('',(-27.3127557464784,93.,-77.4697154045799));
#61045=CARTESIAN_POINT('',(-26.6933795895824,93.,-81.5509949545163));
#61046=CARTESIAN_POINT('',(-29.5678872917897,93.,-79.2718571988556));
#61047=CARTESIAN_POINT('',(-10.65925517077,93.,-64.1614144006423));
#61048=CARTESIAN_POINT('',(-32.2561536395098,93.,-78.2199268888782));
#61049=CARTESIAN_POINT('',(-4.52749723081664,93.,-89.0702707009757));
#61050=CARTESIAN_POINT('',(-32.6892884419185,93.,-75.3658547846251));
#61051=CARTESIAN_POINT('',(-31.6367774826137,93.,-82.3012064388147));
#61052=CARTESIAN_POINT('',(-13.7806563208988,93.,-60.2554119864118));
#61053=CARTESIAN_POINT('',(-23.449836048814,93.,-76.2967081047033));
#61054=CARTESIAN_POINT('',(-20.761569701094,93.,-77.3486384146807));
#61055=CARTESIAN_POINT('',(-2.705500487914,93.,-84.4140568024469));
#61056=CARTESIAN_POINT('',(-20.3284348986853,93.,-80.2027105189338));
#61057=CARTESIAN_POINT('',(-20.2717173550129,93.,-80.5764416490967));
#61058=CARTESIAN_POINT('',(-22.5835664439966,93.,-82.0048523132095));
#61059=CARTESIAN_POINT('',(-6.60443613364973,93.,-69.2354603775928));
#61060=CARTESIAN_POINT('',(-25.2718327917166,93.,-80.9529220032321));
#61061=CARTESIAN_POINT('',(-4.52749723081664,93.,-89.0702707009757));
#61062=CARTESIAN_POINT('',(-25.7049675941254,93.,-78.098849898979));
#61063=CARTESIAN_POINT('',(-25.2151152480443,93.,-81.3266531333951));
#61064=CARTESIAN_POINT('',(-9.72583728377851,93.,-65.3294579633623));
#61065=CARTESIAN_POINT('',(-16.4655152010209,93.,-79.0297032190572));
#61066=CARTESIAN_POINT('',(-13.7772488533009,93.,-80.0816335290346));
#61067=CARTESIAN_POINT('',(-2.70550048791401,93.,-84.4140568024469));
#61068=CARTESIAN_POINT('',(-13.3441140508922,93.,-82.9357056332877));
#61069=CARTESIAN_POINT('',(-13.8500551204434,93.,-79.6018883436771));
#61070=CARTESIAN_POINT('',(-15.5992455962035,93.,-84.7378474275634));
#61071=CARTESIAN_POINT('',(-2.54961709652949,93.,-74.3095063545433));
#61072=CARTESIAN_POINT('',(-18.2875119439235,93.,-83.685917117586));
#61073=CARTESIAN_POINT('',(-4.52749723081664,93.,-89.0702707009757));
#61074=CARTESIAN_POINT('',(-18.7206467463322,93.,-80.8318450133329));
#61075=CARTESIAN_POINT('',(-18.7934530134748,93.,-80.3520998279754));
#61076=CARTESIAN_POINT('',(-5.67101824665826,93.,-70.4035039403128));
#61077=CARTESIAN_POINT('',(-9.48119435322776,93.,-81.7626983334111));
#61078=CARTESIAN_POINT('',(-6.79292800550775,93.,-82.8146286433885));
#61079=CARTESIAN_POINT('',(-2.70550048791401,93.,-84.414056802447));
#61080=CARTESIAN_POINT('',(-6.35979320309903,93.,-85.6687007476416));
#61081=CARTESIAN_POINT('',(-7.42839288587396,93.,-78.6273350382574));
#61082=CARTESIAN_POINT('',(-8.61492474841036,93.,-87.4708425419172));
#61083=CARTESIAN_POINT('',(1.50520194059076,93.,-79.3835523314937));
#61084=CARTESIAN_POINT('',(-11.3031910961304,93.,-86.4189122319399));
#61085=CARTESIAN_POINT('',(-4.52749723081664,93.,-89.0702707009757));
#61086=CARTESIAN_POINT('',(-11.7363258985391,93.,-83.5648401276868));
#61087=CARTESIAN_POINT('',(-12.3717907789053,93.,-79.3775465225557));
#61088=CARTESIAN_POINT('',(-1.61619920953801,93.,-75.4775499172633));
#61089=CARTESIAN_POINT('',(-2.49687350543463,93.,-84.495693447765));
#61090=CARTESIAN_POINT('',(0.191392842285382,93.,-85.5476237577424));
#61091=CARTESIAN_POINT('',(-2.70550048791402,93.,-84.414056802447));
#61092=CARTESIAN_POINT('',(0.6245276446941,93.,-88.4016958619955));
#61093=CARTESIAN_POINT('',(-1.00673065130447,93.,-77.6527817328378));
#61094=CARTESIAN_POINT('',(-1.63060390061722,93.,-90.2038376562712));
#61095=CARTESIAN_POINT('',(5.560020977711,93.,-84.4575983084442));
#61096=CARTESIAN_POINT('',(-4.31887024833725,93.,-89.1519073462937));
#61097=CARTESIAN_POINT('',(-4.52749723081663,93.,-89.0702707009757));
#61098=CARTESIAN_POINT('',(-4.75200505074598,93.,-86.2978352420407));
#61099=CARTESIAN_POINT('',(-5.9501285443359,93.,-78.4029932171361));
#61100=CARTESIAN_POINT('',(2.43861982758224,93.,-80.5515958942137));
#61101=CARTESIAN_POINT('',(4.4874473423585,93.,-87.2286885621189));
#61102=CARTESIAN_POINT('',(7.17571369007852,93.,-88.2806188720963));
#61103=CARTESIAN_POINT('',(-2.70550048791402,93.,-84.414056802447));
#61104=CARTESIAN_POINT('',(7.60884849248723,93.,-91.1346909763494));
#61105=CARTESIAN_POINT('',(5.41493158326502,93.,-76.6782284274182));
#61106=CARTESIAN_POINT('',(5.35371694717591,93.,-92.936832770625));
#61107=CARTESIAN_POINT('',(9.61484001483125,93.,-89.5316442853947));
#61108=CARTESIAN_POINT('',(2.66545059945588,93.,-91.8849024606476));
#61109=CARTESIAN_POINT('',(-4.52749723081663,93.,-89.0702707009757));
#61110=CARTESIAN_POINT('',(2.23231579704715,93.,-89.0308303563946));
#61111=CARTESIAN_POINT('',(0.471533690233556,93.,-77.4284399117164));
#61112=CARTESIAN_POINT('',(6.49343886470249,93.,-85.6256418711642));
#61113=CARTESIAN_POINT('',(39.4090515813242,93.,-100.893664133888));
#61114=CARTESIAN_POINT('',(42.0973179290442,93.,-101.945594443866));
#61115=CARTESIAN_POINT('',(-2.70550048791405,93.,-84.414056802447));
#61116=CARTESIAN_POINT('',(42.5304527314529,93.,-104.799666548119));
#61117=CARTESIAN_POINT('',(37.5232427561124,93.,-71.8054619003202));
#61118=CARTESIAN_POINT('',(40.2753211861416,93.,-106.601808342394));
#61119=CARTESIAN_POINT('',(29.8889352004325,93.,-114.901874170147));
#61120=CARTESIAN_POINT('',(37.5870548384215,93.,-105.549878032417));
#61121=CARTESIAN_POINT('',(-4.52749723081663,93.,-89.0702707009757));
#61122=CARTESIAN_POINT('',(37.1539200360128,93.,-102.695805928164));
#61123=CARTESIAN_POINT('',(32.5798448630808,93.,-72.5556733846182));
#61124=CARTESIAN_POINT('',(26.7675340503037,93.,-110.995871755917));
#61125=CARTESIAN_POINT('',(-45.5281158186408,93.,-60.6826259220946));
#61126=CARTESIAN_POINT('',(-42.8398494709208,93.,-61.734556232072));
#61127=CARTESIAN_POINT('',(-0.338657290464777,93.,-78.3654575200768));
#61128=CARTESIAN_POINT('',(-42.4067146685121,93.,-64.5886283363251));
#61129=CARTESIAN_POINT('',(-39.5367040587214,93.,-83.5001015653555));
#61130=CARTESIAN_POINT('',(-44.6618462138234,93.,-66.3907701306008));
#61131=CARTESIAN_POINT('',(-22.8237122821307,93.,-48.9392764697909));
#61132=CARTESIAN_POINT('',(-47.3501125615434,93.,-65.3388398206233));
#61133=CARTESIAN_POINT('',(-2.16065403336742,93.,-83.0216714186056));
#61134=CARTESIAN_POINT('',(-47.7832473639521,93.,-62.4847677163703));
#61135=CARTESIAN_POINT('',(-44.4801019517526,93.,-84.250313049654));
#61136=CARTESIAN_POINT('',(-25.9451134322595,93.,-45.0332740555604));
#61137=CARTESIAN_POINT('',(-38.5437949708476,93.,-63.4156210364485));
#61138=CARTESIAN_POINT('',(-35.8555286231276,93.,-64.4675513464259));
#61139=CARTESIAN_POINT('',(-0.338657290464782,93.,-78.3654575200768));
#61140=CARTESIAN_POINT('',(-35.4223938207189,93.,-67.321623450679));
#61141=CARTESIAN_POINT('',(-33.1150418241519,93.,-82.5255482599359));
#61142=CARTESIAN_POINT('',(-37.6775253660303,93.,-69.1237652449547));
#61143=CARTESIAN_POINT('',(-18.7688932450105,93.,-54.0133224467414));
#61144=CARTESIAN_POINT('',(-40.3657917137503,93.,-68.0718349349772));
#61145=CARTESIAN_POINT('',(-2.16065403336742,93.,-83.0216714186056));
#61146=CARTESIAN_POINT('',(-40.798926516159,93.,-65.2177628307242));
#61147=CARTESIAN_POINT('',(-38.0584397171832,93.,-83.2757597442344));
#61148=CARTESIAN_POINT('',(-21.8902943951393,93.,-50.1073200325109));
#61149=CARTESIAN_POINT('',(-31.5594741230545,93.,-66.1486161508024));
#61150=CARTESIAN_POINT('',(-28.8712077753345,93.,-67.2005464607798));
#61151=CARTESIAN_POINT('',(-0.338657290464787,93.,-78.3654575200768));
#61152=CARTESIAN_POINT('',(-28.4380729729258,93.,-70.0546185650329));
#61153=CARTESIAN_POINT('',(-26.6933795895825,93.,-81.5509949545163));
#61154=CARTESIAN_POINT('',(-30.6932045182371,93.,-71.8567603593086));
#61155=CARTESIAN_POINT('',(-14.7140742078902,93.,-59.0873684236919));
#61156=CARTESIAN_POINT('',(-33.3814708659571,93.,-70.8048300493311));
#61157=CARTESIAN_POINT('',(-2.16065403336742,93.,-83.0216714186056));
#61158=CARTESIAN_POINT('',(-33.8146056683659,93.,-67.9507579450781));
#61159=CARTESIAN_POINT('',(-31.6367774826137,93.,-82.3012064388147));
#61160=CARTESIAN_POINT('',(-17.835475358019,93.,-55.1813660094614));
#61161=CARTESIAN_POINT('',(32.424730733531,93.,-98.1606690195344));
#61162=CARTESIAN_POINT('',(35.112997081251,93.,-99.2125993295118));
#61163=CARTESIAN_POINT('',(-2.70550048791404,93.,-84.414056802447));
#61164=CARTESIAN_POINT('',(35.5461318836598,93.,-102.066671433765));
#61165=CARTESIAN_POINT('',(31.1015805215429,93.,-72.7800152057398));
#61166=CARTESIAN_POINT('',(33.2910003383484,93.,-103.868813228041));
#61167=CARTESIAN_POINT('',(25.8341161633122,93.,-109.827828193197));
#61168=CARTESIAN_POINT('',(30.6027339906284,93.,-102.816882918063));
#61169=CARTESIAN_POINT('',(-4.52749723081663,93.,-89.0702707009757));
#61170=CARTESIAN_POINT('',(30.1695991882197,93.,-99.9628108138101));
#61171=CARTESIAN_POINT('',(26.1581826285114,93.,-73.5302266900378));
#61172=CARTESIAN_POINT('',(22.7127150131835,93.,-105.921825778966));
#61173=CARTESIAN_POINT('',(25.4404098857379,93.,-95.4276739051805));
#61174=CARTESIAN_POINT('',(28.1286762334579,93.,-96.479604215158));
#61175=CARTESIAN_POINT('',(-2.70550048791404,93.,-84.414056802447));
#61176=CARTESIAN_POINT('',(28.5618110358666,93.,-99.3336763194111));
#61177=CARTESIAN_POINT('',(24.6799182869735,93.,-73.7545685111594));
#61178=CARTESIAN_POINT('',(26.3066794905553,93.,-101.135818113687));
#61179=CARTESIAN_POINT('',(21.779297126192,93.,-104.753782216246));
#61180=CARTESIAN_POINT('',(23.6184131428353,93.,-100.083887803709));
#61181=CARTESIAN_POINT('',(-4.52749723081663,93.,-89.0702707009757));
#61182=CARTESIAN_POINT('',(23.1852783404265,93.,-97.2298156994562));
#61183=CARTESIAN_POINT('',(19.7365203939419,93.,-74.5047799954575));
#61184=CARTESIAN_POINT('',(18.6578959760632,93.,-100.847779802016));
#61185=CARTESIAN_POINT('',(18.4560890379448,93.,-92.6946787908267));
#61186=CARTESIAN_POINT('',(21.1443553856648,93.,-93.7466091008041));
#61187=CARTESIAN_POINT('',(-2.70550048791403,93.,-84.414056802447));
#61188=CARTESIAN_POINT('',(21.5774901880735,93.,-96.6006812050572));
#61189=CARTESIAN_POINT('',(18.258256052404,93.,-74.729121816579));
#61190=CARTESIAN_POINT('',(19.3223586427622,93.,-98.4028229993328));
#61191=CARTESIAN_POINT('',(17.7244780890717,93.,-99.6797362392957));
#61192=CARTESIAN_POINT('',(16.6340922950421,93.,-97.3508926893554));
#61193=CARTESIAN_POINT('',(-4.52749723081663,93.,-89.0702707009757));
#61194=CARTESIAN_POINT('',(16.2009574926334,93.,-94.4968205851023));
#61195=CARTESIAN_POINT('',(13.3148581593725,93.,-75.4793333008771));
#61196=CARTESIAN_POINT('',(14.603076938943,93.,-95.7737338250652));
#61197=CARTESIAN_POINT('',(11.4717681901516,93.,-89.9616836764728));
#61198=CARTESIAN_POINT('',(14.1600345378716,93.,-91.0136139864502));
#61199=CARTESIAN_POINT('',(-2.70550048791403,93.,-84.414056802447));
#61200=CARTESIAN_POINT('',(14.5931693402804,93.,-93.8676860907033));
#61201=CARTESIAN_POINT('',(11.8365938178345,93.,-75.7036751219986));
#61202=CARTESIAN_POINT('',(12.338037794969,93.,-95.6698278849789));
#61203=CARTESIAN_POINT('',(13.6696590519515,93.,-94.6056902623452));
#61204=CARTESIAN_POINT('',(9.64977144724901,93.,-94.6178975750015));
#61205=CARTESIAN_POINT('',(-4.52749723081663,93.,-89.0702707009757));
#61206=CARTESIAN_POINT('',(9.21663664484028,93.,-91.7638254707484));
#61207=CARTESIAN_POINT('',(6.89319592480301,93.,-76.4538866062968));
#61208=CARTESIAN_POINT('',(10.5482579018227,93.,-90.6996878481147));
#61209=CARTESIAN_POINT('',(36.033099901982,93.,-78.6483736152472));
#61210=CARTESIAN_POINT('',(38.721366249702,93.,-79.7003039252246));
#61211=CARTESIAN_POINT('',(4.39502910443358,93.,-66.2682589553367));
#61212=CARTESIAN_POINT('',(39.1545010521108,93.,-82.5543760294777));
#61213=CARTESIAN_POINT('',(37.5232427561122,93.,-71.8054619003202));
#61214=CARTESIAN_POINT('',(36.8993695067994,93.,-84.3565178237533));
#61215=CARTESIAN_POINT('',(17.7244780890717,93.,-99.6797362392957));
#61216=CARTESIAN_POINT('',(34.2111031590794,93.,-83.3045875137759));
#61217=CARTESIAN_POINT('',(2.57303236153103,93.,-70.9244728538654));
#61218=CARTESIAN_POINT('',(33.7779683566707,93.,-80.4505154095229));
#61219=CARTESIAN_POINT('',(32.5798448630807,93.,-72.5556733846182));
#61220=CARTESIAN_POINT('',(14.603076938943,93.,-95.7737338250652));
#61221=CARTESIAN_POINT('',(43.0174207497752,93.,-81.381368729601));
#61222=CARTESIAN_POINT('',(45.7056870974952,93.,-82.4332990395785));
#61223=CARTESIAN_POINT('',(4.39502910443358,93.,-66.2682589553367));
#61224=CARTESIAN_POINT('',(46.1388218999039,93.,-85.2873711438316));
#61225=CARTESIAN_POINT('',(43.9449049906817,93.,-70.8309085949006));
#61226=CARTESIAN_POINT('',(43.8836903545926,93.,-87.0895129381072));
#61227=CARTESIAN_POINT('',(21.779297126192,93.,-104.753782216246));
#61228=CARTESIAN_POINT('',(41.1954240068725,93.,-86.0375826281298));
#61229=CARTESIAN_POINT('',(2.57303236153103,93.,-70.9244728538654));
#61230=CARTESIAN_POINT('',(40.7622892044638,93.,-83.1835105238767));
#61231=CARTESIAN_POINT('',(39.0015070976502,93.,-71.5811200791985));
#61232=CARTESIAN_POINT('',(18.6578959760632,93.,-100.847779802016));
#61233=CARTESIAN_POINT('',(50.0017415975683,93.,-84.1143638439549));
#61234=CARTESIAN_POINT('',(52.6900079452883,93.,-85.1662941539323));
#61235=CARTESIAN_POINT('',(4.39502910443357,93.,-66.2682589553367));
#61236=CARTESIAN_POINT('',(53.123142747697,93.,-88.0203662581854));
#61237=CARTESIAN_POINT('',(50.3665672252512,93.,-69.856355289481));
#61238=CARTESIAN_POINT('',(50.8680112023857,93.,-89.8225080524611));
#61239=CARTESIAN_POINT('',(25.8341161633122,93.,-109.827828193197));
#61240=CARTESIAN_POINT('',(48.1797448546657,93.,-88.7705777424837));
#61241=CARTESIAN_POINT('',(2.57303236153103,93.,-70.9244728538654));
#61242=CARTESIAN_POINT('',(47.7466100522569,93.,-85.9165056382306));
#61243=CARTESIAN_POINT('',(45.4231693322196,93.,-70.6065667737789));
#61244=CARTESIAN_POINT('',(22.7127150131835,93.,-105.921825778966));
#61245=CARTESIAN_POINT('',(-41.9197466501898,93.,-41.1703305178073));
#61246=CARTESIAN_POINT('',(-39.2314803024698,93.,-42.2222608277847));
#61247=CARTESIAN_POINT('',(6.76187230188284,93.,-60.2196596729665));
#61248=CARTESIAN_POINT('',(-38.798345500061,93.,-45.0763329320378));
#61249=CARTESIAN_POINT('',(-33.1150418241522,93.,-82.525548259936));
#61250=CARTESIAN_POINT('',(-41.0534770453724,93.,-46.8784747263135));
#61251=CARTESIAN_POINT('',(-30.9333503563712,93.,-38.7911845158899));
#61252=CARTESIAN_POINT('',(-43.7417433930924,93.,-45.8265444163361));
#61253=CARTESIAN_POINT('',(4.93987555898024,93.,-64.8758735714953));
#61254=CARTESIAN_POINT('',(-44.1748781955011,93.,-42.972472312083));
#61255=CARTESIAN_POINT('',(-38.0584397171832,93.,-83.2757597442344));
#61256=CARTESIAN_POINT('',(-34.0547515065,93.,-34.8851821016595));
#61257=CARTESIAN_POINT('',(29.0487790541889,93.,-75.9153785008933));
#61258=CARTESIAN_POINT('',(31.7370454019089,93.,-76.9673088108707));
#61259=CARTESIAN_POINT('',(4.39502910443359,93.,-66.2682589553367));
#61260=CARTESIAN_POINT('',(32.1701802043176,93.,-79.8213809151238));
#61261=CARTESIAN_POINT('',(31.1015805215427,93.,-72.7800152057398));
#61262=CARTESIAN_POINT('',(29.9150486590063,93.,-81.6235227093995));
#61263=CARTESIAN_POINT('',(13.6696590519515,93.,-94.6056902623452));
#61264=CARTESIAN_POINT('',(27.2267823112863,93.,-80.571592399422));
#61265=CARTESIAN_POINT('',(2.57303236153103,93.,-70.9244728538654));
#61266=CARTESIAN_POINT('',(26.7936475088776,93.,-77.717520295169));
#61267=CARTESIAN_POINT('',(26.1581826285113,93.,-73.5302266900378));
#61268=CARTESIAN_POINT('',(10.5482579018228,93.,-90.6996878481147));
#61269=CARTESIAN_POINT('',(22.0644582063958,93.,-73.1823833865394));
#61270=CARTESIAN_POINT('',(24.7527245541158,93.,-74.2343136965168));
#61271=CARTESIAN_POINT('',(4.39502910443359,93.,-66.2682589553367));
#61272=CARTESIAN_POINT('',(25.1858593565245,93.,-77.0883858007699));
#61273=CARTESIAN_POINT('',(24.6799182869733,93.,-73.7545685111594));
#61274=CARTESIAN_POINT('',(22.9307278112132,93.,-78.8905275950456));
#61275=CARTESIAN_POINT('',(9.61484001483124,93.,-89.5316442853947));
#61276=CARTESIAN_POINT('',(20.2424614634932,93.,-77.8385972850681));
#61277=CARTESIAN_POINT('',(2.57303236153103,93.,-70.9244728538654));
#61278=CARTESIAN_POINT('',(19.8093266610844,93.,-74.9845251808151));
#61279=CARTESIAN_POINT('',(19.7365203939419,93.,-74.5047799954575));
#61280=CARTESIAN_POINT('',(6.4934388647025,93.,-85.6256418711642));
#61281=CARTESIAN_POINT('',(15.0801373586026,93.,-70.4493882721855));
#61282=CARTESIAN_POINT('',(17.7684037063227,93.,-71.5013185821629));
#61283=CARTESIAN_POINT('',(4.3950291044336,93.,-66.2682589553367));
#61284=CARTESIAN_POINT('',(18.2015385087314,93.,-74.355390686416));
#61285=CARTESIAN_POINT('',(18.2582560524038,93.,-74.729121816579));
#61286=CARTESIAN_POINT('',(15.94640696342,93.,-76.1575324806917));
#61287=CARTESIAN_POINT('',(5.560020977711,93.,-84.4575983084442));
#61288=CARTESIAN_POINT('',(13.2581406157,93.,-75.1056021707142));
#61289=CARTESIAN_POINT('',(2.57303236153103,93.,-70.9244728538654));
#61290=CARTESIAN_POINT('',(12.8250058132913,93.,-72.2515300664612));
#61291=CARTESIAN_POINT('',(13.3148581593724,93.,-75.4793333008771));
#61292=CARTESIAN_POINT('',(2.43861982758225,93.,-80.5515958942137));
#61293=CARTESIAN_POINT('',(8.09581651080951,93.,-67.7163931578316));
#61294=CARTESIAN_POINT('',(10.7840828585295,93.,-68.768323467809));
#61295=CARTESIAN_POINT('',(4.3950291044336,93.,-66.2682589553366));
#61296=CARTESIAN_POINT('',(11.2172176609382,93.,-71.6223955720621));
#61297=CARTESIAN_POINT('',(11.8365938178343,93.,-75.7036751219986));
#61298=CARTESIAN_POINT('',(8.96208611562692,93.,-73.4245373663378));
#61299=CARTESIAN_POINT('',(1.50520194059076,93.,-79.3835523314937));
#61300=CARTESIAN_POINT('',(6.27381976790689,93.,-72.3726070563604));
#61301=CARTESIAN_POINT('',(2.57303236153103,93.,-70.9244728538654));
#61302=CARTESIAN_POINT('',(5.84068496549816,93.,-69.5185349521073));
#61303=CARTESIAN_POINT('',(6.89319592480295,93.,-76.4538866062968));
#61304=CARTESIAN_POINT('',(-1.616199209538,93.,-75.4775499172633));
#61305=CARTESIAN_POINT('',(-34.9354258023966,93.,-43.9033256321612));
#61306=CARTESIAN_POINT('',(-32.2471594546766,93.,-44.9552559421386));
#61307=CARTESIAN_POINT('',(6.76187230188284,93.,-60.2196596729665));
#61308=CARTESIAN_POINT('',(-31.8140246522679,93.,-47.8093280463917));
#61309=CARTESIAN_POINT('',(-26.6933795895827,93.,-81.5509949545163));
#61310=CARTESIAN_POINT('',(-34.0691561975792,93.,-49.6114698406674));
#61311=CARTESIAN_POINT('',(-26.878531319251,93.,-43.8652304928404));
#61312=CARTESIAN_POINT('',(-36.7574225452993,93.,-48.55953953069));
#61313=CARTESIAN_POINT('',(4.93987555898024,93.,-64.8758735714953));
#61314=CARTESIAN_POINT('',(-37.190557347708,93.,-45.7054674264369));
#61315=CARTESIAN_POINT('',(-31.6367774826138,93.,-82.3012064388147));
#61316=CARTESIAN_POINT('',(-29.9999324693798,93.,-39.95922807861));
#61317=CARTESIAN_POINT('',(-27.9511049546035,93.,-46.6363207465151));
#61318=CARTESIAN_POINT('',(-25.2628386068835,93.,-47.6882510564925));
#61319=CARTESIAN_POINT('',(6.76187230188283,93.,-60.2196596729665));
#61320=CARTESIAN_POINT('',(-24.8297038044748,93.,-50.5423231607456));
#61321=CARTESIAN_POINT('',(-20.2717173550132,93.,-80.5764416490967));
#61322=CARTESIAN_POINT('',(-27.0848353497861,93.,-52.3444649550213));
#61323=CARTESIAN_POINT('',(-22.8237122821307,93.,-48.9392764697909));
#61324=CARTESIAN_POINT('',(-29.7731016975061,93.,-51.2925346450439));
#61325=CARTESIAN_POINT('',(4.93987555898024,93.,-64.8758735714953));
#61326=CARTESIAN_POINT('',(-30.2062364999149,93.,-48.4384625407908));
#61327=CARTESIAN_POINT('',(-25.2151152480443,93.,-81.3266531333951));
#61328=CARTESIAN_POINT('',(-25.9451134322595,93.,-45.0332740555604));
#61329=CARTESIAN_POINT('',(-20.9667841068104,93.,-49.369315860869));
#61330=CARTESIAN_POINT('',(-18.2785177590904,93.,-50.4212461708464));
#61331=CARTESIAN_POINT('',(6.76187230188283,93.,-60.2196596729665));
#61332=CARTESIAN_POINT('',(-17.8453829566817,93.,-53.2753182750995));
#61333=CARTESIAN_POINT('',(-13.8500551204437,93.,-79.6018883436771));
#61334=CARTESIAN_POINT('',(-20.100514501993,93.,-55.0774600693752));
#61335=CARTESIAN_POINT('',(-18.7688932450105,93.,-54.0133224467414));
#61336=CARTESIAN_POINT('',(-22.788780849713,93.,-54.0255297593977));
#61337=CARTESIAN_POINT('',(4.93987555898024,93.,-64.8758735714953));
#61338=CARTESIAN_POINT('',(-23.2219156521217,93.,-51.1714576551447));
#61339=CARTESIAN_POINT('',(-18.7934530134749,93.,-80.3520998279754));
#61340=CARTESIAN_POINT('',(-21.8902943951393,93.,-50.1073200325109));
#61341=CARTESIAN_POINT('',(-13.9824632590173,93.,-52.1023109752229));
#61342=CARTESIAN_POINT('',(-11.2941969112972,93.,-53.1542412852003));
#61343=CARTESIAN_POINT('',(6.76187230188282,93.,-60.2196596729665));
#61344=CARTESIAN_POINT('',(-10.8610621088885,93.,-56.0083133894534));
#61345=CARTESIAN_POINT('',(-7.42839288587424,93.,-78.6273350382575));
#61346=CARTESIAN_POINT('',(-13.1161936541999,93.,-57.8104551837291));
#61347=CARTESIAN_POINT('',(-14.7140742078902,93.,-59.0873684236919));
#61348=CARTESIAN_POINT('',(-15.8044600019199,93.,-56.7585248737516));
#61349=CARTESIAN_POINT('',(4.93987555898024,93.,-64.8758735714953));
#61350=CARTESIAN_POINT('',(-16.2375948043286,93.,-53.9044527694986));
#61351=CARTESIAN_POINT('',(-12.3717907789054,93.,-79.3775465225558));
#61352=CARTESIAN_POINT('',(-17.835475358019,93.,-55.1813660094614));
#61353=CARTESIAN_POINT('',(-6.99814241122413,93.,-54.8353060895768));
#61354=CARTESIAN_POINT('',(-4.30987606350412,93.,-55.8872363995542));
#61355=CARTESIAN_POINT('',(6.76187230188282,93.,-60.2196596729665));
#61356=CARTESIAN_POINT('',(-3.8767412610954,93.,-58.7413085038073));
#61357=CARTESIAN_POINT('',(-1.00673065130475,93.,-77.6527817328379));
#61358=CARTESIAN_POINT('',(-6.13187280640672,93.,-60.5434502980829));
#61359=CARTESIAN_POINT('',(-10.65925517077,93.,-64.1614144006423));
#61360=CARTESIAN_POINT('',(-8.82013915412675,93.,-59.4915199881055));
#61361=CARTESIAN_POINT('',(4.93987555898024,93.,-64.8758735714953));
#61362=CARTESIAN_POINT('',(-9.25327395653548,93.,-56.6374478838525));
#61363=CARTESIAN_POINT('',(-5.95012854433598,93.,-78.4029932171361));
#61364=CARTESIAN_POINT('',(-13.7806563208988,93.,-60.2554119864119));
#61365=CARTESIAN_POINT('',(-0.0138215634309935,93.,-57.5683012039307));
#61366=CARTESIAN_POINT('',(2.67444478428902,93.,-58.6202315139081));
#61367=CARTESIAN_POINT('',(6.76187230188281,93.,-60.2196596729665));
#61368=CARTESIAN_POINT('',(3.10757958669774,93.,-61.4743036181612));
#61369=CARTESIAN_POINT('',(5.41493158326473,93.,-76.6782284274183));
#61370=CARTESIAN_POINT('',(0.852448041386411,93.,-63.2764454124368));
#61371=CARTESIAN_POINT('',(-6.60443613364974,93.,-69.2354603775928));
#61372=CARTESIAN_POINT('',(-1.83581830633362,93.,-62.2245151024594));
#61373=CARTESIAN_POINT('',(4.93987555898025,93.,-64.8758735714953));
#61374=CARTESIAN_POINT('',(-2.26895310874235,93.,-59.3704429982063));
#61375=CARTESIAN_POINT('',(0.471533690233477,93.,-77.4284399117164));
#61376=CARTESIAN_POINT('',(-9.7258372837785,93.,-65.3294579633623));
#61377=CARTESIAN_POINT('',(6.97049928436214,93.,-60.3012963182845));
#61378=CARTESIAN_POINT('',(9.65876563208215,93.,-61.353226628262));
#61379=CARTESIAN_POINT('',(6.76187230188281,93.,-60.2196596729665));
#61380=CARTESIAN_POINT('',(10.0919004344909,93.,-64.2072987325151));
#61381=CARTESIAN_POINT('',(11.8365938178342,93.,-75.7036751219986));
#61382=CARTESIAN_POINT('',(7.83676888917954,93.,-66.0094405267907));
#61383=CARTESIAN_POINT('',(-2.54961709652949,93.,-74.3095063545433));
#61384=CARTESIAN_POINT('',(5.14850254145952,93.,-64.9575102168133));
#61385=CARTESIAN_POINT('',(4.93987555898025,93.,-64.8758735714953));
#61386=CARTESIAN_POINT('',(4.71536773905078,93.,-62.1034381125602));
#61387=CARTESIAN_POINT('',(6.89319592480293,93.,-76.4538866062968));
#61388=CARTESIAN_POINT('',(-5.67101824665825,93.,-70.4035039403128));
#61389=CARTESIAN_POINT('',(13.9548201321553,93.,-63.0342914326384));
#61390=CARTESIAN_POINT('',(16.6430864798753,93.,-64.0862217426158));
#61391=CARTESIAN_POINT('',(6.7618723018828,93.,-60.2196596729666));
#61392=CARTESIAN_POINT('',(17.076221282284,93.,-66.940293846869));
#61393=CARTESIAN_POINT('',(18.2582560524037,93.,-74.729121816579));
#61394=CARTESIAN_POINT('',(14.8210897369727,93.,-68.7424356411446));
#61395=CARTESIAN_POINT('',(1.50520194059075,93.,-79.3835523314937));
#61396=CARTESIAN_POINT('',(12.1328233892526,93.,-67.6905053311672));
#61397=CARTESIAN_POINT('',(4.93987555898025,93.,-64.8758735714953));
#61398=CARTESIAN_POINT('',(11.6996885868439,93.,-64.8364332269141));
#61399=CARTESIAN_POINT('',(13.3148581593724,93.,-75.4793333008771));
#61400=CARTESIAN_POINT('',(-1.616199209538,93.,-75.4775499172633));
#61401=CARTESIAN_POINT('',(-11.7318288061225,93.,-66.932504654317));
#61402=CARTESIAN_POINT('',(-9.04356245840249,93.,-67.9844349642944));
#61403=CARTESIAN_POINT('',(2.02818590698441,93.,-72.3168582377067));
#61404=CARTESIAN_POINT('',(-8.61042765599378,93.,-70.8385070685475));
#61405=CARTESIAN_POINT('',(-7.42839288587409,93.,-78.6273350382575));
#61406=CARTESIAN_POINT('',(-10.8655592013051,93.,-72.6406488628232));
#61407=CARTESIAN_POINT('',(-6.60443613364973,93.,-69.2354603775928));
#61408=CARTESIAN_POINT('',(-13.5538255490251,93.,-71.5887185528457));
#61409=CARTESIAN_POINT('',(0.206189164081805,93.,-76.9730721362355));
#61410=CARTESIAN_POINT('',(-13.9869603514339,93.,-68.7346464485927));
#61411=CARTESIAN_POINT('',(-12.3717907789054,93.,-79.3775465225557));
#61412=CARTESIAN_POINT('',(-9.72583728377851,93.,-65.3294579633623));
#61413=CARTESIAN_POINT('',(-4.74750795832937,93.,-69.6654997686709));
#61414=CARTESIAN_POINT('',(-2.05924161060936,93.,-70.7174300786483));
#61415=CARTESIAN_POINT('',(2.0281859069844,93.,-72.3168582377067));
#61416=CARTESIAN_POINT('',(-1.62610680820064,93.,-73.5715021829014));
#61417=CARTESIAN_POINT('',(-1.00673065130461,93.,-77.6527817328379));
#61418=CARTESIAN_POINT('',(-3.88123835351197,93.,-75.3736439771771));
#61419=CARTESIAN_POINT('',(-2.54961709652949,93.,-74.3095063545433));
#61420=CARTESIAN_POINT('',(-6.569504701232,93.,-74.3217136671996));
#61421=CARTESIAN_POINT('',(0.206189164081806,93.,-76.9730721362355));
#61422=CARTESIAN_POINT('',(-7.00263950364073,93.,-71.4676415629466));
#61423=CARTESIAN_POINT('',(-5.95012854433593,93.,-78.4029932171361));
#61424=CARTESIAN_POINT('',(-5.67101824665825,93.,-70.4035039403128));
#61425=CARTESIAN_POINT('',(2.23681288946376,93.,-72.3984948830248));
#61426=CARTESIAN_POINT('',(4.92507923718377,93.,-73.4504251930022));
#61427=CARTESIAN_POINT('',(2.0281859069844,93.,-72.3168582377067));
#61428=CARTESIAN_POINT('',(5.35821403959249,93.,-76.3044972972553));
#61429=CARTESIAN_POINT('',(5.41493158326488,93.,-76.6782284274182));
#61430=CARTESIAN_POINT('',(3.10308249428116,93.,-78.1066390915309));
#61431=CARTESIAN_POINT('',(1.50520194059076,93.,-79.3835523314937));
#61432=CARTESIAN_POINT('',(0.414816146561137,93.,-77.0547087815535));
#61433=CARTESIAN_POINT('',(0.206189164081808,93.,-76.9730721362355));
#61434=CARTESIAN_POINT('',(-0.0183186558475948,93.,-74.2006366773005));
#61435=CARTESIAN_POINT('',(0.471533690233522,93.,-77.4284399117164));
#61436=CARTESIAN_POINT('',(-1.616199209538,93.,-75.4775499172633));
#61437=CARTESIAN_POINT('',(9.22113373725689,93.,-75.1314899973787));
#61438=CARTESIAN_POINT('',(11.9094000849769,93.,-76.1834203073561));
#61439=CARTESIAN_POINT('',(2.02818590698439,93.,-72.3168582377068));
#61440=CARTESIAN_POINT('',(12.3425348873856,93.,-79.0374924116092));
#61441=CARTESIAN_POINT('',(11.8365938178344,93.,-75.7036751219986));
#61442=CARTESIAN_POINT('',(10.0874033420743,93.,-80.8396342058848));
#61443=CARTESIAN_POINT('',(5.560020977711,93.,-84.4575983084442));
#61444=CARTESIAN_POINT('',(7.39913699435427,93.,-79.7877038959074));
#61445=CARTESIAN_POINT('',(0.206189164081809,93.,-76.9730721362355));
#61446=CARTESIAN_POINT('',(6.96600219194553,93.,-76.9336317916543));
#61447=CARTESIAN_POINT('',(6.89319592480297,93.,-76.4538866062968));
#61448=CARTESIAN_POINT('',(2.43861982758225,93.,-80.5515958942137));
#61449=CARTESIAN_POINT('',(16.20545458505,93.,-77.8644851117325));
#61450=CARTESIAN_POINT('',(18.89372093277,93.,-78.9164154217099));
#61451=CARTESIAN_POINT('',(2.02818590698439,93.,-72.3168582377068));
#61452=CARTESIAN_POINT('',(19.3268557351787,93.,-81.770487525963));
#61453=CARTESIAN_POINT('',(18.2582560524038,93.,-74.729121816579));
#61454=CARTESIAN_POINT('',(17.0717241898674,93.,-83.5726293202387));
#61455=CARTESIAN_POINT('',(9.61484001483125,93.,-89.5316442853947));
#61456=CARTESIAN_POINT('',(14.3834578421474,93.,-82.5206990102613));
#61457=CARTESIAN_POINT('',(0.20618916408181,93.,-76.9730721362355));
#61458=CARTESIAN_POINT('',(13.9503230397387,93.,-79.6666269060082));
#61459=CARTESIAN_POINT('',(13.3148581593724,93.,-75.4793333008771));
#61460=CARTESIAN_POINT('',(6.4934388647025,93.,-85.6256418711642));
#61461=CARTESIAN_POINT('',(23.1897754328432,93.,-80.5974802260864));
#61462=CARTESIAN_POINT('',(25.8780417805632,93.,-81.6494105360638));
#61463=CARTESIAN_POINT('',(2.02818590698438,93.,-72.3168582377068));
#61464=CARTESIAN_POINT('',(26.3111765829719,93.,-84.5034826403169));
#61465=CARTESIAN_POINT('',(24.6799182869733,93.,-73.7545685111594));
#61466=CARTESIAN_POINT('',(24.0560450376606,93.,-86.3056244345926));
#61467=CARTESIAN_POINT('',(13.6696590519515,93.,-94.6056902623452));
#61468=CARTESIAN_POINT('',(21.3677786899405,93.,-85.2536941246152));
#61469=CARTESIAN_POINT('',(0.206189164081811,93.,-76.9730721362355));
#61470=CARTESIAN_POINT('',(20.9346438875318,93.,-82.3996220203621));
#61471=CARTESIAN_POINT('',(19.7365203939419,93.,-74.5047799954575));
#61472=CARTESIAN_POINT('',(10.5482579018228,93.,-90.6996878481147));
#61473=CARTESIAN_POINT('',(30.1740962806363,93.,-83.3304753404403));
#61474=CARTESIAN_POINT('',(32.8623626283563,93.,-84.3824056504177));
#61475=CARTESIAN_POINT('',(2.02818590698438,93.,-72.3168582377068));
#61476=CARTESIAN_POINT('',(33.295497430765,93.,-87.2364777546708));
#61477=CARTESIAN_POINT('',(31.1015805215428,93.,-72.7800152057398));
#61478=CARTESIAN_POINT('',(31.0403658854537,93.,-89.0386195489465));
#61479=CARTESIAN_POINT('',(17.7244780890717,93.,-99.6797362392957));
#61480=CARTESIAN_POINT('',(28.3520995377337,93.,-87.9866892389691));
#61481=CARTESIAN_POINT('',(0.206189164081812,93.,-76.9730721362355));
#61482=CARTESIAN_POINT('',(27.9189647353249,93.,-85.132617134716));
#61483=CARTESIAN_POINT('',(26.1581826285113,93.,-73.5302266900378));
#61484=CARTESIAN_POINT('',(14.603076938943,93.,-95.7737338250652));
#61485=CARTESIAN_POINT('',(37.1584171284294,93.,-86.0634704547942));
#61486=CARTESIAN_POINT('',(39.8466834761494,93.,-87.1154007647716));
#61487=CARTESIAN_POINT('',(2.02818590698437,93.,-72.3168582377068));
#61488=CARTESIAN_POINT('',(40.2798182785581,93.,-89.9694728690247));
#61489=CARTESIAN_POINT('',(37.5232427561123,93.,-71.8054619003202));
#61490=CARTESIAN_POINT('',(38.0246867332468,93.,-91.7716146633004));
#61491=CARTESIAN_POINT('',(21.779297126192,93.,-104.753782216246));
#61492=CARTESIAN_POINT('',(35.3364203855268,93.,-90.719684353323));
#61493=CARTESIAN_POINT('',(0.206189164081812,93.,-76.9730721362355));
#61494=CARTESIAN_POINT('',(34.903285583118,93.,-87.8656122490699));
#61495=CARTESIAN_POINT('',(32.5798448630808,93.,-72.5556733846182));
#61496=CARTESIAN_POINT('',(18.6578959760632,93.,-100.847779802016));
#61497=CARTESIAN_POINT('',(1.11149566301639,93.,-64.9833980434777));
#61498=CARTESIAN_POINT('',(3.7997620107364,93.,-66.0353283534551));
#61499=CARTESIAN_POINT('',(4.39502910443361,93.,-66.2682589553366));
#61500=CARTESIAN_POINT('',(4.23289681314511,93.,-68.8894004577082));
#61501=CARTESIAN_POINT('',(5.41493158326481,93.,-76.6782284274183));
#61502=CARTESIAN_POINT('',(1.97776526783379,93.,-70.6915422519839));
#61503=CARTESIAN_POINT('',(-2.54961709652949,93.,-74.3095063545433));
#61504=CARTESIAN_POINT('',(-0.710501079886239,93.,-69.6396119420065));
#61505=CARTESIAN_POINT('',(2.57303236153103,93.,-70.9244728538654));
#61506=CARTESIAN_POINT('',(-1.14363588229497,93.,-66.7855398377534));
#61507=CARTESIAN_POINT('',(0.471533690233501,93.,-77.4284399117164));
#61508=CARTESIAN_POINT('',(-5.67101824665825,93.,-70.4035039403128));
#61509=CARTESIAN_POINT('',(-5.87282518477675,93.,-62.2504029291238));
#61510=CARTESIAN_POINT('',(-3.18455883705674,93.,-63.3023332391012));
#61511=CARTESIAN_POINT('',(4.39502910443361,93.,-66.2682589553366));
#61512=CARTESIAN_POINT('',(-2.75142403464802,93.,-66.1564053433543));
#61513=CARTESIAN_POINT('',(-1.00673065130468,93.,-77.6527817328379));
#61514=CARTESIAN_POINT('',(-5.00655557995934,93.,-67.95854713763));
#61515=CARTESIAN_POINT('',(-6.60443613364974,93.,-69.2354603775928));
#61516=CARTESIAN_POINT('',(-7.69482192767937,93.,-66.9066168276526));
#61517=CARTESIAN_POINT('',(2.57303236153103,93.,-70.9244728538654));
#61518=CARTESIAN_POINT('',(-8.1279567300881,93.,-64.0525447233995));
#61519=CARTESIAN_POINT('',(-5.95012854433595,93.,-78.4029932171361));
#61520=CARTESIAN_POINT('',(-9.7258372837785,93.,-65.3294579633623));
#61521=CARTESIAN_POINT('',(-12.8571460325699,93.,-59.5174078147699));
#61522=CARTESIAN_POINT('',(-10.1688796848499,93.,-60.5693381247473));
#61523=CARTESIAN_POINT('',(4.39502910443361,93.,-66.2682589553366));
#61524=CARTESIAN_POINT('',(-9.73574488244115,93.,-63.4234102290004));
#61525=CARTESIAN_POINT('',(-7.42839288587416,93.,-78.6273350382575));
#61526=CARTESIAN_POINT('',(-11.9908764277525,93.,-65.2255520232761));
#61527=CARTESIAN_POINT('',(-10.65925517077,93.,-64.1614144006423));
#61528=CARTESIAN_POINT('',(-14.6791427754725,93.,-64.1736217132987));
#61529=CARTESIAN_POINT('',(2.57303236153102,93.,-70.9244728538654));
#61530=CARTESIAN_POINT('',(-15.1122775778812,93.,-61.3195496090456));
#61531=CARTESIAN_POINT('',(-12.3717907789054,93.,-79.3775465225558));
#61532=CARTESIAN_POINT('',(-13.7806563208988,93.,-60.2554119864119));
#61533=CARTESIAN_POINT('',(-19.841466880363,93.,-56.784412700416));
#61534=CARTESIAN_POINT('',(-17.153200532643,93.,-57.8363430103935));
#61535=CARTESIAN_POINT('',(4.39502910443362,93.,-66.2682589553366));
#61536=CARTESIAN_POINT('',(-16.7200657302343,93.,-60.6904151146466));
#61537=CARTESIAN_POINT('',(-13.8500551204436,93.,-79.6018883436771));
#61538=CARTESIAN_POINT('',(-18.9751972755456,93.,-62.4925569089222));
#61539=CARTESIAN_POINT('',(-14.7140742078902,93.,-59.0873684236919));
#61540=CARTESIAN_POINT('',(-21.6634636232656,93.,-61.4406265989448));
#61541=CARTESIAN_POINT('',(2.57303236153102,93.,-70.9244728538654));
#61542=CARTESIAN_POINT('',(-22.0965984256744,93.,-58.5865544946917));
#61543=CARTESIAN_POINT('',(-18.7934530134749,93.,-80.3520998279754));
#61544=CARTESIAN_POINT('',(-17.835475358019,93.,-55.1813660094614));
#61545=CARTESIAN_POINT('',(44.1427379762225,93.,-88.7964655691481));
#61546=CARTESIAN_POINT('',(46.8310043239425,93.,-89.8483958791255));
#61547=CARTESIAN_POINT('',(2.02818590698437,93.,-72.3168582377068));
#61548=CARTESIAN_POINT('',(47.2641391263513,93.,-92.7024679833786));
#61549=CARTESIAN_POINT('',(43.9449049906818,93.,-70.8309085949006));
#61550=CARTESIAN_POINT('',(45.0090075810399,93.,-94.5046097776543));
#61551=CARTESIAN_POINT('',(25.8341161633122,93.,-109.827828193197));
#61552=CARTESIAN_POINT('',(42.3207412333199,93.,-93.4526794676769));
#61553=CARTESIAN_POINT('',(0.206189164081814,93.,-76.9730721362355));
#61554=CARTESIAN_POINT('',(41.8876064309112,93.,-90.5986073634238));
#61555=CARTESIAN_POINT('',(39.0015070976502,93.,-71.5811200791985));
#61556=CARTESIAN_POINT('',(22.7127150131835,93.,-105.921825778966));
#61557=CARTESIAN_POINT('',(-40.7944294237424,93.,-48.5854273573544));
#61558=CARTESIAN_POINT('',(-38.1061630760224,93.,-49.6373576673318));
#61559=CARTESIAN_POINT('',(4.39502910443363,93.,-66.2682589553366));
#61560=CARTESIAN_POINT('',(-37.6730282736137,93.,-52.4914297715849));
#61561=CARTESIAN_POINT('',(-33.1150418241521,93.,-82.5255482599359));
#61562=CARTESIAN_POINT('',(-39.928159818925,93.,-54.2935715658606));
#61563=CARTESIAN_POINT('',(-26.878531319251,93.,-43.8652304928404));
#61564=CARTESIAN_POINT('',(-42.616426166645,93.,-53.2416412558831));
#61565=CARTESIAN_POINT('',(2.57303236153102,93.,-70.9244728538654));
#61566=CARTESIAN_POINT('',(-43.0495609690538,93.,-50.3875691516301));
#61567=CARTESIAN_POINT('',(-38.0584397171832,93.,-83.2757597442344));
#61568=CARTESIAN_POINT('',(-29.9999324693798,93.,-39.95922807861));
#61569=CARTESIAN_POINT('',(-33.8101085759493,93.,-51.3184224717083));
#61570=CARTESIAN_POINT('',(-31.1218422282293,93.,-52.3703527816857));
#61571=CARTESIAN_POINT('',(4.39502910443363,93.,-66.2682589553366));
#61572=CARTESIAN_POINT('',(-30.6887074258205,93.,-55.2244248859388));
#61573=CARTESIAN_POINT('',(-26.6933795895826,93.,-81.5509949545163));
#61574=CARTESIAN_POINT('',(-32.9438389711319,93.,-57.0265666802144));
#61575=CARTESIAN_POINT('',(-22.8237122821307,93.,-48.9392764697909));
#61576=CARTESIAN_POINT('',(-35.6321053188519,93.,-55.974636370237));
#61577=CARTESIAN_POINT('',(2.57303236153102,93.,-70.9244728538654));
#61578=CARTESIAN_POINT('',(-36.0652401212606,93.,-53.120564265984));
#61579=CARTESIAN_POINT('',(-31.6367774826138,93.,-82.3012064388147));
#61580=CARTESIAN_POINT('',(-25.9451134322595,93.,-45.0332740555604));
#61581=CARTESIAN_POINT('',(-26.8257877281561,93.,-54.0514175860622));
#61582=CARTESIAN_POINT('',(-24.1375213804361,93.,-55.1033478960396));
#61583=CARTESIAN_POINT('',(4.39502910443362,93.,-66.2682589553366));
#61584=CARTESIAN_POINT('',(-23.7043865780274,93.,-57.9574200002927));
#61585=CARTESIAN_POINT('',(-20.2717173550131,93.,-80.5764416490967));
#61586=CARTESIAN_POINT('',(-25.9595181233387,93.,-59.7595617945683));
#61587=CARTESIAN_POINT('',(-18.7688932450105,93.,-54.0133224467414));
#61588=CARTESIAN_POINT('',(-28.6477844710588,93.,-58.7076314845909));
#61589=CARTESIAN_POINT('',(2.57303236153102,93.,-70.9244728538654));
#61590=CARTESIAN_POINT('',(-29.0809192734675,93.,-55.8535593803378));
#61591=CARTESIAN_POINT('',(-25.2151152480443,93.,-81.3266531333951));
#61592=CARTESIAN_POINT('',(-21.8902943951393,93.,-50.1073200325109));
#61593=CARTESIAN_POINT('',(-25.9328879908176,93.,-103.224100348538));
#61594=CARTESIAN_POINT('',(-23.2446216430976,93.,-104.276030658515));
#61595=CARTESIAN_POINT('',(-12.1728732777108,93.,-108.608453931927));
#61596=CARTESIAN_POINT('',(-22.8114868406889,93.,-107.130102762768));
#61597=CARTESIAN_POINT('',(-26.6933795895821,93.,-81.5509949545162));
#61598=CARTESIAN_POINT('',(-25.0666183860002,93.,-108.932244557044));
#61599=CARTESIAN_POINT('',(5.56002097771103,93.,-84.4575983084443));
#61600=CARTESIAN_POINT('',(-27.7548847337203,93.,-107.880314247066));
#61601=CARTESIAN_POINT('',(-13.9948700206135,93.,-113.264667830456));
#61602=CARTESIAN_POINT('',(-28.188019536129,93.,-105.026242142813));
#61603=CARTESIAN_POINT('',(-31.6367774826136,93.,-82.3012064388147));
#61604=CARTESIAN_POINT('',(2.43861982758225,93.,-80.5515958942138));
#61605=CARTESIAN_POINT('',(-18.9485671430245,93.,-105.957095462892));
#61606=CARTESIAN_POINT('',(-16.2603007953045,93.,-107.009025772869));
#61607=CARTESIAN_POINT('',(-12.1728732777108,93.,-108.608453931927));
#61608=CARTESIAN_POINT('',(-15.8271659928958,93.,-109.863097877122));
#61609=CARTESIAN_POINT('',(-20.2717173550126,93.,-80.5764416490966));
#61610=CARTESIAN_POINT('',(-18.0822975382071,93.,-111.665239671398));
#61611=CARTESIAN_POINT('',(9.61484001483127,93.,-89.5316442853947));
#61612=CARTESIAN_POINT('',(-20.7705638859271,93.,-110.61330936142));
#61613=CARTESIAN_POINT('',(-13.9948700206135,93.,-113.264667830456));
#61614=CARTESIAN_POINT('',(-21.2036986883359,93.,-107.759237257167));
#61615=CARTESIAN_POINT('',(-25.2151152480442,93.,-81.326653133395));
#61616=CARTESIAN_POINT('',(6.4934388647025,93.,-85.6256418711642));
#61617=CARTESIAN_POINT('',(-11.9642462952314,93.,-108.690090577245));
#61618=CARTESIAN_POINT('',(-9.27597994751136,93.,-109.742020887223));
#61619=CARTESIAN_POINT('',(-12.1728732777108,93.,-108.608453931927));
#61620=CARTESIAN_POINT('',(-8.84284514510264,93.,-112.596092991476));
#61621=CARTESIAN_POINT('',(-13.8500551204431,93.,-79.601888343677));
#61622=CARTESIAN_POINT('',(-11.097976690414,93.,-114.398234785752));
#61623=CARTESIAN_POINT('',(13.6696590519515,93.,-94.6056902623452));
#61624=CARTESIAN_POINT('',(-13.786243038134,93.,-113.346304475774));
#61625=CARTESIAN_POINT('',(-13.9948700206135,93.,-113.264667830456));
#61626=CARTESIAN_POINT('',(-14.2193778405427,93.,-110.492232371521));
#61627=CARTESIAN_POINT('',(-18.7934530134747,93.,-80.3520998279754));
#61628=CARTESIAN_POINT('',(10.5482579018228,93.,-90.6996878481147));
#61629=CARTESIAN_POINT('',(-4.97992544743824,93.,-111.423085691599));
#61630=CARTESIAN_POINT('',(-2.29165909971822,93.,-112.475016001577));
#61631=CARTESIAN_POINT('',(-12.1728732777108,93.,-108.608453931927));
#61632=CARTESIAN_POINT('',(-1.85852429730951,93.,-115.32908810583));
#61633=CARTESIAN_POINT('',(-7.42839288587365,93.,-78.6273350382574));
#61634=CARTESIAN_POINT('',(-4.11365584262083,93.,-117.131229900105));
#61635=CARTESIAN_POINT('',(17.7244780890718,93.,-99.6797362392957));
#61636=CARTESIAN_POINT('',(-6.80192219034086,93.,-116.079299590128));
#61637=CARTESIAN_POINT('',(-13.9948700206135,93.,-113.264667830456));
#61638=CARTESIAN_POINT('',(-7.23505699274959,93.,-113.225227485875));
#61639=CARTESIAN_POINT('',(-12.3717907789052,93.,-79.3775465225557));
#61640=CARTESIAN_POINT('',(14.603076938943,93.,-95.7737338250652));
#61641=CARTESIAN_POINT('',(2.0043954003549,93.,-114.156080805953));
#61642=CARTESIAN_POINT('',(4.69266174807491,93.,-115.208011115931));
#61643=CARTESIAN_POINT('',(-12.1728732777109,93.,-108.608453931927));
#61644=CARTESIAN_POINT('',(5.12579655048363,93.,-118.062083220184));
#61645=CARTESIAN_POINT('',(-1.00673065130416,93.,-77.6527817328378));
#61646=CARTESIAN_POINT('',(2.8706650051723,93.,-119.864225014459));
#61647=CARTESIAN_POINT('',(21.779297126192,93.,-104.753782216246));
#61648=CARTESIAN_POINT('',(0.182398657452273,93.,-118.812294704482));
#61649=CARTESIAN_POINT('',(-13.9948700206135,93.,-113.264667830456));
#61650=CARTESIAN_POINT('',(-0.250736144956458,93.,-115.958222600229));
#61651=CARTESIAN_POINT('',(-5.95012854433579,93.,-78.4029932171361));
#61652=CARTESIAN_POINT('',(18.6578959760633,93.,-100.847779802016));
#61653=CARTESIAN_POINT('',(8.98871624814803,93.,-116.889075920307));
#61654=CARTESIAN_POINT('',(11.676982595868,93.,-117.941006230285));
#61655=CARTESIAN_POINT('',(-12.1728732777109,93.,-108.608453931927));
#61656=CARTESIAN_POINT('',(12.1101173982768,93.,-120.795078334538));
#61657=CARTESIAN_POINT('',(5.41493158326532,93.,-76.6782284274182));
#61658=CARTESIAN_POINT('',(9.85498585296543,93.,-122.597220128813));
#61659=CARTESIAN_POINT('',(25.8341161633123,93.,-109.827828193197));
#61660=CARTESIAN_POINT('',(7.1667195052454,93.,-121.545289818836));
#61661=CARTESIAN_POINT('',(-13.9948700206135,93.,-113.264667830456));
#61662=CARTESIAN_POINT('',(6.73358470283667,93.,-118.691217714583));
#61663=CARTESIAN_POINT('',(0.471533690233657,93.,-77.4284399117164));
#61664=CARTESIAN_POINT('',(22.7127150131835,93.,-105.921825778966));
#61665=CARTESIAN_POINT('',(15.9730370959412,93.,-119.622071034661));
#61666=CARTESIAN_POINT('',(18.6613034436612,93.,-120.674001344638));
#61667=CARTESIAN_POINT('',(-12.1728732777109,93.,-108.608453931927));
#61668=CARTESIAN_POINT('',(19.0944382460699,93.,-123.528073448892));
#61669=CARTESIAN_POINT('',(11.8365938178348,93.,-75.7036751219986));
#61670=CARTESIAN_POINT('',(16.8393067007586,93.,-125.330215243167));
#61671=CARTESIAN_POINT('',(29.8889352004325,93.,-114.901874170147));
#61672=CARTESIAN_POINT('',(14.1510403530385,93.,-124.27828493319));
#61673=CARTESIAN_POINT('',(-13.9948700206135,93.,-113.264667830456));
#61674=CARTESIAN_POINT('',(13.7179055506298,93.,-121.424212828937));
#61675=CARTESIAN_POINT('',(6.89319592480311,93.,-76.4538866062968));
#61676=CARTESIAN_POINT('',(26.7675340503038,93.,-110.995871755917));
#61677=CARTESIAN_POINT('',(22.9573579437343,93.,-122.355066149015));
#61678=CARTESIAN_POINT('',(25.6456242914543,93.,-123.406996458992));
#61679=CARTESIAN_POINT('',(-12.1728732777109,93.,-108.608453931927));
#61680=CARTESIAN_POINT('',(26.078759093863,93.,-126.261068563245));
#61681=CARTESIAN_POINT('',(18.2582560524043,93.,-74.729121816579));
#61682=CARTESIAN_POINT('',(23.8236275485517,93.,-128.063210357521));
#61683=CARTESIAN_POINT('',(33.9437542375528,93.,-119.975920147098));
#61684=CARTESIAN_POINT('',(21.1353612008317,93.,-127.011280047544));
#61685=CARTESIAN_POINT('',(-13.9948700206135,93.,-113.264667830456));
#61686=CARTESIAN_POINT('',(20.7022263984229,93.,-124.157207943291));
#61687=CARTESIAN_POINT('',(13.3148581593726,93.,-75.4793333008771));
#61688=CARTESIAN_POINT('',(30.822353087424,93.,-116.069917732867));
#61689=CARTESIAN_POINT('',(-48.0111677606444,93.,-87.6100181659289));
#61690=CARTESIAN_POINT('',(-45.3229014129244,93.,-88.6619484759063));
#61691=CARTESIAN_POINT('',(-9.80603008026161,93.,-102.559854649557));
#61692=CARTESIAN_POINT('',(-44.8897666105157,93.,-91.5160205801594));
#61693=CARTESIAN_POINT('',(-45.9583662932906,93.,-84.4746548707751));
#61694=CARTESIAN_POINT('',(-47.144898155827,93.,-93.3181623744351));
#61695=CARTESIAN_POINT('',(-10.65925517077,93.,-64.1614144006424));
#61696=CARTESIAN_POINT('',(-49.833164503547,93.,-92.2662320644577));
#61697=CARTESIAN_POINT('',(-11.6280268231643,93.,-107.216068548086));
#61698=CARTESIAN_POINT('',(-50.2662993059558,93.,-89.4121599602046));
#61699=CARTESIAN_POINT('',(-50.901764186322,93.,-85.2248663550737));
#61700=CARTESIAN_POINT('',(-13.7806563208988,93.,-60.2554119864119));
#61701=CARTESIAN_POINT('',(-41.0268469128513,93.,-90.3430132802828));
#61702=CARTESIAN_POINT('',(-38.3385805651313,93.,-91.3949435902602));
#61703=CARTESIAN_POINT('',(-9.80603008026162,93.,-102.559854649557));
#61704=CARTESIAN_POINT('',(-37.9054457627226,93.,-94.2490156945133));
#61705=CARTESIAN_POINT('',(-39.5367040587211,93.,-83.5001015653555));
#61706=CARTESIAN_POINT('',(-40.1605773080339,93.,-96.051157488789));
#61707=CARTESIAN_POINT('',(-6.60443613364971,93.,-69.2354603775928));
#61708=CARTESIAN_POINT('',(-42.8488436557539,93.,-94.9992271788116));
#61709=CARTESIAN_POINT('',(-11.6280268231643,93.,-107.216068548086));
#61710=CARTESIAN_POINT('',(-43.2819784581626,93.,-92.1451550745585));
#61711=CARTESIAN_POINT('',(-44.4801019517525,93.,-84.250313049654));
#61712=CARTESIAN_POINT('',(-9.7258372837785,93.,-65.3294579633623));
#61713=CARTESIAN_POINT('',(-34.0425260650581,93.,-93.0760083946367));
#61714=CARTESIAN_POINT('',(-31.3542597173381,93.,-94.1279387046141));
#61715=CARTESIAN_POINT('',(-9.80603008026162,93.,-102.559854649557));
#61716=CARTESIAN_POINT('',(-30.9211249149294,93.,-96.9820108088672));
#61717=CARTESIAN_POINT('',(-33.1150418241517,93.,-82.5255482599359));
#61718=CARTESIAN_POINT('',(-33.1762564602408,93.,-98.7841526031429));
#61719=CARTESIAN_POINT('',(-2.54961709652947,93.,-74.3095063545433));
#61720=CARTESIAN_POINT('',(-35.8645228079608,93.,-97.7322222931655));
#61721=CARTESIAN_POINT('',(-11.6280268231643,93.,-107.216068548086));
#61722=CARTESIAN_POINT('',(-36.2976576103695,93.,-94.8781501889124));
#61723=CARTESIAN_POINT('',(-38.0584397171831,93.,-83.2757597442344));
#61724=CARTESIAN_POINT('',(-5.67101824665825,93.,-70.4035039403128));
#61725=CARTESIAN_POINT('',(-27.058205217265,93.,-95.8090035089906));
#61726=CARTESIAN_POINT('',(-24.369938869545,93.,-96.860933818968));
#61727=CARTESIAN_POINT('',(-9.80603008026163,93.,-102.559854649557));
#61728=CARTESIAN_POINT('',(-23.9368040671363,93.,-99.7150059232211));
#61729=CARTESIAN_POINT('',(-26.6933795895822,93.,-81.5509949545163));
#61730=CARTESIAN_POINT('',(-26.1919356124476,93.,-101.517147717497));
#61731=CARTESIAN_POINT('',(1.50520194059078,93.,-79.3835523314938));
#61732=CARTESIAN_POINT('',(-28.8802019601676,93.,-100.465217407519));
#61733=CARTESIAN_POINT('',(-11.6280268231643,93.,-107.216068548086));
#61734=CARTESIAN_POINT('',(-29.3133367625764,93.,-97.6111453032663));
#61735=CARTESIAN_POINT('',(-31.6367774826136,93.,-82.3012064388147));
#61736=CARTESIAN_POINT('',(-1.616199209538,93.,-75.4775499172633));
#61737=CARTESIAN_POINT('',(-20.0738843694719,93.,-98.5419986233445));
#61738=CARTESIAN_POINT('',(-17.3856180217519,93.,-99.5939289333219));
#61739=CARTESIAN_POINT('',(-9.80603008026163,93.,-102.559854649557));
#61740=CARTESIAN_POINT('',(-16.9524832193432,93.,-102.448001037575));
#61741=CARTESIAN_POINT('',(-20.2717173550127,93.,-80.5764416490967));
#61742=CARTESIAN_POINT('',(-19.2076147646545,93.,-104.250142831851));
#61743=CARTESIAN_POINT('',(5.56002097771102,93.,-84.4575983084442));
#61744=CARTESIAN_POINT('',(-21.8958811123745,93.,-103.198212521873));
#61745=CARTESIAN_POINT('',(-11.6280268231643,93.,-107.216068548086));
#61746=CARTESIAN_POINT('',(-22.3290159147832,93.,-100.34414041762));
#61747=CARTESIAN_POINT('',(-25.2151152480442,93.,-81.326653133395));
#61748=CARTESIAN_POINT('',(2.43861982758225,93.,-80.5515958942137));
#61749=CARTESIAN_POINT('',(-13.0895635216788,93.,-101.274993737698));
#61750=CARTESIAN_POINT('',(-10.4012971739587,93.,-102.326924047676));
#61751=CARTESIAN_POINT('',(-9.80603008026164,93.,-102.559854649557));
#61752=CARTESIAN_POINT('',(-9.96816237155003,93.,-105.180996151929));
#61753=CARTESIAN_POINT('',(-13.8500551204432,93.,-79.601888343677));
#61754=CARTESIAN_POINT('',(-12.2232939168614,93.,-106.983137946205));
#61755=CARTESIAN_POINT('',(9.61484001483127,93.,-89.5316442853947));
#61756=CARTESIAN_POINT('',(-14.9115602645814,93.,-105.931207636227));
#61757=CARTESIAN_POINT('',(-11.6280268231643,93.,-107.216068548086));
#61758=CARTESIAN_POINT('',(-15.3446950669901,93.,-103.077135531974));
#61759=CARTESIAN_POINT('',(-18.7934530134747,93.,-80.3520998279754));
#61760=CARTESIAN_POINT('',(6.4934388647025,93.,-85.6256418711642));
#61761=CARTESIAN_POINT('',(-6.10524267388563,93.,-104.007988852052));
#61762=CARTESIAN_POINT('',(-3.41697632616561,93.,-105.05991916203));
#61763=CARTESIAN_POINT('',(-9.80603008026164,93.,-102.559854649557));
#61764=CARTESIAN_POINT('',(-2.9838415237569,93.,-107.913991266283));
#61765=CARTESIAN_POINT('',(-7.42839288587373,93.,-78.6273350382574));
#61766=CARTESIAN_POINT('',(-5.23897306906822,93.,-109.716133060558));
#61767=CARTESIAN_POINT('',(13.6696590519515,93.,-94.6056902623452));
#61768=CARTESIAN_POINT('',(-7.92723941678825,93.,-108.664202750581));
#61769=CARTESIAN_POINT('',(-11.6280268231643,93.,-107.216068548086));
#61770=CARTESIAN_POINT('',(-8.36037421919698,93.,-105.810130646328));
#61771=CARTESIAN_POINT('',(-12.3717907789053,93.,-79.3775465225557));
#61772=CARTESIAN_POINT('',(10.5482579018228,93.,-90.6996878481147));
#61773=CARTESIAN_POINT('',(0.879078173907508,93.,-106.740983966406));
#61774=CARTESIAN_POINT('',(3.56734452162752,93.,-107.792914276384));
#61775=CARTESIAN_POINT('',(-9.80603008026165,93.,-102.559854649557));
#61776=CARTESIAN_POINT('',(4.00047932403624,93.,-110.646986380637));
#61777=CARTESIAN_POINT('',(-1.00673065130425,93.,-77.6527817328378));
#61778=CARTESIAN_POINT('',(1.74534777872491,93.,-112.449128174912));
#61779=CARTESIAN_POINT('',(17.7244780890718,93.,-99.6797362392957));
#61780=CARTESIAN_POINT('',(-0.942918568995116,93.,-111.397197864935));
#61781=CARTESIAN_POINT('',(-11.6280268231643,93.,-107.216068548086));
#61782=CARTESIAN_POINT('',(-1.37605337140385,93.,-108.543125760682));
#61783=CARTESIAN_POINT('',(-5.95012854433583,93.,-78.4029932171361));
#61784=CARTESIAN_POINT('',(14.603076938943,93.,-95.7737338250652));
#61785=CARTESIAN_POINT('',(-23.6822535379229,93.,-118.054294027632));
#61786=CARTESIAN_POINT('',(-20.9939871902029,93.,-119.106224337609));
#61787=CARTESIAN_POINT('',(-16.9065596726093,93.,-120.705652496668));
#61788=CARTESIAN_POINT('',(-20.5608523877941,93.,-121.960296441862));
#61789=CARTESIAN_POINT('',(-26.693379589582,93.,-81.5509949545162));
#61790=CARTESIAN_POINT('',(-22.8159839331055,93.,-123.762438236138));
#61791=CARTESIAN_POINT('',(13.6696590519515,93.,-94.6056902623452));
#61792=CARTESIAN_POINT('',(-25.5042502808255,93.,-122.710507926161));
#61793=CARTESIAN_POINT('',(-18.728556415512,93.,-125.361866395196));
#61794=CARTESIAN_POINT('',(-25.9373850832342,93.,-119.856435821907));
#61795=CARTESIAN_POINT('',(-31.6367774826136,93.,-82.3012064388147));
#61796=CARTESIAN_POINT('',(10.5482579018228,93.,-90.6996878481147));
#61797=CARTESIAN_POINT('',(-16.6979326901297,93.,-120.787289141986));
#61798=CARTESIAN_POINT('',(-14.0096663424097,93.,-121.839219451963));
#61799=CARTESIAN_POINT('',(-16.9065596726093,93.,-120.705652496668));
#61800=CARTESIAN_POINT('',(-13.576531540001,93.,-124.693291556216));
#61801=CARTESIAN_POINT('',(-20.2717173550125,93.,-80.5764416490966));
#61802=CARTESIAN_POINT('',(-15.8316630853124,93.,-126.495433350492));
#61803=CARTESIAN_POINT('',(17.7244780890718,93.,-99.6797362392957));
#61804=CARTESIAN_POINT('',(-18.5199294330324,93.,-125.443503040514));
#61805=CARTESIAN_POINT('',(-18.728556415512,93.,-125.361866395196));
#61806=CARTESIAN_POINT('',(-18.9530642354411,93.,-122.589430936261));
#61807=CARTESIAN_POINT('',(-25.2151152480441,93.,-81.326653133395));
#61808=CARTESIAN_POINT('',(14.603076938943,93.,-95.7737338250652));
#61809=CARTESIAN_POINT('',(-9.71361184233662,93.,-123.52028425634));
#61810=CARTESIAN_POINT('',(-7.02534549461661,93.,-124.572214566317));
#61811=CARTESIAN_POINT('',(-16.9065596726093,93.,-120.705652496668));
#61812=CARTESIAN_POINT('',(-6.59221069220789,93.,-127.42628667057));
#61813=CARTESIAN_POINT('',(-13.850055120443,93.,-79.601888343677));
#61814=CARTESIAN_POINT('',(-8.84734223751921,93.,-129.228428464846));
#61815=CARTESIAN_POINT('',(21.779297126192,93.,-104.753782216246));
#61816=CARTESIAN_POINT('',(-11.5356085852392,93.,-128.176498154868));
#61817=CARTESIAN_POINT('',(-18.728556415512,93.,-125.361866395196));
#61818=CARTESIAN_POINT('',(-11.968743387648,93.,-125.322426050615));
#61819=CARTESIAN_POINT('',(-18.7934530134747,93.,-80.3520998279754));
#61820=CARTESIAN_POINT('',(18.6578959760633,93.,-100.847779802016));
#61821=CARTESIAN_POINT('',(-2.72929099454348,93.,-126.253279370693));
#61822=CARTESIAN_POINT('',(-0.0410246468234739,93.,-127.305209680671));
#61823=CARTESIAN_POINT('',(-16.9065596726093,93.,-120.705652496668));
#61824=CARTESIAN_POINT('',(0.392110155585244,93.,-130.159281784924));
#61825=CARTESIAN_POINT('',(-7.42839288587351,93.,-78.6273350382574));
#61826=CARTESIAN_POINT('',(-1.86302138972608,93.,-131.9614235792));
#61827=CARTESIAN_POINT('',(25.8341161633123,93.,-109.827828193197));
#61828=CARTESIAN_POINT('',(-4.55128773744611,93.,-130.909493269222));
#61829=CARTESIAN_POINT('',(-18.728556415512,93.,-125.361866395196));
#61830=CARTESIAN_POINT('',(-4.98442253985484,93.,-128.055421164969));
#61831=CARTESIAN_POINT('',(-12.3717907789052,93.,-79.3775465225557));
#61832=CARTESIAN_POINT('',(22.7127150131835,93.,-105.921825778966));
#61833=CARTESIAN_POINT('',(-45.7605333077496,93.,-102.440211845023));
#61834=CARTESIAN_POINT('',(-43.0722669600296,93.,-103.492142155));
#61835=CARTESIAN_POINT('',(-14.53971647516,93.,-114.657053214297));
#61836=CARTESIAN_POINT('',(-42.6391321576209,93.,-106.346214259254));
#61837=CARTESIAN_POINT('',(-45.9583662932905,93.,-84.4746548707751));
#61838=CARTESIAN_POINT('',(-44.8942637029322,93.,-108.148356053529));
#61839=CARTESIAN_POINT('',(-2.54961709652946,93.,-74.3095063545433));
#61840=CARTESIAN_POINT('',(-47.5825300506523,93.,-107.096425743552));
#61841=CARTESIAN_POINT('',(-16.3617132180627,93.,-119.313267112826));
#61842=CARTESIAN_POINT('',(-48.015664853061,93.,-104.242353639299));
#61843=CARTESIAN_POINT('',(-50.9017641863219,93.,-85.2248663550736));
#61844=CARTESIAN_POINT('',(-5.67101824665825,93.,-70.4035039403128));
#61845=CARTESIAN_POINT('',(-38.7762124599565,93.,-105.173206959377));
#61846=CARTESIAN_POINT('',(-36.0879461122365,93.,-106.225137269354));
#61847=CARTESIAN_POINT('',(-14.53971647516,93.,-114.657053214297));
#61848=CARTESIAN_POINT('',(-35.6548113098278,93.,-109.079209373607));
#61849=CARTESIAN_POINT('',(-39.536704058721,93.,-83.5001015653555));
#61850=CARTESIAN_POINT('',(-37.9099428551391,93.,-110.881351167883));
#61851=CARTESIAN_POINT('',(1.50520194059079,93.,-79.3835523314938));
#61852=CARTESIAN_POINT('',(-40.5982092028591,93.,-109.829420857906));
#61853=CARTESIAN_POINT('',(-16.3617132180627,93.,-119.313267112826));
#61854=CARTESIAN_POINT('',(-41.0313440052679,93.,-106.975348753653));
#61855=CARTESIAN_POINT('',(-44.4801019517525,93.,-84.250313049654));
#61856=CARTESIAN_POINT('',(-1.616199209538,93.,-75.4775499172633));
#61857=CARTESIAN_POINT('',(-31.7918916121634,93.,-107.906202073731));
#61858=CARTESIAN_POINT('',(-29.1036252644434,93.,-108.958132383708));
#61859=CARTESIAN_POINT('',(-14.53971647516,93.,-114.657053214297));
#61860=CARTESIAN_POINT('',(-28.6704904620347,93.,-111.812204487961));
#61861=CARTESIAN_POINT('',(-33.1150418241515,93.,-82.5255482599358));
#61862=CARTESIAN_POINT('',(-30.925622007346,93.,-113.614346282237));
#61863=CARTESIAN_POINT('',(5.56002097771103,93.,-84.4575983084443));
#61864=CARTESIAN_POINT('',(-33.613888355066,93.,-112.56241597226));
#61865=CARTESIAN_POINT('',(-16.3617132180627,93.,-119.313267112826));
#61866=CARTESIAN_POINT('',(-34.0470231574747,93.,-109.708343868006));
#61867=CARTESIAN_POINT('',(-38.058439717183,93.,-83.2757597442344));
#61868=CARTESIAN_POINT('',(2.43861982758225,93.,-80.5515958942138));
#61869=CARTESIAN_POINT('',(-24.8075707643703,93.,-110.639197188085));
#61870=CARTESIAN_POINT('',(-22.1193044166502,93.,-111.691127498062));
#61871=CARTESIAN_POINT('',(-14.53971647516,93.,-114.657053214297));
#61872=CARTESIAN_POINT('',(-21.6861696142415,93.,-114.545199602315));
#61873=CARTESIAN_POINT('',(-26.693379589582,93.,-81.5509949545162));
#61874=CARTESIAN_POINT('',(-23.9413011595529,93.,-116.347341396591));
#61875=CARTESIAN_POINT('',(9.61484001483128,93.,-89.5316442853947));
#61876=CARTESIAN_POINT('',(-26.6295675072729,93.,-115.295411086613));
#61877=CARTESIAN_POINT('',(-16.3617132180627,93.,-119.313267112826));
#61878=CARTESIAN_POINT('',(-27.0627023096816,93.,-112.44133898236));
#61879=CARTESIAN_POINT('',(-31.6367774826136,93.,-82.3012064388147));
#61880=CARTESIAN_POINT('',(6.4934388647025,93.,-85.6256418711642));
#61881=CARTESIAN_POINT('',(10.1140334745954,93.,-124.304172759854));
#61882=CARTESIAN_POINT('',(12.8022998223154,93.,-125.356103069832));
#61883=CARTESIAN_POINT('',(-14.5397164751601,93.,-114.657053214298));
#61884=CARTESIAN_POINT('',(13.2354346247241,93.,-128.210175174085));
#61885=CARTESIAN_POINT('',(5.41493158326539,93.,-76.6782284274182));
#61886=CARTESIAN_POINT('',(10.9803030794128,93.,-130.01231696836));
#61887=CARTESIAN_POINT('',(29.8889352004325,93.,-114.901874170147));
#61888=CARTESIAN_POINT('',(8.29203673169278,93.,-128.960386658383));
#61889=CARTESIAN_POINT('',(-16.3617132180627,93.,-119.313267112826));
#61890=CARTESIAN_POINT('',(7.85890192928405,93.,-126.10631455413));
#61891=CARTESIAN_POINT('',(0.47153369023368,93.,-77.4284399117164));
#61892=CARTESIAN_POINT('',(26.7675340503038,93.,-110.995871755917));
#61893=CARTESIAN_POINT('',(-46.885850534197,93.,-95.025115005476));
#61894=CARTESIAN_POINT('',(-44.197584186477,93.,-96.0770453154534));
#61895=CARTESIAN_POINT('',(-12.1728732777108,93.,-108.608453931927));
#61896=CARTESIAN_POINT('',(-43.7644493840683,93.,-98.9311174197065));
#61897=CARTESIAN_POINT('',(-45.9583662932906,93.,-84.4746548707751));
#61898=CARTESIAN_POINT('',(-46.0195809293796,93.,-100.733259213982));
#61899=CARTESIAN_POINT('',(-6.6044361336497,93.,-69.2354603775928));
#61900=CARTESIAN_POINT('',(-48.7078472770996,93.,-99.6813289040047));
#61901=CARTESIAN_POINT('',(-13.9948700206135,93.,-113.264667830456));
#61902=CARTESIAN_POINT('',(-49.1409820795084,93.,-96.8272567997517));
#61903=CARTESIAN_POINT('',(-50.901764186322,93.,-85.2248663550736));
#61904=CARTESIAN_POINT('',(-9.7258372837785,93.,-65.3294579633623));
#61905=CARTESIAN_POINT('',(-39.9015296864039,93.,-97.7581101198299));
#61906=CARTESIAN_POINT('',(-37.2132633386839,93.,-98.8100404298073));
#61907=CARTESIAN_POINT('',(-12.1728732777108,93.,-108.608453931927));
#61908=CARTESIAN_POINT('',(-36.7801285362752,93.,-101.66411253406));
#61909=CARTESIAN_POINT('',(-39.5367040587211,93.,-83.5001015653555));
#61910=CARTESIAN_POINT('',(-39.0352600815865,93.,-103.466254328336));
#61911=CARTESIAN_POINT('',(-2.54961709652946,93.,-74.3095063545433));
#61912=CARTESIAN_POINT('',(-41.7235264293065,93.,-102.414324018359));
#61913=CARTESIAN_POINT('',(-13.9948700206135,93.,-113.264667830456));
#61914=CARTESIAN_POINT('',(-42.1566612317152,93.,-99.5602519141056));
#61915=CARTESIAN_POINT('',(-44.4801019517525,93.,-84.250313049654));
#61916=CARTESIAN_POINT('',(-5.67101824665825,93.,-70.4035039403128));
#61917=CARTESIAN_POINT('',(-32.9172088386108,93.,-100.491105234184));
#61918=CARTESIAN_POINT('',(-30.2289424908907,93.,-101.543035544161));
#61919=CARTESIAN_POINT('',(-12.1728732777108,93.,-108.608453931927));
#61920=CARTESIAN_POINT('',(-29.795807688482,93.,-104.397107648414));
#61921=CARTESIAN_POINT('',(-33.1150418241516,93.,-82.5255482599359));
#61922=CARTESIAN_POINT('',(-32.0509392337934,93.,-106.19924944269));
#61923=CARTESIAN_POINT('',(1.50520194059079,93.,-79.3835523314938));
#61924=CARTESIAN_POINT('',(-34.7392055815134,93.,-105.147319132713));
#61925=CARTESIAN_POINT('',(-13.9948700206135,93.,-113.264667830456));
#61926=CARTESIAN_POINT('',(-35.1723403839221,93.,-102.293247028459));
#61927=CARTESIAN_POINT('',(-38.058439717183,93.,-83.2757597442344));
#61928=CARTESIAN_POINT('',(-1.616199209538,93.,-75.4775499172633));
#61929=CARTESIAN_POINT('',(3.12971262680227,93.,-121.5711776455));
#61930=CARTESIAN_POINT('',(5.81797897452228,93.,-122.623107955478));
#61931=CARTESIAN_POINT('',(-14.5397164751601,93.,-114.657053214297));
#61932=CARTESIAN_POINT('',(6.251113776931,93.,-125.477180059731));
#61933=CARTESIAN_POINT('',(-1.00673065130409,93.,-77.6527817328378));
#61934=CARTESIAN_POINT('',(3.99598223161968,93.,-127.279321854006));
#61935=CARTESIAN_POINT('',(25.8341161633122,93.,-109.827828193197));
#61936=CARTESIAN_POINT('',(1.30771588389965,93.,-126.227391544029));
#61937=CARTESIAN_POINT('',(-16.3617132180627,93.,-119.313267112826));
#61938=CARTESIAN_POINT('',(0.874581081490917,93.,-123.373319439776));
#61939=CARTESIAN_POINT('',(-5.95012854433577,93.,-78.4029932171361));
#61940=CARTESIAN_POINT('',(22.7127150131835,93.,-105.921825778966));
#61941=CARTESIAN_POINT('',(-3.85460822099086,93.,-118.838182531146));
#61942=CARTESIAN_POINT('',(-1.16634187327085,93.,-119.890112841124));
#61943=CARTESIAN_POINT('',(-14.5397164751601,93.,-114.657053214298));
#61944=CARTESIAN_POINT('',(-0.733207070862132,93.,-122.744184945377));
#61945=CARTESIAN_POINT('',(-7.42839288587358,93.,-78.6273350382574));
#61946=CARTESIAN_POINT('',(-2.98833861617346,93.,-124.546326739653));
#61947=CARTESIAN_POINT('',(21.779297126192,93.,-104.753782216246));
#61948=CARTESIAN_POINT('',(-5.67660496389348,93.,-123.494396429675));
#61949=CARTESIAN_POINT('',(-16.3617132180627,93.,-119.313267112826));
#61950=CARTESIAN_POINT('',(-6.10973976630222,93.,-120.640324325422));
#61951=CARTESIAN_POINT('',(-12.3717907789052,93.,-79.3775465225557));
#61952=CARTESIAN_POINT('',(18.6578959760633,93.,-100.847779802016));
#61953=CARTESIAN_POINT('',(-10.838929068784,93.,-116.105187416792));
#61954=CARTESIAN_POINT('',(-8.15066272106398,93.,-117.15711772677));
#61955=CARTESIAN_POINT('',(-14.5397164751601,93.,-114.657053214297));
#61956=CARTESIAN_POINT('',(-7.71752791865526,93.,-120.011189831023));
#61957=CARTESIAN_POINT('',(-13.8500551204431,93.,-79.601888343677));
#61958=CARTESIAN_POINT('',(-9.97265946396659,93.,-121.813331625299));
#61959=CARTESIAN_POINT('',(17.7244780890718,93.,-99.6797362392957));
#61960=CARTESIAN_POINT('',(-12.6609258116866,93.,-120.761401315321));
#61961=CARTESIAN_POINT('',(-16.3617132180627,93.,-119.313267112826));
#61962=CARTESIAN_POINT('',(-13.0940606140953,93.,-117.907329211068));
#61963=CARTESIAN_POINT('',(-18.7934530134747,93.,-80.3520998279754));
#61964=CARTESIAN_POINT('',(14.603076938943,93.,-95.7737338250652));
#61965=CARTESIAN_POINT('',(-17.8232499165771,93.,-113.372192302439));
#61966=CARTESIAN_POINT('',(-15.1349835688571,93.,-114.424122612416));
#61967=CARTESIAN_POINT('',(-14.53971647516,93.,-114.657053214297));
#61968=CARTESIAN_POINT('',(-14.7018487664484,93.,-117.278194716669));
#61969=CARTESIAN_POINT('',(-20.2717173550125,93.,-80.5764416490966));
#61970=CARTESIAN_POINT('',(-16.9569803117597,93.,-119.080336510945));
#61971=CARTESIAN_POINT('',(13.6696590519515,93.,-94.6056902623452));
#61972=CARTESIAN_POINT('',(-19.6452466594797,93.,-118.028406200967));
#61973=CARTESIAN_POINT('',(-16.3617132180627,93.,-119.313267112826));
#61974=CARTESIAN_POINT('',(-20.0783814618885,93.,-115.174334096714));
#61975=CARTESIAN_POINT('',(-25.2151152480441,93.,-81.326653133395));
#61976=CARTESIAN_POINT('',(10.5482579018228,93.,-90.6996878481147));
#61977=CARTESIAN_POINT('',(-8.35587712678037,93.,-89.1777951729581));
#61978=CARTESIAN_POINT('',(-5.66761077906036,93.,-90.2297254829355));
#61979=CARTESIAN_POINT('',(-5.07234368536322,93.,-90.462656084817));
#61980=CARTESIAN_POINT('',(-5.23447597665164,93.,-93.0837975871887));
#61981=CARTESIAN_POINT('',(-7.42839288587387,93.,-78.6273350382574));
#61982=CARTESIAN_POINT('',(-7.48960752196297,93.,-94.8859393814643));
#61983=CARTESIAN_POINT('',(5.56002097771101,93.,-84.4575983084442));
#61984=CARTESIAN_POINT('',(-10.177873869683,93.,-93.8340090714869));
#61985=CARTESIAN_POINT('',(-6.89434042826585,93.,-95.1188699833458));
#61986=CARTESIAN_POINT('',(-10.6110086720917,93.,-90.9799369672338));
#61987=CARTESIAN_POINT('',(-12.3717907789053,93.,-79.3775465225557));
#61988=CARTESIAN_POINT('',(2.43861982758225,93.,-80.5515958942137));
#61989=CARTESIAN_POINT('',(-15.3401979745735,93.,-86.4448000586042));
#61990=CARTESIAN_POINT('',(-12.6519316268535,93.,-87.4967303685817));
#61991=CARTESIAN_POINT('',(-5.07234368536321,93.,-90.462656084817));
#61992=CARTESIAN_POINT('',(-12.2187968244448,93.,-90.3508024728348));
#61993=CARTESIAN_POINT('',(-13.8500551204434,93.,-79.6018883436771));
#61994=CARTESIAN_POINT('',(-14.4739283697561,93.,-92.1529442671104));
#61995=CARTESIAN_POINT('',(1.50520194059077,93.,-79.3835523314938));
#61996=CARTESIAN_POINT('',(-17.1621947174761,93.,-91.101013957133));
#61997=CARTESIAN_POINT('',(-6.89434042826585,93.,-95.1188699833458));
#61998=CARTESIAN_POINT('',(-17.5953295198849,93.,-88.2469418528799));
#61999=CARTESIAN_POINT('',(-18.7934530134748,93.,-80.3520998279754));
#62000=CARTESIAN_POINT('',(-1.616199209538,93.,-75.4775499172633));
#62001=CARTESIAN_POINT('',(-22.3245188223666,93.,-83.7118049442504));
#62002=CARTESIAN_POINT('',(-19.6362524746466,93.,-84.7637352542278));
#62003=CARTESIAN_POINT('',(-5.07234368536321,93.,-90.462656084817));
#62004=CARTESIAN_POINT('',(-19.2031176722379,93.,-87.6178073584809));
#62005=CARTESIAN_POINT('',(-20.2717173550128,93.,-80.5764416490967));
#62006=CARTESIAN_POINT('',(-21.4582492175492,93.,-89.4199491527566));
#62007=CARTESIAN_POINT('',(-2.54961709652948,93.,-74.3095063545433));
#62008=CARTESIAN_POINT('',(-24.1465155652693,93.,-88.3680188427791));
#62009=CARTESIAN_POINT('',(-6.89434042826585,93.,-95.1188699833458));
#62010=CARTESIAN_POINT('',(-24.579650367678,93.,-85.5139467385261));
#62011=CARTESIAN_POINT('',(-25.2151152480442,93.,-81.326653133395));
#62012=CARTESIAN_POINT('',(-5.67101824665826,93.,-70.4035039403128));
#62013=CARTESIAN_POINT('',(-29.3088396701598,93.,-80.9788098298965));
#62014=CARTESIAN_POINT('',(-26.6205733224398,93.,-82.0307401398739));
#62015=CARTESIAN_POINT('',(-5.0723436853632,93.,-90.462656084817));
#62016=CARTESIAN_POINT('',(-26.187438520031,93.,-84.884812244127));
#62017=CARTESIAN_POINT('',(-26.6933795895823,93.,-81.5509949545163));
#62018=CARTESIAN_POINT('',(-28.4425700653424,93.,-86.6869540384027));
#62019=CARTESIAN_POINT('',(-6.60443613364972,93.,-69.2354603775928));
#62020=CARTESIAN_POINT('',(-31.1308364130624,93.,-85.6350237284252));
#62021=CARTESIAN_POINT('',(-6.89434042826586,93.,-95.1188699833458));
#62022=CARTESIAN_POINT('',(-31.5639712154711,93.,-82.7809516241722));
#62023=CARTESIAN_POINT('',(-31.6367774826137,93.,-82.3012064388147));
#62024=CARTESIAN_POINT('',(-9.72583728377851,93.,-65.3294579633623));
#62025=CARTESIAN_POINT('',(34.6753651864258,93.,-112.990862698629));
#62026=CARTESIAN_POINT('',(37.3636315341458,93.,-114.042793008606));
#62027=CARTESIAN_POINT('',(-7.43918688281246,93.,-96.5112553671872));
#62028=CARTESIAN_POINT('',(37.7967663365545,93.,-116.896865112859));
#62029=CARTESIAN_POINT('',(31.1015805215431,93.,-72.7800152057397));
#62030=CARTESIAN_POINT('',(35.5416347912432,93.,-118.699006907135));
#62031=CARTESIAN_POINT('',(33.9437542375527,93.,-119.975920147098));
#62032=CARTESIAN_POINT('',(32.8533684435232,93.,-117.647076597157));
#62033=CARTESIAN_POINT('',(-9.26118362571507,93.,-101.167469265716));
#62034=CARTESIAN_POINT('',(32.4202336411144,93.,-114.793004492904));
#62035=CARTESIAN_POINT('',(26.1581826285114,93.,-73.5302266900378));
#62036=CARTESIAN_POINT('',(30.822353087424,93.,-116.069917732867));
#62037=CARTESIAN_POINT('',(-50.2618022135392,93.,-72.7798244868348));
#62038=CARTESIAN_POINT('',(-47.5735358658191,93.,-73.8317547968122));
#62039=CARTESIAN_POINT('',(-5.07234368536319,93.,-90.462656084817));
#62040=CARTESIAN_POINT('',(-47.1404010634104,93.,-76.6858269010653));
#62041=CARTESIAN_POINT('',(-45.9583662932908,93.,-84.4746548707751));
#62042=CARTESIAN_POINT('',(-49.3955326087217,93.,-78.487968695341));
#62043=CARTESIAN_POINT('',(-18.7688932450105,93.,-54.0133224467414));
#62044=CARTESIAN_POINT('',(-52.0837989564418,93.,-77.4360383853636));
#62045=CARTESIAN_POINT('',(-6.89434042826586,93.,-95.1188699833458));
#62046=CARTESIAN_POINT('',(-52.5169337588505,93.,-74.5819662811105));
#62047=CARTESIAN_POINT('',(-50.901764186322,93.,-85.2248663550737));
#62048=CARTESIAN_POINT('',(-21.8902943951393,93.,-50.1073200325109));
#62049=CARTESIAN_POINT('',(-43.277481365746,93.,-75.5128196011887));
#62050=CARTESIAN_POINT('',(-40.589215018026,93.,-76.5647499111661));
#62051=CARTESIAN_POINT('',(-5.07234368536319,93.,-90.462656084817));
#62052=CARTESIAN_POINT('',(-40.1560802156173,93.,-79.4188220154192));
#62053=CARTESIAN_POINT('',(-39.5367040587213,93.,-83.5001015653555));
#62054=CARTESIAN_POINT('',(-42.4112117609286,93.,-81.2209638096949));
#62055=CARTESIAN_POINT('',(-14.7140742078902,93.,-59.0873684236919));
#62056=CARTESIAN_POINT('',(-45.0994781086486,93.,-80.1690334997174));
#62057=CARTESIAN_POINT('',(-6.89434042826586,93.,-95.1188699833458));
#62058=CARTESIAN_POINT('',(-45.5326129110574,93.,-77.3149613954644));
#62059=CARTESIAN_POINT('',(-44.4801019517526,93.,-84.250313049654));
#62060=CARTESIAN_POINT('',(-17.835475358019,93.,-55.1813660094614));
#62061=CARTESIAN_POINT('',(-36.2931605179529,93.,-78.2458147155426));
#62062=CARTESIAN_POINT('',(-33.6048941702329,93.,-79.29774502552));
#62063=CARTESIAN_POINT('',(-5.0723436853632,93.,-90.462656084817));
#62064=CARTESIAN_POINT('',(-33.1717593678242,93.,-82.1518171297731));
#62065=CARTESIAN_POINT('',(-33.1150418241518,93.,-82.5255482599359));
#62066=CARTESIAN_POINT('',(-35.4268909131355,93.,-83.9539589240488));
#62067=CARTESIAN_POINT('',(-10.65925517077,93.,-64.1614144006423));
#62068=CARTESIAN_POINT('',(-38.1151572608555,93.,-82.9020286140714));
#62069=CARTESIAN_POINT('',(-6.89434042826586,93.,-95.1188699833458));
#62070=CARTESIAN_POINT('',(-38.5482920632642,93.,-80.0479565098183));
#62071=CARTESIAN_POINT('',(-38.0584397171831,93.,-83.2757597442344));
#62072=CARTESIAN_POINT('',(-13.7806563208988,93.,-60.2554119864119));
#62073=CARTESIAN_POINT('',(26.5657271121853,93.,-102.842770744728));
#62074=CARTESIAN_POINT('',(29.2539934599053,93.,-103.894701054705));
#62075=CARTESIAN_POINT('',(-5.07234368536324,93.,-90.4626560848171));
#62076=CARTESIAN_POINT('',(29.687128262314,93.,-106.748773158958));
#62077=CARTESIAN_POINT('',(24.6799182869735,93.,-73.7545685111594));
#62078=CARTESIAN_POINT('',(27.4319967170027,93.,-108.550914953234));
#62079=CARTESIAN_POINT('',(25.8341161633122,93.,-109.827828193197));
#62080=CARTESIAN_POINT('',(24.7437303692827,93.,-107.498984643256));
#62081=CARTESIAN_POINT('',(-6.89434042826585,93.,-95.1188699833458));
#62082=CARTESIAN_POINT('',(24.3105955668739,93.,-104.644912539003));
#62083=CARTESIAN_POINT('',(19.7365203939419,93.,-74.5047799954575));
#62084=CARTESIAN_POINT('',(22.7127150131835,93.,-105.921825778966));
#62085=CARTESIAN_POINT('',(33.5500479599784,93.,-105.575765859081));
#62086=CARTESIAN_POINT('',(36.2383143076984,93.,-106.627696169059));
#62087=CARTESIAN_POINT('',(-5.07234368536325,93.,-90.4626560848171));
#62088=CARTESIAN_POINT('',(36.6714491101071,93.,-109.481768273312));
#62089=CARTESIAN_POINT('',(31.101580521543,93.,-72.7800152057397));
#62090=CARTESIAN_POINT('',(34.4163175647958,93.,-111.283910067588));
#62091=CARTESIAN_POINT('',(29.8889352004325,93.,-114.901874170147));
#62092=CARTESIAN_POINT('',(31.7280512170758,93.,-110.23197975761));
#62093=CARTESIAN_POINT('',(-6.89434042826585,93.,-95.1188699833458));
#62094=CARTESIAN_POINT('',(31.2949164146671,93.,-107.377907653357));
#62095=CARTESIAN_POINT('',(26.1581826285114,93.,-73.5302266900378));
#62096=CARTESIAN_POINT('',(26.7675340503038,93.,-110.995871755917));
#62097=CARTESIAN_POINT('',(40.5343688077715,93.,-108.308760973435));
#62098=CARTESIAN_POINT('',(43.2226351554916,93.,-109.360691283413));
#62099=CARTESIAN_POINT('',(-5.07234368536325,93.,-90.4626560848171));
#62100=CARTESIAN_POINT('',(43.6557699579003,93.,-112.214763387666));
#62101=CARTESIAN_POINT('',(37.5232427561125,93.,-71.8054619003202));
#62102=CARTESIAN_POINT('',(41.4006384125889,93.,-114.016905181942));
#62103=CARTESIAN_POINT('',(33.9437542375527,93.,-119.975920147098));
#62104=CARTESIAN_POINT('',(38.7123720648689,93.,-112.964974871964));
#62105=CARTESIAN_POINT('',(-6.89434042826584,93.,-95.1188699833458));
#62106=CARTESIAN_POINT('',(38.2792372624602,93.,-110.110902767711));
#62107=CARTESIAN_POINT('',(32.5798448630808,93.,-72.5556733846182));
#62108=CARTESIAN_POINT('',(30.822353087424,93.,-116.069917732867));
#62109=CARTESIAN_POINT('',(-51.3871194399865,93.,-65.3647276472878));
#62110=CARTESIAN_POINT('',(-48.6988530922665,93.,-66.4166579572652));
#62111=CARTESIAN_POINT('',(-2.70550048791398,93.,-84.4140568024469));
#62112=CARTESIAN_POINT('',(-48.2657182898578,93.,-69.2707300615183));
#62113=CARTESIAN_POINT('',(-45.9583662932909,93.,-84.4746548707751));
#62114=CARTESIAN_POINT('',(-50.5208498351691,93.,-71.0728718557939));
#62115=CARTESIAN_POINT('',(-22.8237122821307,93.,-48.9392764697909));
#62116=CARTESIAN_POINT('',(-53.2091161828892,93.,-70.0209415458165));
#62117=CARTESIAN_POINT('',(-4.52749723081664,93.,-89.0702707009757));
#62118=CARTESIAN_POINT('',(-53.6422509852979,93.,-67.1668694415634));
#62119=CARTESIAN_POINT('',(-50.901764186322,93.,-85.2248663550737));
#62120=CARTESIAN_POINT('',(-25.9451134322595,93.,-45.0332740555604));
#62121=CARTESIAN_POINT('',(19.5814062643922,93.,-100.109775630374));
#62122=CARTESIAN_POINT('',(22.2696726121122,93.,-101.161705940351));
#62123=CARTESIAN_POINT('',(-5.07234368536324,93.,-90.4626560848171));
#62124=CARTESIAN_POINT('',(22.7028074145209,93.,-104.015778044604));
#62125=CARTESIAN_POINT('',(18.2582560524041,93.,-74.729121816579));
#62126=CARTESIAN_POINT('',(20.4476758692096,93.,-105.81791983888));
#62127=CARTESIAN_POINT('',(21.779297126192,93.,-104.753782216246));
#62128=CARTESIAN_POINT('',(17.7594095214895,93.,-104.765989528902));
#62129=CARTESIAN_POINT('',(-6.89434042826585,93.,-95.1188699833458));
#62130=CARTESIAN_POINT('',(17.3262747190808,93.,-101.911917424649));
#62131=CARTESIAN_POINT('',(13.3148581593725,93.,-75.4793333008771));
#62132=CARTESIAN_POINT('',(18.6578959760632,93.,-100.847779802016));
#62133=CARTESIAN_POINT('',(12.597085416599,93.,-97.3767805160198));
#62134=CARTESIAN_POINT('',(15.285351764319,93.,-98.4287108259972));
#62135=CARTESIAN_POINT('',(-5.07234368536323,93.,-90.4626560848171));
#62136=CARTESIAN_POINT('',(15.7184865667278,93.,-101.28278293025));
#62137=CARTESIAN_POINT('',(11.8365938178346,93.,-75.7036751219986));
#62138=CARTESIAN_POINT('',(13.4633550214164,93.,-103.084924724526));
#62139=CARTESIAN_POINT('',(17.7244780890717,93.,-99.6797362392957));
#62140=CARTESIAN_POINT('',(10.7750886736964,93.,-102.032994414549));
#62141=CARTESIAN_POINT('',(-6.89434042826585,93.,-95.1188699833458));
#62142=CARTESIAN_POINT('',(10.3419538712877,93.,-99.1789223102955));
#62143=CARTESIAN_POINT('',(6.89319592480304,93.,-76.4538866062968));
#62144=CARTESIAN_POINT('',(14.603076938943,93.,-95.7737338250652));
#62145=CARTESIAN_POINT('',(5.6127645688059,93.,-94.6437854016659));
#62146=CARTESIAN_POINT('',(8.3010309165259,93.,-95.6957157116433));
#62147=CARTESIAN_POINT('',(-5.07234368536323,93.,-90.4626560848171));
#62148=CARTESIAN_POINT('',(8.73416571893462,93.,-98.5497878158964));
#62149=CARTESIAN_POINT('',(5.4149315832651,93.,-76.6782284274182));
#62150=CARTESIAN_POINT('',(6.4790341736233,93.,-100.351929610172));
#62151=CARTESIAN_POINT('',(13.6696590519515,93.,-94.6056902623452));
#62152=CARTESIAN_POINT('',(3.79076782590327,93.,-99.2999993001947));
#62153=CARTESIAN_POINT('',(-6.89434042826585,93.,-95.1188699833458));
#62154=CARTESIAN_POINT('',(3.35763302349454,93.,-96.4459271959416));
#62155=CARTESIAN_POINT('',(0.471533690233591,93.,-77.4284399117164));
#62156=CARTESIAN_POINT('',(10.5482579018228,93.,-90.6996878481147));
#62157=CARTESIAN_POINT('',(-1.37155627898724,93.,-91.910790287312));
#62158=CARTESIAN_POINT('',(1.31671006873277,93.,-92.9627205972894));
#62159=CARTESIAN_POINT('',(-5.07234368536322,93.,-90.4626560848171));
#62160=CARTESIAN_POINT('',(1.74984487114149,93.,-95.8167927015425));
#62161=CARTESIAN_POINT('',(-1.00673065130438,93.,-77.6527817328378));
#62162=CARTESIAN_POINT('',(-0.505286674169835,93.,-97.6189344958182));
#62163=CARTESIAN_POINT('',(9.61484001483126,93.,-89.5316442853947));
#62164=CARTESIAN_POINT('',(-3.19355302188986,93.,-96.5670041858408));
#62165=CARTESIAN_POINT('',(-6.89434042826585,93.,-95.1188699833458));
#62166=CARTESIAN_POINT('',(-3.6266878242986,93.,-93.7129320815877));
#62167=CARTESIAN_POINT('',(-5.95012854433586,93.,-78.4029932171361));
#62168=CARTESIAN_POINT('',(6.4934388647025,93.,-85.6256418711642));
#62169=CARTESIAN_POINT('',(7.86339902170064,93.,-109.47397908076));
#62170=CARTESIAN_POINT('',(10.5516653694206,93.,-110.525909390737));
#62171=CARTESIAN_POINT('',(-9.80603008026165,93.,-102.559854649557));
#62172=CARTESIAN_POINT('',(10.9848001718294,93.,-113.379981494991));
#62173=CARTESIAN_POINT('',(5.41493158326524,93.,-76.6782284274182));
#62174=CARTESIAN_POINT('',(8.72966862651804,93.,-115.182123289266));
#62175=CARTESIAN_POINT('',(21.779297126192,93.,-104.753782216246));
#62176=CARTESIAN_POINT('',(6.04140227879801,93.,-114.130192979289));
#62177=CARTESIAN_POINT('',(-11.6280268231643,93.,-107.216068548086));
#62178=CARTESIAN_POINT('',(5.60826747638928,93.,-111.276120875036));
#62179=CARTESIAN_POINT('',(0.471533690233623,93.,-77.4284399117164));
#62180=CARTESIAN_POINT('',(18.6578959760633,93.,-100.847779802016));
#62181=CARTESIAN_POINT('',(14.8477198694938,93.,-112.206974195114));
#62182=CARTESIAN_POINT('',(17.5359862172138,93.,-113.258904505091));
#62183=CARTESIAN_POINT('',(-9.80603008026165,93.,-102.559854649557));
#62184=CARTESIAN_POINT('',(17.9691210196225,93.,-116.112976609344));
#62185=CARTESIAN_POINT('',(11.8365938178347,93.,-75.7036751219986));
#62186=CARTESIAN_POINT('',(15.7139894743112,93.,-117.91511840362));
#62187=CARTESIAN_POINT('',(25.8341161633122,93.,-109.827828193197));
#62188=CARTESIAN_POINT('',(13.0257231265911,93.,-116.863188093643));
#62189=CARTESIAN_POINT('',(-11.6280268231643,93.,-107.216068548086));
#62190=CARTESIAN_POINT('',(12.5925883241824,93.,-114.00911598939));
#62191=CARTESIAN_POINT('',(6.89319592480307,93.,-76.4538866062968));
#62192=CARTESIAN_POINT('',(22.7127150131835,93.,-105.921825778966));
#62193=CARTESIAN_POINT('',(21.8320407172869,93.,-114.939969309468));
#62194=CARTESIAN_POINT('',(24.5203070650069,93.,-115.991899619445));
#62195=CARTESIAN_POINT('',(-9.80603008026166,93.,-102.559854649557));
#62196=CARTESIAN_POINT('',(24.9534418674156,93.,-118.845971723698));
#62197=CARTESIAN_POINT('',(18.2582560524042,93.,-74.729121816579));
#62198=CARTESIAN_POINT('',(22.6983103221043,93.,-120.648113517974));
#62199=CARTESIAN_POINT('',(29.8889352004325,93.,-114.901874170147));
#62200=CARTESIAN_POINT('',(20.0100439743843,93.,-119.596183207997));
#62201=CARTESIAN_POINT('',(-11.6280268231643,93.,-107.216068548086));
#62202=CARTESIAN_POINT('',(19.5769091719755,93.,-116.742111103744));
#62203=CARTESIAN_POINT('',(13.3148581593725,93.,-75.4793333008771));
#62204=CARTESIAN_POINT('',(26.7675340503038,93.,-110.995871755917));
#62205=CARTESIAN_POINT('',(28.81636156508,93.,-117.672964423822));
#62206=CARTESIAN_POINT('',(31.5046279128,93.,-118.724894733799));
#62207=CARTESIAN_POINT('',(-9.80603008026167,93.,-102.559854649557));
#62208=CARTESIAN_POINT('',(31.9377627152088,93.,-121.578966838052));
#62209=CARTESIAN_POINT('',(24.6799182869737,93.,-73.7545685111593));
#62210=CARTESIAN_POINT('',(29.6826311698974,93.,-123.381108632328));
#62211=CARTESIAN_POINT('',(33.9437542375527,93.,-119.975920147098));
#62212=CARTESIAN_POINT('',(26.9943648221774,93.,-122.32917832235));
#62213=CARTESIAN_POINT('',(-11.6280268231643,93.,-107.216068548086));
#62214=CARTESIAN_POINT('',(26.5612300197687,93.,-119.475106218097));
#62215=CARTESIAN_POINT('',(19.736520393942,93.,-74.5047799954575));
#62216=CARTESIAN_POINT('',(30.822353087424,93.,-116.069917732867));
#62217=CARTESIAN_POINT('',(-49.1364849870918,93.,-80.1949213263819));
#62218=CARTESIAN_POINT('',(-46.4482186393718,93.,-81.2468516363593));
#62219=CARTESIAN_POINT('',(-7.4391868828124,93.,-96.5112553671871));
#62220=CARTESIAN_POINT('',(-46.0150838369631,93.,-84.1009237406124));
#62221=CARTESIAN_POINT('',(-45.9583662932907,93.,-84.4746548707751));
#62222=CARTESIAN_POINT('',(-48.2702153822744,93.,-85.9030655348881));
#62223=CARTESIAN_POINT('',(-14.7140742078902,93.,-59.0873684236919));
#62224=CARTESIAN_POINT('',(-50.9584817299944,93.,-84.8511352249106));
#62225=CARTESIAN_POINT('',(-9.26118362571508,93.,-101.167469265716));
#62226=CARTESIAN_POINT('',(-51.3916165324031,93.,-81.9970631206576));
#62227=CARTESIAN_POINT('',(-50.901764186322,93.,-85.2248663550737));
#62228=CARTESIAN_POINT('',(-17.835475358019,93.,-55.1813660094614));
#62229=CARTESIAN_POINT('',(-42.1521641392987,93.,-82.9279164407358));
#62230=CARTESIAN_POINT('',(-39.4638977915786,93.,-83.9798467507132));
#62231=CARTESIAN_POINT('',(-7.43918688281241,93.,-96.5112553671871));
#62232=CARTESIAN_POINT('',(-39.0307629891699,93.,-86.8339188549663));
#62233=CARTESIAN_POINT('',(-39.5367040587212,93.,-83.5001015653555));
#62234=CARTESIAN_POINT('',(-41.2858945344813,93.,-88.636060649242));
#62235=CARTESIAN_POINT('',(-10.65925517077,93.,-64.1614144006424));
#62236=CARTESIAN_POINT('',(-43.9741608822013,93.,-87.5841303392645));
#62237=CARTESIAN_POINT('',(-9.26118362571508,93.,-101.167469265716));
#62238=CARTESIAN_POINT('',(-44.40729568461,93.,-84.7300582350115));
#62239=CARTESIAN_POINT('',(-44.4801019517526,93.,-84.250313049654));
#62240=CARTESIAN_POINT('',(-13.7806563208988,93.,-60.2554119864119));
#62241=CARTESIAN_POINT('',(-35.1678432915055,93.,-85.6609115550896));
#62242=CARTESIAN_POINT('',(-32.4795769437855,93.,-86.7128418650671));
#62243=CARTESIAN_POINT('',(-7.43918688281241,93.,-96.5112553671871));
#62244=CARTESIAN_POINT('',(-32.0464421413768,93.,-89.5669139693202));
#62245=CARTESIAN_POINT('',(-33.1150418241517,93.,-82.5255482599359));
#62246=CARTESIAN_POINT('',(-34.3015736866881,93.,-91.3690557635958));
#62247=CARTESIAN_POINT('',(-6.60443613364972,93.,-69.2354603775928));
#62248=CARTESIAN_POINT('',(-36.9898400344081,93.,-90.3171254536184));
#62249=CARTESIAN_POINT('',(-9.26118362571508,93.,-101.167469265716));
#62250=CARTESIAN_POINT('',(-37.4229748368169,93.,-87.4630533493654));
#62251=CARTESIAN_POINT('',(-38.0584397171831,93.,-83.2757597442344));
#62252=CARTESIAN_POINT('',(-9.7258372837785,93.,-65.3294579633623));
#62253=CARTESIAN_POINT('',(-28.1835224437124,93.,-88.3939066694435));
#62254=CARTESIAN_POINT('',(-25.4952560959924,93.,-89.4458369794209));
#62255=CARTESIAN_POINT('',(-7.43918688281242,93.,-96.5112553671871));
#62256=CARTESIAN_POINT('',(-25.0621212935837,93.,-92.2999090836741));
#62257=CARTESIAN_POINT('',(-26.6933795895823,93.,-81.5509949545163));
#62258=CARTESIAN_POINT('',(-27.317252838895,93.,-94.1020508779497));
#62259=CARTESIAN_POINT('',(-2.54961709652947,93.,-74.3095063545433));
#62260=CARTESIAN_POINT('',(-30.005519186615,93.,-93.0501205679723));
#62261=CARTESIAN_POINT('',(-9.26118362571508,93.,-101.167469265716));
#62262=CARTESIAN_POINT('',(-30.4386539890237,93.,-90.1960484637193));
#62263=CARTESIAN_POINT('',(-31.6367774826137,93.,-82.3012064388147));
#62264=CARTESIAN_POINT('',(-5.67101824665825,93.,-70.4035039403128));
#62265=CARTESIAN_POINT('',(-21.1992015959193,93.,-91.1269017837974));
#62266=CARTESIAN_POINT('',(-18.5109352481993,93.,-92.1788320937748));
#62267=CARTESIAN_POINT('',(-7.43918688281242,93.,-96.5112553671871));
#62268=CARTESIAN_POINT('',(-18.0778004457905,93.,-95.0329041980279));
#62269=CARTESIAN_POINT('',(-20.2717173550128,93.,-80.5764416490967));
#62270=CARTESIAN_POINT('',(-20.3329319911019,93.,-96.8350459923036));
#62271=CARTESIAN_POINT('',(1.50520194059077,93.,-79.3835523314938));
#62272=CARTESIAN_POINT('',(-23.0211983388219,93.,-95.7831156823262));
#62273=CARTESIAN_POINT('',(-9.26118362571508,93.,-101.167469265716));
#62274=CARTESIAN_POINT('',(-23.4543331412306,93.,-92.9290435780731));
#62275=CARTESIAN_POINT('',(-25.2151152480442,93.,-81.326653133395));
#62276=CARTESIAN_POINT('',(-1.616199209538,93.,-75.4775499172633));
#62277=CARTESIAN_POINT('',(-14.2148807481261,93.,-93.8598968981513));
#62278=CARTESIAN_POINT('',(-11.5266144004061,93.,-94.9118272081287));
#62279=CARTESIAN_POINT('',(-7.43918688281243,93.,-96.5112553671872));
#62280=CARTESIAN_POINT('',(-11.0934795979974,93.,-97.7658993123818));
#62281=CARTESIAN_POINT('',(-13.8500551204433,93.,-79.601888343677));
#62282=CARTESIAN_POINT('',(-13.3486111433087,93.,-99.5680411066575));
#62283=CARTESIAN_POINT('',(5.56002097771102,93.,-84.4575983084442));
#62284=CARTESIAN_POINT('',(-16.0368774910288,93.,-98.5161107966801));
#62285=CARTESIAN_POINT('',(-9.26118362571508,93.,-101.167469265716));
#62286=CARTESIAN_POINT('',(-16.4700122934375,93.,-95.662038692427));
#62287=CARTESIAN_POINT('',(-18.7934530134748,93.,-80.3520998279754));
#62288=CARTESIAN_POINT('',(2.43861982758225,93.,-80.5515958942138));
#62289=CARTESIAN_POINT('',(-7.230559900333,93.,-96.5928920125052));
#62290=CARTESIAN_POINT('',(-4.54229355261299,93.,-97.6448223224826));
#62291=CARTESIAN_POINT('',(-7.43918688281243,93.,-96.5112553671872));
#62292=CARTESIAN_POINT('',(-4.10915875020428,93.,-100.498894426736));
#62293=CARTESIAN_POINT('',(-7.42839288587381,93.,-78.6273350382574));
#62294=CARTESIAN_POINT('',(-6.3642902955156,93.,-102.301036221011));
#62295=CARTESIAN_POINT('',(9.61484001483127,93.,-89.5316442853947));
#62296=CARTESIAN_POINT('',(-9.05255664323563,93.,-101.249105911034));
#62297=CARTESIAN_POINT('',(-9.26118362571508,93.,-101.167469265716));
#62298=CARTESIAN_POINT('',(-9.48569144564436,93.,-98.3950338067809));
#62299=CARTESIAN_POINT('',(-12.3717907789053,93.,-79.3775465225557));
#62300=CARTESIAN_POINT('',(6.4934388647025,93.,-85.6256418711642));
#62301=CARTESIAN_POINT('',(-0.246239052539871,93.,-99.3258871268591));
#62302=CARTESIAN_POINT('',(2.44202729518014,93.,-100.377817436837));
#62303=CARTESIAN_POINT('',(-7.43918688281244,93.,-96.5112553671872));
#62304=CARTESIAN_POINT('',(2.87516209758886,93.,-103.23188954109));
#62305=CARTESIAN_POINT('',(-1.00673065130432,93.,-77.6527817328378));
#62306=CARTESIAN_POINT('',(0.620030552277533,93.,-105.034031335365));
#62307=CARTESIAN_POINT('',(13.6696590519515,93.,-94.6056902623452));
#62308=CARTESIAN_POINT('',(-2.06823579544249,93.,-103.982101025388));
#62309=CARTESIAN_POINT('',(-9.26118362571508,93.,-101.167469265716));
#62310=CARTESIAN_POINT('',(-2.50137059785123,93.,-101.128028921135));
#62311=CARTESIAN_POINT('',(-5.95012854433585,93.,-78.4029932171361));
#62312=CARTESIAN_POINT('',(10.5482579018228,93.,-90.6996878481147));
#62313=CARTESIAN_POINT('',(6.73808179525326,93.,-102.058882241213));
#62314=CARTESIAN_POINT('',(9.42634814297327,93.,-103.11081255119));
#62315=CARTESIAN_POINT('',(-7.43918688281244,93.,-96.5112553671872));
#62316=CARTESIAN_POINT('',(9.85948294538199,93.,-105.964884655444));
#62317=CARTESIAN_POINT('',(5.41493158326516,93.,-76.6782284274182));
#62318=CARTESIAN_POINT('',(7.60435140007067,93.,-107.767026449719));
#62319=CARTESIAN_POINT('',(17.7244780890718,93.,-99.6797362392957));
#62320=CARTESIAN_POINT('',(4.91608505235064,93.,-106.715096139742));
#62321=CARTESIAN_POINT('',(-9.26118362571508,93.,-101.167469265716));
#62322=CARTESIAN_POINT('',(4.48295024994191,93.,-103.861024035489));
#62323=CARTESIAN_POINT('',(0.471533690233602,93.,-77.4284399117164));
#62324=CARTESIAN_POINT('',(14.603076938943,93.,-95.7737338250652));
#62325=CARTESIAN_POINT('',(13.7224026430464,93.,-104.791877355567));
#62326=CARTESIAN_POINT('',(16.4106689907664,93.,-105.843807665544));
#62327=CARTESIAN_POINT('',(-7.43918688281245,93.,-96.5112553671872));
#62328=CARTESIAN_POINT('',(16.8438037931751,93.,-108.697879769797));
#62329=CARTESIAN_POINT('',(11.8365938178346,93.,-75.7036751219986));
#62330=CARTESIAN_POINT('',(14.5886722478638,93.,-110.500021564073));
#62331=CARTESIAN_POINT('',(21.779297126192,93.,-104.753782216246));
#62332=CARTESIAN_POINT('',(11.9004059001438,93.,-109.448091254096));
#62333=CARTESIAN_POINT('',(-9.26118362571507,93.,-101.167469265716));
#62334=CARTESIAN_POINT('',(11.467271097735,93.,-106.594019149843));
#62335=CARTESIAN_POINT('',(6.89319592480305,93.,-76.4538866062968));
#62336=CARTESIAN_POINT('',(18.6578959760633,93.,-100.847779802016));
#62337=CARTESIAN_POINT('',(20.7067234908395,93.,-107.524872469921));
#62338=CARTESIAN_POINT('',(23.3949898385595,93.,-108.576802779898));
#62339=CARTESIAN_POINT('',(-7.43918688281245,93.,-96.5112553671872));
#62340=CARTESIAN_POINT('',(23.8281246409682,93.,-111.430874884151));
#62341=CARTESIAN_POINT('',(18.2582560524041,93.,-74.729121816579));
#62342=CARTESIAN_POINT('',(21.5729930956569,93.,-113.233016678427));
#62343=CARTESIAN_POINT('',(25.8341161633122,93.,-109.827828193197));
#62344=CARTESIAN_POINT('',(18.8847267479369,93.,-112.18108636845));
#62345=CARTESIAN_POINT('',(-9.26118362571507,93.,-101.167469265716));
#62346=CARTESIAN_POINT('',(18.4515919455282,93.,-109.327014264196));
#62347=CARTESIAN_POINT('',(13.3148581593725,93.,-75.4793333008771));
#62348=CARTESIAN_POINT('',(22.7127150131835,93.,-105.921825778966));
#62349=CARTESIAN_POINT('',(27.6910443386327,93.,-110.257867584275));
#62350=CARTESIAN_POINT('',(30.3793106863527,93.,-111.309797894252));
#62351=CARTESIAN_POINT('',(-7.43918688281246,93.,-96.5112553671872));
#62352=CARTESIAN_POINT('',(30.8124454887614,93.,-114.163869998505));
#62353=CARTESIAN_POINT('',(24.6799182869736,93.,-73.7545685111594));
#62354=CARTESIAN_POINT('',(28.5573139434501,93.,-115.966011792781));
#62355=CARTESIAN_POINT('',(29.8889352004325,93.,-114.901874170147));
#62356=CARTESIAN_POINT('',(25.86904759573,93.,-114.914081482803));
#62357=CARTESIAN_POINT('',(-9.26118362571507,93.,-101.167469265716));
#62358=CARTESIAN_POINT('',(25.4359127933213,93.,-112.06000937855));
#62359=CARTESIAN_POINT('',(19.736520393942,93.,-74.5047799954575));
#62360=CARTESIAN_POINT('',(26.7675340503038,93.,-110.995871755917));
#62361=CARTESIAN_POINT('',(2.46923037857264,93.,-30.6409089600963));
#62362=CARTESIAN_POINT('',(5.15749672629266,93.,-31.6928392700737));
#62363=CARTESIAN_POINT('',(16.2292450916797,93.,-36.0252625434861));
#62364=CARTESIAN_POINT('',(5.59063152870137,93.,-34.5469113743268));
#62365=CARTESIAN_POINT('',(11.8365938178339,93.,-75.7036751219987));
#62366=CARTESIAN_POINT('',(3.33549998339005,93.,-36.3490531686025));
#62367=CARTESIAN_POINT('',(-18.7688932450105,93.,-54.0133224467414));
#62368=CARTESIAN_POINT('',(0.647233635670021,93.,-35.2971228586251));
#62369=CARTESIAN_POINT('',(14.4072483487771,93.,-40.6814764420149));
#62370=CARTESIAN_POINT('',(0.214098833261289,93.,-32.443050754372));
#62371=CARTESIAN_POINT('',(6.89319592480286,93.,-76.4538866062968));
#62372=CARTESIAN_POINT('',(-21.8902943951393,93.,-50.1073200325109));
#62373=CARTESIAN_POINT('',(-4.51509046922049,93.,-27.9079138457424));
#62374=CARTESIAN_POINT('',(-1.82682412150048,93.,-28.9598441557198));
#62375=CARTESIAN_POINT('',(16.2292450916797,93.,-36.0252625434861));
#62376=CARTESIAN_POINT('',(-1.39368931909176,93.,-31.8139162599729));
#62377=CARTESIAN_POINT('',(5.41493158326445,93.,-76.6782284274183));
#62378=CARTESIAN_POINT('',(-3.64882086440308,93.,-33.6160580542486));
#62379=CARTESIAN_POINT('',(-22.8237122821307,93.,-48.9392764697909));
#62380=CARTESIAN_POINT('',(-6.33708721212311,93.,-32.5641277442712));
#62381=CARTESIAN_POINT('',(14.4072483487771,93.,-40.6814764420149));
#62382=CARTESIAN_POINT('',(-6.77022201453184,93.,-29.7100556400181));
#62383=CARTESIAN_POINT('',(0.471533690233403,93.,-77.4284399117165));
#62384=CARTESIAN_POINT('',(-25.9451134322595,93.,-45.0332740555604));
#62385=CARTESIAN_POINT('',(-11.4994113170136,93.,-25.1749187313885));
#62386=CARTESIAN_POINT('',(-8.81114496929361,93.,-26.2268490413659));
#62387=CARTESIAN_POINT('',(16.2292450916797,93.,-36.0252625434861));
#62388=CARTESIAN_POINT('',(-8.37801016688489,93.,-29.080921145619));
#62389=CARTESIAN_POINT('',(-1.00673065130503,93.,-77.6527817328379));
#62390=CARTESIAN_POINT('',(-10.6331417121962,93.,-30.8830629398947));
#62391=CARTESIAN_POINT('',(-26.878531319251,93.,-43.8652304928404));
#62392=CARTESIAN_POINT('',(-13.3214080599162,93.,-29.8311326299173));
#62393=CARTESIAN_POINT('',(14.4072483487771,93.,-40.6814764420149));
#62394=CARTESIAN_POINT('',(-13.754542862325,93.,-26.9770605256642));
#62395=CARTESIAN_POINT('',(-5.95012854433605,93.,-78.4029932171361));
#62396=CARTESIAN_POINT('',(-29.9999324693798,93.,-39.9592280786099));
#62397=CARTESIAN_POINT('',(45.5004726917788,93.,-54.4539764857667));
#62398=CARTESIAN_POINT('',(48.1887390394988,93.,-55.5059067957441));
#62399=CARTESIAN_POINT('',(13.8624018942304,93.,-42.0738618258563));
#62400=CARTESIAN_POINT('',(48.6218738419075,93.,-58.3599788999972));
#62401=CARTESIAN_POINT('',(50.3665672252509,93.,-69.856355289481));
#62402=CARTESIAN_POINT('',(46.3667422965962,93.,-60.1621206942729));
#62403=CARTESIAN_POINT('',(9.61484001483123,93.,-89.5316442853947));
#62404=CARTESIAN_POINT('',(43.6784759488762,93.,-59.1101903842955));
#62405=CARTESIAN_POINT('',(12.0404051513279,93.,-46.730075724385));
#62406=CARTESIAN_POINT('',(43.2453411464674,93.,-56.2561182800424));
#62407=CARTESIAN_POINT('',(45.4231693322196,93.,-70.6065667737789));
#62408=CARTESIAN_POINT('',(6.4934388647025,93.,-85.6256418711642));
#62409=CARTESIAN_POINT('',(9.45355122636578,93.,-33.3739040744502));
#62410=CARTESIAN_POINT('',(12.1418175740858,93.,-34.4258343844276));
#62411=CARTESIAN_POINT('',(16.2292450916796,93.,-36.0252625434861));
#62412=CARTESIAN_POINT('',(12.5749523764945,93.,-37.2799064886807));
#62413=CARTESIAN_POINT('',(18.2582560524034,93.,-74.7291218165791));
#62414=CARTESIAN_POINT('',(10.3198208311832,93.,-39.0820482829564));
#62415=CARTESIAN_POINT('',(-14.7140742078902,93.,-59.0873684236918));
#62416=CARTESIAN_POINT('',(7.63155448346315,93.,-38.030117972979));
#62417=CARTESIAN_POINT('',(14.4072483487771,93.,-40.6814764420149));
#62418=CARTESIAN_POINT('',(7.19841968105442,93.,-35.1760458687259));
#62419=CARTESIAN_POINT('',(13.3148581593723,93.,-75.4793333008772));
#62420=CARTESIAN_POINT('',(-17.835475358019,93.,-55.1813660094614));
#62421=CARTESIAN_POINT('',(16.4378720741589,93.,-36.1068991888041));
#62422=CARTESIAN_POINT('',(19.1261384218789,93.,-37.1588294987815));
#62423=CARTESIAN_POINT('',(16.2292450916796,93.,-36.0252625434861));
#62424=CARTESIAN_POINT('',(19.5592732242876,93.,-40.0129016030346));
#62425=CARTESIAN_POINT('',(24.6799182869729,93.,-73.7545685111595));
#62426=CARTESIAN_POINT('',(17.3041416789763,93.,-41.8150433973103));
#62427=CARTESIAN_POINT('',(-10.65925517077,93.,-64.1614144006423));
#62428=CARTESIAN_POINT('',(14.6158753312563,93.,-40.7631130873329));
#62429=CARTESIAN_POINT('',(14.4072483487771,93.,-40.6814764420149));
#62430=CARTESIAN_POINT('',(14.1827405288475,93.,-37.9090409830798));
#62431=CARTESIAN_POINT('',(19.7365203939418,93.,-74.5047799954575));
#62432=CARTESIAN_POINT('',(-13.7806563208988,93.,-60.2554119864119));
#62433=CARTESIAN_POINT('',(23.422192921952,93.,-38.839894303158));
#62434=CARTESIAN_POINT('',(26.110459269672,93.,-39.8918246131354));
#62435=CARTESIAN_POINT('',(16.2292450916796,93.,-36.0252625434861));
#62436=CARTESIAN_POINT('',(26.5435940720808,93.,-42.7458967173885));
#62437=CARTESIAN_POINT('',(31.1015805215424,93.,-72.7800152057398));
#62438=CARTESIAN_POINT('',(24.2884625267694,93.,-44.5480385116642));
#62439=CARTESIAN_POINT('',(-6.60443613364976,93.,-69.2354603775928));
#62440=CARTESIAN_POINT('',(21.6001961790494,93.,-43.4961082016867));
#62441=CARTESIAN_POINT('',(14.4072483487771,93.,-40.6814764420149));
#62442=CARTESIAN_POINT('',(21.1670613766407,93.,-40.6420360974337));
#62443=CARTESIAN_POINT('',(26.1581826285112,93.,-73.5302266900378));
#62444=CARTESIAN_POINT('',(-9.7258372837785,93.,-65.3294579633623));
#62445=CARTESIAN_POINT('',(30.4065137697452,93.,-41.5728894175119));
#62446=CARTESIAN_POINT('',(33.0947801174652,93.,-42.6248197274893));
#62447=CARTESIAN_POINT('',(16.2292450916796,93.,-36.0252625434861));
#62448=CARTESIAN_POINT('',(33.5279149198739,93.,-45.4788918317424));
#62449=CARTESIAN_POINT('',(37.5232427561119,93.,-71.8054619003202));
#62450=CARTESIAN_POINT('',(31.2727833745626,93.,-47.2810336260181));
#62451=CARTESIAN_POINT('',(-2.54961709652951,93.,-74.3095063545433));
#62452=CARTESIAN_POINT('',(28.5845170268425,93.,-46.2291033160406));
#62453=CARTESIAN_POINT('',(14.4072483487771,93.,-40.6814764420149));
#62454=CARTESIAN_POINT('',(28.1513822244338,93.,-43.3750312117876));
#62455=CARTESIAN_POINT('',(32.5798448630807,93.,-72.5556733846182));
#62456=CARTESIAN_POINT('',(-5.67101824665825,93.,-70.4035039403128));
#62457=CARTESIAN_POINT('',(38.5161518439857,93.,-51.7209813714128));
#62458=CARTESIAN_POINT('',(41.2044181917057,93.,-52.7729116813902));
#62459=CARTESIAN_POINT('',(13.8624018942304,93.,-42.0738618258563));
#62460=CARTESIAN_POINT('',(41.6375529941144,93.,-55.6269837856433));
#62461=CARTESIAN_POINT('',(43.9449049906814,93.,-70.8309085949006));
#62462=CARTESIAN_POINT('',(39.3824214488031,93.,-57.429125579919));
#62463=CARTESIAN_POINT('',(5.56002097771098,93.,-84.4575983084442));
#62464=CARTESIAN_POINT('',(36.694155101083,93.,-56.3771952699416));
#62465=CARTESIAN_POINT('',(12.0404051513279,93.,-46.730075724385));
#62466=CARTESIAN_POINT('',(36.2610202986743,93.,-53.5231231656885));
#62467=CARTESIAN_POINT('',(39.0015070976501,93.,-71.5811200791985));
#62468=CARTESIAN_POINT('',(2.43861982758225,93.,-80.5515958942137));
#62469=CARTESIAN_POINT('',(31.5318309961925,93.,-48.9879862570589));
#62470=CARTESIAN_POINT('',(34.2200973439125,93.,-50.0399165670363));
#62471=CARTESIAN_POINT('',(13.8624018942304,93.,-42.0738618258563));
#62472=CARTESIAN_POINT('',(34.6532321463213,93.,-52.8939886712894));
#62473=CARTESIAN_POINT('',(37.5232427561119,93.,-71.8054619003202));
#62474=CARTESIAN_POINT('',(32.3981006010099,93.,-54.6961304655651));
#62475=CARTESIAN_POINT('',(1.50520194059074,93.,-79.3835523314937));
#62476=CARTESIAN_POINT('',(29.7098342532899,93.,-53.6442001555877));
#62477=CARTESIAN_POINT('',(12.0404051513279,93.,-46.730075724385));
#62478=CARTESIAN_POINT('',(29.2766994508812,93.,-50.7901280513346));
#62479=CARTESIAN_POINT('',(32.5798448630807,93.,-72.5556733846182));
#62480=CARTESIAN_POINT('',(-1.616199209538,93.,-75.4775499172633));
#62481=CARTESIAN_POINT('',(24.5475101483994,93.,-46.254991142705));
#62482=CARTESIAN_POINT('',(27.2357764961194,93.,-47.3069214526824));
#62483=CARTESIAN_POINT('',(13.8624018942304,93.,-42.0738618258562));
#62484=CARTESIAN_POINT('',(27.6689112985281,93.,-50.1609935569356));
#62485=CARTESIAN_POINT('',(31.1015805215425,93.,-72.7800152057398));
#62486=CARTESIAN_POINT('',(25.4137797532168,93.,-51.9631353512112));
#62487=CARTESIAN_POINT('',(-2.5496170965295,93.,-74.3095063545433));
#62488=CARTESIAN_POINT('',(22.7255134054968,93.,-50.9112050412338));
#62489=CARTESIAN_POINT('',(12.0404051513279,93.,-46.730075724385));
#62490=CARTESIAN_POINT('',(22.2923786030881,93.,-48.0571329369807));
#62491=CARTESIAN_POINT('',(26.1581826285112,93.,-73.5302266900378));
#62492=CARTESIAN_POINT('',(-5.67101824665825,93.,-70.4035039403128));
#62493=CARTESIAN_POINT('',(17.5631893006063,93.,-43.5219960283511));
#62494=CARTESIAN_POINT('',(20.2514556483263,93.,-44.5739263383286));
#62495=CARTESIAN_POINT('',(13.8624018942304,93.,-42.0738618258562));
#62496=CARTESIAN_POINT('',(20.684590450735,93.,-47.4279984425817));
#62497=CARTESIAN_POINT('',(24.679918286973,93.,-73.7545685111594));
#62498=CARTESIAN_POINT('',(18.4294589054237,93.,-49.2301402368573));
#62499=CARTESIAN_POINT('',(-6.60443613364975,93.,-69.2354603775928));
#62500=CARTESIAN_POINT('',(15.7411925577037,93.,-48.1782099268799));
#62501=CARTESIAN_POINT('',(12.0404051513279,93.,-46.730075724385));
#62502=CARTESIAN_POINT('',(15.3080577552949,93.,-45.3241378226269));
#62503=CARTESIAN_POINT('',(19.7365203939418,93.,-74.5047799954575));
#62504=CARTESIAN_POINT('',(-9.7258372837785,93.,-65.3294579633623));
#62505=CARTESIAN_POINT('',(10.5788684528132,93.,-40.7890009139973));
#62506=CARTESIAN_POINT('',(13.2671348005332,93.,-41.8409312239747));
#62507=CARTESIAN_POINT('',(13.8624018942304,93.,-42.0738618258562));
#62508=CARTESIAN_POINT('',(13.7002696029419,93.,-44.6950033282278));
#62509=CARTESIAN_POINT('',(18.2582560524035,93.,-74.7291218165791));
#62510=CARTESIAN_POINT('',(11.4451380576306,93.,-46.4971451225034));
#62511=CARTESIAN_POINT('',(-10.65925517077,93.,-64.1614144006423));
#62512=CARTESIAN_POINT('',(8.75687170991053,93.,-45.445214812526));
#62513=CARTESIAN_POINT('',(12.0404051513279,93.,-46.730075724385));
#62514=CARTESIAN_POINT('',(8.32373690750179,93.,-42.591142708273));
#62515=CARTESIAN_POINT('',(13.3148581593723,93.,-75.4793333008771));
#62516=CARTESIAN_POINT('',(-13.7806563208988,93.,-60.2554119864119));
#62517=CARTESIAN_POINT('',(3.59454760502002,93.,-38.0560057996434));
#62518=CARTESIAN_POINT('',(6.28281395274003,93.,-39.1079361096208));
#62519=CARTESIAN_POINT('',(13.8624018942304,93.,-42.0738618258562));
#62520=CARTESIAN_POINT('',(6.71594875514875,93.,-41.9620082138739));
#62521=CARTESIAN_POINT('',(11.836593817834,93.,-75.7036751219987));
#62522=CARTESIAN_POINT('',(4.46081720983743,93.,-43.7641500081495));
#62523=CARTESIAN_POINT('',(-14.7140742078902,93.,-59.0873684236918));
#62524=CARTESIAN_POINT('',(1.7725508621174,93.,-42.7122196981721));
#62525=CARTESIAN_POINT('',(12.0404051513279,93.,-46.730075724385));
#62526=CARTESIAN_POINT('',(1.33941605970866,93.,-39.8581475939191));
#62527=CARTESIAN_POINT('',(6.89319592480288,93.,-76.4538866062968));
#62528=CARTESIAN_POINT('',(-17.835475358019,93.,-55.1813660094614));
#62529=CARTESIAN_POINT('',(-3.38977324277311,93.,-35.3230106852895));
#62530=CARTESIAN_POINT('',(-0.701506895053102,93.,-36.3749409952669));
#62531=CARTESIAN_POINT('',(13.8624018942304,93.,-42.0738618258562));
#62532=CARTESIAN_POINT('',(-0.268372092644385,93.,-39.22901309952));
#62533=CARTESIAN_POINT('',(5.41493158326452,93.,-76.6782284274183));
#62534=CARTESIAN_POINT('',(-2.52350363795571,93.,-41.0311548937957));
#62535=CARTESIAN_POINT('',(-18.7688932450105,93.,-54.0133224467414));
#62536=CARTESIAN_POINT('',(-5.21176998567574,93.,-39.9792245838182));
#62537=CARTESIAN_POINT('',(12.0404051513279,93.,-46.730075724385));
#62538=CARTESIAN_POINT('',(-5.64490478808447,93.,-37.1251524795652));
#62539=CARTESIAN_POINT('',(0.471533690233424,93.,-77.4284399117165));
#62540=CARTESIAN_POINT('',(-21.8902943951393,93.,-50.1073200325109));
#62541=CARTESIAN_POINT('',(-10.3740940905662,93.,-32.5900155709356));
#62542=CARTESIAN_POINT('',(-7.68582774284623,93.,-33.641945880913));
#62543=CARTESIAN_POINT('',(13.8624018942304,93.,-42.0738618258562));
#62544=CARTESIAN_POINT('',(-7.25269294043752,93.,-36.4960179851661));
#62545=CARTESIAN_POINT('',(-1.00673065130496,93.,-77.6527817328379));
#62546=CARTESIAN_POINT('',(-9.50782448574884,93.,-38.2981597794418));
#62547=CARTESIAN_POINT('',(-22.8237122821307,93.,-48.9392764697909));
#62548=CARTESIAN_POINT('',(-12.1960908334689,93.,-37.2462294694643));
#62549=CARTESIAN_POINT('',(12.0404051513279,93.,-46.730075724385));
#62550=CARTESIAN_POINT('',(-12.6292256358776,93.,-34.3921573652113));
#62551=CARTESIAN_POINT('',(-5.95012854433603,93.,-78.4029932171361));
#62552=CARTESIAN_POINT('',(-25.9451134322595,93.,-45.0332740555604));
#62553=CARTESIAN_POINT('',(36.2655173910909,93.,-36.8907876923187));
#62554=CARTESIAN_POINT('',(38.9537837388109,93.,-37.9427180022961));
#62555=CARTESIAN_POINT('',(18.5960882891288,93.,-29.976663261116));
#62556=CARTESIAN_POINT('',(39.3869185412196,93.,-40.7967901065492));
#62557=CARTESIAN_POINT('',(43.9449049906813,93.,-70.8309085949006));
#62558=CARTESIAN_POINT('',(37.1317869959083,93.,-42.5989319008249));
#62559=CARTESIAN_POINT('',(-2.54961709652952,93.,-74.3095063545432));
#62560=CARTESIAN_POINT('',(34.4435206481883,93.,-41.5470015908475));
#62561=CARTESIAN_POINT('',(16.7740915462264,93.,-34.6328771596448));
#62562=CARTESIAN_POINT('',(34.0103858457796,93.,-38.6929294865944));
#62563=CARTESIAN_POINT('',(39.0015070976501,93.,-71.5811200791985));
#62564=CARTESIAN_POINT('',(-5.67101824665826,93.,-70.4035039403128));
#62565=CARTESIAN_POINT('',(29.2811965432978,93.,-34.1577925779648));
#62566=CARTESIAN_POINT('',(31.9694628910178,93.,-35.2097228879422));
#62567=CARTESIAN_POINT('',(18.5960882891288,93.,-29.976663261116));
#62568=CARTESIAN_POINT('',(32.4025976934265,93.,-38.0637949921953));
#62569=CARTESIAN_POINT('',(37.5232427561118,93.,-71.8054619003203));
#62570=CARTESIAN_POINT('',(30.1474661481152,93.,-39.865936786471));
#62571=CARTESIAN_POINT('',(-6.60443613364976,93.,-69.2354603775928));
#62572=CARTESIAN_POINT('',(27.4591998003952,93.,-38.8140064764936));
#62573=CARTESIAN_POINT('',(16.7740915462264,93.,-34.6328771596448));
#62574=CARTESIAN_POINT('',(27.0260649979864,93.,-35.9599343722405));
#62575=CARTESIAN_POINT('',(32.5798448630806,93.,-72.5556733846182));
#62576=CARTESIAN_POINT('',(-9.72583728377851,93.,-65.3294579633623));
#62577=CARTESIAN_POINT('',(22.2968756955047,93.,-31.4247974636109));
#62578=CARTESIAN_POINT('',(24.9851420432247,93.,-32.4767277735883));
#62579=CARTESIAN_POINT('',(18.5960882891288,93.,-29.976663261116));
#62580=CARTESIAN_POINT('',(25.4182768456334,93.,-35.3307998778414));
#62581=CARTESIAN_POINT('',(31.1015805215423,93.,-72.7800152057399));
#62582=CARTESIAN_POINT('',(23.1631453003221,93.,-37.1329416721171));
#62583=CARTESIAN_POINT('',(-10.65925517077,93.,-64.1614144006423));
#62584=CARTESIAN_POINT('',(20.474878952602,93.,-36.0810113621397));
#62585=CARTESIAN_POINT('',(16.7740915462264,93.,-34.6328771596448));
#62586=CARTESIAN_POINT('',(20.0417441501933,93.,-33.2269392578866));
#62587=CARTESIAN_POINT('',(26.1581826285112,93.,-73.5302266900378));
#62588=CARTESIAN_POINT('',(-13.7806563208988,93.,-60.2554119864118));
#62589=CARTESIAN_POINT('',(15.3125548477115,93.,-28.691802349257));
#62590=CARTESIAN_POINT('',(18.0008211954315,93.,-29.7437326592344));
#62591=CARTESIAN_POINT('',(18.5960882891289,93.,-29.976663261116));
#62592=CARTESIAN_POINT('',(18.4339559978403,93.,-32.5978047634875));
#62593=CARTESIAN_POINT('',(24.6799182869728,93.,-73.7545685111595));
#62594=CARTESIAN_POINT('',(16.1788244525289,93.,-34.3999465577632));
#62595=CARTESIAN_POINT('',(-14.7140742078902,93.,-59.0873684236918));
#62596=CARTESIAN_POINT('',(13.4905581048089,93.,-33.3480162477858));
#62597=CARTESIAN_POINT('',(16.7740915462264,93.,-34.6328771596448));
#62598=CARTESIAN_POINT('',(13.0574233024002,93.,-30.4939441435327));
#62599=CARTESIAN_POINT('',(19.7365203939417,93.,-74.5047799954575));
#62600=CARTESIAN_POINT('',(-17.835475358019,93.,-55.1813660094614));
#62601=CARTESIAN_POINT('',(8.3282339999184,93.,-25.9588072349031));
#62602=CARTESIAN_POINT('',(11.0165003476384,93.,-27.0107375448806));
#62603=CARTESIAN_POINT('',(18.5960882891289,93.,-29.976663261116));
#62604=CARTESIAN_POINT('',(11.4496351500471,93.,-29.8648096491337));
#62605=CARTESIAN_POINT('',(18.2582560524034,93.,-74.7291218165791));
#62606=CARTESIAN_POINT('',(9.1945036047358,93.,-31.6669514434093));
#62607=CARTESIAN_POINT('',(-18.7688932450105,93.,-54.0133224467413));
#62608=CARTESIAN_POINT('',(6.50623725701577,93.,-30.6150211334319));
#62609=CARTESIAN_POINT('',(16.7740915462264,93.,-34.6328771596448));
#62610=CARTESIAN_POINT('',(6.07310245460704,93.,-27.7609490291788));
#62611=CARTESIAN_POINT('',(13.3148581593723,93.,-75.4793333008772));
#62612=CARTESIAN_POINT('',(-21.8902943951393,93.,-50.1073200325109));
#62613=CARTESIAN_POINT('',(1.34391315212527,93.,-23.2258121205493));
#62614=CARTESIAN_POINT('',(4.03217949984528,93.,-24.2777424305267));
#62615=CARTESIAN_POINT('',(18.5960882891289,93.,-29.976663261116));
#62616=CARTESIAN_POINT('',(4.465314302254,93.,-27.1318145347798));
#62617=CARTESIAN_POINT('',(11.8365938178339,93.,-75.7036751219987));
#62618=CARTESIAN_POINT('',(2.21018275694267,93.,-28.9339563290554));
#62619=CARTESIAN_POINT('',(-22.8237122821307,93.,-48.9392764697909));
#62620=CARTESIAN_POINT('',(-0.478083590777355,93.,-27.882026019078));
#62621=CARTESIAN_POINT('',(16.7740915462264,93.,-34.6328771596448));
#62622=CARTESIAN_POINT('',(-0.911218393186086,93.,-25.0279539148249));
#62623=CARTESIAN_POINT('',(6.89319592480284,93.,-76.4538866062968));
#62624=CARTESIAN_POINT('',(-25.9451134322595,93.,-45.0332740555604));
#62625=CARTESIAN_POINT('',(44.3751554653314,93.,-47.0388796462197));
#62626=CARTESIAN_POINT('',(47.0634218130514,93.,-48.0908099561971));
#62627=CARTESIAN_POINT('',(16.2292450916796,93.,-36.0252625434862));
#62628=CARTESIAN_POINT('',(47.4965566154602,93.,-50.9448820604502));
#62629=CARTESIAN_POINT('',(50.3665672252508,93.,-69.856355289481));
#62630=CARTESIAN_POINT('',(45.2414250701488,93.,-52.7470238547258));
#62631=CARTESIAN_POINT('',(5.56002097771098,93.,-84.4575983084442));
#62632=CARTESIAN_POINT('',(42.5531587224288,93.,-51.6950935447484));
#62633=CARTESIAN_POINT('',(14.4072483487771,93.,-40.6814764420149));
#62634=CARTESIAN_POINT('',(42.1200239200201,93.,-48.8410214404954));
#62635=CARTESIAN_POINT('',(45.4231693322196,93.,-70.6065667737789));
#62636=CARTESIAN_POINT('',(2.43861982758225,93.,-80.5515958942138));
#62637=CARTESIAN_POINT('',(37.3908346175383,93.,-44.3058845318658));
#62638=CARTESIAN_POINT('',(40.0791009652583,93.,-45.3578148418432));
#62639=CARTESIAN_POINT('',(16.2292450916796,93.,-36.0252625434862));
#62640=CARTESIAN_POINT('',(40.512235767667,93.,-48.2118869460963));
#62641=CARTESIAN_POINT('',(43.9449049906814,93.,-70.8309085949006));
#62642=CARTESIAN_POINT('',(38.2571042223557,93.,-50.014028740372));
#62643=CARTESIAN_POINT('',(1.50520194059074,93.,-79.3835523314937));
#62644=CARTESIAN_POINT('',(35.5688378746357,93.,-48.9620984303945));
#62645=CARTESIAN_POINT('',(14.4072483487771,93.,-40.6814764420149));
#62646=CARTESIAN_POINT('',(35.1357030722269,93.,-46.1080263261415));
#62647=CARTESIAN_POINT('',(39.0015070976501,93.,-71.5811200791985));
#62648=CARTESIAN_POINT('',(-1.616199209538,93.,-75.4775499172633));
#62649=CARTESIAN_POINT('',(33.7824654490873,93.,-63.818179936153));
#62650=CARTESIAN_POINT('',(36.4707317968073,93.,-64.8701102461305));
#62651=CARTESIAN_POINT('',(9.128715499332,93.,-54.1710603905965));
#62652=CARTESIAN_POINT('',(36.903866599216,93.,-67.7241823503836));
#62653=CARTESIAN_POINT('',(37.5232427561121,93.,-71.8054619003202));
#62654=CARTESIAN_POINT('',(34.6487350539047,93.,-69.5263241446592));
#62655=CARTESIAN_POINT('',(9.61484001483124,93.,-89.5316442853947));
#62656=CARTESIAN_POINT('',(31.9604687061847,93.,-68.4743938346818));
#62657=CARTESIAN_POINT('',(7.30671875642947,93.,-58.8272742891252));
#62658=CARTESIAN_POINT('',(31.5273339037759,93.,-65.6203217304287));
#62659=CARTESIAN_POINT('',(32.5798448630807,93.,-72.5556733846182));
#62660=CARTESIAN_POINT('',(6.4934388647025,93.,-85.6256418711642));
#62661=CARTESIAN_POINT('',(26.7981446012942,93.,-61.0851848217992));
#62662=CARTESIAN_POINT('',(29.4864109490142,93.,-62.1371151317766));
#62663=CARTESIAN_POINT('',(9.128715499332,93.,-54.1710603905965));
#62664=CARTESIAN_POINT('',(29.9195457514229,93.,-64.9911872360297));
#62665=CARTESIAN_POINT('',(31.1015805215426,93.,-72.7800152057398));
#62666=CARTESIAN_POINT('',(27.6644142061116,93.,-66.7933290303053));
#62667=CARTESIAN_POINT('',(5.560020977711,93.,-84.4575983084442));
#62668=CARTESIAN_POINT('',(24.9761478583915,93.,-65.7413987203279));
#62669=CARTESIAN_POINT('',(7.30671875642947,93.,-58.8272742891252));
#62670=CARTESIAN_POINT('',(24.5430130559828,93.,-62.8873266160749));
#62671=CARTESIAN_POINT('',(26.1581826285113,93.,-73.5302266900378));
#62672=CARTESIAN_POINT('',(2.43861982758225,93.,-80.5515958942138));
#62673=CARTESIAN_POINT('',(19.813823753501,93.,-58.3521897074453));
#62674=CARTESIAN_POINT('',(22.502090101221,93.,-59.4041200174227));
#62675=CARTESIAN_POINT('',(9.12871549933201,93.,-54.1710603905965));
#62676=CARTESIAN_POINT('',(22.9352249036298,93.,-62.2581921216758));
#62677=CARTESIAN_POINT('',(24.6799182869731,93.,-73.7545685111594));
#62678=CARTESIAN_POINT('',(20.6800933583184,93.,-64.0603339159514));
#62679=CARTESIAN_POINT('',(1.50520194059075,93.,-79.3835523314937));
#62680=CARTESIAN_POINT('',(17.9918270105984,93.,-63.008403605974));
#62681=CARTESIAN_POINT('',(7.30671875642947,93.,-58.8272742891252));
#62682=CARTESIAN_POINT('',(17.5586922081897,93.,-60.154331501721));
#62683=CARTESIAN_POINT('',(19.7365203939418,93.,-74.5047799954575));
#62684=CARTESIAN_POINT('',(-1.616199209538,93.,-75.4775499172633));
#62685=CARTESIAN_POINT('',(12.8295029057079,93.,-55.6191945930914));
#62686=CARTESIAN_POINT('',(15.5177692534279,93.,-56.6711249030688));
#62687=CARTESIAN_POINT('',(9.12871549933201,93.,-54.1710603905965));
#62688=CARTESIAN_POINT('',(15.9509040558366,93.,-59.5251970073219));
#62689=CARTESIAN_POINT('',(18.2582560524036,93.,-74.7291218165791));
#62690=CARTESIAN_POINT('',(13.6957725105253,93.,-61.3273388015976));
#62691=CARTESIAN_POINT('',(-2.54961709652949,93.,-74.3095063545433));
#62692=CARTESIAN_POINT('',(11.0075061628053,93.,-60.2754084916201));
#62693=CARTESIAN_POINT('',(7.30671875642947,93.,-58.8272742891252));
#62694=CARTESIAN_POINT('',(10.5743713603965,93.,-57.4213363873671));
#62695=CARTESIAN_POINT('',(13.3148581593724,93.,-75.4793333008771));
#62696=CARTESIAN_POINT('',(-5.67101824665825,93.,-70.4035039403128));
#62697=CARTESIAN_POINT('',(5.84518205791477,93.,-52.8861994787375));
#62698=CARTESIAN_POINT('',(8.53344840563478,93.,-53.9381297887149));
#62699=CARTESIAN_POINT('',(9.12871549933202,93.,-54.1710603905964));
#62700=CARTESIAN_POINT('',(8.9665832080435,93.,-56.792201892968));
#62701=CARTESIAN_POINT('',(11.8365938178341,93.,-75.7036751219987));
#62702=CARTESIAN_POINT('',(6.71145166273218,93.,-58.5943436872437));
#62703=CARTESIAN_POINT('',(-6.60443613364974,93.,-69.2354603775928));
#62704=CARTESIAN_POINT('',(4.02318531501215,93.,-57.5424133772663));
#62705=CARTESIAN_POINT('',(7.30671875642947,93.,-58.8272742891252));
#62706=CARTESIAN_POINT('',(3.59005051260342,93.,-54.6883412730132));
#62707=CARTESIAN_POINT('',(6.89319592480292,93.,-76.4538866062968));
#62708=CARTESIAN_POINT('',(-9.7258372837785,93.,-65.3294579633623));
#62709=CARTESIAN_POINT('',(-1.13913878987836,93.,-50.1532043643836));
#62710=CARTESIAN_POINT('',(1.54912755784165,93.,-51.205134674361));
#62711=CARTESIAN_POINT('',(9.12871549933202,93.,-54.1710603905964));
#62712=CARTESIAN_POINT('',(1.98226236025037,93.,-54.0592067786141));
#62713=CARTESIAN_POINT('',(5.41493158326467,93.,-76.6782284274183));
#62714=CARTESIAN_POINT('',(-0.272869185060958,93.,-55.8613485728898));
#62715=CARTESIAN_POINT('',(-10.65925517077,93.,-64.1614144006423));
#62716=CARTESIAN_POINT('',(-2.96113553278099,93.,-54.8094182629124));
#62717=CARTESIAN_POINT('',(7.30671875642947,93.,-58.8272742891252));
#62718=CARTESIAN_POINT('',(-3.39427033518972,93.,-51.9553461586593));
#62719=CARTESIAN_POINT('',(0.471533690233463,93.,-77.4284399117164));
#62720=CARTESIAN_POINT('',(-13.7806563208987,93.,-60.2554119864119));
#62721=CARTESIAN_POINT('',(-8.12345963767149,93.,-47.4202092500297));
#62722=CARTESIAN_POINT('',(-5.43519328995148,93.,-48.4721395600071));
#62723=CARTESIAN_POINT('',(9.12871549933203,93.,-54.1710603905964));
#62724=CARTESIAN_POINT('',(-5.00205848754277,93.,-51.3262116642602));
#62725=CARTESIAN_POINT('',(-1.00673065130482,93.,-77.6527817328379));
#62726=CARTESIAN_POINT('',(-7.25719003285409,93.,-53.1283534585359));
#62727=CARTESIAN_POINT('',(-14.7140742078902,93.,-59.0873684236919));
#62728=CARTESIAN_POINT('',(-9.94545638057412,93.,-52.0764231485585));
#62729=CARTESIAN_POINT('',(7.30671875642947,93.,-58.8272742891252));
#62730=CARTESIAN_POINT('',(-10.3785911829829,93.,-49.2223510443054));
#62731=CARTESIAN_POINT('',(-5.95012854433599,93.,-78.4029932171361));
#62732=CARTESIAN_POINT('',(-17.835475358019,93.,-55.1813660094614));
#62733=CARTESIAN_POINT('',(-15.1077804854646,93.,-44.6872141356758));
#62734=CARTESIAN_POINT('',(-12.4195141377446,93.,-45.7391444456532));
#62735=CARTESIAN_POINT('',(9.12871549933203,93.,-54.1710603905964));
#62736=CARTESIAN_POINT('',(-11.9863793353359,93.,-48.5932165499063));
#62737=CARTESIAN_POINT('',(-7.4283928858743,93.,-78.6273350382575));
#62738=CARTESIAN_POINT('',(-14.2415108806472,93.,-50.395358344182));
#62739=CARTESIAN_POINT('',(-18.7688932450105,93.,-54.0133224467414));
#62740=CARTESIAN_POINT('',(-16.9297772283673,93.,-49.3434280342046));
#62741=CARTESIAN_POINT('',(7.30671875642947,93.,-58.8272742891252));
#62742=CARTESIAN_POINT('',(-17.362912030776,93.,-46.4893559299515));
#62743=CARTESIAN_POINT('',(-12.3717907789054,93.,-79.3775465225558));
#62744=CARTESIAN_POINT('',(-21.8902943951393,93.,-50.1073200325109));
#62745=CARTESIAN_POINT('',(20.9391409799484,93.,-65.7672865469923));
#62746=CARTESIAN_POINT('',(23.6274073276684,93.,-66.8192168569697));
#62747=CARTESIAN_POINT('',(6.7618723018828,93.,-60.2196596729666));
#62748=CARTESIAN_POINT('',(24.0605421300771,93.,-69.6732889612228));
#62749=CARTESIAN_POINT('',(24.6799182869732,93.,-73.7545685111594));
#62750=CARTESIAN_POINT('',(21.8054105847658,93.,-71.4754307554985));
#62751=CARTESIAN_POINT('',(5.560020977711,93.,-84.4575983084442));
#62752=CARTESIAN_POINT('',(19.1171442370458,93.,-70.4235004455211));
#62753=CARTESIAN_POINT('',(4.93987555898025,93.,-64.8758735714953));
#62754=CARTESIAN_POINT('',(18.684009434637,93.,-67.569428341268));
#62755=CARTESIAN_POINT('',(19.7365203939418,93.,-74.5047799954575));
#62756=CARTESIAN_POINT('',(2.43861982758225,93.,-80.5515958942137));
#62757=CARTESIAN_POINT('',(27.9234618277415,93.,-68.5002816613462));
#62758=CARTESIAN_POINT('',(30.6117281754615,93.,-69.5522119713236));
#62759=CARTESIAN_POINT('',(6.76187230188279,93.,-60.2196596729666));
#62760=CARTESIAN_POINT('',(31.0448629778703,93.,-72.4062840755767));
#62761=CARTESIAN_POINT('',(31.1015805215427,93.,-72.7800152057398));
#62762=CARTESIAN_POINT('',(28.7897314325589,93.,-74.2084258698524));
#62763=CARTESIAN_POINT('',(9.61484001483124,93.,-89.5316442853947));
#62764=CARTESIAN_POINT('',(26.1014650848389,93.,-73.156495559875));
#62765=CARTESIAN_POINT('',(4.93987555898025,93.,-64.8758735714953));
#62766=CARTESIAN_POINT('',(25.6683302824302,93.,-70.3024234556219));
#62767=CARTESIAN_POINT('',(26.1581826285113,93.,-73.5302266900378));
#62768=CARTESIAN_POINT('',(6.4934388647025,93.,-85.6256418711642));
#62769=CARTESIAN_POINT('',(34.9077826755347,93.,-71.2332767757001));
#62770=CARTESIAN_POINT('',(37.5960490232547,93.,-72.2852070856775));
#62771=CARTESIAN_POINT('',(6.76187230188279,93.,-60.2196596729666));
#62772=CARTESIAN_POINT('',(38.0291838256634,93.,-75.1392791899306));
#62773=CARTESIAN_POINT('',(37.5232427561121,93.,-71.8054619003202));
#62774=CARTESIAN_POINT('',(35.7740522803521,93.,-76.9414209842063));
#62775=CARTESIAN_POINT('',(13.6696590519515,93.,-94.6056902623452));
#62776=CARTESIAN_POINT('',(33.085785932632,93.,-75.8894906742289));
#62777=CARTESIAN_POINT('',(4.93987555898025,93.,-64.8758735714953));
#62778=CARTESIAN_POINT('',(32.6526511302233,93.,-73.0354185699758));
#62779=CARTESIAN_POINT('',(32.5798448630807,93.,-72.5556733846182));
#62780=CARTESIAN_POINT('',(10.5482579018227,93.,-90.6996878481147));
#62781=CARTESIAN_POINT('',(41.8921035233278,93.,-73.966271890054));
#62782=CARTESIAN_POINT('',(44.5803698710478,93.,-75.0182022000314));
#62783=CARTESIAN_POINT('',(6.76187230188278,93.,-60.2196596729666));
#62784=CARTESIAN_POINT('',(45.0135046734565,93.,-77.8722743042845));
#62785=CARTESIAN_POINT('',(43.9449049906816,93.,-70.8309085949006));
#62786=CARTESIAN_POINT('',(42.7583731281452,93.,-79.6744160985602));
#62787=CARTESIAN_POINT('',(17.7244780890717,93.,-99.6797362392957));
#62788=CARTESIAN_POINT('',(40.0701067804252,93.,-78.6224857885828));
#62789=CARTESIAN_POINT('',(4.93987555898025,93.,-64.8758735714953));
#62790=CARTESIAN_POINT('',(39.6369719780164,93.,-75.7684136843297));
#62791=CARTESIAN_POINT('',(39.0015070976502,93.,-71.5811200791985));
#62792=CARTESIAN_POINT('',(14.603076938943,93.,-95.7737338250652));
#62793=CARTESIAN_POINT('',(-22.0921013332578,93.,-41.9542190213219));
#62794=CARTESIAN_POINT('',(-19.4038349855377,93.,-43.0061493312993));
#62795=CARTESIAN_POINT('',(9.12871549933204,93.,-54.1710603905964));
#62796=CARTESIAN_POINT('',(-18.970700183129,93.,-45.8602214355524));
#62797=CARTESIAN_POINT('',(-13.8500551204438,93.,-79.6018883436771));
#62798=CARTESIAN_POINT('',(-21.2258317284404,93.,-47.6623632298281));
#62799=CARTESIAN_POINT('',(-22.8237122821307,93.,-48.9392764697909));
#62800=CARTESIAN_POINT('',(-23.9140980761604,93.,-46.6104329198507));
#62801=CARTESIAN_POINT('',(7.30671875642946,93.,-58.8272742891252));
#62802=CARTESIAN_POINT('',(-24.3472328785691,93.,-43.7563608155976));
#62803=CARTESIAN_POINT('',(-18.7934530134749,93.,-80.3520998279754));
#62804=CARTESIAN_POINT('',(-25.9451134322595,93.,-45.0332740555604));
#62805=CARTESIAN_POINT('',(-29.0764221810509,93.,-39.221223906968));
#62806=CARTESIAN_POINT('',(-26.3881558333309,93.,-40.2731542169454));
#62807=CARTESIAN_POINT('',(9.12871549933204,93.,-54.1710603905964));
#62808=CARTESIAN_POINT('',(-25.9550210309222,93.,-43.1272263211986));
#62809=CARTESIAN_POINT('',(-20.2717173550133,93.,-80.5764416490967));
#62810=CARTESIAN_POINT('',(-28.2101525762335,93.,-44.9293681154742));
#62811=CARTESIAN_POINT('',(-26.878531319251,93.,-43.8652304928404));
#62812=CARTESIAN_POINT('',(-30.8984189239535,93.,-43.8774378054968));
#62813=CARTESIAN_POINT('',(7.30671875642946,93.,-58.8272742891252));
#62814=CARTESIAN_POINT('',(-31.3315537263622,93.,-41.0233657012437));
#62815=CARTESIAN_POINT('',(-25.2151152480443,93.,-81.3266531333951));
#62816=CARTESIAN_POINT('',(-29.9999324693798,93.,-39.95922807861));
#62817=CARTESIAN_POINT('',(-36.060743028844,93.,-36.4882287926142));
#62818=CARTESIAN_POINT('',(-33.372476681124,93.,-37.5401591025916));
#62819=CARTESIAN_POINT('',(9.12871549933205,93.,-54.1710603905964));
#62820=CARTESIAN_POINT('',(-32.9393418787153,93.,-40.3942312068447));
#62821=CARTESIAN_POINT('',(-26.6933795895828,93.,-81.5509949545164));
#62822=CARTESIAN_POINT('',(-35.1944734240266,93.,-42.1963730011203));
#62823=CARTESIAN_POINT('',(-30.9333503563712,93.,-38.7911845158899));
#62824=CARTESIAN_POINT('',(-37.8827397717466,93.,-41.1444426911429));
#62825=CARTESIAN_POINT('',(7.30671875642946,93.,-58.8272742891252));
#62826=CARTESIAN_POINT('',(-38.3158745741554,93.,-38.2903705868898));
#62827=CARTESIAN_POINT('',(-31.6367774826138,93.,-82.3012064388147));
#62828=CARTESIAN_POINT('',(-34.0547515065,93.,-34.8851821016595));
#62829=CARTESIAN_POINT('',(48.8764243711209,93.,-76.6992670044079));
#62830=CARTESIAN_POINT('',(51.5646907188409,93.,-77.7511973143853));
#62831=CARTESIAN_POINT('',(6.76187230188278,93.,-60.2196596729666));
#62832=CARTESIAN_POINT('',(51.9978255212496,93.,-80.6052694186384));
#62833=CARTESIAN_POINT('',(50.3665672252511,93.,-69.856355289481));
#62834=CARTESIAN_POINT('',(49.7426939759383,93.,-82.4074112129141));
#62835=CARTESIAN_POINT('',(21.779297126192,93.,-104.753782216246));
#62836=CARTESIAN_POINT('',(47.0544276282183,93.,-81.3554809029366));
#62837=CARTESIAN_POINT('',(4.93987555898025,93.,-64.8758735714953));
#62838=CARTESIAN_POINT('',(46.6212928258096,93.,-78.5014087986836));
#62839=CARTESIAN_POINT('',(45.4231693322196,93.,-70.6065667737789));
#62840=CARTESIAN_POINT('',(18.6578959760632,93.,-100.847779802016));
#62841=CARTESIAN_POINT('',(11.7041856792605,93.,-48.2040977535443));
#62842=CARTESIAN_POINT('',(14.3924520269805,93.,-49.2560280635217));
#62843=CARTESIAN_POINT('',(11.4955586967812,93.,-48.1224611082263));
#62844=CARTESIAN_POINT('',(14.8255868293893,93.,-52.1101001677748));
#62845=CARTESIAN_POINT('',(18.2582560524036,93.,-74.7291218165791));
#62846=CARTESIAN_POINT('',(12.5704552840779,93.,-53.9122419620505));
#62847=CARTESIAN_POINT('',(-6.60443613364975,93.,-69.2354603775928));
#62848=CARTESIAN_POINT('',(9.8821889363579,93.,-52.8603116520731));
#62849=CARTESIAN_POINT('',(9.67356195387869,93.,-52.7786750067551));
#62850=CARTESIAN_POINT('',(9.44905413394917,93.,-50.00623954782));
#62851=CARTESIAN_POINT('',(13.3148581593723,93.,-75.4793333008771));
#62852=CARTESIAN_POINT('',(-9.7258372837785,93.,-65.3294579633623));
#62853=CARTESIAN_POINT('',(18.6885065270537,93.,-50.9370928678982));
#62854=CARTESIAN_POINT('',(21.3767728747737,93.,-51.9890231778756));
#62855=CARTESIAN_POINT('',(11.4955586967812,93.,-48.1224611082263));
#62856=CARTESIAN_POINT('',(21.8099076771824,93.,-54.8430952821287));
#62857=CARTESIAN_POINT('',(24.679918286973,93.,-73.7545685111594));
#62858=CARTESIAN_POINT('',(19.5547761318711,93.,-56.6452370764044));
#62859=CARTESIAN_POINT('',(-2.5496170965295,93.,-74.3095063545433));
#62860=CARTESIAN_POINT('',(16.866509784151,93.,-55.593306766427));
#62861=CARTESIAN_POINT('',(9.6735619538787,93.,-52.7786750067551));
#62862=CARTESIAN_POINT('',(16.4333749817423,93.,-52.7392346621739));
#62863=CARTESIAN_POINT('',(19.7365203939418,93.,-74.5047799954575));
#62864=CARTESIAN_POINT('',(-5.67101824665825,93.,-70.4035039403128));
#62865=CARTESIAN_POINT('',(25.6728273748468,93.,-53.6700879822521));
#62866=CARTESIAN_POINT('',(28.3610937225668,93.,-54.7220182922295));
#62867=CARTESIAN_POINT('',(11.4955586967812,93.,-48.1224611082263));
#62868=CARTESIAN_POINT('',(28.7942285249755,93.,-57.5760903964826));
#62869=CARTESIAN_POINT('',(31.1015805215425,93.,-72.7800152057398));
#62870=CARTESIAN_POINT('',(26.5390969796642,93.,-59.3782321907583));
#62871=CARTESIAN_POINT('',(1.50520194059074,93.,-79.3835523314937));
#62872=CARTESIAN_POINT('',(23.8508306319442,93.,-58.3263018807808));
#62873=CARTESIAN_POINT('',(9.6735619538787,93.,-52.7786750067551));
#62874=CARTESIAN_POINT('',(23.4176958295354,93.,-55.4722297765278));
#62875=CARTESIAN_POINT('',(26.1581826285112,93.,-73.5302266900378));
#62876=CARTESIAN_POINT('',(-1.616199209538,93.,-75.4775499172633));
#62877=CARTESIAN_POINT('',(32.6571482226399,93.,-56.403083096606));
#62878=CARTESIAN_POINT('',(35.3454145703599,93.,-57.4550134065834));
#62879=CARTESIAN_POINT('',(11.4955586967812,93.,-48.1224611082264));
#62880=CARTESIAN_POINT('',(35.7785493727686,93.,-60.3090855108365));
#62881=CARTESIAN_POINT('',(37.523242756112,93.,-71.8054619003202));
#62882=CARTESIAN_POINT('',(33.5234178274573,93.,-62.1112273051122));
#62883=CARTESIAN_POINT('',(5.56002097771099,93.,-84.4575983084442));
#62884=CARTESIAN_POINT('',(30.8351514797373,93.,-61.0592969951347));
#62885=CARTESIAN_POINT('',(9.6735619538787,93.,-52.7786750067551));
#62886=CARTESIAN_POINT('',(30.4020166773286,93.,-58.2052248908817));
#62887=CARTESIAN_POINT('',(32.5798448630807,93.,-72.5556733846182));
#62888=CARTESIAN_POINT('',(2.43861982758225,93.,-80.5515958942137));
#62889=CARTESIAN_POINT('',(39.641469070433,93.,-59.1360782109599));
#62890=CARTESIAN_POINT('',(42.3297354181531,93.,-60.1880085209373));
#62891=CARTESIAN_POINT('',(11.4955586967812,93.,-48.1224611082264));
#62892=CARTESIAN_POINT('',(42.7628702205618,93.,-63.0420806251904));
#62893=CARTESIAN_POINT('',(43.9449049906815,93.,-70.8309085949006));
#62894=CARTESIAN_POINT('',(40.5077386752504,93.,-64.8442224194661));
#62895=CARTESIAN_POINT('',(9.61484001483123,93.,-89.5316442853947));
#62896=CARTESIAN_POINT('',(37.8194723275304,93.,-63.7922921094886));
#62897=CARTESIAN_POINT('',(9.6735619538787,93.,-52.7786750067551));
#62898=CARTESIAN_POINT('',(37.3863375251217,93.,-60.9382200052356));
#62899=CARTESIAN_POINT('',(39.0015070976501,93.,-71.5811200791985));
#62900=CARTESIAN_POINT('',(6.4934388647025,93.,-85.6256418711642));
#62901=CARTESIAN_POINT('',(46.6257899182262,93.,-61.8690733253138));
#62902=CARTESIAN_POINT('',(49.3140562659462,93.,-62.9210036352912));
#62903=CARTESIAN_POINT('',(11.4955586967812,93.,-48.1224611082264));
#62904=CARTESIAN_POINT('',(49.7471910683549,93.,-65.7750757395443));
#62905=CARTESIAN_POINT('',(50.366567225251,93.,-69.856355289481));
#62906=CARTESIAN_POINT('',(47.4920595230436,93.,-67.5772175338199));
#62907=CARTESIAN_POINT('',(13.6696590519515,93.,-94.6056902623451));
#62908=CARTESIAN_POINT('',(44.8037931753235,93.,-66.5252872238425));
#62909=CARTESIAN_POINT('',(9.6735619538787,93.,-52.7786750067551));
#62910=CARTESIAN_POINT('',(44.3706583729148,93.,-63.6712151195895));
#62911=CARTESIAN_POINT('',(45.4231693322196,93.,-70.6065667737789));
#62912=CARTESIAN_POINT('',(10.5482579018228,93.,-90.6996878481147));
#62913=CARTESIAN_POINT('',(-24.3427357861525,93.,-27.1240253422278));
#62914=CARTESIAN_POINT('',(-21.6544694384325,93.,-28.1759556522052));
#62915=CARTESIAN_POINT('',(13.8624018942305,93.,-42.0738618258562));
#62916=CARTESIAN_POINT('',(-21.2213346360238,93.,-31.0300277564583));
#62917=CARTESIAN_POINT('',(-13.8500551204439,93.,-79.6018883436771));
#62918=CARTESIAN_POINT('',(-23.4764661813351,93.,-32.832169550734));
#62919=CARTESIAN_POINT('',(-30.9333503563712,93.,-38.7911845158899));
#62920=CARTESIAN_POINT('',(-26.1647325290551,93.,-31.7802392407566));
#62921=CARTESIAN_POINT('',(12.0404051513279,93.,-46.730075724385));
#62922=CARTESIAN_POINT('',(-26.5978673314639,93.,-28.9261671365035));
#62923=CARTESIAN_POINT('',(-18.7934530134749,93.,-80.3520998279754));
#62924=CARTESIAN_POINT('',(-34.0547515065,93.,-34.8851821016595));
#62925=CARTESIAN_POINT('',(-17.3584149383594,93.,-29.8570204565817));
#62926=CARTESIAN_POINT('',(-14.6701485906394,93.,-30.9089507665591));
#62927=CARTESIAN_POINT('',(13.8624018942305,93.,-42.0738618258562));
#62928=CARTESIAN_POINT('',(-14.2370137882306,93.,-33.7630228708122));
#62929=CARTESIAN_POINT('',(-7.42839288587444,93.,-78.6273350382575));
#62930=CARTESIAN_POINT('',(-16.492145333542,93.,-35.5651646650879));
#62931=CARTESIAN_POINT('',(-26.878531319251,93.,-43.8652304928404));
#62932=CARTESIAN_POINT('',(-19.180411681262,93.,-34.5132343551105));
#62933=CARTESIAN_POINT('',(12.0404051513279,93.,-46.730075724385));
#62934=CARTESIAN_POINT('',(-19.6135464836707,93.,-31.6591622508574));
#62935=CARTESIAN_POINT('',(-12.3717907789055,93.,-79.3775465225558));
#62936=CARTESIAN_POINT('',(-29.9999324693798,93.,-39.95922807861));
#62937=CARTESIAN_POINT('',(40.7667862968804,93.,-66.5511750505069));
#62938=CARTESIAN_POINT('',(43.4550526446004,93.,-67.6031053604843));
#62939=CARTESIAN_POINT('',(9.12871549933199,93.,-54.1710603905965));
#62940=CARTESIAN_POINT('',(43.8881874470091,93.,-70.4571774647375));
#62941=CARTESIAN_POINT('',(43.9449049906816,93.,-70.8309085949006));
#62942=CARTESIAN_POINT('',(41.6330559016978,93.,-72.2593192590131));
#62943=CARTESIAN_POINT('',(13.6696590519515,93.,-94.6056902623452));
#62944=CARTESIAN_POINT('',(38.9447895539778,93.,-71.2073889490357));
#62945=CARTESIAN_POINT('',(7.30671875642947,93.,-58.8272742891252));
#62946=CARTESIAN_POINT('',(38.5116547515691,93.,-68.3533168447826));
#62947=CARTESIAN_POINT('',(39.0015070976502,93.,-71.5811200791985));
#62948=CARTESIAN_POINT('',(10.5482579018228,93.,-90.6996878481147));
#62949=CARTESIAN_POINT('',(47.7511071446736,93.,-69.2841701648608));
#62950=CARTESIAN_POINT('',(50.4393734923936,93.,-70.3361004748382));
#62951=CARTESIAN_POINT('',(9.12871549933199,93.,-54.1710603905965));
#62952=CARTESIAN_POINT('',(50.8725082948023,93.,-73.1901725790914));
#62953=CARTESIAN_POINT('',(50.366567225251,93.,-69.856355289481));
#62954=CARTESIAN_POINT('',(48.617376749491,93.,-74.992314373367));
#62955=CARTESIAN_POINT('',(17.7244780890717,93.,-99.6797362392957));
#62956=CARTESIAN_POINT('',(45.9291104017709,93.,-73.9403840633896));
#62957=CARTESIAN_POINT('',(7.30671875642947,93.,-58.8272742891252));
#62958=CARTESIAN_POINT('',(45.4959755993622,93.,-71.0863119591365));
#62959=CARTESIAN_POINT('',(45.4231693322196,93.,-70.6065667737789));
#62960=CARTESIAN_POINT('',(14.603076938943,93.,-95.7737338250652));
#62961=CARTESIAN_POINT('',(-30.2017394074983,93.,-31.806127067421));
#62962=CARTESIAN_POINT('',(-27.5134730597783,93.,-32.8580573773984));
#62963=CARTESIAN_POINT('',(11.4955586967813,93.,-48.1224611082263));
#62964=CARTESIAN_POINT('',(-27.0803382573695,93.,-35.7121294816515));
#62965=CARTESIAN_POINT('',(-20.2717173550133,93.,-80.5764416490967));
#62966=CARTESIAN_POINT('',(-29.3354698026809,93.,-37.5142712759272));
#62967=CARTESIAN_POINT('',(-30.9333503563712,93.,-38.7911845158899));
#62968=CARTESIAN_POINT('',(-32.0237361504009,93.,-36.4623409659497));
#62969=CARTESIAN_POINT('',(9.67356195387868,93.,-52.7786750067551));
#62970=CARTESIAN_POINT('',(-32.4568709528096,93.,-33.6082688616967));
#62971=CARTESIAN_POINT('',(-25.2151152480444,93.,-81.3266531333951));
#62972=CARTESIAN_POINT('',(-34.0547515065,93.,-34.8851821016595));
#62973=CARTESIAN_POINT('',(-23.2174185597051,93.,-34.5391221817749));
#62974=CARTESIAN_POINT('',(-20.5291522119851,93.,-35.5910524917523));
#62975=CARTESIAN_POINT('',(11.4955586967813,93.,-48.1224611082263));
#62976=CARTESIAN_POINT('',(-20.0960174095764,93.,-38.4451245960054));
#62977=CARTESIAN_POINT('',(-13.8500551204439,93.,-79.6018883436771));
#62978=CARTESIAN_POINT('',(-22.3511489548877,93.,-40.2472663902811));
#62979=CARTESIAN_POINT('',(-26.878531319251,93.,-43.8652304928404));
#62980=CARTESIAN_POINT('',(-25.0394153026078,93.,-39.1953360803036));
#62981=CARTESIAN_POINT('',(9.67356195387869,93.,-52.7786750067551));
#62982=CARTESIAN_POINT('',(-25.4725501050165,93.,-36.3412639760506));
#62983=CARTESIAN_POINT('',(-18.7934530134749,93.,-80.3520998279754));
#62984=CARTESIAN_POINT('',(-29.9999324693798,93.,-39.9592280786099));
#62985=CARTESIAN_POINT('',(-16.233097711912,93.,-37.2721172961288));
#62986=CARTESIAN_POINT('',(-13.544831364192,93.,-38.3240476061062));
#62987=CARTESIAN_POINT('',(11.4955586967812,93.,-48.1224611082263));
#62988=CARTESIAN_POINT('',(-13.1116965617833,93.,-41.1781197103593));
#62989=CARTESIAN_POINT('',(-7.42839288587437,93.,-78.6273350382575));
#62990=CARTESIAN_POINT('',(-15.3668281070946,93.,-42.9802615046349));
#62991=CARTESIAN_POINT('',(-22.8237122821307,93.,-48.9392764697909));
#62992=CARTESIAN_POINT('',(-18.0550944548146,93.,-41.9283311946575));
#62993=CARTESIAN_POINT('',(9.67356195387869,93.,-52.7786750067551));
#62994=CARTESIAN_POINT('',(-18.4882292572234,93.,-39.0742590904044));
#62995=CARTESIAN_POINT('',(-12.3717907789055,93.,-79.3775465225558));
#62996=CARTESIAN_POINT('',(-25.9451134322595,93.,-45.0332740555604));
#62997=CARTESIAN_POINT('',(-9.24877686411887,93.,-40.0051124104826));
#62998=CARTESIAN_POINT('',(-6.56051051639886,93.,-41.0570427204601));
#62999=CARTESIAN_POINT('',(11.4955586967812,93.,-48.1224611082263));
#63000=CARTESIAN_POINT('',(-6.12737571399014,93.,-43.9111148247132));
#63001=CARTESIAN_POINT('',(-1.00673065130489,93.,-77.6527817328379));
#63002=CARTESIAN_POINT('',(-8.38250725930147,93.,-45.7132566189888));
#63003=CARTESIAN_POINT('',(-18.7688932450105,93.,-54.0133224467414));
#63004=CARTESIAN_POINT('',(-11.0707736070215,93.,-44.6613263090114));
#63005=CARTESIAN_POINT('',(9.67356195387869,93.,-52.7786750067551));
#63006=CARTESIAN_POINT('',(-11.5039084094302,93.,-41.8072542047583));
#63007=CARTESIAN_POINT('',(-5.95012854433601,93.,-78.4029932171361));
#63008=CARTESIAN_POINT('',(-21.8902943951393,93.,-50.1073200325109));
#63009=CARTESIAN_POINT('',(-2.26445601632574,93.,-42.7381075248365));
#63010=CARTESIAN_POINT('',(0.423810331394273,93.,-43.7900378348139));
#63011=CARTESIAN_POINT('',(11.4955586967812,93.,-48.1224611082263));
#63012=CARTESIAN_POINT('',(0.856945133802991,93.,-46.6441099390671));
#63013=CARTESIAN_POINT('',(5.4149315832646,93.,-76.6782284274183));
#63014=CARTESIAN_POINT('',(-1.39818641150833,93.,-48.4462517333427));
#63015=CARTESIAN_POINT('',(-14.7140742078902,93.,-59.0873684236918));
#63016=CARTESIAN_POINT('',(-4.08645275922836,93.,-47.3943214233653));
#63017=CARTESIAN_POINT('',(9.67356195387869,93.,-52.7786750067551));
#63018=CARTESIAN_POINT('',(-4.51958756163709,93.,-44.5402493191122));
#63019=CARTESIAN_POINT('',(0.471533690233444,93.,-77.4284399117165));
#63020=CARTESIAN_POINT('',(-17.835475358019,93.,-55.1813660094614));
#63021=CARTESIAN_POINT('',(4.7198648314674,93.,-45.4711026391904));
#63022=CARTESIAN_POINT('',(7.40813117918741,93.,-46.5230329491678));
#63023=CARTESIAN_POINT('',(11.4955586967812,93.,-48.1224611082263));
#63024=CARTESIAN_POINT('',(7.84126598159612,93.,-49.3771050534209));
#63025=CARTESIAN_POINT('',(11.8365938178341,93.,-75.7036751219987));
#63026=CARTESIAN_POINT('',(5.5861344362848,93.,-51.1792468476966));
#63027=CARTESIAN_POINT('',(-10.65925517077,93.,-64.1614144006423));
#63028=CARTESIAN_POINT('',(2.89786808856477,93.,-50.1273165377192));
#63029=CARTESIAN_POINT('',(9.67356195387869,93.,-52.7786750067551));
#63030=CARTESIAN_POINT('',(2.46473328615604,93.,-47.2732444334661));
#63031=CARTESIAN_POINT('',(6.8931959248029,93.,-76.4538866062968));
#63032=CARTESIAN_POINT('',(-13.7806563208988,93.,-60.2554119864119));
#63033=CARTESIAN_POINT('',(-37.6508952335091,93.,-112.588303798924));
#63034=CARTESIAN_POINT('',(-34.9626288857891,93.,-113.640234108901));
#63035=CARTESIAN_POINT('',(-16.9065596726092,93.,-120.705652496668));
#63036=CARTESIAN_POINT('',(-34.5294940833804,93.,-116.494306213155));
#63037=CARTESIAN_POINT('',(-39.5367040587209,93.,-83.5001015653555));
#63038=CARTESIAN_POINT('',(-36.7846256286917,93.,-118.29644800743));
#63039=CARTESIAN_POINT('',(5.56002097771104,93.,-84.4575983084443));
#63040=CARTESIAN_POINT('',(-39.4728919764118,93.,-117.244517697453));
#63041=CARTESIAN_POINT('',(-18.728556415512,93.,-125.361866395196));
#63042=CARTESIAN_POINT('',(-39.9060267788205,93.,-114.3904455932));
#63043=CARTESIAN_POINT('',(-44.4801019517525,93.,-84.250313049654));
#63044=CARTESIAN_POINT('',(2.43861982758226,93.,-80.5515958942138));
#63045=CARTESIAN_POINT('',(-30.666574385716,93.,-115.321298913278));
#63046=CARTESIAN_POINT('',(-27.978308037996,93.,-116.373229223255));
#63047=CARTESIAN_POINT('',(-16.9065596726093,93.,-120.705652496668));
#63048=CARTESIAN_POINT('',(-27.5451732355873,93.,-119.227301327508));
#63049=CARTESIAN_POINT('',(-33.1150418241515,93.,-82.5255482599358));
#63050=CARTESIAN_POINT('',(-29.8003047808986,93.,-121.029443121784));
#63051=CARTESIAN_POINT('',(9.6148400148313,93.,-89.5316442853948));
#63052=CARTESIAN_POINT('',(-32.4885711286186,93.,-119.977512811807));
#63053=CARTESIAN_POINT('',(-18.728556415512,93.,-125.361866395196));
#63054=CARTESIAN_POINT('',(-32.9217059310274,93.,-117.123440707554));
#63055=CARTESIAN_POINT('',(-38.058439717183,93.,-83.2757597442344));
#63056=CARTESIAN_POINT('',(6.49343886470252,93.,-85.6256418711642));
#63057=CARTESIAN_POINT('Origin',(-27.978308037996,83.8,-116.373229223255));
#63058=CARTESIAN_POINT('',(-27.978308037996,83.8,-116.373229223255));
#63059=CARTESIAN_POINT('',(-27.5451732355873,83.8,-119.227301327508));
#63060=CARTESIAN_POINT('Origin',(-30.666574385716,83.8,-115.321298913278));
#63061=CARTESIAN_POINT('',(-30.666574385716,83.8,-115.321298913278));
#63062=CARTESIAN_POINT('Origin',(-32.9217059310274,83.8,-117.123440707554));
#63063=CARTESIAN_POINT('',(-32.9217059310274,83.8,-117.123440707554));
#63064=CARTESIAN_POINT('Origin',(-32.4885711286186,83.8,-119.977512811807));
#63065=CARTESIAN_POINT('',(-32.4885711286186,83.8,-119.977512811807));
#63066=CARTESIAN_POINT('Origin',(-29.8003047808986,83.8,-121.029443121784));
#63067=CARTESIAN_POINT('',(-29.8003047808986,83.8,-121.029443121784));
#63068=CARTESIAN_POINT('Origin',(-27.5451732355873,83.8,-119.227301327508));
#63069=CARTESIAN_POINT('Origin',(-34.9626288857891,83.8,-113.640234108901));
#63070=CARTESIAN_POINT('',(-34.9626288857891,83.8,-113.640234108901));
#63071=CARTESIAN_POINT('',(-34.5294940833804,83.8,-116.494306213155));
#63072=CARTESIAN_POINT('Origin',(-37.6508952335091,83.8,-112.588303798924));
#63073=CARTESIAN_POINT('',(-37.6508952335091,83.8,-112.588303798924));
#63074=CARTESIAN_POINT('Origin',(-39.9060267788205,83.8,-114.3904455932));
#63075=CARTESIAN_POINT('',(-39.9060267788205,83.8,-114.3904455932));
#63076=CARTESIAN_POINT('Origin',(-39.4728919764118,83.8,-117.244517697453));
#63077=CARTESIAN_POINT('',(-39.4728919764118,83.8,-117.244517697453));
#63078=CARTESIAN_POINT('Origin',(-36.7846256286917,83.8,-118.29644800743));
#63079=CARTESIAN_POINT('',(-36.7846256286917,83.8,-118.29644800743));
#63080=CARTESIAN_POINT('Origin',(-34.5294940833804,83.8,-116.494306213155));
#63081=CARTESIAN_POINT('Origin',(7.40813117918741,83.8,-46.5230329491678));
#63082=CARTESIAN_POINT('',(7.40813117918741,83.8,-46.5230329491678));
#63083=CARTESIAN_POINT('',(7.84126598159612,83.8,-49.3771050534209));
#63084=CARTESIAN_POINT('Origin',(4.7198648314674,83.8,-45.4711026391904));
#63085=CARTESIAN_POINT('',(4.7198648314674,83.8,-45.4711026391904));
#63086=CARTESIAN_POINT('Origin',(2.46473328615604,83.8,-47.2732444334661));
#63087=CARTESIAN_POINT('',(2.46473328615604,83.8,-47.2732444334661));
#63088=CARTESIAN_POINT('Origin',(2.89786808856477,83.8,-50.1273165377192));
#63089=CARTESIAN_POINT('',(2.89786808856477,83.8,-50.1273165377192));
#63090=CARTESIAN_POINT('Origin',(5.5861344362848,83.8,-51.1792468476966));
#63091=CARTESIAN_POINT('',(5.5861344362848,83.8,-51.1792468476966));
#63092=CARTESIAN_POINT('Origin',(7.84126598159612,83.8,-49.3771050534209));
#63093=CARTESIAN_POINT('Origin',(0.423810331394273,83.8,-43.7900378348139));
#63094=CARTESIAN_POINT('',(0.423810331394273,83.8,-43.7900378348139));
#63095=CARTESIAN_POINT('',(0.856945133802991,83.8,-46.6441099390671));
#63096=CARTESIAN_POINT('Origin',(-2.26445601632574,83.8,-42.7381075248365));
#63097=CARTESIAN_POINT('',(-2.26445601632574,83.8,-42.7381075248365));
#63098=CARTESIAN_POINT('Origin',(-4.51958756163709,83.8,-44.5402493191122));
#63099=CARTESIAN_POINT('',(-4.51958756163709,83.8,-44.5402493191122));
#63100=CARTESIAN_POINT('Origin',(-4.08645275922836,83.8,-47.3943214233653));
#63101=CARTESIAN_POINT('',(-4.08645275922836,83.8,-47.3943214233653));
#63102=CARTESIAN_POINT('Origin',(-1.39818641150833,83.8,-48.4462517333427));
#63103=CARTESIAN_POINT('',(-1.39818641150833,83.8,-48.4462517333427));
#63104=CARTESIAN_POINT('Origin',(0.856945133802991,83.8,-46.6441099390671));
#63105=CARTESIAN_POINT('Origin',(-6.56051051639886,83.8,-41.0570427204601));
#63106=CARTESIAN_POINT('',(-6.56051051639886,83.8,-41.0570427204601));
#63107=CARTESIAN_POINT('',(-6.12737571399014,83.8,-43.9111148247132));
#63108=CARTESIAN_POINT('Origin',(-9.24877686411887,83.8,-40.0051124104826));
#63109=CARTESIAN_POINT('',(-9.24877686411887,83.8,-40.0051124104826));
#63110=CARTESIAN_POINT('Origin',(-11.5039084094302,83.8,-41.8072542047583));
#63111=CARTESIAN_POINT('',(-11.5039084094302,83.8,-41.8072542047583));
#63112=CARTESIAN_POINT('Origin',(-11.0707736070215,83.8,-44.6613263090114));
#63113=CARTESIAN_POINT('',(-11.0707736070215,83.8,-44.6613263090114));
#63114=CARTESIAN_POINT('Origin',(-8.38250725930147,83.8,-45.7132566189888));
#63115=CARTESIAN_POINT('',(-8.38250725930147,83.8,-45.7132566189888));
#63116=CARTESIAN_POINT('Origin',(-6.12737571399014,83.8,-43.9111148247132));
#63117=CARTESIAN_POINT('Origin',(-13.544831364192,83.8,-38.3240476061062));
#63118=CARTESIAN_POINT('',(-13.544831364192,83.8,-38.3240476061062));
#63119=CARTESIAN_POINT('',(-13.1116965617833,83.8,-41.1781197103593));
#63120=CARTESIAN_POINT('Origin',(-16.233097711912,83.8,-37.2721172961288));
#63121=CARTESIAN_POINT('',(-16.233097711912,83.8,-37.2721172961288));
#63122=CARTESIAN_POINT('Origin',(-18.4882292572234,83.8,-39.0742590904044));
#63123=CARTESIAN_POINT('',(-18.4882292572234,83.8,-39.0742590904044));
#63124=CARTESIAN_POINT('Origin',(-18.0550944548146,83.8,-41.9283311946575));
#63125=CARTESIAN_POINT('',(-18.0550944548146,83.8,-41.9283311946575));
#63126=CARTESIAN_POINT('Origin',(-15.3668281070946,83.8,-42.9802615046349));
#63127=CARTESIAN_POINT('',(-15.3668281070946,83.8,-42.9802615046349));
#63128=CARTESIAN_POINT('Origin',(-13.1116965617833,83.8,-41.1781197103593));
#63129=CARTESIAN_POINT('Origin',(-20.5291522119851,83.8,-35.5910524917523));
#63130=CARTESIAN_POINT('',(-20.5291522119851,83.8,-35.5910524917523));
#63131=CARTESIAN_POINT('',(-20.0960174095764,83.8,-38.4451245960054));
#63132=CARTESIAN_POINT('Origin',(-23.2174185597051,83.8,-34.5391221817749));
#63133=CARTESIAN_POINT('',(-23.2174185597051,83.8,-34.5391221817749));
#63134=CARTESIAN_POINT('Origin',(-25.4725501050165,83.8,-36.3412639760506));
#63135=CARTESIAN_POINT('',(-25.4725501050165,83.8,-36.3412639760506));
#63136=CARTESIAN_POINT('Origin',(-25.0394153026078,83.8,-39.1953360803036));
#63137=CARTESIAN_POINT('',(-25.0394153026078,83.8,-39.1953360803036));
#63138=CARTESIAN_POINT('Origin',(-22.3511489548877,83.8,-40.2472663902811));
#63139=CARTESIAN_POINT('',(-22.3511489548877,83.8,-40.2472663902811));
#63140=CARTESIAN_POINT('Origin',(-20.0960174095764,83.8,-38.4451245960054));
#63141=CARTESIAN_POINT('Origin',(-27.5134730597783,83.8,-32.8580573773984));
#63142=CARTESIAN_POINT('',(-27.5134730597783,83.8,-32.8580573773984));
#63143=CARTESIAN_POINT('',(-27.0803382573695,83.8,-35.7121294816515));
#63144=CARTESIAN_POINT('Origin',(-30.2017394074983,83.8,-31.806127067421));
#63145=CARTESIAN_POINT('',(-30.2017394074983,83.8,-31.806127067421));
#63146=CARTESIAN_POINT('Origin',(-32.4568709528096,83.8,-33.6082688616967));
#63147=CARTESIAN_POINT('',(-32.4568709528096,83.8,-33.6082688616967));
#63148=CARTESIAN_POINT('Origin',(-32.0237361504009,83.8,-36.4623409659497));
#63149=CARTESIAN_POINT('',(-32.0237361504009,83.8,-36.4623409659497));
#63150=CARTESIAN_POINT('Origin',(-29.3354698026809,83.8,-37.5142712759272));
#63151=CARTESIAN_POINT('',(-29.3354698026809,83.8,-37.5142712759272));
#63152=CARTESIAN_POINT('Origin',(-27.0803382573695,83.8,-35.7121294816515));
#63153=CARTESIAN_POINT('Origin',(50.4393734923936,83.8,-70.3361004748382));
#63154=CARTESIAN_POINT('',(50.4393734923936,83.8,-70.3361004748382));
#63155=CARTESIAN_POINT('',(50.8725082948023,83.8,-73.1901725790914));
#63156=CARTESIAN_POINT('Origin',(47.7511071446736,83.8,-69.2841701648608));
#63157=CARTESIAN_POINT('',(47.7511071446736,83.8,-69.2841701648608));
#63158=CARTESIAN_POINT('Origin',(45.4959755993622,83.8,-71.0863119591365));
#63159=CARTESIAN_POINT('',(45.4959755993622,83.8,-71.0863119591365));
#63160=CARTESIAN_POINT('Origin',(45.9291104017709,83.8,-73.9403840633896));
#63161=CARTESIAN_POINT('',(45.9291104017709,83.8,-73.9403840633896));
#63162=CARTESIAN_POINT('Origin',(48.617376749491,83.8,-74.992314373367));
#63163=CARTESIAN_POINT('',(48.617376749491,83.8,-74.992314373367));
#63164=CARTESIAN_POINT('Origin',(50.8725082948023,83.8,-73.1901725790914));
#63165=CARTESIAN_POINT('Origin',(43.4550526446004,83.8,-67.6031053604843));
#63166=CARTESIAN_POINT('',(43.4550526446004,83.8,-67.6031053604843));
#63167=CARTESIAN_POINT('',(43.8881874470091,83.8,-70.4571774647375));
#63168=CARTESIAN_POINT('Origin',(40.7667862968804,83.8,-66.5511750505069));
#63169=CARTESIAN_POINT('',(40.7667862968804,83.8,-66.5511750505069));
#63170=CARTESIAN_POINT('Origin',(38.5116547515691,83.8,-68.3533168447826));
#63171=CARTESIAN_POINT('',(38.5116547515691,83.8,-68.3533168447826));
#63172=CARTESIAN_POINT('Origin',(38.9447895539778,83.8,-71.2073889490357));
#63173=CARTESIAN_POINT('',(38.9447895539778,83.8,-71.2073889490357));
#63174=CARTESIAN_POINT('Origin',(41.6330559016978,83.8,-72.2593192590131));
#63175=CARTESIAN_POINT('',(41.6330559016978,83.8,-72.2593192590131));
#63176=CARTESIAN_POINT('Origin',(43.8881874470091,83.8,-70.4571774647375));
#63177=CARTESIAN_POINT('Origin',(-14.6701485906394,83.8,-30.9089507665591));
#63178=CARTESIAN_POINT('',(-14.6701485906394,83.8,-30.9089507665591));
#63179=CARTESIAN_POINT('',(-14.2370137882306,83.8,-33.7630228708122));
#63180=CARTESIAN_POINT('Origin',(-17.3584149383594,83.8,-29.8570204565817));
#63181=CARTESIAN_POINT('',(-17.3584149383594,83.8,-29.8570204565817));
#63182=CARTESIAN_POINT('Origin',(-19.6135464836707,83.8,-31.6591622508574));
#63183=CARTESIAN_POINT('',(-19.6135464836707,83.8,-31.6591622508574));
#63184=CARTESIAN_POINT('Origin',(-19.180411681262,83.8,-34.5132343551105));
#63185=CARTESIAN_POINT('',(-19.180411681262,83.8,-34.5132343551105));
#63186=CARTESIAN_POINT('Origin',(-16.492145333542,83.8,-35.5651646650879));
#63187=CARTESIAN_POINT('',(-16.492145333542,83.8,-35.5651646650879));
#63188=CARTESIAN_POINT('Origin',(-14.2370137882306,83.8,-33.7630228708122));
#63189=CARTESIAN_POINT('Origin',(-21.6544694384325,83.8,-28.1759556522052));
#63190=CARTESIAN_POINT('',(-21.6544694384325,83.8,-28.1759556522052));
#63191=CARTESIAN_POINT('',(-21.2213346360238,83.8,-31.0300277564583));
#63192=CARTESIAN_POINT('Origin',(-24.3427357861525,83.8,-27.1240253422278));
#63193=CARTESIAN_POINT('',(-24.3427357861525,83.8,-27.1240253422278));
#63194=CARTESIAN_POINT('Origin',(-26.5978673314639,83.8,-28.9261671365035));
#63195=CARTESIAN_POINT('',(-26.5978673314639,83.8,-28.9261671365035));
#63196=CARTESIAN_POINT('Origin',(-26.1647325290551,83.8,-31.7802392407566));
#63197=CARTESIAN_POINT('',(-26.1647325290551,83.8,-31.7802392407566));
#63198=CARTESIAN_POINT('Origin',(-23.4764661813351,83.8,-32.832169550734));
#63199=CARTESIAN_POINT('',(-23.4764661813351,83.8,-32.832169550734));
#63200=CARTESIAN_POINT('Origin',(-21.2213346360238,83.8,-31.0300277564583));
#63201=CARTESIAN_POINT('Origin',(49.3140562659462,83.8,-62.9210036352912));
#63202=CARTESIAN_POINT('',(49.3140562659462,83.8,-62.9210036352912));
#63203=CARTESIAN_POINT('',(49.7471910683549,83.8,-65.7750757395443));
#63204=CARTESIAN_POINT('Origin',(46.6257899182262,83.8,-61.8690733253138));
#63205=CARTESIAN_POINT('',(46.6257899182262,83.8,-61.8690733253138));
#63206=CARTESIAN_POINT('Origin',(44.3706583729148,83.8,-63.6712151195895));
#63207=CARTESIAN_POINT('',(44.3706583729148,83.8,-63.6712151195895));
#63208=CARTESIAN_POINT('Origin',(44.8037931753235,83.8,-66.5252872238425));
#63209=CARTESIAN_POINT('',(44.8037931753235,83.8,-66.5252872238425));
#63210=CARTESIAN_POINT('Origin',(47.4920595230436,83.8,-67.5772175338199));
#63211=CARTESIAN_POINT('',(47.4920595230436,83.8,-67.5772175338199));
#63212=CARTESIAN_POINT('Origin',(49.7471910683549,83.8,-65.7750757395443));
#63213=CARTESIAN_POINT('Origin',(42.3297354181531,83.8,-60.1880085209373));
#63214=CARTESIAN_POINT('',(42.3297354181531,83.8,-60.1880085209373));
#63215=CARTESIAN_POINT('',(42.7628702205618,83.8,-63.0420806251904));
#63216=CARTESIAN_POINT('Origin',(39.641469070433,83.8,-59.1360782109599));
#63217=CARTESIAN_POINT('',(39.641469070433,83.8,-59.1360782109599));
#63218=CARTESIAN_POINT('Origin',(37.3863375251217,83.8,-60.9382200052356));
#63219=CARTESIAN_POINT('',(37.3863375251217,83.8,-60.9382200052356));
#63220=CARTESIAN_POINT('Origin',(37.8194723275304,83.8,-63.7922921094886));
#63221=CARTESIAN_POINT('',(37.8194723275304,83.8,-63.7922921094886));
#63222=CARTESIAN_POINT('Origin',(40.5077386752504,83.8,-64.844222419466));
#63223=CARTESIAN_POINT('',(40.5077386752504,83.8,-64.844222419466));
#63224=CARTESIAN_POINT('Origin',(42.7628702205618,83.8,-63.0420806251904));
#63225=CARTESIAN_POINT('Origin',(35.3454145703599,83.8,-57.4550134065834));
#63226=CARTESIAN_POINT('',(35.3454145703599,83.8,-57.4550134065834));
#63227=CARTESIAN_POINT('',(35.7785493727686,83.8,-60.3090855108365));
#63228=CARTESIAN_POINT('Origin',(32.6571482226399,83.8,-56.403083096606));
#63229=CARTESIAN_POINT('',(32.6571482226399,83.8,-56.403083096606));
#63230=CARTESIAN_POINT('Origin',(30.4020166773286,83.8,-58.2052248908817));
#63231=CARTESIAN_POINT('',(30.4020166773286,83.8,-58.2052248908817));
#63232=CARTESIAN_POINT('Origin',(30.8351514797373,83.8,-61.0592969951347));
#63233=CARTESIAN_POINT('',(30.8351514797373,83.8,-61.0592969951347));
#63234=CARTESIAN_POINT('Origin',(33.5234178274573,83.8,-62.1112273051122));
#63235=CARTESIAN_POINT('',(33.5234178274573,83.8,-62.1112273051122));
#63236=CARTESIAN_POINT('Origin',(35.7785493727686,83.8,-60.3090855108365));
#63237=CARTESIAN_POINT('Origin',(28.3610937225668,83.8,-54.7220182922295));
#63238=CARTESIAN_POINT('',(28.3610937225668,83.8,-54.7220182922295));
#63239=CARTESIAN_POINT('',(28.7942285249755,83.8,-57.5760903964826));
#63240=CARTESIAN_POINT('Origin',(25.6728273748468,83.8,-53.6700879822521));
#63241=CARTESIAN_POINT('',(25.6728273748468,83.8,-53.6700879822521));
#63242=CARTESIAN_POINT('Origin',(23.4176958295354,83.8,-55.4722297765278));
#63243=CARTESIAN_POINT('',(23.4176958295354,83.8,-55.4722297765278));
#63244=CARTESIAN_POINT('Origin',(23.8508306319442,83.8,-58.3263018807808));
#63245=CARTESIAN_POINT('',(23.8508306319442,83.8,-58.3263018807808));
#63246=CARTESIAN_POINT('Origin',(26.5390969796642,83.8,-59.3782321907583));
#63247=CARTESIAN_POINT('',(26.5390969796642,83.8,-59.3782321907583));
#63248=CARTESIAN_POINT('Origin',(28.7942285249755,83.8,-57.5760903964826));
#63249=CARTESIAN_POINT('Origin',(21.3767728747737,83.8,-51.9890231778756));
#63250=CARTESIAN_POINT('',(21.3767728747737,83.8,-51.9890231778756));
#63251=CARTESIAN_POINT('',(21.8099076771824,83.8,-54.8430952821287));
#63252=CARTESIAN_POINT('Origin',(18.6885065270537,83.8,-50.9370928678982));
#63253=CARTESIAN_POINT('',(18.6885065270537,83.8,-50.9370928678982));
#63254=CARTESIAN_POINT('Origin',(16.4333749817423,83.8,-52.7392346621739));
#63255=CARTESIAN_POINT('',(16.4333749817423,83.8,-52.7392346621739));
#63256=CARTESIAN_POINT('Origin',(16.866509784151,83.8,-55.593306766427));
#63257=CARTESIAN_POINT('',(16.866509784151,83.8,-55.593306766427));
#63258=CARTESIAN_POINT('Origin',(19.5547761318711,83.8,-56.6452370764044));
#63259=CARTESIAN_POINT('',(19.5547761318711,83.8,-56.6452370764044));
#63260=CARTESIAN_POINT('Origin',(21.8099076771824,83.8,-54.8430952821287));
#63261=CARTESIAN_POINT('Origin',(14.3924520269805,83.8,-49.2560280635217));
#63262=CARTESIAN_POINT('',(14.3924520269805,83.8,-49.2560280635217));
#63263=CARTESIAN_POINT('',(14.8255868293893,83.8,-52.1101001677748));
#63264=CARTESIAN_POINT('Origin',(11.7041856792605,83.8,-48.2040977535443));
#63265=CARTESIAN_POINT('',(11.7041856792605,83.8,-48.2040977535443));
#63266=CARTESIAN_POINT('Origin',(9.44905413394917,83.8,-50.00623954782));
#63267=CARTESIAN_POINT('',(9.44905413394917,83.8,-50.00623954782));
#63268=CARTESIAN_POINT('Origin',(9.8821889363579,83.8,-52.8603116520731));
#63269=CARTESIAN_POINT('',(9.8821889363579,83.8,-52.8603116520731));
#63270=CARTESIAN_POINT('Origin',(12.5704552840779,83.8,-53.9122419620505));
#63271=CARTESIAN_POINT('',(12.5704552840779,83.8,-53.9122419620505));
#63272=CARTESIAN_POINT('Origin',(14.8255868293893,83.8,-52.1101001677748));
#63273=CARTESIAN_POINT('Origin',(51.5646907188409,83.8,-77.7511973143853));
#63274=CARTESIAN_POINT('',(51.5646907188409,83.8,-77.7511973143853));
#63275=CARTESIAN_POINT('',(51.9978255212496,83.8,-80.6052694186384));
#63276=CARTESIAN_POINT('Origin',(48.8764243711209,83.8,-76.6992670044079));
#63277=CARTESIAN_POINT('',(48.8764243711209,83.8,-76.6992670044079));
#63278=CARTESIAN_POINT('Origin',(46.6212928258096,83.8,-78.5014087986836));
#63279=CARTESIAN_POINT('',(46.6212928258096,83.8,-78.5014087986836));
#63280=CARTESIAN_POINT('Origin',(47.0544276282183,83.8,-81.3554809029366));
#63281=CARTESIAN_POINT('',(47.0544276282183,83.8,-81.3554809029366));
#63282=CARTESIAN_POINT('Origin',(49.7426939759383,83.8,-82.4074112129141));
#63283=CARTESIAN_POINT('',(49.7426939759383,83.8,-82.4074112129141));
#63284=CARTESIAN_POINT('Origin',(51.9978255212496,83.8,-80.6052694186384));
#63285=CARTESIAN_POINT('Origin',(-33.372476681124,83.8,-37.5401591025916));
#63286=CARTESIAN_POINT('',(-33.372476681124,83.8,-37.5401591025916));
#63287=CARTESIAN_POINT('',(-32.9393418787153,83.8,-40.3942312068447));
#63288=CARTESIAN_POINT('Origin',(-36.060743028844,83.8,-36.4882287926142));
#63289=CARTESIAN_POINT('',(-36.060743028844,83.8,-36.4882287926142));
#63290=CARTESIAN_POINT('Origin',(-38.3158745741554,83.8,-38.2903705868898));
#63291=CARTESIAN_POINT('',(-38.3158745741554,83.8,-38.2903705868898));
#63292=CARTESIAN_POINT('Origin',(-37.8827397717466,83.8,-41.1444426911429));
#63293=CARTESIAN_POINT('',(-37.8827397717466,83.8,-41.1444426911429));
#63294=CARTESIAN_POINT('Origin',(-35.1944734240266,83.8,-42.1963730011203));
#63295=CARTESIAN_POINT('',(-35.1944734240266,83.8,-42.1963730011203));
#63296=CARTESIAN_POINT('Origin',(-32.9393418787153,83.8,-40.3942312068447));
#63297=CARTESIAN_POINT('Origin',(-26.3881558333309,83.8,-40.2731542169454));
#63298=CARTESIAN_POINT('',(-26.3881558333309,83.8,-40.2731542169454));
#63299=CARTESIAN_POINT('',(-25.9550210309222,83.8,-43.1272263211986));
#63300=CARTESIAN_POINT('Origin',(-29.0764221810509,83.8,-39.221223906968));
#63301=CARTESIAN_POINT('',(-29.0764221810509,83.8,-39.221223906968));
#63302=CARTESIAN_POINT('Origin',(-31.3315537263622,83.8,-41.0233657012437));
#63303=CARTESIAN_POINT('',(-31.3315537263622,83.8,-41.0233657012437));
#63304=CARTESIAN_POINT('Origin',(-30.8984189239535,83.8,-43.8774378054968));
#63305=CARTESIAN_POINT('',(-30.8984189239535,83.8,-43.8774378054968));
#63306=CARTESIAN_POINT('Origin',(-28.2101525762335,83.8,-44.9293681154742));
#63307=CARTESIAN_POINT('',(-28.2101525762335,83.8,-44.9293681154742));
#63308=CARTESIAN_POINT('Origin',(-25.9550210309222,83.8,-43.1272263211986));
#63309=CARTESIAN_POINT('Origin',(-19.4038349855377,83.8,-43.0061493312993));
#63310=CARTESIAN_POINT('',(-19.4038349855377,83.8,-43.0061493312993));
#63311=CARTESIAN_POINT('',(-18.970700183129,83.8,-45.8602214355524));
#63312=CARTESIAN_POINT('Origin',(-22.0921013332578,83.8,-41.9542190213219));
#63313=CARTESIAN_POINT('',(-22.0921013332578,83.8,-41.9542190213219));
#63314=CARTESIAN_POINT('Origin',(-24.3472328785691,83.8,-43.7563608155976));
#63315=CARTESIAN_POINT('',(-24.3472328785691,83.8,-43.7563608155976));
#63316=CARTESIAN_POINT('Origin',(-23.9140980761604,83.8,-46.6104329198507));
#63317=CARTESIAN_POINT('',(-23.9140980761604,83.8,-46.6104329198507));
#63318=CARTESIAN_POINT('Origin',(-21.2258317284404,83.8,-47.6623632298281));
#63319=CARTESIAN_POINT('',(-21.2258317284404,83.8,-47.6623632298281));
#63320=CARTESIAN_POINT('Origin',(-18.970700183129,83.8,-45.8602214355524));
#63321=CARTESIAN_POINT('Origin',(44.5803698710478,83.8,-75.0182022000314));
#63322=CARTESIAN_POINT('',(44.5803698710478,83.8,-75.0182022000314));
#63323=CARTESIAN_POINT('',(45.0135046734565,83.8,-77.8722743042845));
#63324=CARTESIAN_POINT('Origin',(41.8921035233278,83.8,-73.966271890054));
#63325=CARTESIAN_POINT('',(41.8921035233278,83.8,-73.966271890054));
#63326=CARTESIAN_POINT('Origin',(39.6369719780164,83.8,-75.7684136843297));
#63327=CARTESIAN_POINT('',(39.6369719780164,83.8,-75.7684136843297));
#63328=CARTESIAN_POINT('Origin',(40.0701067804252,83.8,-78.6224857885828));
#63329=CARTESIAN_POINT('',(40.0701067804252,83.8,-78.6224857885828));
#63330=CARTESIAN_POINT('Origin',(42.7583731281452,83.8,-79.6744160985602));
#63331=CARTESIAN_POINT('',(42.7583731281452,83.8,-79.6744160985602));
#63332=CARTESIAN_POINT('Origin',(45.0135046734565,83.8,-77.8722743042845));
#63333=CARTESIAN_POINT('Origin',(37.5960490232547,83.8,-72.2852070856775));
#63334=CARTESIAN_POINT('',(37.5960490232547,83.8,-72.2852070856775));
#63335=CARTESIAN_POINT('',(38.0291838256634,83.8,-75.1392791899306));
#63336=CARTESIAN_POINT('Origin',(34.9077826755347,83.8,-71.2332767757001));
#63337=CARTESIAN_POINT('',(34.9077826755347,83.8,-71.2332767757001));
#63338=CARTESIAN_POINT('Origin',(32.6526511302233,83.8,-73.0354185699758));
#63339=CARTESIAN_POINT('',(32.6526511302233,83.8,-73.0354185699758));
#63340=CARTESIAN_POINT('Origin',(33.085785932632,83.8,-75.8894906742289));
#63341=CARTESIAN_POINT('',(33.085785932632,83.8,-75.8894906742289));
#63342=CARTESIAN_POINT('Origin',(35.7740522803521,83.8,-76.9414209842063));
#63343=CARTESIAN_POINT('',(35.7740522803521,83.8,-76.9414209842063));
#63344=CARTESIAN_POINT('Origin',(38.0291838256634,83.8,-75.1392791899306));
#63345=CARTESIAN_POINT('Origin',(30.6117281754615,83.8,-69.5522119713236));
#63346=CARTESIAN_POINT('',(30.6117281754615,83.8,-69.5522119713236));
#63347=CARTESIAN_POINT('',(31.0448629778703,83.8,-72.4062840755767));
#63348=CARTESIAN_POINT('Origin',(27.9234618277415,83.8,-68.5002816613462));
#63349=CARTESIAN_POINT('',(27.9234618277415,83.8,-68.5002816613462));
#63350=CARTESIAN_POINT('Origin',(25.6683302824302,83.8,-70.3024234556219));
#63351=CARTESIAN_POINT('',(25.6683302824302,83.8,-70.3024234556219));
#63352=CARTESIAN_POINT('Origin',(26.1014650848389,83.8,-73.156495559875));
#63353=CARTESIAN_POINT('',(26.1014650848389,83.8,-73.156495559875));
#63354=CARTESIAN_POINT('Origin',(28.7897314325589,83.8,-74.2084258698524));
#63355=CARTESIAN_POINT('',(28.7897314325589,83.8,-74.2084258698524));
#63356=CARTESIAN_POINT('Origin',(31.0448629778703,83.8,-72.4062840755767));
#63357=CARTESIAN_POINT('Origin',(23.6274073276684,83.8,-66.8192168569697));
#63358=CARTESIAN_POINT('',(23.6274073276684,83.8,-66.8192168569697));
#63359=CARTESIAN_POINT('',(24.0605421300771,83.8,-69.6732889612228));
#63360=CARTESIAN_POINT('Origin',(20.9391409799484,83.8,-65.7672865469923));
#63361=CARTESIAN_POINT('',(20.9391409799484,83.8,-65.7672865469923));
#63362=CARTESIAN_POINT('Origin',(18.684009434637,83.8,-67.569428341268));
#63363=CARTESIAN_POINT('',(18.684009434637,83.8,-67.569428341268));
#63364=CARTESIAN_POINT('Origin',(19.1171442370458,83.8,-70.4235004455211));
#63365=CARTESIAN_POINT('',(19.1171442370458,83.8,-70.4235004455211));
#63366=CARTESIAN_POINT('Origin',(21.8054105847658,83.8,-71.4754307554985));
#63367=CARTESIAN_POINT('',(21.8054105847658,83.8,-71.4754307554985));
#63368=CARTESIAN_POINT('Origin',(24.0605421300771,83.8,-69.6732889612228));
#63369=CARTESIAN_POINT('Origin',(-12.4195141377446,83.8,-45.7391444456532));
#63370=CARTESIAN_POINT('',(-12.4195141377446,83.8,-45.7391444456532));
#63371=CARTESIAN_POINT('',(-11.9863793353359,83.8,-48.5932165499063));
#63372=CARTESIAN_POINT('Origin',(-15.1077804854646,83.8,-44.6872141356758));
#63373=CARTESIAN_POINT('',(-15.1077804854646,83.8,-44.6872141356758));
#63374=CARTESIAN_POINT('Origin',(-17.362912030776,83.8,-46.4893559299515));
#63375=CARTESIAN_POINT('',(-17.362912030776,83.8,-46.4893559299515));
#63376=CARTESIAN_POINT('Origin',(-16.9297772283673,83.8,-49.3434280342046));
#63377=CARTESIAN_POINT('',(-16.9297772283673,83.8,-49.3434280342046));
#63378=CARTESIAN_POINT('Origin',(-14.2415108806472,83.8,-50.395358344182));
#63379=CARTESIAN_POINT('',(-14.2415108806472,83.8,-50.395358344182));
#63380=CARTESIAN_POINT('Origin',(-11.9863793353359,83.8,-48.5932165499063));
#63381=CARTESIAN_POINT('Origin',(-5.43519328995148,83.8,-48.4721395600071));
#63382=CARTESIAN_POINT('',(-5.43519328995148,83.8,-48.4721395600071));
#63383=CARTESIAN_POINT('',(-5.00205848754277,83.8,-51.3262116642602));
#63384=CARTESIAN_POINT('Origin',(-8.12345963767149,83.8,-47.4202092500297));
#63385=CARTESIAN_POINT('',(-8.12345963767149,83.8,-47.4202092500297));
#63386=CARTESIAN_POINT('Origin',(-10.3785911829829,83.8,-49.2223510443054));
#63387=CARTESIAN_POINT('',(-10.3785911829829,83.8,-49.2223510443054));
#63388=CARTESIAN_POINT('Origin',(-9.94545638057412,83.8,-52.0764231485585));
#63389=CARTESIAN_POINT('',(-9.94545638057412,83.8,-52.0764231485585));
#63390=CARTESIAN_POINT('Origin',(-7.25719003285409,83.8,-53.1283534585359));
#63391=CARTESIAN_POINT('',(-7.25719003285409,83.8,-53.1283534585359));
#63392=CARTESIAN_POINT('Origin',(-5.00205848754277,83.8,-51.3262116642602));
#63393=CARTESIAN_POINT('Origin',(1.54912755784165,83.8,-51.205134674361));
#63394=CARTESIAN_POINT('',(1.54912755784165,83.8,-51.205134674361));
#63395=CARTESIAN_POINT('',(1.98226236025037,83.8,-54.0592067786141));
#63396=CARTESIAN_POINT('Origin',(-1.13913878987836,83.8,-50.1532043643836));
#63397=CARTESIAN_POINT('',(-1.13913878987836,83.8,-50.1532043643836));
#63398=CARTESIAN_POINT('Origin',(-3.39427033518972,83.8,-51.9553461586593));
#63399=CARTESIAN_POINT('',(-3.39427033518972,83.8,-51.9553461586593));
#63400=CARTESIAN_POINT('Origin',(-2.96113553278099,83.8,-54.8094182629124));
#63401=CARTESIAN_POINT('',(-2.96113553278099,83.8,-54.8094182629124));
#63402=CARTESIAN_POINT('Origin',(-0.272869185060958,83.8,-55.8613485728898));
#63403=CARTESIAN_POINT('',(-0.272869185060958,83.8,-55.8613485728898));
#63404=CARTESIAN_POINT('Origin',(1.98226236025037,83.8,-54.0592067786141));
#63405=CARTESIAN_POINT('Origin',(8.53344840563478,83.8,-53.9381297887149));
#63406=CARTESIAN_POINT('',(8.53344840563478,83.8,-53.9381297887149));
#63407=CARTESIAN_POINT('',(8.9665832080435,83.8,-56.792201892968));
#63408=CARTESIAN_POINT('Origin',(5.84518205791477,83.8,-52.8861994787375));
#63409=CARTESIAN_POINT('',(5.84518205791477,83.8,-52.8861994787375));
#63410=CARTESIAN_POINT('Origin',(3.59005051260342,83.8,-54.6883412730132));
#63411=CARTESIAN_POINT('',(3.59005051260342,83.8,-54.6883412730132));
#63412=CARTESIAN_POINT('Origin',(4.02318531501215,83.8,-57.5424133772663));
#63413=CARTESIAN_POINT('',(4.02318531501215,83.8,-57.5424133772663));
#63414=CARTESIAN_POINT('Origin',(6.71145166273218,83.8,-58.5943436872437));
#63415=CARTESIAN_POINT('',(6.71145166273218,83.8,-58.5943436872437));
#63416=CARTESIAN_POINT('Origin',(8.9665832080435,83.8,-56.792201892968));
#63417=CARTESIAN_POINT('Origin',(15.5177692534279,83.8,-56.6711249030688));
#63418=CARTESIAN_POINT('',(15.5177692534279,83.8,-56.6711249030688));
#63419=CARTESIAN_POINT('',(15.9509040558366,83.8,-59.5251970073219));
#63420=CARTESIAN_POINT('Origin',(12.8295029057079,83.8,-55.6191945930914));
#63421=CARTESIAN_POINT('',(12.8295029057079,83.8,-55.6191945930914));
#63422=CARTESIAN_POINT('Origin',(10.5743713603965,83.8,-57.4213363873671));
#63423=CARTESIAN_POINT('',(10.5743713603965,83.8,-57.4213363873671));
#63424=CARTESIAN_POINT('Origin',(11.0075061628053,83.8,-60.2754084916201));
#63425=CARTESIAN_POINT('',(11.0075061628053,83.8,-60.2754084916201));
#63426=CARTESIAN_POINT('Origin',(13.6957725105253,83.8,-61.3273388015976));
#63427=CARTESIAN_POINT('',(13.6957725105253,83.8,-61.3273388015976));
#63428=CARTESIAN_POINT('Origin',(15.9509040558366,83.8,-59.5251970073219));
#63429=CARTESIAN_POINT('Origin',(22.502090101221,83.8,-59.4041200174227));
#63430=CARTESIAN_POINT('',(22.502090101221,83.8,-59.4041200174227));
#63431=CARTESIAN_POINT('',(22.9352249036298,83.8,-62.2581921216758));
#63432=CARTESIAN_POINT('Origin',(19.813823753501,83.8,-58.3521897074453));
#63433=CARTESIAN_POINT('',(19.813823753501,83.8,-58.3521897074453));
#63434=CARTESIAN_POINT('Origin',(17.5586922081897,83.8,-60.154331501721));
#63435=CARTESIAN_POINT('',(17.5586922081897,83.8,-60.154331501721));
#63436=CARTESIAN_POINT('Origin',(17.9918270105984,83.8,-63.008403605974));
#63437=CARTESIAN_POINT('',(17.9918270105984,83.8,-63.008403605974));
#63438=CARTESIAN_POINT('Origin',(20.6800933583184,83.8,-64.0603339159514));
#63439=CARTESIAN_POINT('',(20.6800933583184,83.8,-64.0603339159514));
#63440=CARTESIAN_POINT('Origin',(22.9352249036298,83.8,-62.2581921216758));
#63441=CARTESIAN_POINT('Origin',(29.4864109490142,83.8,-62.1371151317766));
#63442=CARTESIAN_POINT('',(29.4864109490142,83.8,-62.1371151317766));
#63443=CARTESIAN_POINT('',(29.9195457514229,83.8,-64.9911872360297));
#63444=CARTESIAN_POINT('Origin',(26.7981446012942,83.8,-61.0851848217992));
#63445=CARTESIAN_POINT('',(26.7981446012942,83.8,-61.0851848217992));
#63446=CARTESIAN_POINT('Origin',(24.5430130559828,83.8,-62.8873266160749));
#63447=CARTESIAN_POINT('',(24.5430130559828,83.8,-62.8873266160749));
#63448=CARTESIAN_POINT('Origin',(24.9761478583915,83.8,-65.7413987203279));
#63449=CARTESIAN_POINT('',(24.9761478583915,83.8,-65.7413987203279));
#63450=CARTESIAN_POINT('Origin',(27.6644142061116,83.8,-66.7933290303053));
#63451=CARTESIAN_POINT('',(27.6644142061116,83.8,-66.7933290303053));
#63452=CARTESIAN_POINT('Origin',(29.9195457514229,83.8,-64.9911872360297));
#63453=CARTESIAN_POINT('Origin',(36.4707317968073,83.8,-64.8701102461305));
#63454=CARTESIAN_POINT('',(36.4707317968073,83.8,-64.8701102461305));
#63455=CARTESIAN_POINT('',(36.903866599216,83.8,-67.7241823503836));
#63456=CARTESIAN_POINT('Origin',(33.7824654490873,83.8,-63.818179936153));
#63457=CARTESIAN_POINT('',(33.7824654490873,83.8,-63.818179936153));
#63458=CARTESIAN_POINT('Origin',(31.5273339037759,83.8,-65.6203217304287));
#63459=CARTESIAN_POINT('',(31.5273339037759,83.8,-65.6203217304287));
#63460=CARTESIAN_POINT('Origin',(31.9604687061847,83.8,-68.4743938346818));
#63461=CARTESIAN_POINT('',(31.9604687061847,83.8,-68.4743938346818));
#63462=CARTESIAN_POINT('Origin',(34.6487350539047,83.8,-69.5263241446592));
#63463=CARTESIAN_POINT('',(34.6487350539047,83.8,-69.5263241446592));
#63464=CARTESIAN_POINT('Origin',(36.903866599216,83.8,-67.7241823503836));
#63465=CARTESIAN_POINT('Origin',(40.0791009652583,83.8,-45.3578148418432));
#63466=CARTESIAN_POINT('',(40.0791009652583,83.8,-45.3578148418432));
#63467=CARTESIAN_POINT('',(40.512235767667,83.8,-48.2118869460963));
#63468=CARTESIAN_POINT('Origin',(37.3908346175383,83.8,-44.3058845318658));
#63469=CARTESIAN_POINT('',(37.3908346175383,83.8,-44.3058845318658));
#63470=CARTESIAN_POINT('Origin',(35.1357030722269,83.8,-46.1080263261415));
#63471=CARTESIAN_POINT('',(35.1357030722269,83.8,-46.1080263261415));
#63472=CARTESIAN_POINT('Origin',(35.5688378746357,83.8,-48.9620984303945));
#63473=CARTESIAN_POINT('',(35.5688378746357,83.8,-48.9620984303945));
#63474=CARTESIAN_POINT('Origin',(38.2571042223557,83.8,-50.014028740372));
#63475=CARTESIAN_POINT('',(38.2571042223557,83.8,-50.014028740372));
#63476=CARTESIAN_POINT('Origin',(40.512235767667,83.8,-48.2118869460963));
#63477=CARTESIAN_POINT('Origin',(47.0634218130514,83.8,-48.0908099561971));
#63478=CARTESIAN_POINT('',(47.0634218130514,83.8,-48.0908099561971));
#63479=CARTESIAN_POINT('',(47.4965566154602,83.8,-50.9448820604502));
#63480=CARTESIAN_POINT('Origin',(44.3751554653314,83.8,-47.0388796462197));
#63481=CARTESIAN_POINT('',(44.3751554653314,83.8,-47.0388796462197));
#63482=CARTESIAN_POINT('Origin',(42.1200239200201,83.8,-48.8410214404954));
#63483=CARTESIAN_POINT('',(42.1200239200201,83.8,-48.8410214404954));
#63484=CARTESIAN_POINT('Origin',(42.5531587224288,83.8,-51.6950935447484));
#63485=CARTESIAN_POINT('',(42.5531587224288,83.8,-51.6950935447484));
#63486=CARTESIAN_POINT('Origin',(45.2414250701488,83.8,-52.7470238547258));
#63487=CARTESIAN_POINT('',(45.2414250701488,83.8,-52.7470238547258));
#63488=CARTESIAN_POINT('Origin',(47.4965566154602,83.8,-50.9448820604502));
#63489=CARTESIAN_POINT('Origin',(4.03217949984528,83.8,-24.2777424305267));
#63490=CARTESIAN_POINT('',(4.03217949984528,83.8,-24.2777424305267));
#63491=CARTESIAN_POINT('',(4.465314302254,83.8,-27.1318145347798));
#63492=CARTESIAN_POINT('Origin',(1.34391315212527,83.8,-23.2258121205493));
#63493=CARTESIAN_POINT('',(1.34391315212527,83.8,-23.2258121205493));
#63494=CARTESIAN_POINT('Origin',(-0.911218393186086,83.8,-25.0279539148249));
#63495=CARTESIAN_POINT('',(-0.911218393186086,83.8,-25.0279539148249));
#63496=CARTESIAN_POINT('Origin',(-0.478083590777355,83.8,-27.882026019078));
#63497=CARTESIAN_POINT('',(-0.478083590777355,83.8,-27.882026019078));
#63498=CARTESIAN_POINT('Origin',(2.21018275694267,83.8,-28.9339563290554));
#63499=CARTESIAN_POINT('',(2.21018275694267,83.8,-28.9339563290554));
#63500=CARTESIAN_POINT('Origin',(4.465314302254,83.8,-27.1318145347798));
#63501=CARTESIAN_POINT('Origin',(11.0165003476384,83.8,-27.0107375448806));
#63502=CARTESIAN_POINT('',(11.0165003476384,83.8,-27.0107375448806));
#63503=CARTESIAN_POINT('',(11.4496351500471,83.8,-29.8648096491337));
#63504=CARTESIAN_POINT('Origin',(8.3282339999184,83.8,-25.9588072349031));
#63505=CARTESIAN_POINT('',(8.3282339999184,83.8,-25.9588072349031));
#63506=CARTESIAN_POINT('Origin',(6.07310245460704,83.8,-27.7609490291788));
#63507=CARTESIAN_POINT('',(6.07310245460704,83.8,-27.7609490291788));
#63508=CARTESIAN_POINT('Origin',(6.50623725701577,83.8,-30.6150211334319));
#63509=CARTESIAN_POINT('',(6.50623725701577,83.8,-30.6150211334319));
#63510=CARTESIAN_POINT('Origin',(9.1945036047358,83.8,-31.6669514434093));
#63511=CARTESIAN_POINT('',(9.1945036047358,83.8,-31.6669514434093));
#63512=CARTESIAN_POINT('Origin',(11.4496351500471,83.8,-29.8648096491337));
#63513=CARTESIAN_POINT('Origin',(18.0008211954315,83.8,-29.7437326592344));
#63514=CARTESIAN_POINT('',(18.0008211954315,83.8,-29.7437326592344));
#63515=CARTESIAN_POINT('',(18.4339559978403,83.8,-32.5978047634875));
#63516=CARTESIAN_POINT('Origin',(15.3125548477115,83.8,-28.691802349257));
#63517=CARTESIAN_POINT('',(15.3125548477115,83.8,-28.691802349257));
#63518=CARTESIAN_POINT('Origin',(13.0574233024002,83.8,-30.4939441435327));
#63519=CARTESIAN_POINT('',(13.0574233024002,83.8,-30.4939441435327));
#63520=CARTESIAN_POINT('Origin',(13.4905581048089,83.8,-33.3480162477858));
#63521=CARTESIAN_POINT('',(13.4905581048089,83.8,-33.3480162477858));
#63522=CARTESIAN_POINT('Origin',(16.1788244525289,83.8,-34.3999465577632));
#63523=CARTESIAN_POINT('',(16.1788244525289,83.8,-34.3999465577632));
#63524=CARTESIAN_POINT('Origin',(18.4339559978403,83.8,-32.5978047634875));
#63525=CARTESIAN_POINT('Origin',(24.9851420432247,83.8,-32.4767277735883));
#63526=CARTESIAN_POINT('',(24.9851420432247,83.8,-32.4767277735883));
#63527=CARTESIAN_POINT('',(25.4182768456334,83.8,-35.3307998778414));
#63528=CARTESIAN_POINT('Origin',(22.2968756955047,83.8,-31.4247974636109));
#63529=CARTESIAN_POINT('',(22.2968756955047,83.8,-31.4247974636109));
#63530=CARTESIAN_POINT('Origin',(20.0417441501933,83.8,-33.2269392578866));
#63531=CARTESIAN_POINT('',(20.0417441501933,83.8,-33.2269392578866));
#63532=CARTESIAN_POINT('Origin',(20.474878952602,83.8,-36.0810113621397));
#63533=CARTESIAN_POINT('',(20.474878952602,83.8,-36.0810113621397));
#63534=CARTESIAN_POINT('Origin',(23.1631453003221,83.8,-37.1329416721171));
#63535=CARTESIAN_POINT('',(23.1631453003221,83.8,-37.1329416721171));
#63536=CARTESIAN_POINT('Origin',(25.4182768456334,83.8,-35.3307998778414));
#63537=CARTESIAN_POINT('Origin',(31.9694628910178,83.8,-35.2097228879422));
#63538=CARTESIAN_POINT('',(31.9694628910178,83.8,-35.2097228879422));
#63539=CARTESIAN_POINT('',(32.4025976934265,83.8,-38.0637949921953));
#63540=CARTESIAN_POINT('Origin',(29.2811965432978,83.8,-34.1577925779648));
#63541=CARTESIAN_POINT('',(29.2811965432978,83.8,-34.1577925779648));
#63542=CARTESIAN_POINT('Origin',(27.0260649979864,83.8,-35.9599343722405));
#63543=CARTESIAN_POINT('',(27.0260649979864,83.8,-35.9599343722405));
#63544=CARTESIAN_POINT('Origin',(27.4591998003952,83.8,-38.8140064764936));
#63545=CARTESIAN_POINT('',(27.4591998003952,83.8,-38.8140064764936));
#63546=CARTESIAN_POINT('Origin',(30.1474661481152,83.8,-39.865936786471));
#63547=CARTESIAN_POINT('',(30.1474661481152,83.8,-39.865936786471));
#63548=CARTESIAN_POINT('Origin',(32.4025976934265,83.8,-38.0637949921953));
#63549=CARTESIAN_POINT('Origin',(38.9537837388109,83.8,-37.9427180022961));
#63550=CARTESIAN_POINT('',(38.9537837388109,83.8,-37.9427180022961));
#63551=CARTESIAN_POINT('',(39.3869185412196,83.8,-40.7967901065492));
#63552=CARTESIAN_POINT('Origin',(36.2655173910909,83.8,-36.8907876923187));
#63553=CARTESIAN_POINT('',(36.2655173910909,83.8,-36.8907876923187));
#63554=CARTESIAN_POINT('Origin',(34.0103858457796,83.8,-38.6929294865944));
#63555=CARTESIAN_POINT('',(34.0103858457796,83.8,-38.6929294865944));
#63556=CARTESIAN_POINT('Origin',(34.4435206481883,83.8,-41.5470015908475));
#63557=CARTESIAN_POINT('',(34.4435206481883,83.8,-41.5470015908475));
#63558=CARTESIAN_POINT('Origin',(37.1317869959083,83.8,-42.5989319008249));
#63559=CARTESIAN_POINT('',(37.1317869959083,83.8,-42.5989319008249));
#63560=CARTESIAN_POINT('Origin',(39.3869185412196,83.8,-40.7967901065492));
#63561=CARTESIAN_POINT('Origin',(-7.68582774284623,83.8,-33.641945880913));
#63562=CARTESIAN_POINT('',(-7.68582774284623,83.8,-33.641945880913));
#63563=CARTESIAN_POINT('',(-7.25269294043752,83.8,-36.4960179851661));
#63564=CARTESIAN_POINT('Origin',(-10.3740940905662,83.8,-32.5900155709356));
#63565=CARTESIAN_POINT('',(-10.3740940905662,83.8,-32.5900155709356));
#63566=CARTESIAN_POINT('Origin',(-12.6292256358776,83.8,-34.3921573652113));
#63567=CARTESIAN_POINT('',(-12.6292256358776,83.8,-34.3921573652113));
#63568=CARTESIAN_POINT('Origin',(-12.1960908334689,83.8,-37.2462294694643));
#63569=CARTESIAN_POINT('',(-12.1960908334689,83.8,-37.2462294694643));
#63570=CARTESIAN_POINT('Origin',(-9.50782448574884,83.8,-38.2981597794418));
#63571=CARTESIAN_POINT('',(-9.50782448574884,83.8,-38.2981597794418));
#63572=CARTESIAN_POINT('Origin',(-7.25269294043752,83.8,-36.4960179851661));
#63573=CARTESIAN_POINT('Origin',(-0.701506895053102,83.8,-36.3749409952669));
#63574=CARTESIAN_POINT('',(-0.701506895053102,83.8,-36.3749409952669));
#63575=CARTESIAN_POINT('',(-0.268372092644385,83.8,-39.22901309952));
#63576=CARTESIAN_POINT('Origin',(-3.38977324277311,83.8,-35.3230106852895));
#63577=CARTESIAN_POINT('',(-3.38977324277311,83.8,-35.3230106852895));
#63578=CARTESIAN_POINT('Origin',(-5.64490478808447,83.8,-37.1251524795652));
#63579=CARTESIAN_POINT('',(-5.64490478808447,83.8,-37.1251524795652));
#63580=CARTESIAN_POINT('Origin',(-5.21176998567574,83.8,-39.9792245838182));
#63581=CARTESIAN_POINT('',(-5.21176998567574,83.8,-39.9792245838182));
#63582=CARTESIAN_POINT('Origin',(-2.52350363795571,83.8,-41.0311548937957));
#63583=CARTESIAN_POINT('',(-2.52350363795571,83.8,-41.0311548937957));
#63584=CARTESIAN_POINT('Origin',(-0.268372092644385,83.8,-39.22901309952));
#63585=CARTESIAN_POINT('Origin',(6.28281395274003,83.8,-39.1079361096208));
#63586=CARTESIAN_POINT('',(6.28281395274003,83.8,-39.1079361096208));
#63587=CARTESIAN_POINT('',(6.71594875514875,83.8,-41.9620082138739));
#63588=CARTESIAN_POINT('Origin',(3.59454760502002,83.8,-38.0560057996434));
#63589=CARTESIAN_POINT('',(3.59454760502002,83.8,-38.0560057996434));
#63590=CARTESIAN_POINT('Origin',(1.33941605970866,83.8,-39.8581475939191));
#63591=CARTESIAN_POINT('',(1.33941605970866,83.8,-39.8581475939191));
#63592=CARTESIAN_POINT('Origin',(1.7725508621174,83.8,-42.7122196981721));
#63593=CARTESIAN_POINT('',(1.7725508621174,83.8,-42.7122196981721));
#63594=CARTESIAN_POINT('Origin',(4.46081720983742,83.8,-43.7641500081495));
#63595=CARTESIAN_POINT('',(4.46081720983742,83.8,-43.7641500081495));
#63596=CARTESIAN_POINT('Origin',(6.71594875514875,83.8,-41.9620082138739));
#63597=CARTESIAN_POINT('Origin',(13.2671348005332,83.8,-41.8409312239747));
#63598=CARTESIAN_POINT('',(13.2671348005332,83.8,-41.8409312239747));
#63599=CARTESIAN_POINT('',(13.7002696029419,83.8,-44.6950033282278));
#63600=CARTESIAN_POINT('Origin',(10.5788684528132,83.8,-40.7890009139973));
#63601=CARTESIAN_POINT('',(10.5788684528132,83.8,-40.7890009139973));
#63602=CARTESIAN_POINT('Origin',(8.32373690750179,83.8,-42.591142708273));
#63603=CARTESIAN_POINT('',(8.32373690750179,83.8,-42.591142708273));
#63604=CARTESIAN_POINT('Origin',(8.75687170991053,83.8,-45.445214812526));
#63605=CARTESIAN_POINT('',(8.75687170991053,83.8,-45.445214812526));
#63606=CARTESIAN_POINT('Origin',(11.4451380576306,83.8,-46.4971451225034));
#63607=CARTESIAN_POINT('',(11.4451380576306,83.8,-46.4971451225034));
#63608=CARTESIAN_POINT('Origin',(13.7002696029419,83.8,-44.6950033282278));
#63609=CARTESIAN_POINT('Origin',(20.2514556483263,83.8,-44.5739263383286));
#63610=CARTESIAN_POINT('',(20.2514556483263,83.8,-44.5739263383286));
#63611=CARTESIAN_POINT('',(20.684590450735,83.8,-47.4279984425817));
#63612=CARTESIAN_POINT('Origin',(17.5631893006063,83.8,-43.5219960283511));
#63613=CARTESIAN_POINT('',(17.5631893006063,83.8,-43.5219960283511));
#63614=CARTESIAN_POINT('Origin',(15.3080577552949,83.8,-45.3241378226269));
#63615=CARTESIAN_POINT('',(15.3080577552949,83.8,-45.3241378226269));
#63616=CARTESIAN_POINT('Origin',(15.7411925577037,83.8,-48.1782099268799));
#63617=CARTESIAN_POINT('',(15.7411925577037,83.8,-48.1782099268799));
#63618=CARTESIAN_POINT('Origin',(18.4294589054237,83.8,-49.2301402368573));
#63619=CARTESIAN_POINT('',(18.4294589054237,83.8,-49.2301402368573));
#63620=CARTESIAN_POINT('Origin',(20.684590450735,83.8,-47.4279984425817));
#63621=CARTESIAN_POINT('Origin',(27.2357764961194,83.8,-47.3069214526824));
#63622=CARTESIAN_POINT('',(27.2357764961194,83.8,-47.3069214526824));
#63623=CARTESIAN_POINT('',(27.6689112985281,83.8,-50.1609935569356));
#63624=CARTESIAN_POINT('Origin',(24.5475101483994,83.8,-46.254991142705));
#63625=CARTESIAN_POINT('',(24.5475101483994,83.8,-46.254991142705));
#63626=CARTESIAN_POINT('Origin',(22.2923786030881,83.8,-48.0571329369807));
#63627=CARTESIAN_POINT('',(22.2923786030881,83.8,-48.0571329369807));
#63628=CARTESIAN_POINT('Origin',(22.7255134054968,83.8,-50.9112050412338));
#63629=CARTESIAN_POINT('',(22.7255134054968,83.8,-50.9112050412338));
#63630=CARTESIAN_POINT('Origin',(25.4137797532168,83.8,-51.9631353512112));
#63631=CARTESIAN_POINT('',(25.4137797532168,83.8,-51.9631353512112));
#63632=CARTESIAN_POINT('Origin',(27.6689112985281,83.8,-50.1609935569356));
#63633=CARTESIAN_POINT('Origin',(34.2200973439125,83.8,-50.0399165670363));
#63634=CARTESIAN_POINT('',(34.2200973439125,83.8,-50.0399165670363));
#63635=CARTESIAN_POINT('',(34.6532321463213,83.8,-52.8939886712894));
#63636=CARTESIAN_POINT('Origin',(31.5318309961925,83.8,-48.9879862570589));
#63637=CARTESIAN_POINT('',(31.5318309961925,83.8,-48.9879862570589));
#63638=CARTESIAN_POINT('Origin',(29.2766994508812,83.8,-50.7901280513346));
#63639=CARTESIAN_POINT('',(29.2766994508812,83.8,-50.7901280513346));
#63640=CARTESIAN_POINT('Origin',(29.7098342532899,83.8,-53.6442001555877));
#63641=CARTESIAN_POINT('',(29.7098342532899,83.8,-53.6442001555877));
#63642=CARTESIAN_POINT('Origin',(32.3981006010099,83.8,-54.6961304655651));
#63643=CARTESIAN_POINT('',(32.3981006010099,83.8,-54.6961304655651));
#63644=CARTESIAN_POINT('Origin',(34.6532321463213,83.8,-52.8939886712894));
#63645=CARTESIAN_POINT('Origin',(41.2044181917057,83.8,-52.7729116813902));
#63646=CARTESIAN_POINT('',(41.2044181917057,83.8,-52.7729116813902));
#63647=CARTESIAN_POINT('',(41.6375529941144,83.8,-55.6269837856433));
#63648=CARTESIAN_POINT('Origin',(38.5161518439857,83.8,-51.7209813714128));
#63649=CARTESIAN_POINT('',(38.5161518439857,83.8,-51.7209813714128));
#63650=CARTESIAN_POINT('Origin',(36.2610202986743,83.8,-53.5231231656885));
#63651=CARTESIAN_POINT('',(36.2610202986743,83.8,-53.5231231656885));
#63652=CARTESIAN_POINT('Origin',(36.694155101083,83.8,-56.3771952699416));
#63653=CARTESIAN_POINT('',(36.694155101083,83.8,-56.3771952699416));
#63654=CARTESIAN_POINT('Origin',(39.3824214488031,83.8,-57.429125579919));
#63655=CARTESIAN_POINT('',(39.3824214488031,83.8,-57.429125579919));
#63656=CARTESIAN_POINT('Origin',(41.6375529941144,83.8,-55.6269837856433));
#63657=CARTESIAN_POINT('Origin',(33.0947801174652,83.8,-42.6248197274893));
#63658=CARTESIAN_POINT('',(33.0947801174652,83.8,-42.6248197274893));
#63659=CARTESIAN_POINT('',(33.5279149198739,83.8,-45.4788918317424));
#63660=CARTESIAN_POINT('Origin',(30.4065137697452,83.8,-41.5728894175119));
#63661=CARTESIAN_POINT('',(30.4065137697452,83.8,-41.5728894175119));
#63662=CARTESIAN_POINT('Origin',(28.1513822244338,83.8,-43.3750312117876));
#63663=CARTESIAN_POINT('',(28.1513822244338,83.8,-43.3750312117876));
#63664=CARTESIAN_POINT('Origin',(28.5845170268425,83.8,-46.2291033160406));
#63665=CARTESIAN_POINT('',(28.5845170268425,83.8,-46.2291033160406));
#63666=CARTESIAN_POINT('Origin',(31.2727833745626,83.8,-47.2810336260181));
#63667=CARTESIAN_POINT('',(31.2727833745626,83.8,-47.2810336260181));
#63668=CARTESIAN_POINT('Origin',(33.5279149198739,83.8,-45.4788918317424));
#63669=CARTESIAN_POINT('Origin',(26.110459269672,83.8,-39.8918246131354));
#63670=CARTESIAN_POINT('',(26.110459269672,83.8,-39.8918246131354));
#63671=CARTESIAN_POINT('',(26.5435940720808,83.8,-42.7458967173885));
#63672=CARTESIAN_POINT('Origin',(23.422192921952,83.8,-38.839894303158));
#63673=CARTESIAN_POINT('',(23.422192921952,83.8,-38.839894303158));
#63674=CARTESIAN_POINT('Origin',(21.1670613766407,83.8,-40.6420360974337));
#63675=CARTESIAN_POINT('',(21.1670613766407,83.8,-40.6420360974337));
#63676=CARTESIAN_POINT('Origin',(21.6001961790494,83.8,-43.4961082016867));
#63677=CARTESIAN_POINT('',(21.6001961790494,83.8,-43.4961082016867));
#63678=CARTESIAN_POINT('Origin',(24.2884625267694,83.8,-44.5480385116642));
#63679=CARTESIAN_POINT('',(24.2884625267694,83.8,-44.5480385116642));
#63680=CARTESIAN_POINT('Origin',(26.5435940720808,83.8,-42.7458967173885));
#63681=CARTESIAN_POINT('Origin',(19.1261384218789,83.8,-37.1588294987815));
#63682=CARTESIAN_POINT('',(19.1261384218789,83.8,-37.1588294987815));
#63683=CARTESIAN_POINT('',(19.5592732242876,83.8,-40.0129016030346));
#63684=CARTESIAN_POINT('Origin',(16.4378720741589,83.8,-36.1068991888041));
#63685=CARTESIAN_POINT('',(16.4378720741589,83.8,-36.1068991888041));
#63686=CARTESIAN_POINT('Origin',(14.1827405288475,83.8,-37.9090409830798));
#63687=CARTESIAN_POINT('',(14.1827405288475,83.8,-37.9090409830798));
#63688=CARTESIAN_POINT('Origin',(14.6158753312563,83.8,-40.7631130873329));
#63689=CARTESIAN_POINT('',(14.6158753312563,83.8,-40.7631130873329));
#63690=CARTESIAN_POINT('Origin',(17.3041416789763,83.8,-41.8150433973103));
#63691=CARTESIAN_POINT('',(17.3041416789763,83.8,-41.8150433973103));
#63692=CARTESIAN_POINT('Origin',(19.5592732242876,83.8,-40.0129016030346));
#63693=CARTESIAN_POINT('Origin',(12.1418175740858,83.8,-34.4258343844276));
#63694=CARTESIAN_POINT('',(12.1418175740858,83.8,-34.4258343844276));
#63695=CARTESIAN_POINT('',(12.5749523764945,83.8,-37.2799064886807));
#63696=CARTESIAN_POINT('Origin',(9.45355122636578,83.8,-33.3739040744502));
#63697=CARTESIAN_POINT('',(9.45355122636578,83.8,-33.3739040744502));
#63698=CARTESIAN_POINT('Origin',(7.19841968105442,83.8,-35.1760458687259));
#63699=CARTESIAN_POINT('',(7.19841968105442,83.8,-35.1760458687259));
#63700=CARTESIAN_POINT('Origin',(7.63155448346315,83.8,-38.030117972979));
#63701=CARTESIAN_POINT('',(7.63155448346315,83.8,-38.030117972979));
#63702=CARTESIAN_POINT('Origin',(10.3198208311832,83.8,-39.0820482829564));
#63703=CARTESIAN_POINT('',(10.3198208311832,83.8,-39.0820482829564));
#63704=CARTESIAN_POINT('Origin',(12.5749523764945,83.8,-37.2799064886807));
#63705=CARTESIAN_POINT('Origin',(48.1887390394988,83.8,-55.5059067957441));
#63706=CARTESIAN_POINT('',(48.1887390394988,83.8,-55.5059067957441));
#63707=CARTESIAN_POINT('',(48.6218738419075,83.8,-58.3599788999972));
#63708=CARTESIAN_POINT('Origin',(45.5004726917788,83.8,-54.4539764857667));
#63709=CARTESIAN_POINT('',(45.5004726917788,83.8,-54.4539764857667));
#63710=CARTESIAN_POINT('Origin',(43.2453411464674,83.8,-56.2561182800424));
#63711=CARTESIAN_POINT('',(43.2453411464674,83.8,-56.2561182800424));
#63712=CARTESIAN_POINT('Origin',(43.6784759488762,83.8,-59.1101903842955));
#63713=CARTESIAN_POINT('',(43.6784759488762,83.8,-59.1101903842955));
#63714=CARTESIAN_POINT('Origin',(46.3667422965962,83.8,-60.1621206942729));
#63715=CARTESIAN_POINT('',(46.3667422965962,83.8,-60.1621206942729));
#63716=CARTESIAN_POINT('Origin',(48.6218738419075,83.8,-58.3599788999972));
#63717=CARTESIAN_POINT('Origin',(-8.81114496929361,83.8,-26.2268490413659));
#63718=CARTESIAN_POINT('',(-8.81114496929361,83.8,-26.2268490413659));
#63719=CARTESIAN_POINT('',(-8.37801016688489,83.8,-29.080921145619));
#63720=CARTESIAN_POINT('Origin',(-11.4994113170136,83.8,-25.1749187313885));
#63721=CARTESIAN_POINT('',(-11.4994113170136,83.8,-25.1749187313885));
#63722=CARTESIAN_POINT('Origin',(-13.754542862325,83.8,-26.9770605256642));
#63723=CARTESIAN_POINT('',(-13.754542862325,83.8,-26.9770605256642));
#63724=CARTESIAN_POINT('Origin',(-13.3214080599162,83.8,-29.8311326299173));
#63725=CARTESIAN_POINT('',(-13.3214080599162,83.8,-29.8311326299173));
#63726=CARTESIAN_POINT('Origin',(-10.6331417121962,83.8,-30.8830629398947));
#63727=CARTESIAN_POINT('',(-10.6331417121962,83.8,-30.8830629398947));
#63728=CARTESIAN_POINT('Origin',(-8.37801016688489,83.8,-29.080921145619));
#63729=CARTESIAN_POINT('Origin',(-1.82682412150048,83.8,-28.9598441557198));
#63730=CARTESIAN_POINT('',(-1.82682412150048,83.8,-28.9598441557198));
#63731=CARTESIAN_POINT('',(-1.39368931909176,83.8,-31.8139162599729));
#63732=CARTESIAN_POINT('Origin',(-4.51509046922049,83.8,-27.9079138457424));
#63733=CARTESIAN_POINT('',(-4.51509046922049,83.8,-27.9079138457424));
#63734=CARTESIAN_POINT('Origin',(-6.77022201453184,83.8,-29.7100556400181));
#63735=CARTESIAN_POINT('',(-6.77022201453184,83.8,-29.7100556400181));
#63736=CARTESIAN_POINT('Origin',(-6.33708721212311,83.8,-32.5641277442712));
#63737=CARTESIAN_POINT('',(-6.33708721212311,83.8,-32.5641277442712));
#63738=CARTESIAN_POINT('Origin',(-3.64882086440308,83.8,-33.6160580542486));
#63739=CARTESIAN_POINT('',(-3.64882086440308,83.8,-33.6160580542486));
#63740=CARTESIAN_POINT('Origin',(-1.39368931909176,83.8,-31.8139162599729));
#63741=CARTESIAN_POINT('Origin',(5.15749672629266,83.8,-31.6928392700737));
#63742=CARTESIAN_POINT('',(5.15749672629266,83.8,-31.6928392700737));
#63743=CARTESIAN_POINT('',(5.59063152870137,83.8,-34.5469113743268));
#63744=CARTESIAN_POINT('Origin',(2.46923037857264,83.8,-30.6409089600963));
#63745=CARTESIAN_POINT('',(2.46923037857264,83.8,-30.6409089600963));
#63746=CARTESIAN_POINT('Origin',(0.214098833261289,83.8,-32.443050754372));
#63747=CARTESIAN_POINT('',(0.214098833261289,83.8,-32.443050754372));
#63748=CARTESIAN_POINT('Origin',(0.647233635670021,83.8,-35.2971228586251));
#63749=CARTESIAN_POINT('',(0.647233635670021,83.8,-35.2971228586251));
#63750=CARTESIAN_POINT('Origin',(3.33549998339005,83.8,-36.3490531686025));
#63751=CARTESIAN_POINT('',(3.33549998339005,83.8,-36.3490531686025));
#63752=CARTESIAN_POINT('Origin',(5.59063152870137,83.8,-34.5469113743268));
#63753=CARTESIAN_POINT('Origin',(30.3793106863527,83.8,-111.309797894252));
#63754=CARTESIAN_POINT('',(30.3793106863527,83.8,-111.309797894252));
#63755=CARTESIAN_POINT('',(30.8124454887614,83.8,-114.163869998505));
#63756=CARTESIAN_POINT('Origin',(27.6910443386327,83.8,-110.257867584275));
#63757=CARTESIAN_POINT('',(27.6910443386327,83.8,-110.257867584275));
#63758=CARTESIAN_POINT('Origin',(25.4359127933213,83.8,-112.06000937855));
#63759=CARTESIAN_POINT('',(25.4359127933213,83.8,-112.06000937855));
#63760=CARTESIAN_POINT('Origin',(25.86904759573,83.8,-114.914081482803));
#63761=CARTESIAN_POINT('',(25.86904759573,83.8,-114.914081482803));
#63762=CARTESIAN_POINT('Origin',(28.5573139434501,83.8,-115.966011792781));
#63763=CARTESIAN_POINT('',(28.5573139434501,83.8,-115.966011792781));
#63764=CARTESIAN_POINT('Origin',(30.8124454887614,83.8,-114.163869998505));
#63765=CARTESIAN_POINT('Origin',(23.3949898385595,83.8,-108.576802779898));
#63766=CARTESIAN_POINT('',(23.3949898385595,83.8,-108.576802779898));
#63767=CARTESIAN_POINT('',(23.8281246409682,83.8,-111.430874884151));
#63768=CARTESIAN_POINT('Origin',(20.7067234908395,83.8,-107.524872469921));
#63769=CARTESIAN_POINT('',(20.7067234908395,83.8,-107.524872469921));
#63770=CARTESIAN_POINT('Origin',(18.4515919455282,83.8,-109.327014264196));
#63771=CARTESIAN_POINT('',(18.4515919455282,83.8,-109.327014264196));
#63772=CARTESIAN_POINT('Origin',(18.8847267479369,83.8,-112.18108636845));
#63773=CARTESIAN_POINT('',(18.8847267479369,83.8,-112.18108636845));
#63774=CARTESIAN_POINT('Origin',(21.5729930956569,83.8,-113.233016678427));
#63775=CARTESIAN_POINT('',(21.5729930956569,83.8,-113.233016678427));
#63776=CARTESIAN_POINT('Origin',(23.8281246409682,83.8,-111.430874884151));
#63777=CARTESIAN_POINT('Origin',(16.4106689907664,83.8,-105.843807665544));
#63778=CARTESIAN_POINT('',(16.4106689907664,83.8,-105.843807665544));
#63779=CARTESIAN_POINT('',(16.8438037931751,83.8,-108.697879769797));
#63780=CARTESIAN_POINT('Origin',(13.7224026430464,83.8,-104.791877355567));
#63781=CARTESIAN_POINT('',(13.7224026430464,83.8,-104.791877355567));
#63782=CARTESIAN_POINT('Origin',(11.467271097735,83.8,-106.594019149843));
#63783=CARTESIAN_POINT('',(11.467271097735,83.8,-106.594019149843));
#63784=CARTESIAN_POINT('Origin',(11.9004059001438,83.8,-109.448091254096));
#63785=CARTESIAN_POINT('',(11.9004059001438,83.8,-109.448091254096));
#63786=CARTESIAN_POINT('Origin',(14.5886722478638,83.8,-110.500021564073));
#63787=CARTESIAN_POINT('',(14.5886722478638,83.8,-110.500021564073));
#63788=CARTESIAN_POINT('Origin',(16.8438037931751,83.8,-108.697879769797));
#63789=CARTESIAN_POINT('Origin',(9.42634814297327,83.8,-103.11081255119));
#63790=CARTESIAN_POINT('',(9.42634814297327,83.8,-103.11081255119));
#63791=CARTESIAN_POINT('',(9.85948294538199,83.8,-105.964884655444));
#63792=CARTESIAN_POINT('Origin',(6.73808179525326,83.8,-102.058882241213));
#63793=CARTESIAN_POINT('',(6.73808179525326,83.8,-102.058882241213));
#63794=CARTESIAN_POINT('Origin',(4.48295024994191,83.8,-103.861024035489));
#63795=CARTESIAN_POINT('',(4.48295024994191,83.8,-103.861024035489));
#63796=CARTESIAN_POINT('Origin',(4.91608505235064,83.8,-106.715096139742));
#63797=CARTESIAN_POINT('',(4.91608505235064,83.8,-106.715096139742));
#63798=CARTESIAN_POINT('Origin',(7.60435140007067,83.8,-107.767026449719));
#63799=CARTESIAN_POINT('',(7.60435140007067,83.8,-107.767026449719));
#63800=CARTESIAN_POINT('Origin',(9.85948294538199,83.8,-105.964884655444));
#63801=CARTESIAN_POINT('Origin',(2.44202729518014,83.8,-100.377817436837));
#63802=CARTESIAN_POINT('',(2.44202729518014,83.8,-100.377817436837));
#63803=CARTESIAN_POINT('',(2.87516209758886,83.8,-103.23188954109));
#63804=CARTESIAN_POINT('Origin',(-0.246239052539871,83.8,-99.3258871268591));
#63805=CARTESIAN_POINT('',(-0.246239052539871,83.8,-99.3258871268591));
#63806=CARTESIAN_POINT('Origin',(-2.50137059785123,83.8,-101.128028921135));
#63807=CARTESIAN_POINT('',(-2.50137059785123,83.8,-101.128028921135));
#63808=CARTESIAN_POINT('Origin',(-2.06823579544249,83.8,-103.982101025388));
#63809=CARTESIAN_POINT('',(-2.06823579544249,83.8,-103.982101025388));
#63810=CARTESIAN_POINT('Origin',(0.620030552277533,83.8,-105.034031335365));
#63811=CARTESIAN_POINT('',(0.620030552277533,83.8,-105.034031335365));
#63812=CARTESIAN_POINT('Origin',(2.87516209758886,83.8,-103.23188954109));
#63813=CARTESIAN_POINT('Origin',(-4.54229355261299,83.8,-97.6448223224826));
#63814=CARTESIAN_POINT('',(-4.54229355261299,83.8,-97.6448223224826));
#63815=CARTESIAN_POINT('',(-4.10915875020428,83.8,-100.498894426736));
#63816=CARTESIAN_POINT('Origin',(-7.230559900333,83.8,-96.5928920125052));
#63817=CARTESIAN_POINT('',(-7.230559900333,83.8,-96.5928920125052));
#63818=CARTESIAN_POINT('Origin',(-9.48569144564436,83.8,-98.3950338067809));
#63819=CARTESIAN_POINT('',(-9.48569144564436,83.8,-98.3950338067809));
#63820=CARTESIAN_POINT('Origin',(-9.05255664323563,83.8,-101.249105911034));
#63821=CARTESIAN_POINT('',(-9.05255664323563,83.8,-101.249105911034));
#63822=CARTESIAN_POINT('Origin',(-6.3642902955156,83.8,-102.301036221011));
#63823=CARTESIAN_POINT('',(-6.3642902955156,83.8,-102.301036221011));
#63824=CARTESIAN_POINT('Origin',(-4.10915875020428,83.8,-100.498894426736));
#63825=CARTESIAN_POINT('Origin',(-11.5266144004061,83.8,-94.9118272081287));
#63826=CARTESIAN_POINT('',(-11.5266144004061,83.8,-94.9118272081287));
#63827=CARTESIAN_POINT('',(-11.0934795979974,83.8,-97.7658993123818));
#63828=CARTESIAN_POINT('Origin',(-14.2148807481261,83.8,-93.8598968981513));
#63829=CARTESIAN_POINT('',(-14.2148807481261,83.8,-93.8598968981513));
#63830=CARTESIAN_POINT('Origin',(-16.4700122934375,83.8,-95.662038692427));
#63831=CARTESIAN_POINT('',(-16.4700122934375,83.8,-95.662038692427));
#63832=CARTESIAN_POINT('Origin',(-16.0368774910288,83.8,-98.5161107966801));
#63833=CARTESIAN_POINT('',(-16.0368774910288,83.8,-98.5161107966801));
#63834=CARTESIAN_POINT('Origin',(-13.3486111433087,83.8,-99.5680411066575));
#63835=CARTESIAN_POINT('',(-13.3486111433087,83.8,-99.5680411066575));
#63836=CARTESIAN_POINT('Origin',(-11.0934795979974,83.8,-97.7658993123818));
#63837=CARTESIAN_POINT('Origin',(-18.5109352481993,83.8,-92.1788320937748));
#63838=CARTESIAN_POINT('',(-18.5109352481993,83.8,-92.1788320937748));
#63839=CARTESIAN_POINT('',(-18.0778004457905,83.8,-95.0329041980279));
#63840=CARTESIAN_POINT('Origin',(-21.1992015959193,83.8,-91.1269017837974));
#63841=CARTESIAN_POINT('',(-21.1992015959193,83.8,-91.1269017837974));
#63842=CARTESIAN_POINT('Origin',(-23.4543331412306,83.8,-92.9290435780731));
#63843=CARTESIAN_POINT('',(-23.4543331412306,83.8,-92.9290435780731));
#63844=CARTESIAN_POINT('Origin',(-23.0211983388219,83.8,-95.7831156823262));
#63845=CARTESIAN_POINT('',(-23.0211983388219,83.8,-95.7831156823262));
#63846=CARTESIAN_POINT('Origin',(-20.3329319911019,83.8,-96.8350459923036));
#63847=CARTESIAN_POINT('',(-20.3329319911019,83.8,-96.8350459923036));
#63848=CARTESIAN_POINT('Origin',(-18.0778004457905,83.8,-95.0329041980279));
#63849=CARTESIAN_POINT('Origin',(-25.4952560959924,83.8,-89.4458369794209));
#63850=CARTESIAN_POINT('',(-25.4952560959924,83.8,-89.4458369794209));
#63851=CARTESIAN_POINT('',(-25.0621212935837,83.8,-92.2999090836741));
#63852=CARTESIAN_POINT('Origin',(-28.1835224437124,83.8,-88.3939066694435));
#63853=CARTESIAN_POINT('',(-28.1835224437124,83.8,-88.3939066694435));
#63854=CARTESIAN_POINT('Origin',(-30.4386539890237,83.8,-90.1960484637193));
#63855=CARTESIAN_POINT('',(-30.4386539890237,83.8,-90.1960484637193));
#63856=CARTESIAN_POINT('Origin',(-30.005519186615,83.8,-93.0501205679723));
#63857=CARTESIAN_POINT('',(-30.005519186615,83.8,-93.0501205679723));
#63858=CARTESIAN_POINT('Origin',(-27.317252838895,83.8,-94.1020508779497));
#63859=CARTESIAN_POINT('',(-27.317252838895,83.8,-94.1020508779497));
#63860=CARTESIAN_POINT('Origin',(-25.0621212935837,83.8,-92.2999090836741));
#63861=CARTESIAN_POINT('Origin',(-32.4795769437855,83.8,-86.7128418650671));
#63862=CARTESIAN_POINT('',(-32.4795769437855,83.8,-86.7128418650671));
#63863=CARTESIAN_POINT('',(-32.0464421413768,83.8,-89.5669139693202));
#63864=CARTESIAN_POINT('Origin',(-35.1678432915055,83.8,-85.6609115550896));
#63865=CARTESIAN_POINT('',(-35.1678432915055,83.8,-85.6609115550896));
#63866=CARTESIAN_POINT('Origin',(-37.4229748368169,83.8,-87.4630533493654));
#63867=CARTESIAN_POINT('',(-37.4229748368169,83.8,-87.4630533493654));
#63868=CARTESIAN_POINT('Origin',(-36.9898400344081,83.8,-90.3171254536184));
#63869=CARTESIAN_POINT('',(-36.9898400344081,83.8,-90.3171254536184));
#63870=CARTESIAN_POINT('Origin',(-34.3015736866881,83.8,-91.3690557635958));
#63871=CARTESIAN_POINT('',(-34.3015736866881,83.8,-91.3690557635958));
#63872=CARTESIAN_POINT('Origin',(-32.0464421413768,83.8,-89.5669139693202));
#63873=CARTESIAN_POINT('Origin',(-39.4638977915786,83.8,-83.9798467507132));
#63874=CARTESIAN_POINT('',(-39.4638977915786,83.8,-83.9798467507132));
#63875=CARTESIAN_POINT('',(-39.0307629891699,83.8,-86.8339188549663));
#63876=CARTESIAN_POINT('Origin',(-42.1521641392987,83.8,-82.9279164407358));
#63877=CARTESIAN_POINT('',(-42.1521641392987,83.8,-82.9279164407358));
#63878=CARTESIAN_POINT('Origin',(-44.40729568461,83.8,-84.7300582350115));
#63879=CARTESIAN_POINT('',(-44.40729568461,83.8,-84.7300582350115));
#63880=CARTESIAN_POINT('Origin',(-43.9741608822013,83.8,-87.5841303392645));
#63881=CARTESIAN_POINT('',(-43.9741608822013,83.8,-87.5841303392645));
#63882=CARTESIAN_POINT('Origin',(-41.2858945344812,83.8,-88.636060649242));
#63883=CARTESIAN_POINT('',(-41.2858945344812,83.8,-88.636060649242));
#63884=CARTESIAN_POINT('Origin',(-39.0307629891699,83.8,-86.8339188549663));
#63885=CARTESIAN_POINT('Origin',(-46.4482186393718,83.8,-81.2468516363593));
#63886=CARTESIAN_POINT('',(-46.4482186393718,83.8,-81.2468516363593));
#63887=CARTESIAN_POINT('',(-46.0150838369631,83.8,-84.1009237406124));
#63888=CARTESIAN_POINT('Origin',(-49.1364849870918,83.8,-80.1949213263819));
#63889=CARTESIAN_POINT('',(-49.1364849870918,83.8,-80.1949213263819));
#63890=CARTESIAN_POINT('Origin',(-51.3916165324031,83.8,-81.9970631206576));
#63891=CARTESIAN_POINT('',(-51.3916165324031,83.8,-81.9970631206576));
#63892=CARTESIAN_POINT('Origin',(-50.9584817299944,83.8,-84.8511352249106));
#63893=CARTESIAN_POINT('',(-50.9584817299944,83.8,-84.8511352249106));
#63894=CARTESIAN_POINT('Origin',(-48.2702153822744,83.8,-85.9030655348881));
#63895=CARTESIAN_POINT('',(-48.2702153822744,83.8,-85.9030655348881));
#63896=CARTESIAN_POINT('Origin',(-46.0150838369631,83.8,-84.1009237406124));
#63897=CARTESIAN_POINT('Origin',(31.5046279128,83.8,-118.724894733799));
#63898=CARTESIAN_POINT('',(31.5046279128,83.8,-118.724894733799));
#63899=CARTESIAN_POINT('',(31.9377627152088,83.8,-121.578966838052));
#63900=CARTESIAN_POINT('Origin',(28.81636156508,83.8,-117.672964423822));
#63901=CARTESIAN_POINT('',(28.81636156508,83.8,-117.672964423822));
#63902=CARTESIAN_POINT('Origin',(26.5612300197687,83.8,-119.475106218097));
#63903=CARTESIAN_POINT('',(26.5612300197687,83.8,-119.475106218097));
#63904=CARTESIAN_POINT('Origin',(26.9943648221774,83.8,-122.32917832235));
#63905=CARTESIAN_POINT('',(26.9943648221774,83.8,-122.32917832235));
#63906=CARTESIAN_POINT('Origin',(29.6826311698974,83.8,-123.381108632328));
#63907=CARTESIAN_POINT('',(29.6826311698974,83.8,-123.381108632328));
#63908=CARTESIAN_POINT('Origin',(31.9377627152088,83.8,-121.578966838052));
#63909=CARTESIAN_POINT('Origin',(24.5203070650069,83.8,-115.991899619445));
#63910=CARTESIAN_POINT('',(24.5203070650069,83.8,-115.991899619445));
#63911=CARTESIAN_POINT('',(24.9534418674156,83.8,-118.845971723698));
#63912=CARTESIAN_POINT('Origin',(21.8320407172869,83.8,-114.939969309468));
#63913=CARTESIAN_POINT('',(21.8320407172869,83.8,-114.939969309468));
#63914=CARTESIAN_POINT('Origin',(19.5769091719755,83.8,-116.742111103744));
#63915=CARTESIAN_POINT('',(19.5769091719755,83.8,-116.742111103744));
#63916=CARTESIAN_POINT('Origin',(20.0100439743843,83.8,-119.596183207997));
#63917=CARTESIAN_POINT('',(20.0100439743843,83.8,-119.596183207997));
#63918=CARTESIAN_POINT('Origin',(22.6983103221043,83.8,-120.648113517974));
#63919=CARTESIAN_POINT('',(22.6983103221043,83.8,-120.648113517974));
#63920=CARTESIAN_POINT('Origin',(24.9534418674156,83.8,-118.845971723698));
#63921=CARTESIAN_POINT('Origin',(17.5359862172138,83.8,-113.258904505091));
#63922=CARTESIAN_POINT('',(17.5359862172138,83.8,-113.258904505091));
#63923=CARTESIAN_POINT('',(17.9691210196225,83.8,-116.112976609344));
#63924=CARTESIAN_POINT('Origin',(14.8477198694938,83.8,-112.206974195114));
#63925=CARTESIAN_POINT('',(14.8477198694938,83.8,-112.206974195114));
#63926=CARTESIAN_POINT('Origin',(12.5925883241824,83.8,-114.00911598939));
#63927=CARTESIAN_POINT('',(12.5925883241824,83.8,-114.00911598939));
#63928=CARTESIAN_POINT('Origin',(13.0257231265911,83.8,-116.863188093643));
#63929=CARTESIAN_POINT('',(13.0257231265911,83.8,-116.863188093643));
#63930=CARTESIAN_POINT('Origin',(15.7139894743112,83.8,-117.91511840362));
#63931=CARTESIAN_POINT('',(15.7139894743112,83.8,-117.91511840362));
#63932=CARTESIAN_POINT('Origin',(17.9691210196225,83.8,-116.112976609344));
#63933=CARTESIAN_POINT('Origin',(10.5516653694206,83.8,-110.525909390737));
#63934=CARTESIAN_POINT('',(10.5516653694206,83.8,-110.525909390737));
#63935=CARTESIAN_POINT('',(10.9848001718294,83.8,-113.379981494991));
#63936=CARTESIAN_POINT('Origin',(7.86339902170064,83.8,-109.47397908076));
#63937=CARTESIAN_POINT('',(7.86339902170064,83.8,-109.47397908076));
#63938=CARTESIAN_POINT('Origin',(5.60826747638928,83.8,-111.276120875036));
#63939=CARTESIAN_POINT('',(5.60826747638928,83.8,-111.276120875036));
#63940=CARTESIAN_POINT('Origin',(6.04140227879801,83.8,-114.130192979289));
#63941=CARTESIAN_POINT('',(6.04140227879801,83.8,-114.130192979289));
#63942=CARTESIAN_POINT('Origin',(8.72966862651804,83.8,-115.182123289266));
#63943=CARTESIAN_POINT('',(8.72966862651804,83.8,-115.182123289266));
#63944=CARTESIAN_POINT('Origin',(10.9848001718294,83.8,-113.379981494991));
#63945=CARTESIAN_POINT('Origin',(1.31671006873277,83.8,-92.9627205972894));
#63946=CARTESIAN_POINT('',(1.31671006873277,83.8,-92.9627205972894));
#63947=CARTESIAN_POINT('',(1.74984487114149,83.8,-95.8167927015425));
#63948=CARTESIAN_POINT('Origin',(-1.37155627898724,83.8,-91.910790287312));
#63949=CARTESIAN_POINT('',(-1.37155627898724,83.8,-91.910790287312));
#63950=CARTESIAN_POINT('Origin',(-3.6266878242986,83.8,-93.7129320815877));
#63951=CARTESIAN_POINT('',(-3.6266878242986,83.8,-93.7129320815877));
#63952=CARTESIAN_POINT('Origin',(-3.19355302188986,83.8,-96.5670041858408));
#63953=CARTESIAN_POINT('',(-3.19355302188986,83.8,-96.5670041858408));
#63954=CARTESIAN_POINT('Origin',(-0.505286674169835,83.8,-97.6189344958182));
#63955=CARTESIAN_POINT('',(-0.505286674169835,83.8,-97.6189344958182));
#63956=CARTESIAN_POINT('Origin',(1.74984487114149,83.8,-95.8167927015425));
#63957=CARTESIAN_POINT('Origin',(8.3010309165259,83.8,-95.6957157116433));
#63958=CARTESIAN_POINT('',(8.3010309165259,83.8,-95.6957157116433));
#63959=CARTESIAN_POINT('',(8.73416571893462,83.8,-98.5497878158964));
#63960=CARTESIAN_POINT('Origin',(5.6127645688059,83.8,-94.6437854016659));
#63961=CARTESIAN_POINT('',(5.6127645688059,83.8,-94.6437854016659));
#63962=CARTESIAN_POINT('Origin',(3.35763302349454,83.8,-96.4459271959416));
#63963=CARTESIAN_POINT('',(3.35763302349454,83.8,-96.4459271959416));
#63964=CARTESIAN_POINT('Origin',(3.79076782590327,83.8,-99.2999993001947));
#63965=CARTESIAN_POINT('',(3.79076782590327,83.8,-99.2999993001947));
#63966=CARTESIAN_POINT('Origin',(6.4790341736233,83.8,-100.351929610172));
#63967=CARTESIAN_POINT('',(6.4790341736233,83.8,-100.351929610172));
#63968=CARTESIAN_POINT('Origin',(8.73416571893462,83.8,-98.5497878158964));
#63969=CARTESIAN_POINT('Origin',(15.285351764319,83.8,-98.4287108259972));
#63970=CARTESIAN_POINT('',(15.285351764319,83.8,-98.4287108259972));
#63971=CARTESIAN_POINT('',(15.7184865667278,83.8,-101.28278293025));
#63972=CARTESIAN_POINT('Origin',(12.597085416599,83.8,-97.3767805160198));
#63973=CARTESIAN_POINT('',(12.597085416599,83.8,-97.3767805160198));
#63974=CARTESIAN_POINT('Origin',(10.3419538712877,83.8,-99.1789223102955));
#63975=CARTESIAN_POINT('',(10.3419538712877,83.8,-99.1789223102955));
#63976=CARTESIAN_POINT('Origin',(10.7750886736964,83.8,-102.032994414549));
#63977=CARTESIAN_POINT('',(10.7750886736964,83.8,-102.032994414549));
#63978=CARTESIAN_POINT('Origin',(13.4633550214164,83.8,-103.084924724526));
#63979=CARTESIAN_POINT('',(13.4633550214164,83.8,-103.084924724526));
#63980=CARTESIAN_POINT('Origin',(15.7184865667278,83.8,-101.28278293025));
#63981=CARTESIAN_POINT('Origin',(22.2696726121122,83.8,-101.161705940351));
#63982=CARTESIAN_POINT('',(22.2696726121122,83.8,-101.161705940351));
#63983=CARTESIAN_POINT('',(22.7028074145209,83.8,-104.015778044604));
#63984=CARTESIAN_POINT('Origin',(19.5814062643922,83.8,-100.109775630374));
#63985=CARTESIAN_POINT('',(19.5814062643922,83.8,-100.109775630374));
#63986=CARTESIAN_POINT('Origin',(17.3262747190808,83.8,-101.911917424649));
#63987=CARTESIAN_POINT('',(17.3262747190808,83.8,-101.911917424649));
#63988=CARTESIAN_POINT('Origin',(17.7594095214895,83.8,-104.765989528902));
#63989=CARTESIAN_POINT('',(17.7594095214895,83.8,-104.765989528902));
#63990=CARTESIAN_POINT('Origin',(20.4476758692096,83.8,-105.81791983888));
#63991=CARTESIAN_POINT('',(20.4476758692096,83.8,-105.81791983888));
#63992=CARTESIAN_POINT('Origin',(22.7028074145209,83.8,-104.015778044604));
#63993=CARTESIAN_POINT('Origin',(-48.6988530922665,83.8,-66.4166579572652));
#63994=CARTESIAN_POINT('',(-48.6988530922665,83.8,-66.4166579572652));
#63995=CARTESIAN_POINT('',(-48.2657182898578,83.8,-69.2707300615183));
#63996=CARTESIAN_POINT('Origin',(-51.3871194399865,83.8,-65.3647276472878));
#63997=CARTESIAN_POINT('',(-51.3871194399865,83.8,-65.3647276472878));
#63998=CARTESIAN_POINT('Origin',(-53.6422509852979,83.8,-67.1668694415634));
#63999=CARTESIAN_POINT('',(-53.6422509852979,83.8,-67.1668694415634));
#64000=CARTESIAN_POINT('Origin',(-53.2091161828892,83.8,-70.0209415458165));
#64001=CARTESIAN_POINT('',(-53.2091161828892,83.8,-70.0209415458165));
#64002=CARTESIAN_POINT('Origin',(-50.5208498351691,83.8,-71.0728718557939));
#64003=CARTESIAN_POINT('',(-50.5208498351691,83.8,-71.0728718557939));
#64004=CARTESIAN_POINT('Origin',(-48.2657182898578,83.8,-69.2707300615183));
#64005=CARTESIAN_POINT('Origin',(43.2226351554916,83.8,-109.360691283413));
#64006=CARTESIAN_POINT('',(43.2226351554916,83.8,-109.360691283413));
#64007=CARTESIAN_POINT('',(43.6557699579003,83.8,-112.214763387666));
#64008=CARTESIAN_POINT('Origin',(40.5343688077715,83.8,-108.308760973435));
#64009=CARTESIAN_POINT('',(40.5343688077715,83.8,-108.308760973435));
#64010=CARTESIAN_POINT('Origin',(38.2792372624602,83.8,-110.110902767711));
#64011=CARTESIAN_POINT('',(38.2792372624602,83.8,-110.110902767711));
#64012=CARTESIAN_POINT('Origin',(38.7123720648689,83.8,-112.964974871964));
#64013=CARTESIAN_POINT('',(38.7123720648689,83.8,-112.964974871964));
#64014=CARTESIAN_POINT('Origin',(41.4006384125889,83.8,-114.016905181942));
#64015=CARTESIAN_POINT('',(41.4006384125889,83.8,-114.016905181942));
#64016=CARTESIAN_POINT('Origin',(43.6557699579003,83.8,-112.214763387666));
#64017=CARTESIAN_POINT('Origin',(36.2383143076984,83.8,-106.627696169059));
#64018=CARTESIAN_POINT('',(36.2383143076984,83.8,-106.627696169059));
#64019=CARTESIAN_POINT('',(36.6714491101071,83.8,-109.481768273312));
#64020=CARTESIAN_POINT('Origin',(33.5500479599784,83.8,-105.575765859081));
#64021=CARTESIAN_POINT('',(33.5500479599784,83.8,-105.575765859081));
#64022=CARTESIAN_POINT('Origin',(31.2949164146671,83.8,-107.377907653357));
#64023=CARTESIAN_POINT('',(31.2949164146671,83.8,-107.377907653357));
#64024=CARTESIAN_POINT('Origin',(31.7280512170758,83.8,-110.23197975761));
#64025=CARTESIAN_POINT('',(31.7280512170758,83.8,-110.23197975761));
#64026=CARTESIAN_POINT('Origin',(34.4163175647958,83.8,-111.283910067588));
#64027=CARTESIAN_POINT('',(34.4163175647958,83.8,-111.283910067588));
#64028=CARTESIAN_POINT('Origin',(36.6714491101071,83.8,-109.481768273312));
#64029=CARTESIAN_POINT('Origin',(29.2539934599053,83.8,-103.894701054705));
#64030=CARTESIAN_POINT('',(29.2539934599053,83.8,-103.894701054705));
#64031=CARTESIAN_POINT('',(29.687128262314,83.8,-106.748773158958));
#64032=CARTESIAN_POINT('Origin',(26.5657271121853,83.8,-102.842770744728));
#64033=CARTESIAN_POINT('',(26.5657271121853,83.8,-102.842770744728));
#64034=CARTESIAN_POINT('Origin',(24.3105955668739,83.8,-104.644912539003));
#64035=CARTESIAN_POINT('',(24.3105955668739,83.8,-104.644912539003));
#64036=CARTESIAN_POINT('Origin',(24.7437303692827,83.8,-107.498984643256));
#64037=CARTESIAN_POINT('',(24.7437303692827,83.8,-107.498984643256));
#64038=CARTESIAN_POINT('Origin',(27.4319967170027,83.8,-108.550914953234));
#64039=CARTESIAN_POINT('',(27.4319967170027,83.8,-108.550914953234));
#64040=CARTESIAN_POINT('Origin',(29.687128262314,83.8,-106.748773158958));
#64041=CARTESIAN_POINT('Origin',(-33.6048941702329,83.8,-79.29774502552));
#64042=CARTESIAN_POINT('',(-33.6048941702329,83.8,-79.29774502552));
#64043=CARTESIAN_POINT('',(-33.1717593678242,83.8,-82.1518171297731));
#64044=CARTESIAN_POINT('Origin',(-36.2931605179529,83.8,-78.2458147155426));
#64045=CARTESIAN_POINT('',(-36.2931605179529,83.8,-78.2458147155426));
#64046=CARTESIAN_POINT('Origin',(-38.5482920632642,83.8,-80.0479565098183));
#64047=CARTESIAN_POINT('',(-38.5482920632642,83.8,-80.0479565098183));
#64048=CARTESIAN_POINT('Origin',(-38.1151572608555,83.8,-82.9020286140714));
#64049=CARTESIAN_POINT('',(-38.1151572608555,83.8,-82.9020286140714));
#64050=CARTESIAN_POINT('Origin',(-35.4268909131355,83.8,-83.9539589240488));
#64051=CARTESIAN_POINT('',(-35.4268909131355,83.8,-83.9539589240488));
#64052=CARTESIAN_POINT('Origin',(-33.1717593678242,83.8,-82.1518171297731));
#64053=CARTESIAN_POINT('Origin',(-40.589215018026,83.8,-76.5647499111661));
#64054=CARTESIAN_POINT('',(-40.589215018026,83.8,-76.5647499111661));
#64055=CARTESIAN_POINT('',(-40.1560802156173,83.8,-79.4188220154192));
#64056=CARTESIAN_POINT('Origin',(-43.277481365746,83.8,-75.5128196011887));
#64057=CARTESIAN_POINT('',(-43.277481365746,83.8,-75.5128196011887));
#64058=CARTESIAN_POINT('Origin',(-45.5326129110574,83.8,-77.3149613954644));
#64059=CARTESIAN_POINT('',(-45.5326129110574,83.8,-77.3149613954644));
#64060=CARTESIAN_POINT('Origin',(-45.0994781086486,83.8,-80.1690334997174));
#64061=CARTESIAN_POINT('',(-45.0994781086486,83.8,-80.1690334997174));
#64062=CARTESIAN_POINT('Origin',(-42.4112117609286,83.8,-81.2209638096949));
#64063=CARTESIAN_POINT('',(-42.4112117609286,83.8,-81.2209638096949));
#64064=CARTESIAN_POINT('Origin',(-40.1560802156173,83.8,-79.4188220154192));
#64065=CARTESIAN_POINT('Origin',(-47.5735358658191,83.8,-73.8317547968122));
#64066=CARTESIAN_POINT('',(-47.5735358658191,83.8,-73.8317547968122));
#64067=CARTESIAN_POINT('',(-47.1404010634104,83.8,-76.6858269010653));
#64068=CARTESIAN_POINT('Origin',(-50.2618022135392,83.8,-72.7798244868348));
#64069=CARTESIAN_POINT('',(-50.2618022135392,83.8,-72.7798244868348));
#64070=CARTESIAN_POINT('Origin',(-52.5169337588505,83.8,-74.5819662811105));
#64071=CARTESIAN_POINT('',(-52.5169337588505,83.8,-74.5819662811105));
#64072=CARTESIAN_POINT('Origin',(-52.0837989564418,83.8,-77.4360383853636));
#64073=CARTESIAN_POINT('',(-52.0837989564418,83.8,-77.4360383853636));
#64074=CARTESIAN_POINT('Origin',(-49.3955326087217,83.8,-78.487968695341));
#64075=CARTESIAN_POINT('',(-49.3955326087217,83.8,-78.487968695341));
#64076=CARTESIAN_POINT('Origin',(-47.1404010634104,83.8,-76.6858269010653));
#64077=CARTESIAN_POINT('Origin',(37.3636315341458,83.8,-114.042793008606));
#64078=CARTESIAN_POINT('',(37.3636315341458,83.8,-114.042793008606));
#64079=CARTESIAN_POINT('',(37.7967663365545,83.8,-116.896865112859));
#64080=CARTESIAN_POINT('Origin',(34.6753651864258,83.8,-112.990862698629));
#64081=CARTESIAN_POINT('',(34.6753651864258,83.8,-112.990862698629));
#64082=CARTESIAN_POINT('Origin',(32.4202336411144,83.8,-114.793004492904));
#64083=CARTESIAN_POINT('',(32.4202336411144,83.8,-114.793004492904));
#64084=CARTESIAN_POINT('Origin',(32.8533684435232,83.8,-117.647076597157));
#64085=CARTESIAN_POINT('',(32.8533684435232,83.8,-117.647076597157));
#64086=CARTESIAN_POINT('Origin',(35.5416347912432,83.8,-118.699006907135));
#64087=CARTESIAN_POINT('',(35.5416347912432,83.8,-118.699006907135));
#64088=CARTESIAN_POINT('Origin',(37.7967663365545,83.8,-116.896865112859));
#64089=CARTESIAN_POINT('Origin',(-26.6205733224398,83.8,-82.0307401398739));
#64090=CARTESIAN_POINT('',(-26.6205733224398,83.8,-82.0307401398739));
#64091=CARTESIAN_POINT('',(-26.187438520031,83.8,-84.884812244127));
#64092=CARTESIAN_POINT('Origin',(-29.3088396701598,83.8,-80.9788098298965));
#64093=CARTESIAN_POINT('',(-29.3088396701598,83.8,-80.9788098298965));
#64094=CARTESIAN_POINT('Origin',(-31.5639712154711,83.8,-82.7809516241722));
#64095=CARTESIAN_POINT('',(-31.5639712154711,83.8,-82.7809516241722));
#64096=CARTESIAN_POINT('Origin',(-31.1308364130624,83.8,-85.6350237284252));
#64097=CARTESIAN_POINT('',(-31.1308364130624,83.8,-85.6350237284252));
#64098=CARTESIAN_POINT('Origin',(-28.4425700653424,83.8,-86.6869540384027));
#64099=CARTESIAN_POINT('',(-28.4425700653424,83.8,-86.6869540384027));
#64100=CARTESIAN_POINT('Origin',(-26.187438520031,83.8,-84.884812244127));
#64101=CARTESIAN_POINT('Origin',(-19.6362524746466,83.8,-84.7637352542278));
#64102=CARTESIAN_POINT('',(-19.6362524746466,83.8,-84.7637352542278));
#64103=CARTESIAN_POINT('',(-19.2031176722379,83.8,-87.6178073584809));
#64104=CARTESIAN_POINT('Origin',(-22.3245188223666,83.8,-83.7118049442504));
#64105=CARTESIAN_POINT('',(-22.3245188223666,83.8,-83.7118049442504));
#64106=CARTESIAN_POINT('Origin',(-24.579650367678,83.8,-85.5139467385261));
#64107=CARTESIAN_POINT('',(-24.579650367678,83.8,-85.5139467385261));
#64108=CARTESIAN_POINT('Origin',(-24.1465155652693,83.8,-88.3680188427791));
#64109=CARTESIAN_POINT('',(-24.1465155652693,83.8,-88.3680188427791));
#64110=CARTESIAN_POINT('Origin',(-21.4582492175492,83.8,-89.4199491527566));
#64111=CARTESIAN_POINT('',(-21.4582492175492,83.8,-89.4199491527566));
#64112=CARTESIAN_POINT('Origin',(-19.2031176722379,83.8,-87.6178073584809));
#64113=CARTESIAN_POINT('Origin',(-12.6519316268535,83.8,-87.4967303685817));
#64114=CARTESIAN_POINT('',(-12.6519316268535,83.8,-87.4967303685817));
#64115=CARTESIAN_POINT('',(-12.2187968244448,83.8,-90.3508024728348));
#64116=CARTESIAN_POINT('Origin',(-15.3401979745735,83.8,-86.4448000586042));
#64117=CARTESIAN_POINT('',(-15.3401979745735,83.8,-86.4448000586042));
#64118=CARTESIAN_POINT('Origin',(-17.5953295198849,83.8,-88.2469418528799));
#64119=CARTESIAN_POINT('',(-17.5953295198849,83.8,-88.2469418528799));
#64120=CARTESIAN_POINT('Origin',(-17.1621947174761,83.8,-91.101013957133));
#64121=CARTESIAN_POINT('',(-17.1621947174761,83.8,-91.101013957133));
#64122=CARTESIAN_POINT('Origin',(-14.4739283697561,83.8,-92.1529442671104));
#64123=CARTESIAN_POINT('',(-14.4739283697561,83.8,-92.1529442671104));
#64124=CARTESIAN_POINT('Origin',(-12.2187968244448,83.8,-90.3508024728348));
#64125=CARTESIAN_POINT('Origin',(-5.66761077906036,83.8,-90.2297254829355));
#64126=CARTESIAN_POINT('',(-5.66761077906036,83.8,-90.2297254829355));
#64127=CARTESIAN_POINT('',(-5.23447597665164,83.8,-93.0837975871887));
#64128=CARTESIAN_POINT('Origin',(-8.35587712678037,83.8,-89.1777951729581));
#64129=CARTESIAN_POINT('',(-8.35587712678037,83.8,-89.1777951729581));
#64130=CARTESIAN_POINT('Origin',(-10.6110086720917,83.8,-90.9799369672338));
#64131=CARTESIAN_POINT('',(-10.6110086720917,83.8,-90.9799369672338));
#64132=CARTESIAN_POINT('Origin',(-10.177873869683,83.8,-93.8340090714869));
#64133=CARTESIAN_POINT('',(-10.177873869683,83.8,-93.8340090714869));
#64134=CARTESIAN_POINT('Origin',(-7.48960752196297,83.8,-94.8859393814643));
#64135=CARTESIAN_POINT('',(-7.48960752196297,83.8,-94.8859393814643));
#64136=CARTESIAN_POINT('Origin',(-5.23447597665164,83.8,-93.0837975871887));
#64137=CARTESIAN_POINT('Origin',(-15.1349835688571,83.8,-114.424122612416));
#64138=CARTESIAN_POINT('',(-15.1349835688571,83.8,-114.424122612416));
#64139=CARTESIAN_POINT('',(-14.7018487664484,83.8,-117.278194716669));
#64140=CARTESIAN_POINT('Origin',(-17.8232499165771,83.8,-113.372192302439));
#64141=CARTESIAN_POINT('',(-17.8232499165771,83.8,-113.372192302439));
#64142=CARTESIAN_POINT('Origin',(-20.0783814618885,83.8,-115.174334096714));
#64143=CARTESIAN_POINT('',(-20.0783814618885,83.8,-115.174334096714));
#64144=CARTESIAN_POINT('Origin',(-19.6452466594797,83.8,-118.028406200967));
#64145=CARTESIAN_POINT('',(-19.6452466594797,83.8,-118.028406200967));
#64146=CARTESIAN_POINT('Origin',(-16.9569803117597,83.8,-119.080336510945));
#64147=CARTESIAN_POINT('',(-16.9569803117597,83.8,-119.080336510945));
#64148=CARTESIAN_POINT('Origin',(-14.7018487664484,83.8,-117.278194716669));
#64149=CARTESIAN_POINT('Origin',(-8.15066272106398,83.8,-117.15711772677));
#64150=CARTESIAN_POINT('',(-8.15066272106398,83.8,-117.15711772677));
#64151=CARTESIAN_POINT('',(-7.71752791865526,83.8,-120.011189831023));
#64152=CARTESIAN_POINT('Origin',(-10.838929068784,83.8,-116.105187416792));
#64153=CARTESIAN_POINT('',(-10.838929068784,83.8,-116.105187416792));
#64154=CARTESIAN_POINT('Origin',(-13.0940606140953,83.8,-117.907329211068));
#64155=CARTESIAN_POINT('',(-13.0940606140953,83.8,-117.907329211068));
#64156=CARTESIAN_POINT('Origin',(-12.6609258116866,83.8,-120.761401315321));
#64157=CARTESIAN_POINT('',(-12.6609258116866,83.8,-120.761401315321));
#64158=CARTESIAN_POINT('Origin',(-9.97265946396659,83.8,-121.813331625299));
#64159=CARTESIAN_POINT('',(-9.97265946396659,83.8,-121.813331625299));
#64160=CARTESIAN_POINT('Origin',(-7.71752791865526,83.8,-120.011189831023));
#64161=CARTESIAN_POINT('Origin',(-1.16634187327085,83.8,-119.890112841124));
#64162=CARTESIAN_POINT('',(-1.16634187327085,83.8,-119.890112841124));
#64163=CARTESIAN_POINT('',(-0.733207070862132,83.8,-122.744184945377));
#64164=CARTESIAN_POINT('Origin',(-3.85460822099086,83.8,-118.838182531146));
#64165=CARTESIAN_POINT('',(-3.85460822099086,83.8,-118.838182531146));
#64166=CARTESIAN_POINT('Origin',(-6.10973976630222,83.8,-120.640324325422));
#64167=CARTESIAN_POINT('',(-6.10973976630222,83.8,-120.640324325422));
#64168=CARTESIAN_POINT('Origin',(-5.67660496389348,83.8,-123.494396429675));
#64169=CARTESIAN_POINT('',(-5.67660496389348,83.8,-123.494396429675));
#64170=CARTESIAN_POINT('Origin',(-2.98833861617346,83.8,-124.546326739653));
#64171=CARTESIAN_POINT('',(-2.98833861617346,83.8,-124.546326739653));
#64172=CARTESIAN_POINT('Origin',(-0.733207070862132,83.8,-122.744184945377));
#64173=CARTESIAN_POINT('Origin',(5.81797897452228,83.8,-122.623107955478));
#64174=CARTESIAN_POINT('',(5.81797897452228,83.8,-122.623107955478));
#64175=CARTESIAN_POINT('',(6.251113776931,83.8,-125.477180059731));
#64176=CARTESIAN_POINT('Origin',(3.12971262680227,83.8,-121.5711776455));
#64177=CARTESIAN_POINT('',(3.12971262680227,83.8,-121.5711776455));
#64178=CARTESIAN_POINT('Origin',(0.874581081490917,83.8,-123.373319439776));
#64179=CARTESIAN_POINT('',(0.874581081490917,83.8,-123.373319439776));
#64180=CARTESIAN_POINT('Origin',(1.30771588389965,83.8,-126.227391544029));
#64181=CARTESIAN_POINT('',(1.30771588389965,83.8,-126.227391544029));
#64182=CARTESIAN_POINT('Origin',(3.99598223161968,83.8,-127.279321854006));
#64183=CARTESIAN_POINT('',(3.99598223161968,83.8,-127.279321854006));
#64184=CARTESIAN_POINT('Origin',(6.251113776931,83.8,-125.477180059731));
#64185=CARTESIAN_POINT('Origin',(-30.2289424908907,83.8,-101.543035544161));
#64186=CARTESIAN_POINT('',(-30.2289424908907,83.8,-101.543035544161));
#64187=CARTESIAN_POINT('',(-29.795807688482,83.8,-104.397107648414));
#64188=CARTESIAN_POINT('Origin',(-32.9172088386108,83.8,-100.491105234184));
#64189=CARTESIAN_POINT('',(-32.9172088386108,83.8,-100.491105234184));
#64190=CARTESIAN_POINT('Origin',(-35.1723403839221,83.8,-102.293247028459));
#64191=CARTESIAN_POINT('',(-35.1723403839221,83.8,-102.293247028459));
#64192=CARTESIAN_POINT('Origin',(-34.7392055815134,83.8,-105.147319132713));
#64193=CARTESIAN_POINT('',(-34.7392055815134,83.8,-105.147319132713));
#64194=CARTESIAN_POINT('Origin',(-32.0509392337934,83.8,-106.19924944269));
#64195=CARTESIAN_POINT('',(-32.0509392337934,83.8,-106.19924944269));
#64196=CARTESIAN_POINT('Origin',(-29.795807688482,83.8,-104.397107648414));
#64197=CARTESIAN_POINT('Origin',(-37.2132633386839,83.8,-98.8100404298073));
#64198=CARTESIAN_POINT('',(-37.2132633386839,83.8,-98.8100404298073));
#64199=CARTESIAN_POINT('',(-36.7801285362752,83.8,-101.66411253406));
#64200=CARTESIAN_POINT('Origin',(-39.9015296864039,83.8,-97.7581101198299));
#64201=CARTESIAN_POINT('',(-39.9015296864039,83.8,-97.7581101198299));
#64202=CARTESIAN_POINT('Origin',(-42.1566612317152,83.8,-99.5602519141056));
#64203=CARTESIAN_POINT('',(-42.1566612317152,83.8,-99.5602519141056));
#64204=CARTESIAN_POINT('Origin',(-41.7235264293065,83.8,-102.414324018359));
#64205=CARTESIAN_POINT('',(-41.7235264293065,83.8,-102.414324018359));
#64206=CARTESIAN_POINT('Origin',(-39.0352600815865,83.8,-103.466254328336));
#64207=CARTESIAN_POINT('',(-39.0352600815865,83.8,-103.466254328336));
#64208=CARTESIAN_POINT('Origin',(-36.7801285362752,83.8,-101.66411253406));
#64209=CARTESIAN_POINT('Origin',(-44.197584186477,83.8,-96.0770453154534));
#64210=CARTESIAN_POINT('',(-44.197584186477,83.8,-96.0770453154534));
#64211=CARTESIAN_POINT('',(-43.7644493840683,83.8,-98.9311174197065));
#64212=CARTESIAN_POINT('Origin',(-46.885850534197,83.8,-95.025115005476));
#64213=CARTESIAN_POINT('',(-46.885850534197,83.8,-95.025115005476));
#64214=CARTESIAN_POINT('Origin',(-49.1409820795084,83.8,-96.8272567997517));
#64215=CARTESIAN_POINT('',(-49.1409820795084,83.8,-96.8272567997517));
#64216=CARTESIAN_POINT('Origin',(-48.7078472770996,83.8,-99.6813289040047));
#64217=CARTESIAN_POINT('',(-48.7078472770996,83.8,-99.6813289040047));
#64218=CARTESIAN_POINT('Origin',(-46.0195809293796,83.8,-100.733259213982));
#64219=CARTESIAN_POINT('',(-46.0195809293796,83.8,-100.733259213982));
#64220=CARTESIAN_POINT('Origin',(-43.7644493840683,83.8,-98.9311174197065));
#64221=CARTESIAN_POINT('Origin',(12.8022998223154,83.8,-125.356103069832));
#64222=CARTESIAN_POINT('',(12.8022998223154,83.8,-125.356103069832));
#64223=CARTESIAN_POINT('',(13.2354346247241,83.8,-128.210175174085));
#64224=CARTESIAN_POINT('Origin',(10.1140334745954,83.8,-124.304172759854));
#64225=CARTESIAN_POINT('',(10.1140334745954,83.8,-124.304172759854));
#64226=CARTESIAN_POINT('Origin',(7.85890192928405,83.8,-126.10631455413));
#64227=CARTESIAN_POINT('',(7.85890192928405,83.8,-126.10631455413));
#64228=CARTESIAN_POINT('Origin',(8.29203673169278,83.8,-128.960386658383));
#64229=CARTESIAN_POINT('',(8.29203673169278,83.8,-128.960386658383));
#64230=CARTESIAN_POINT('Origin',(10.9803030794128,83.8,-130.01231696836));
#64231=CARTESIAN_POINT('',(10.9803030794128,83.8,-130.01231696836));
#64232=CARTESIAN_POINT('Origin',(13.2354346247241,83.8,-128.210175174085));
#64233=CARTESIAN_POINT('Origin',(-22.1193044166502,83.8,-111.691127498062));
#64234=CARTESIAN_POINT('',(-22.1193044166502,83.8,-111.691127498062));
#64235=CARTESIAN_POINT('',(-21.6861696142415,83.8,-114.545199602315));
#64236=CARTESIAN_POINT('Origin',(-24.8075707643703,83.8,-110.639197188085));
#64237=CARTESIAN_POINT('',(-24.8075707643703,83.8,-110.639197188085));
#64238=CARTESIAN_POINT('Origin',(-27.0627023096816,83.8,-112.44133898236));
#64239=CARTESIAN_POINT('',(-27.0627023096816,83.8,-112.44133898236));
#64240=CARTESIAN_POINT('Origin',(-26.6295675072729,83.8,-115.295411086613));
#64241=CARTESIAN_POINT('',(-26.6295675072729,83.8,-115.295411086613));
#64242=CARTESIAN_POINT('Origin',(-23.9413011595528,83.8,-116.347341396591));
#64243=CARTESIAN_POINT('',(-23.9413011595528,83.8,-116.347341396591));
#64244=CARTESIAN_POINT('Origin',(-21.6861696142415,83.8,-114.545199602315));
#64245=CARTESIAN_POINT('Origin',(-29.1036252644434,83.8,-108.958132383708));
#64246=CARTESIAN_POINT('',(-29.1036252644434,83.8,-108.958132383708));
#64247=CARTESIAN_POINT('',(-28.6704904620347,83.8,-111.812204487961));
#64248=CARTESIAN_POINT('Origin',(-31.7918916121634,83.8,-107.906202073731));
#64249=CARTESIAN_POINT('',(-31.7918916121634,83.8,-107.906202073731));
#64250=CARTESIAN_POINT('Origin',(-34.0470231574747,83.8,-109.708343868006));
#64251=CARTESIAN_POINT('',(-34.0470231574747,83.8,-109.708343868006));
#64252=CARTESIAN_POINT('Origin',(-33.613888355066,83.8,-112.56241597226));
#64253=CARTESIAN_POINT('',(-33.613888355066,83.8,-112.56241597226));
#64254=CARTESIAN_POINT('Origin',(-30.925622007346,83.8,-113.614346282237));
#64255=CARTESIAN_POINT('',(-30.925622007346,83.8,-113.614346282237));
#64256=CARTESIAN_POINT('Origin',(-28.6704904620347,83.8,-111.812204487961));
#64257=CARTESIAN_POINT('Origin',(-36.0879461122365,83.8,-106.225137269354));
#64258=CARTESIAN_POINT('',(-36.0879461122365,83.8,-106.225137269354));
#64259=CARTESIAN_POINT('',(-35.6548113098278,83.8,-109.079209373607));
#64260=CARTESIAN_POINT('Origin',(-38.7762124599565,83.8,-105.173206959377));
#64261=CARTESIAN_POINT('',(-38.7762124599565,83.8,-105.173206959377));
#64262=CARTESIAN_POINT('Origin',(-41.0313440052679,83.8,-106.975348753653));
#64263=CARTESIAN_POINT('',(-41.0313440052679,83.8,-106.975348753653));
#64264=CARTESIAN_POINT('Origin',(-40.5982092028591,83.8,-109.829420857906));
#64265=CARTESIAN_POINT('',(-40.5982092028591,83.8,-109.829420857906));
#64266=CARTESIAN_POINT('Origin',(-37.9099428551391,83.8,-110.881351167883));
#64267=CARTESIAN_POINT('',(-37.9099428551391,83.8,-110.881351167883));
#64268=CARTESIAN_POINT('Origin',(-35.6548113098278,83.8,-109.079209373607));
#64269=CARTESIAN_POINT('Origin',(-43.0722669600296,83.8,-103.492142155));
#64270=CARTESIAN_POINT('',(-43.0722669600296,83.8,-103.492142155));
#64271=CARTESIAN_POINT('',(-42.6391321576209,83.8,-106.346214259254));
#64272=CARTESIAN_POINT('Origin',(-45.7605333077496,83.8,-102.440211845023));
#64273=CARTESIAN_POINT('',(-45.7605333077496,83.8,-102.440211845023));
#64274=CARTESIAN_POINT('Origin',(-48.015664853061,83.8,-104.242353639299));
#64275=CARTESIAN_POINT('',(-48.015664853061,83.8,-104.242353639299));
#64276=CARTESIAN_POINT('Origin',(-47.5825300506523,83.8,-107.096425743552));
#64277=CARTESIAN_POINT('',(-47.5825300506523,83.8,-107.096425743552));
#64278=CARTESIAN_POINT('Origin',(-44.8942637029322,83.8,-108.148356053529));
#64279=CARTESIAN_POINT('',(-44.8942637029322,83.8,-108.148356053529));
#64280=CARTESIAN_POINT('Origin',(-42.6391321576209,83.8,-106.346214259254));
#64281=CARTESIAN_POINT('Origin',(-0.0410246468234739,83.8,-127.305209680671));
#64282=CARTESIAN_POINT('',(-0.0410246468234739,83.8,-127.305209680671));
#64283=CARTESIAN_POINT('',(0.392110155585244,83.8,-130.159281784924));
#64284=CARTESIAN_POINT('Origin',(-2.72929099454348,83.8,-126.253279370693));
#64285=CARTESIAN_POINT('',(-2.72929099454348,83.8,-126.253279370693));
#64286=CARTESIAN_POINT('Origin',(-4.98442253985484,83.8,-128.055421164969));
#64287=CARTESIAN_POINT('',(-4.98442253985484,83.8,-128.055421164969));
#64288=CARTESIAN_POINT('Origin',(-4.55128773744611,83.8,-130.909493269222));
#64289=CARTESIAN_POINT('',(-4.55128773744611,83.8,-130.909493269222));
#64290=CARTESIAN_POINT('Origin',(-1.86302138972608,83.8,-131.9614235792));
#64291=CARTESIAN_POINT('',(-1.86302138972608,83.8,-131.9614235792));
#64292=CARTESIAN_POINT('Origin',(0.392110155585244,83.8,-130.159281784924));
#64293=CARTESIAN_POINT('Origin',(-7.02534549461661,83.8,-124.572214566317));
#64294=CARTESIAN_POINT('',(-7.02534549461661,83.8,-124.572214566317));
#64295=CARTESIAN_POINT('',(-6.59221069220789,83.8,-127.42628667057));
#64296=CARTESIAN_POINT('Origin',(-9.71361184233662,83.8,-123.52028425634));
#64297=CARTESIAN_POINT('',(-9.71361184233662,83.8,-123.52028425634));
#64298=CARTESIAN_POINT('Origin',(-11.968743387648,83.8,-125.322426050615));
#64299=CARTESIAN_POINT('',(-11.968743387648,83.8,-125.322426050615));
#64300=CARTESIAN_POINT('Origin',(-11.5356085852392,83.8,-128.176498154868));
#64301=CARTESIAN_POINT('',(-11.5356085852392,83.8,-128.176498154868));
#64302=CARTESIAN_POINT('Origin',(-8.84734223751921,83.8,-129.228428464846));
#64303=CARTESIAN_POINT('',(-8.84734223751921,83.8,-129.228428464846));
#64304=CARTESIAN_POINT('Origin',(-6.59221069220789,83.8,-127.42628667057));
#64305=CARTESIAN_POINT('Origin',(-14.0096663424097,83.8,-121.839219451963));
#64306=CARTESIAN_POINT('',(-14.0096663424097,83.8,-121.839219451963));
#64307=CARTESIAN_POINT('',(-13.576531540001,83.8,-124.693291556216));
#64308=CARTESIAN_POINT('Origin',(-16.6979326901297,83.8,-120.787289141986));
#64309=CARTESIAN_POINT('',(-16.6979326901297,83.8,-120.787289141986));
#64310=CARTESIAN_POINT('Origin',(-18.9530642354411,83.8,-122.589430936261));
#64311=CARTESIAN_POINT('',(-18.9530642354411,83.8,-122.589430936261));
#64312=CARTESIAN_POINT('Origin',(-18.5199294330324,83.8,-125.443503040514));
#64313=CARTESIAN_POINT('',(-18.5199294330324,83.8,-125.443503040514));
#64314=CARTESIAN_POINT('Origin',(-15.8316630853123,83.8,-126.495433350492));
#64315=CARTESIAN_POINT('',(-15.8316630853123,83.8,-126.495433350492));
#64316=CARTESIAN_POINT('Origin',(-13.576531540001,83.8,-124.693291556216));
#64317=CARTESIAN_POINT('Origin',(-20.9939871902029,83.8,-119.106224337609));
#64318=CARTESIAN_POINT('',(-20.9939871902029,83.8,-119.106224337609));
#64319=CARTESIAN_POINT('',(-20.5608523877941,83.8,-121.960296441862));
#64320=CARTESIAN_POINT('Origin',(-23.6822535379229,83.8,-118.054294027632));
#64321=CARTESIAN_POINT('',(-23.6822535379229,83.8,-118.054294027632));
#64322=CARTESIAN_POINT('Origin',(-25.9373850832342,83.8,-119.856435821907));
#64323=CARTESIAN_POINT('',(-25.9373850832342,83.8,-119.856435821907));
#64324=CARTESIAN_POINT('Origin',(-25.5042502808255,83.8,-122.710507926161));
#64325=CARTESIAN_POINT('',(-25.5042502808255,83.8,-122.710507926161));
#64326=CARTESIAN_POINT('Origin',(-22.8159839331055,83.8,-123.762438236138));
#64327=CARTESIAN_POINT('',(-22.8159839331055,83.8,-123.762438236138));
#64328=CARTESIAN_POINT('Origin',(-20.5608523877941,83.8,-121.960296441862));
#64329=CARTESIAN_POINT('Origin',(3.56734452162752,83.8,-107.792914276384));
#64330=CARTESIAN_POINT('',(3.56734452162752,83.8,-107.792914276384));
#64331=CARTESIAN_POINT('',(4.00047932403624,83.8,-110.646986380637));
#64332=CARTESIAN_POINT('Origin',(0.879078173907508,83.8,-106.740983966406));
#64333=CARTESIAN_POINT('',(0.879078173907508,83.8,-106.740983966406));
#64334=CARTESIAN_POINT('Origin',(-1.37605337140385,83.8,-108.543125760682));
#64335=CARTESIAN_POINT('',(-1.37605337140385,83.8,-108.543125760682));
#64336=CARTESIAN_POINT('Origin',(-0.942918568995116,83.8,-111.397197864935));
#64337=CARTESIAN_POINT('',(-0.942918568995116,83.8,-111.397197864935));
#64338=CARTESIAN_POINT('Origin',(1.74534777872491,83.8,-112.449128174912));
#64339=CARTESIAN_POINT('',(1.74534777872491,83.8,-112.449128174912));
#64340=CARTESIAN_POINT('Origin',(4.00047932403624,83.8,-110.646986380637));
#64341=CARTESIAN_POINT('Origin',(-3.41697632616561,83.8,-105.05991916203));
#64342=CARTESIAN_POINT('',(-3.41697632616561,83.8,-105.05991916203));
#64343=CARTESIAN_POINT('',(-2.9838415237569,83.8,-107.913991266283));
#64344=CARTESIAN_POINT('Origin',(-6.10524267388563,83.8,-104.007988852052));
#64345=CARTESIAN_POINT('',(-6.10524267388563,83.8,-104.007988852052));
#64346=CARTESIAN_POINT('Origin',(-8.36037421919698,83.8,-105.810130646328));
#64347=CARTESIAN_POINT('',(-8.36037421919698,83.8,-105.810130646328));
#64348=CARTESIAN_POINT('Origin',(-7.92723941678825,83.8,-108.664202750581));
#64349=CARTESIAN_POINT('',(-7.92723941678825,83.8,-108.664202750581));
#64350=CARTESIAN_POINT('Origin',(-5.23897306906822,83.8,-109.716133060558));
#64351=CARTESIAN_POINT('',(-5.23897306906822,83.8,-109.716133060558));
#64352=CARTESIAN_POINT('Origin',(-2.9838415237569,83.8,-107.913991266283));
#64353=CARTESIAN_POINT('Origin',(-10.4012971739587,83.8,-102.326924047676));
#64354=CARTESIAN_POINT('',(-10.4012971739587,83.8,-102.326924047676));
#64355=CARTESIAN_POINT('',(-9.96816237155003,83.8,-105.180996151929));
#64356=CARTESIAN_POINT('Origin',(-13.0895635216788,83.8,-101.274993737698));
#64357=CARTESIAN_POINT('',(-13.0895635216788,83.8,-101.274993737698));
#64358=CARTESIAN_POINT('Origin',(-15.3446950669901,83.8,-103.077135531974));
#64359=CARTESIAN_POINT('',(-15.3446950669901,83.8,-103.077135531974));
#64360=CARTESIAN_POINT('Origin',(-14.9115602645814,83.8,-105.931207636227));
#64361=CARTESIAN_POINT('',(-14.9115602645814,83.8,-105.931207636227));
#64362=CARTESIAN_POINT('Origin',(-12.2232939168614,83.8,-106.983137946205));
#64363=CARTESIAN_POINT('',(-12.2232939168614,83.8,-106.983137946205));
#64364=CARTESIAN_POINT('Origin',(-9.96816237155003,83.8,-105.180996151929));
#64365=CARTESIAN_POINT('Origin',(-17.3856180217519,83.8,-99.5939289333219));
#64366=CARTESIAN_POINT('',(-17.3856180217519,83.8,-99.5939289333219));
#64367=CARTESIAN_POINT('',(-16.9524832193432,83.8,-102.448001037575));
#64368=CARTESIAN_POINT('Origin',(-20.0738843694719,83.8,-98.5419986233445));
#64369=CARTESIAN_POINT('',(-20.0738843694719,83.8,-98.5419986233445));
#64370=CARTESIAN_POINT('Origin',(-22.3290159147832,83.8,-100.34414041762));
#64371=CARTESIAN_POINT('',(-22.3290159147832,83.8,-100.34414041762));
#64372=CARTESIAN_POINT('Origin',(-21.8958811123745,83.8,-103.198212521873));
#64373=CARTESIAN_POINT('',(-21.8958811123745,83.8,-103.198212521873));
#64374=CARTESIAN_POINT('Origin',(-19.2076147646545,83.8,-104.250142831851));
#64375=CARTESIAN_POINT('',(-19.2076147646545,83.8,-104.250142831851));
#64376=CARTESIAN_POINT('Origin',(-16.9524832193432,83.8,-102.448001037575));
#64377=CARTESIAN_POINT('Origin',(-24.369938869545,83.8,-96.860933818968));
#64378=CARTESIAN_POINT('',(-24.369938869545,83.8,-96.860933818968));
#64379=CARTESIAN_POINT('',(-23.9368040671363,83.8,-99.7150059232211));
#64380=CARTESIAN_POINT('Origin',(-27.058205217265,83.8,-95.8090035089906));
#64381=CARTESIAN_POINT('',(-27.058205217265,83.8,-95.8090035089906));
#64382=CARTESIAN_POINT('Origin',(-29.3133367625764,83.8,-97.6111453032663));
#64383=CARTESIAN_POINT('',(-29.3133367625764,83.8,-97.6111453032663));
#64384=CARTESIAN_POINT('Origin',(-28.8802019601676,83.8,-100.465217407519));
#64385=CARTESIAN_POINT('',(-28.8802019601676,83.8,-100.465217407519));
#64386=CARTESIAN_POINT('Origin',(-26.1919356124476,83.8,-101.517147717497));
#64387=CARTESIAN_POINT('',(-26.1919356124476,83.8,-101.517147717497));
#64388=CARTESIAN_POINT('Origin',(-23.9368040671363,83.8,-99.7150059232211));
#64389=CARTESIAN_POINT('Origin',(-31.3542597173381,83.8,-94.1279387046141));
#64390=CARTESIAN_POINT('',(-31.3542597173381,83.8,-94.1279387046141));
#64391=CARTESIAN_POINT('',(-30.9211249149294,83.8,-96.9820108088672));
#64392=CARTESIAN_POINT('Origin',(-34.0425260650581,83.8,-93.0760083946367));
#64393=CARTESIAN_POINT('',(-34.0425260650581,83.8,-93.0760083946367));
#64394=CARTESIAN_POINT('Origin',(-36.2976576103695,83.8,-94.8781501889124));
#64395=CARTESIAN_POINT('',(-36.2976576103695,83.8,-94.8781501889124));
#64396=CARTESIAN_POINT('Origin',(-35.8645228079608,83.8,-97.7322222931655));
#64397=CARTESIAN_POINT('',(-35.8645228079608,83.8,-97.7322222931655));
#64398=CARTESIAN_POINT('Origin',(-33.1762564602408,83.8,-98.7841526031429));
#64399=CARTESIAN_POINT('',(-33.1762564602408,83.8,-98.7841526031429));
#64400=CARTESIAN_POINT('Origin',(-30.9211249149294,83.8,-96.9820108088672));
#64401=CARTESIAN_POINT('Origin',(-38.3385805651313,83.8,-91.3949435902602));
#64402=CARTESIAN_POINT('',(-38.3385805651313,83.8,-91.3949435902602));
#64403=CARTESIAN_POINT('',(-37.9054457627226,83.8,-94.2490156945133));
#64404=CARTESIAN_POINT('Origin',(-41.0268469128513,83.8,-90.3430132802828));
#64405=CARTESIAN_POINT('',(-41.0268469128513,83.8,-90.3430132802828));
#64406=CARTESIAN_POINT('Origin',(-43.2819784581626,83.8,-92.1451550745585));
#64407=CARTESIAN_POINT('',(-43.2819784581626,83.8,-92.1451550745585));
#64408=CARTESIAN_POINT('Origin',(-42.8488436557539,83.8,-94.9992271788116));
#64409=CARTESIAN_POINT('',(-42.8488436557539,83.8,-94.9992271788116));
#64410=CARTESIAN_POINT('Origin',(-40.1605773080339,83.8,-96.051157488789));
#64411=CARTESIAN_POINT('',(-40.1605773080339,83.8,-96.051157488789));
#64412=CARTESIAN_POINT('Origin',(-37.9054457627226,83.8,-94.2490156945133));
#64413=CARTESIAN_POINT('Origin',(-45.3229014129244,83.8,-88.6619484759063));
#64414=CARTESIAN_POINT('',(-45.3229014129244,83.8,-88.6619484759063));
#64415=CARTESIAN_POINT('',(-44.8897666105157,83.8,-91.5160205801594));
#64416=CARTESIAN_POINT('Origin',(-48.0111677606444,83.8,-87.6100181659289));
#64417=CARTESIAN_POINT('',(-48.0111677606444,83.8,-87.6100181659289));
#64418=CARTESIAN_POINT('Origin',(-50.2662993059558,83.8,-89.4121599602046));
#64419=CARTESIAN_POINT('',(-50.2662993059558,83.8,-89.4121599602046));
#64420=CARTESIAN_POINT('Origin',(-49.833164503547,83.8,-92.2662320644577));
#64421=CARTESIAN_POINT('',(-49.833164503547,83.8,-92.2662320644577));
#64422=CARTESIAN_POINT('Origin',(-47.144898155827,83.8,-93.3181623744351));
#64423=CARTESIAN_POINT('',(-47.144898155827,83.8,-93.3181623744351));
#64424=CARTESIAN_POINT('Origin',(-44.8897666105157,83.8,-91.5160205801594));
#64425=CARTESIAN_POINT('Origin',(25.6456242914543,83.8,-123.406996458992));
#64426=CARTESIAN_POINT('',(25.6456242914543,83.8,-123.406996458992));
#64427=CARTESIAN_POINT('',(26.078759093863,83.8,-126.261068563245));
#64428=CARTESIAN_POINT('Origin',(22.9573579437343,83.8,-122.355066149015));
#64429=CARTESIAN_POINT('',(22.9573579437343,83.8,-122.355066149015));
#64430=CARTESIAN_POINT('Origin',(20.7022263984229,83.8,-124.157207943291));
#64431=CARTESIAN_POINT('',(20.7022263984229,83.8,-124.157207943291));
#64432=CARTESIAN_POINT('Origin',(21.1353612008317,83.8,-127.011280047544));
#64433=CARTESIAN_POINT('',(21.1353612008317,83.8,-127.011280047544));
#64434=CARTESIAN_POINT('Origin',(23.8236275485517,83.8,-128.063210357521));
#64435=CARTESIAN_POINT('',(23.8236275485517,83.8,-128.063210357521));
#64436=CARTESIAN_POINT('Origin',(26.078759093863,83.8,-126.261068563245));
#64437=CARTESIAN_POINT('Origin',(18.6613034436612,83.8,-120.674001344638));
#64438=CARTESIAN_POINT('',(18.6613034436612,83.8,-120.674001344638));
#64439=CARTESIAN_POINT('',(19.0944382460699,83.8,-123.528073448892));
#64440=CARTESIAN_POINT('Origin',(15.9730370959412,83.8,-119.622071034661));
#64441=CARTESIAN_POINT('',(15.9730370959412,83.8,-119.622071034661));
#64442=CARTESIAN_POINT('Origin',(13.7179055506298,83.8,-121.424212828937));
#64443=CARTESIAN_POINT('',(13.7179055506298,83.8,-121.424212828937));
#64444=CARTESIAN_POINT('Origin',(14.1510403530385,83.8,-124.27828493319));
#64445=CARTESIAN_POINT('',(14.1510403530385,83.8,-124.27828493319));
#64446=CARTESIAN_POINT('Origin',(16.8393067007586,83.8,-125.330215243167));
#64447=CARTESIAN_POINT('',(16.8393067007586,83.8,-125.330215243167));
#64448=CARTESIAN_POINT('Origin',(19.0944382460699,83.8,-123.528073448892));
#64449=CARTESIAN_POINT('Origin',(11.676982595868,83.8,-117.941006230285));
#64450=CARTESIAN_POINT('',(11.676982595868,83.8,-117.941006230285));
#64451=CARTESIAN_POINT('',(12.1101173982768,83.8,-120.795078334538));
#64452=CARTESIAN_POINT('Origin',(8.98871624814803,83.8,-116.889075920307));
#64453=CARTESIAN_POINT('',(8.98871624814803,83.8,-116.889075920307));
#64454=CARTESIAN_POINT('Origin',(6.73358470283667,83.8,-118.691217714583));
#64455=CARTESIAN_POINT('',(6.73358470283667,83.8,-118.691217714583));
#64456=CARTESIAN_POINT('Origin',(7.1667195052454,83.8,-121.545289818836));
#64457=CARTESIAN_POINT('',(7.1667195052454,83.8,-121.545289818836));
#64458=CARTESIAN_POINT('Origin',(9.85498585296543,83.8,-122.597220128813));
#64459=CARTESIAN_POINT('',(9.85498585296543,83.8,-122.597220128813));
#64460=CARTESIAN_POINT('Origin',(12.1101173982768,83.8,-120.795078334538));
#64461=CARTESIAN_POINT('Origin',(4.69266174807491,83.8,-115.208011115931));
#64462=CARTESIAN_POINT('',(4.69266174807491,83.8,-115.208011115931));
#64463=CARTESIAN_POINT('',(5.12579655048363,83.8,-118.062083220184));
#64464=CARTESIAN_POINT('Origin',(2.0043954003549,83.8,-114.156080805953));
#64465=CARTESIAN_POINT('',(2.0043954003549,83.8,-114.156080805953));
#64466=CARTESIAN_POINT('Origin',(-0.250736144956458,83.8,-115.958222600229));
#64467=CARTESIAN_POINT('',(-0.250736144956458,83.8,-115.958222600229));
#64468=CARTESIAN_POINT('Origin',(0.182398657452273,83.8,-118.812294704482));
#64469=CARTESIAN_POINT('',(0.182398657452273,83.8,-118.812294704482));
#64470=CARTESIAN_POINT('Origin',(2.8706650051723,83.8,-119.864225014459));
#64471=CARTESIAN_POINT('',(2.8706650051723,83.8,-119.864225014459));
#64472=CARTESIAN_POINT('Origin',(5.12579655048363,83.8,-118.062083220184));
#64473=CARTESIAN_POINT('Origin',(-2.29165909971822,83.8,-112.475016001577));
#64474=CARTESIAN_POINT('',(-2.29165909971822,83.8,-112.475016001577));
#64475=CARTESIAN_POINT('',(-1.85852429730951,83.8,-115.32908810583));
#64476=CARTESIAN_POINT('Origin',(-4.97992544743824,83.8,-111.423085691599));
#64477=CARTESIAN_POINT('',(-4.97992544743824,83.8,-111.423085691599));
#64478=CARTESIAN_POINT('Origin',(-7.23505699274959,83.8,-113.225227485875));
#64479=CARTESIAN_POINT('',(-7.23505699274959,83.8,-113.225227485875));
#64480=CARTESIAN_POINT('Origin',(-6.80192219034086,83.8,-116.079299590128));
#64481=CARTESIAN_POINT('',(-6.80192219034086,83.8,-116.079299590128));
#64482=CARTESIAN_POINT('Origin',(-4.11365584262083,83.8,-117.131229900105));
#64483=CARTESIAN_POINT('',(-4.11365584262083,83.8,-117.131229900105));
#64484=CARTESIAN_POINT('Origin',(-1.85852429730951,83.8,-115.32908810583));
#64485=CARTESIAN_POINT('Origin',(-9.27597994751136,83.8,-109.742020887223));
#64486=CARTESIAN_POINT('',(-9.27597994751136,83.8,-109.742020887223));
#64487=CARTESIAN_POINT('',(-8.84284514510264,83.8,-112.596092991476));
#64488=CARTESIAN_POINT('Origin',(-11.9642462952314,83.8,-108.690090577245));
#64489=CARTESIAN_POINT('',(-11.9642462952314,83.8,-108.690090577245));
#64490=CARTESIAN_POINT('Origin',(-14.2193778405427,83.8,-110.492232371521));
#64491=CARTESIAN_POINT('',(-14.2193778405427,83.8,-110.492232371521));
#64492=CARTESIAN_POINT('Origin',(-13.786243038134,83.8,-113.346304475774));
#64493=CARTESIAN_POINT('',(-13.786243038134,83.8,-113.346304475774));
#64494=CARTESIAN_POINT('Origin',(-11.097976690414,83.8,-114.398234785752));
#64495=CARTESIAN_POINT('',(-11.097976690414,83.8,-114.398234785752));
#64496=CARTESIAN_POINT('Origin',(-8.84284514510264,83.8,-112.596092991476));
#64497=CARTESIAN_POINT('Origin',(-16.2603007953045,83.8,-107.009025772869));
#64498=CARTESIAN_POINT('',(-16.2603007953045,83.8,-107.009025772869));
#64499=CARTESIAN_POINT('',(-15.8271659928958,83.8,-109.863097877122));
#64500=CARTESIAN_POINT('Origin',(-18.9485671430245,83.8,-105.957095462892));
#64501=CARTESIAN_POINT('',(-18.9485671430245,83.8,-105.957095462892));
#64502=CARTESIAN_POINT('Origin',(-21.2036986883359,83.8,-107.759237257167));
#64503=CARTESIAN_POINT('',(-21.2036986883359,83.8,-107.759237257167));
#64504=CARTESIAN_POINT('Origin',(-20.7705638859271,83.8,-110.61330936142));
#64505=CARTESIAN_POINT('',(-20.7705638859271,83.8,-110.61330936142));
#64506=CARTESIAN_POINT('Origin',(-18.0822975382071,83.8,-111.665239671398));
#64507=CARTESIAN_POINT('',(-18.0822975382071,83.8,-111.665239671398));
#64508=CARTESIAN_POINT('Origin',(-15.8271659928958,83.8,-109.863097877122));
#64509=CARTESIAN_POINT('Origin',(-23.2446216430976,83.8,-104.276030658515));
#64510=CARTESIAN_POINT('',(-23.2446216430976,83.8,-104.276030658515));
#64511=CARTESIAN_POINT('',(-22.8114868406889,83.8,-107.130102762768));
#64512=CARTESIAN_POINT('Origin',(-25.9328879908176,83.8,-103.224100348538));
#64513=CARTESIAN_POINT('',(-25.9328879908176,83.8,-103.224100348538));
#64514=CARTESIAN_POINT('Origin',(-28.188019536129,83.8,-105.026242142813));
#64515=CARTESIAN_POINT('',(-28.188019536129,83.8,-105.026242142813));
#64516=CARTESIAN_POINT('Origin',(-27.7548847337203,83.8,-107.880314247066));
#64517=CARTESIAN_POINT('',(-27.7548847337203,83.8,-107.880314247066));
#64518=CARTESIAN_POINT('Origin',(-25.0666183860002,83.8,-108.932244557044));
#64519=CARTESIAN_POINT('',(-25.0666183860002,83.8,-108.932244557044));
#64520=CARTESIAN_POINT('Origin',(-22.8114868406889,83.8,-107.130102762768));
#64521=CARTESIAN_POINT('Origin',(-24.1375213804361,83.8,-55.1033478960396));
#64522=CARTESIAN_POINT('',(-24.1375213804361,83.8,-55.1033478960396));
#64523=CARTESIAN_POINT('',(-23.7043865780274,83.8,-57.9574200002927));
#64524=CARTESIAN_POINT('Origin',(-26.8257877281561,83.8,-54.0514175860622));
#64525=CARTESIAN_POINT('',(-26.8257877281561,83.8,-54.0514175860622));
#64526=CARTESIAN_POINT('Origin',(-29.0809192734675,83.8,-55.8535593803378));
#64527=CARTESIAN_POINT('',(-29.0809192734675,83.8,-55.8535593803378));
#64528=CARTESIAN_POINT('Origin',(-28.6477844710588,83.8,-58.7076314845909));
#64529=CARTESIAN_POINT('',(-28.6477844710588,83.8,-58.7076314845909));
#64530=CARTESIAN_POINT('Origin',(-25.9595181233387,83.8,-59.7595617945683));
#64531=CARTESIAN_POINT('',(-25.9595181233387,83.8,-59.7595617945683));
#64532=CARTESIAN_POINT('Origin',(-23.7043865780274,83.8,-57.9574200002927));
#64533=CARTESIAN_POINT('Origin',(-31.1218422282293,83.8,-52.3703527816857));
#64534=CARTESIAN_POINT('',(-31.1218422282293,83.8,-52.3703527816857));
#64535=CARTESIAN_POINT('',(-30.6887074258205,83.8,-55.2244248859388));
#64536=CARTESIAN_POINT('Origin',(-33.8101085759493,83.8,-51.3184224717083));
#64537=CARTESIAN_POINT('',(-33.8101085759493,83.8,-51.3184224717083));
#64538=CARTESIAN_POINT('Origin',(-36.0652401212606,83.8,-53.120564265984));
#64539=CARTESIAN_POINT('',(-36.0652401212606,83.8,-53.120564265984));
#64540=CARTESIAN_POINT('Origin',(-35.6321053188519,83.8,-55.974636370237));
#64541=CARTESIAN_POINT('',(-35.6321053188519,83.8,-55.974636370237));
#64542=CARTESIAN_POINT('Origin',(-32.9438389711319,83.8,-57.0265666802144));
#64543=CARTESIAN_POINT('',(-32.9438389711319,83.8,-57.0265666802144));
#64544=CARTESIAN_POINT('Origin',(-30.6887074258205,83.8,-55.2244248859388));
#64545=CARTESIAN_POINT('Origin',(-38.1061630760224,83.8,-49.6373576673318));
#64546=CARTESIAN_POINT('',(-38.1061630760224,83.8,-49.6373576673318));
#64547=CARTESIAN_POINT('',(-37.6730282736137,83.8,-52.4914297715849));
#64548=CARTESIAN_POINT('Origin',(-40.7944294237424,83.8,-48.5854273573544));
#64549=CARTESIAN_POINT('',(-40.7944294237424,83.8,-48.5854273573544));
#64550=CARTESIAN_POINT('Origin',(-43.0495609690538,83.8,-50.3875691516301));
#64551=CARTESIAN_POINT('',(-43.0495609690538,83.8,-50.3875691516301));
#64552=CARTESIAN_POINT('Origin',(-42.616426166645,83.8,-53.2416412558831));
#64553=CARTESIAN_POINT('',(-42.616426166645,83.8,-53.2416412558831));
#64554=CARTESIAN_POINT('Origin',(-39.928159818925,83.8,-54.2935715658606));
#64555=CARTESIAN_POINT('',(-39.928159818925,83.8,-54.2935715658606));
#64556=CARTESIAN_POINT('Origin',(-37.6730282736137,83.8,-52.4914297715849));
#64557=CARTESIAN_POINT('Origin',(46.8310043239425,83.8,-89.8483958791255));
#64558=CARTESIAN_POINT('',(46.8310043239425,83.8,-89.8483958791255));
#64559=CARTESIAN_POINT('',(47.2641391263513,83.8,-92.7024679833786));
#64560=CARTESIAN_POINT('Origin',(44.1427379762225,83.8,-88.7964655691481));
#64561=CARTESIAN_POINT('',(44.1427379762225,83.8,-88.7964655691481));
#64562=CARTESIAN_POINT('Origin',(41.8876064309112,83.8,-90.5986073634238));
#64563=CARTESIAN_POINT('',(41.8876064309112,83.8,-90.5986073634238));
#64564=CARTESIAN_POINT('Origin',(42.3207412333199,83.8,-93.4526794676769));
#64565=CARTESIAN_POINT('',(42.3207412333199,83.8,-93.4526794676769));
#64566=CARTESIAN_POINT('Origin',(45.0090075810399,83.8,-94.5046097776543));
#64567=CARTESIAN_POINT('',(45.0090075810399,83.8,-94.5046097776543));
#64568=CARTESIAN_POINT('Origin',(47.2641391263513,83.8,-92.7024679833786));
#64569=CARTESIAN_POINT('Origin',(-17.153200532643,83.8,-57.8363430103935));
#64570=CARTESIAN_POINT('',(-17.153200532643,83.8,-57.8363430103935));
#64571=CARTESIAN_POINT('',(-16.7200657302343,83.8,-60.6904151146466));
#64572=CARTESIAN_POINT('Origin',(-19.841466880363,83.8,-56.784412700416));
#64573=CARTESIAN_POINT('',(-19.841466880363,83.8,-56.784412700416));
#64574=CARTESIAN_POINT('Origin',(-22.0965984256744,83.8,-58.5865544946917));
#64575=CARTESIAN_POINT('',(-22.0965984256744,83.8,-58.5865544946917));
#64576=CARTESIAN_POINT('Origin',(-21.6634636232656,83.8,-61.4406265989448));
#64577=CARTESIAN_POINT('',(-21.6634636232656,83.8,-61.4406265989448));
#64578=CARTESIAN_POINT('Origin',(-18.9751972755456,83.8,-62.4925569089222));
#64579=CARTESIAN_POINT('',(-18.9751972755456,83.8,-62.4925569089222));
#64580=CARTESIAN_POINT('Origin',(-16.7200657302343,83.8,-60.6904151146466));
#64581=CARTESIAN_POINT('Origin',(-10.1688796848499,83.8,-60.5693381247473));
#64582=CARTESIAN_POINT('',(-10.1688796848499,83.8,-60.5693381247473));
#64583=CARTESIAN_POINT('',(-9.73574488244115,83.8,-63.4234102290004));
#64584=CARTESIAN_POINT('Origin',(-12.8571460325699,83.8,-59.5174078147699));
#64585=CARTESIAN_POINT('',(-12.8571460325699,83.8,-59.5174078147699));
#64586=CARTESIAN_POINT('Origin',(-15.1122775778812,83.8,-61.3195496090456));
#64587=CARTESIAN_POINT('',(-15.1122775778812,83.8,-61.3195496090456));
#64588=CARTESIAN_POINT('Origin',(-14.6791427754725,83.8,-64.1736217132987));
#64589=CARTESIAN_POINT('',(-14.6791427754725,83.8,-64.1736217132987));
#64590=CARTESIAN_POINT('Origin',(-11.9908764277525,83.8,-65.2255520232761));
#64591=CARTESIAN_POINT('',(-11.9908764277525,83.8,-65.2255520232761));
#64592=CARTESIAN_POINT('Origin',(-9.73574488244115,83.8,-63.4234102290004));
#64593=CARTESIAN_POINT('Origin',(-3.18455883705674,83.8,-63.3023332391012));
#64594=CARTESIAN_POINT('',(-3.18455883705674,83.8,-63.3023332391012));
#64595=CARTESIAN_POINT('',(-2.75142403464802,83.8,-66.1564053433543));
#64596=CARTESIAN_POINT('Origin',(-5.87282518477675,83.8,-62.2504029291238));
#64597=CARTESIAN_POINT('',(-5.87282518477675,83.8,-62.2504029291238));
#64598=CARTESIAN_POINT('Origin',(-8.1279567300881,83.8,-64.0525447233995));
#64599=CARTESIAN_POINT('',(-8.1279567300881,83.8,-64.0525447233995));
#64600=CARTESIAN_POINT('Origin',(-7.69482192767937,83.8,-66.9066168276526));
#64601=CARTESIAN_POINT('',(-7.69482192767937,83.8,-66.9066168276526));
#64602=CARTESIAN_POINT('Origin',(-5.00655557995934,83.8,-67.95854713763));
#64603=CARTESIAN_POINT('',(-5.00655557995934,83.8,-67.95854713763));
#64604=CARTESIAN_POINT('Origin',(-2.75142403464802,83.8,-66.1564053433543));
#64605=CARTESIAN_POINT('Origin',(3.7997620107364,83.8,-66.0353283534551));
#64606=CARTESIAN_POINT('',(3.7997620107364,83.8,-66.0353283534551));
#64607=CARTESIAN_POINT('',(4.23289681314511,83.8,-68.8894004577082));
#64608=CARTESIAN_POINT('Origin',(1.11149566301639,83.8,-64.9833980434777));
#64609=CARTESIAN_POINT('',(1.11149566301639,83.8,-64.9833980434777));
#64610=CARTESIAN_POINT('Origin',(-1.14363588229497,83.8,-66.7855398377534));
#64611=CARTESIAN_POINT('',(-1.14363588229497,83.8,-66.7855398377534));
#64612=CARTESIAN_POINT('Origin',(-0.710501079886239,83.8,-69.6396119420065));
#64613=CARTESIAN_POINT('',(-0.710501079886239,83.8,-69.6396119420065));
#64614=CARTESIAN_POINT('Origin',(1.97776526783379,83.8,-70.6915422519839));
#64615=CARTESIAN_POINT('',(1.97776526783379,83.8,-70.6915422519839));
#64616=CARTESIAN_POINT('Origin',(4.23289681314511,83.8,-68.8894004577082));
#64617=CARTESIAN_POINT('Origin',(39.8466834761494,83.8,-87.1154007647716));
#64618=CARTESIAN_POINT('',(39.8466834761494,83.8,-87.1154007647716));
#64619=CARTESIAN_POINT('',(40.2798182785581,83.8,-89.9694728690247));
#64620=CARTESIAN_POINT('Origin',(37.1584171284294,83.8,-86.0634704547942));
#64621=CARTESIAN_POINT('',(37.1584171284294,83.8,-86.0634704547942));
#64622=CARTESIAN_POINT('Origin',(34.903285583118,83.8,-87.8656122490699));
#64623=CARTESIAN_POINT('',(34.903285583118,83.8,-87.8656122490699));
#64624=CARTESIAN_POINT('Origin',(35.3364203855268,83.8,-90.719684353323));
#64625=CARTESIAN_POINT('',(35.3364203855268,83.8,-90.719684353323));
#64626=CARTESIAN_POINT('Origin',(38.0246867332468,83.8,-91.7716146633004));
#64627=CARTESIAN_POINT('',(38.0246867332468,83.8,-91.7716146633004));
#64628=CARTESIAN_POINT('Origin',(40.2798182785581,83.8,-89.9694728690247));
#64629=CARTESIAN_POINT('Origin',(32.8623626283563,83.8,-84.3824056504177));
#64630=CARTESIAN_POINT('',(32.8623626283563,83.8,-84.3824056504177));
#64631=CARTESIAN_POINT('',(33.295497430765,83.8,-87.2364777546708));
#64632=CARTESIAN_POINT('Origin',(30.1740962806363,83.8,-83.3304753404403));
#64633=CARTESIAN_POINT('',(30.1740962806363,83.8,-83.3304753404403));
#64634=CARTESIAN_POINT('Origin',(27.9189647353249,83.8,-85.132617134716));
#64635=CARTESIAN_POINT('',(27.9189647353249,83.8,-85.132617134716));
#64636=CARTESIAN_POINT('Origin',(28.3520995377337,83.8,-87.9866892389691));
#64637=CARTESIAN_POINT('',(28.3520995377337,83.8,-87.9866892389691));
#64638=CARTESIAN_POINT('Origin',(31.0403658854537,83.8,-89.0386195489465));
#64639=CARTESIAN_POINT('',(31.0403658854537,83.8,-89.0386195489465));
#64640=CARTESIAN_POINT('Origin',(33.295497430765,83.8,-87.2364777546708));
#64641=CARTESIAN_POINT('Origin',(25.8780417805632,83.8,-81.6494105360638));
#64642=CARTESIAN_POINT('',(25.8780417805632,83.8,-81.6494105360638));
#64643=CARTESIAN_POINT('',(26.3111765829719,83.8,-84.5034826403169));
#64644=CARTESIAN_POINT('Origin',(23.1897754328432,83.8,-80.5974802260864));
#64645=CARTESIAN_POINT('',(23.1897754328432,83.8,-80.5974802260864));
#64646=CARTESIAN_POINT('Origin',(20.9346438875318,83.8,-82.3996220203621));
#64647=CARTESIAN_POINT('',(20.9346438875318,83.8,-82.3996220203621));
#64648=CARTESIAN_POINT('Origin',(21.3677786899405,83.8,-85.2536941246152));
#64649=CARTESIAN_POINT('',(21.3677786899405,83.8,-85.2536941246152));
#64650=CARTESIAN_POINT('Origin',(24.0560450376606,83.8,-86.3056244345926));
#64651=CARTESIAN_POINT('',(24.0560450376606,83.8,-86.3056244345926));
#64652=CARTESIAN_POINT('Origin',(26.3111765829719,83.8,-84.5034826403169));
#64653=CARTESIAN_POINT('Origin',(18.89372093277,83.8,-78.9164154217099));
#64654=CARTESIAN_POINT('',(18.89372093277,83.8,-78.9164154217099));
#64655=CARTESIAN_POINT('',(19.3268557351787,83.8,-81.770487525963));
#64656=CARTESIAN_POINT('Origin',(16.20545458505,83.8,-77.8644851117325));
#64657=CARTESIAN_POINT('',(16.20545458505,83.8,-77.8644851117325));
#64658=CARTESIAN_POINT('Origin',(13.9503230397387,83.8,-79.6666269060082));
#64659=CARTESIAN_POINT('',(13.9503230397387,83.8,-79.6666269060082));
#64660=CARTESIAN_POINT('Origin',(14.3834578421474,83.8,-82.5206990102613));
#64661=CARTESIAN_POINT('',(14.3834578421474,83.8,-82.5206990102613));
#64662=CARTESIAN_POINT('Origin',(17.0717241898674,83.8,-83.5726293202387));
#64663=CARTESIAN_POINT('',(17.0717241898674,83.8,-83.5726293202387));
#64664=CARTESIAN_POINT('Origin',(19.3268557351787,83.8,-81.770487525963));
#64665=CARTESIAN_POINT('Origin',(11.9094000849769,83.8,-76.1834203073561));
#64666=CARTESIAN_POINT('',(11.9094000849769,83.8,-76.1834203073561));
#64667=CARTESIAN_POINT('',(12.3425348873856,83.8,-79.0374924116092));
#64668=CARTESIAN_POINT('Origin',(9.22113373725689,83.8,-75.1314899973787));
#64669=CARTESIAN_POINT('',(9.22113373725689,83.8,-75.1314899973787));
#64670=CARTESIAN_POINT('Origin',(6.96600219194553,83.8,-76.9336317916543));
#64671=CARTESIAN_POINT('',(6.96600219194553,83.8,-76.9336317916543));
#64672=CARTESIAN_POINT('Origin',(7.39913699435427,83.8,-79.7877038959074));
#64673=CARTESIAN_POINT('',(7.39913699435427,83.8,-79.7877038959074));
#64674=CARTESIAN_POINT('Origin',(10.0874033420743,83.8,-80.8396342058848));
#64675=CARTESIAN_POINT('',(10.0874033420743,83.8,-80.8396342058848));
#64676=CARTESIAN_POINT('Origin',(12.3425348873856,83.8,-79.0374924116092));
#64677=CARTESIAN_POINT('Origin',(4.92507923718377,83.8,-73.4504251930022));
#64678=CARTESIAN_POINT('',(4.92507923718377,83.8,-73.4504251930022));
#64679=CARTESIAN_POINT('',(5.35821403959249,83.8,-76.3044972972553));
#64680=CARTESIAN_POINT('Origin',(2.23681288946376,83.8,-72.3984948830248));
#64681=CARTESIAN_POINT('',(2.23681288946376,83.8,-72.3984948830248));
#64682=CARTESIAN_POINT('Origin',(-0.0183186558475948,83.8,-74.2006366773005));
#64683=CARTESIAN_POINT('',(-0.0183186558475948,83.8,-74.2006366773005));
#64684=CARTESIAN_POINT('Origin',(0.414816146561137,83.8,-77.0547087815535));
#64685=CARTESIAN_POINT('',(0.414816146561137,83.8,-77.0547087815535));
#64686=CARTESIAN_POINT('Origin',(3.10308249428116,83.8,-78.1066390915309));
#64687=CARTESIAN_POINT('',(3.10308249428116,83.8,-78.1066390915309));
#64688=CARTESIAN_POINT('Origin',(5.35821403959249,83.8,-76.3044972972553));
#64689=CARTESIAN_POINT('Origin',(-2.05924161060936,83.8,-70.7174300786483));
#64690=CARTESIAN_POINT('',(-2.05924161060936,83.8,-70.7174300786483));
#64691=CARTESIAN_POINT('',(-1.62610680820064,83.8,-73.5715021829014));
#64692=CARTESIAN_POINT('Origin',(-4.74750795832937,83.8,-69.6654997686709));
#64693=CARTESIAN_POINT('',(-4.74750795832937,83.8,-69.6654997686709));
#64694=CARTESIAN_POINT('Origin',(-7.00263950364073,83.8,-71.4676415629466));
#64695=CARTESIAN_POINT('',(-7.00263950364073,83.8,-71.4676415629466));
#64696=CARTESIAN_POINT('Origin',(-6.569504701232,83.8,-74.3217136671996));
#64697=CARTESIAN_POINT('',(-6.569504701232,83.8,-74.3217136671996));
#64698=CARTESIAN_POINT('Origin',(-3.88123835351197,83.8,-75.3736439771771));
#64699=CARTESIAN_POINT('',(-3.88123835351197,83.8,-75.3736439771771));
#64700=CARTESIAN_POINT('Origin',(-1.62610680820064,83.8,-73.5715021829014));
#64701=CARTESIAN_POINT('Origin',(-9.04356245840249,83.8,-67.9844349642944));
#64702=CARTESIAN_POINT('',(-9.04356245840249,83.8,-67.9844349642944));
#64703=CARTESIAN_POINT('',(-8.61042765599378,83.8,-70.8385070685475));
#64704=CARTESIAN_POINT('Origin',(-11.7318288061225,83.8,-66.932504654317));
#64705=CARTESIAN_POINT('',(-11.7318288061225,83.8,-66.932504654317));
#64706=CARTESIAN_POINT('Origin',(-13.9869603514339,83.8,-68.7346464485927));
#64707=CARTESIAN_POINT('',(-13.9869603514339,83.8,-68.7346464485927));
#64708=CARTESIAN_POINT('Origin',(-13.5538255490251,83.8,-71.5887185528457));
#64709=CARTESIAN_POINT('',(-13.5538255490251,83.8,-71.5887185528457));
#64710=CARTESIAN_POINT('Origin',(-10.8655592013051,83.8,-72.6406488628232));
#64711=CARTESIAN_POINT('',(-10.8655592013051,83.8,-72.6406488628232));
#64712=CARTESIAN_POINT('Origin',(-8.61042765599378,83.8,-70.8385070685475));
#64713=CARTESIAN_POINT('Origin',(16.6430864798753,83.8,-64.0862217426158));
#64714=CARTESIAN_POINT('',(16.6430864798753,83.8,-64.0862217426158));
#64715=CARTESIAN_POINT('',(17.076221282284,83.8,-66.940293846869));
#64716=CARTESIAN_POINT('Origin',(13.9548201321553,83.8,-63.0342914326384));
#64717=CARTESIAN_POINT('',(13.9548201321553,83.8,-63.0342914326384));
#64718=CARTESIAN_POINT('Origin',(11.6996885868439,83.8,-64.8364332269141));
#64719=CARTESIAN_POINT('',(11.6996885868439,83.8,-64.8364332269141));
#64720=CARTESIAN_POINT('Origin',(12.1328233892526,83.8,-67.6905053311672));
#64721=CARTESIAN_POINT('',(12.1328233892526,83.8,-67.6905053311672));
#64722=CARTESIAN_POINT('Origin',(14.8210897369727,83.8,-68.7424356411446));
#64723=CARTESIAN_POINT('',(14.8210897369727,83.8,-68.7424356411446));
#64724=CARTESIAN_POINT('Origin',(17.076221282284,83.8,-66.940293846869));
#64725=CARTESIAN_POINT('Origin',(9.65876563208215,83.8,-61.353226628262));
#64726=CARTESIAN_POINT('',(9.65876563208215,83.8,-61.353226628262));
#64727=CARTESIAN_POINT('',(10.0919004344909,83.8,-64.2072987325151));
#64728=CARTESIAN_POINT('Origin',(6.97049928436214,83.8,-60.3012963182845));
#64729=CARTESIAN_POINT('',(6.97049928436214,83.8,-60.3012963182845));
#64730=CARTESIAN_POINT('Origin',(4.71536773905078,83.8,-62.1034381125602));
#64731=CARTESIAN_POINT('',(4.71536773905078,83.8,-62.1034381125602));
#64732=CARTESIAN_POINT('Origin',(5.14850254145952,83.8,-64.9575102168133));
#64733=CARTESIAN_POINT('',(5.14850254145952,83.8,-64.9575102168133));
#64734=CARTESIAN_POINT('Origin',(7.83676888917954,83.8,-66.0094405267907));
#64735=CARTESIAN_POINT('',(7.83676888917954,83.8,-66.0094405267907));
#64736=CARTESIAN_POINT('Origin',(10.0919004344909,83.8,-64.2072987325151));
#64737=CARTESIAN_POINT('Origin',(2.67444478428902,83.8,-58.6202315139081));
#64738=CARTESIAN_POINT('',(2.67444478428902,83.8,-58.6202315139081));
#64739=CARTESIAN_POINT('',(3.10757958669774,83.8,-61.4743036181612));
#64740=CARTESIAN_POINT('Origin',(-0.0138215634309935,83.8,-57.5683012039307));
#64741=CARTESIAN_POINT('',(-0.0138215634309935,83.8,-57.5683012039307));
#64742=CARTESIAN_POINT('Origin',(-2.26895310874235,83.8,-59.3704429982063));
#64743=CARTESIAN_POINT('',(-2.26895310874235,83.8,-59.3704429982063));
#64744=CARTESIAN_POINT('Origin',(-1.83581830633362,83.8,-62.2245151024594));
#64745=CARTESIAN_POINT('',(-1.83581830633362,83.8,-62.2245151024594));
#64746=CARTESIAN_POINT('Origin',(0.852448041386411,83.8,-63.2764454124368));
#64747=CARTESIAN_POINT('',(0.852448041386411,83.8,-63.2764454124368));
#64748=CARTESIAN_POINT('Origin',(3.10757958669774,83.8,-61.4743036181612));
#64749=CARTESIAN_POINT('Origin',(-4.30987606350412,83.8,-55.8872363995542));
#64750=CARTESIAN_POINT('',(-4.30987606350412,83.8,-55.8872363995542));
#64751=CARTESIAN_POINT('',(-3.8767412610954,83.8,-58.7413085038073));
#64752=CARTESIAN_POINT('Origin',(-6.99814241122413,83.8,-54.8353060895768));
#64753=CARTESIAN_POINT('',(-6.99814241122413,83.8,-54.8353060895768));
#64754=CARTESIAN_POINT('Origin',(-9.25327395653548,83.8,-56.6374478838525));
#64755=CARTESIAN_POINT('',(-9.25327395653548,83.8,-56.6374478838525));
#64756=CARTESIAN_POINT('Origin',(-8.82013915412675,83.8,-59.4915199881055));
#64757=CARTESIAN_POINT('',(-8.82013915412675,83.8,-59.4915199881055));
#64758=CARTESIAN_POINT('Origin',(-6.13187280640672,83.8,-60.543450298083));
#64759=CARTESIAN_POINT('',(-6.13187280640672,83.8,-60.543450298083));
#64760=CARTESIAN_POINT('Origin',(-3.8767412610954,83.8,-58.7413085038073));
#64761=CARTESIAN_POINT('Origin',(-11.2941969112972,83.8,-53.1542412852003));
#64762=CARTESIAN_POINT('',(-11.2941969112972,83.8,-53.1542412852003));
#64763=CARTESIAN_POINT('',(-10.8610621088885,83.8,-56.0083133894534));
#64764=CARTESIAN_POINT('Origin',(-13.9824632590173,83.8,-52.1023109752229));
#64765=CARTESIAN_POINT('',(-13.9824632590173,83.8,-52.1023109752229));
#64766=CARTESIAN_POINT('Origin',(-16.2375948043286,83.8,-53.9044527694986));
#64767=CARTESIAN_POINT('',(-16.2375948043286,83.8,-53.9044527694986));
#64768=CARTESIAN_POINT('Origin',(-15.8044600019199,83.8,-56.7585248737516));
#64769=CARTESIAN_POINT('',(-15.8044600019199,83.8,-56.7585248737516));
#64770=CARTESIAN_POINT('Origin',(-13.1161936541999,83.8,-57.8104551837291));
#64771=CARTESIAN_POINT('',(-13.1161936541999,83.8,-57.8104551837291));
#64772=CARTESIAN_POINT('Origin',(-10.8610621088885,83.8,-56.0083133894534));
#64773=CARTESIAN_POINT('Origin',(-18.2785177590904,83.8,-50.4212461708464));
#64774=CARTESIAN_POINT('',(-18.2785177590904,83.8,-50.4212461708464));
#64775=CARTESIAN_POINT('',(-17.8453829566817,83.8,-53.2753182750995));
#64776=CARTESIAN_POINT('Origin',(-20.9667841068104,83.8,-49.369315860869));
#64777=CARTESIAN_POINT('',(-20.9667841068104,83.8,-49.369315860869));
#64778=CARTESIAN_POINT('Origin',(-23.2219156521217,83.8,-51.1714576551447));
#64779=CARTESIAN_POINT('',(-23.2219156521217,83.8,-51.1714576551447));
#64780=CARTESIAN_POINT('Origin',(-22.788780849713,83.8,-54.0255297593977));
#64781=CARTESIAN_POINT('',(-22.788780849713,83.8,-54.0255297593977));
#64782=CARTESIAN_POINT('Origin',(-20.100514501993,83.8,-55.0774600693752));
#64783=CARTESIAN_POINT('',(-20.100514501993,83.8,-55.0774600693752));
#64784=CARTESIAN_POINT('Origin',(-17.8453829566817,83.8,-53.2753182750995));
#64785=CARTESIAN_POINT('Origin',(-25.2628386068835,83.8,-47.6882510564925));
#64786=CARTESIAN_POINT('',(-25.2628386068835,83.8,-47.6882510564925));
#64787=CARTESIAN_POINT('',(-24.8297038044748,83.8,-50.5423231607456));
#64788=CARTESIAN_POINT('Origin',(-27.9511049546035,83.8,-46.6363207465151));
#64789=CARTESIAN_POINT('',(-27.9511049546035,83.8,-46.6363207465151));
#64790=CARTESIAN_POINT('Origin',(-30.2062364999149,83.8,-48.4384625407908));
#64791=CARTESIAN_POINT('',(-30.2062364999149,83.8,-48.4384625407908));
#64792=CARTESIAN_POINT('Origin',(-29.7731016975061,83.8,-51.2925346450439));
#64793=CARTESIAN_POINT('',(-29.7731016975061,83.8,-51.2925346450439));
#64794=CARTESIAN_POINT('Origin',(-27.0848353497861,83.8,-52.3444649550213));
#64795=CARTESIAN_POINT('',(-27.0848353497861,83.8,-52.3444649550213));
#64796=CARTESIAN_POINT('Origin',(-24.8297038044748,83.8,-50.5423231607456));
#64797=CARTESIAN_POINT('Origin',(-32.2471594546766,83.8,-44.9552559421386));
#64798=CARTESIAN_POINT('',(-32.2471594546766,83.8,-44.9552559421386));
#64799=CARTESIAN_POINT('',(-31.8140246522679,83.8,-47.8093280463917));
#64800=CARTESIAN_POINT('Origin',(-34.9354258023966,83.8,-43.9033256321612));
#64801=CARTESIAN_POINT('',(-34.9354258023966,83.8,-43.9033256321612));
#64802=CARTESIAN_POINT('Origin',(-37.190557347708,83.8,-45.7054674264369));
#64803=CARTESIAN_POINT('',(-37.190557347708,83.8,-45.7054674264369));
#64804=CARTESIAN_POINT('Origin',(-36.7574225452993,83.8,-48.55953953069));
#64805=CARTESIAN_POINT('',(-36.7574225452993,83.8,-48.55953953069));
#64806=CARTESIAN_POINT('Origin',(-34.0691561975792,83.8,-49.6114698406674));
#64807=CARTESIAN_POINT('',(-34.0691561975792,83.8,-49.6114698406674));
#64808=CARTESIAN_POINT('Origin',(-31.8140246522679,83.8,-47.8093280463917));
#64809=CARTESIAN_POINT('Origin',(10.7840828585295,83.8,-68.768323467809));
#64810=CARTESIAN_POINT('',(10.7840828585295,83.8,-68.768323467809));
#64811=CARTESIAN_POINT('',(11.2172176609382,83.8,-71.6223955720621));
#64812=CARTESIAN_POINT('Origin',(8.09581651080951,83.8,-67.7163931578316));
#64813=CARTESIAN_POINT('',(8.09581651080951,83.8,-67.7163931578316));
#64814=CARTESIAN_POINT('Origin',(5.84068496549816,83.8,-69.5185349521073));
#64815=CARTESIAN_POINT('',(5.84068496549816,83.8,-69.5185349521073));
#64816=CARTESIAN_POINT('Origin',(6.27381976790689,83.8,-72.3726070563604));
#64817=CARTESIAN_POINT('',(6.27381976790689,83.8,-72.3726070563604));
#64818=CARTESIAN_POINT('Origin',(8.96208611562692,83.8,-73.4245373663378));
#64819=CARTESIAN_POINT('',(8.96208611562692,83.8,-73.4245373663378));
#64820=CARTESIAN_POINT('Origin',(11.2172176609382,83.8,-71.6223955720621));
#64821=CARTESIAN_POINT('Origin',(17.7684037063227,83.8,-71.5013185821629));
#64822=CARTESIAN_POINT('',(17.7684037063227,83.8,-71.5013185821629));
#64823=CARTESIAN_POINT('',(18.2015385087314,83.8,-74.355390686416));
#64824=CARTESIAN_POINT('Origin',(15.0801373586026,83.8,-70.4493882721855));
#64825=CARTESIAN_POINT('',(15.0801373586026,83.8,-70.4493882721855));
#64826=CARTESIAN_POINT('Origin',(12.8250058132913,83.8,-72.2515300664612));
#64827=CARTESIAN_POINT('',(12.8250058132913,83.8,-72.2515300664612));
#64828=CARTESIAN_POINT('Origin',(13.2581406157,83.8,-75.1056021707142));
#64829=CARTESIAN_POINT('',(13.2581406157,83.8,-75.1056021707142));
#64830=CARTESIAN_POINT('Origin',(15.94640696342,83.8,-76.1575324806917));
#64831=CARTESIAN_POINT('',(15.94640696342,83.8,-76.1575324806917));
#64832=CARTESIAN_POINT('Origin',(18.2015385087314,83.8,-74.355390686416));
#64833=CARTESIAN_POINT('Origin',(24.7527245541158,83.8,-74.2343136965168));
#64834=CARTESIAN_POINT('',(24.7527245541158,83.8,-74.2343136965168));
#64835=CARTESIAN_POINT('',(25.1858593565245,83.8,-77.0883858007699));
#64836=CARTESIAN_POINT('Origin',(22.0644582063958,83.8,-73.1823833865394));
#64837=CARTESIAN_POINT('',(22.0644582063958,83.8,-73.1823833865394));
#64838=CARTESIAN_POINT('Origin',(19.8093266610844,83.8,-74.9845251808151));
#64839=CARTESIAN_POINT('',(19.8093266610844,83.8,-74.9845251808151));
#64840=CARTESIAN_POINT('Origin',(20.2424614634932,83.8,-77.8385972850681));
#64841=CARTESIAN_POINT('',(20.2424614634932,83.8,-77.8385972850681));
#64842=CARTESIAN_POINT('Origin',(22.9307278112132,83.8,-78.8905275950456));
#64843=CARTESIAN_POINT('',(22.9307278112132,83.8,-78.8905275950456));
#64844=CARTESIAN_POINT('Origin',(25.1858593565245,83.8,-77.0883858007699));
#64845=CARTESIAN_POINT('Origin',(31.7370454019089,83.8,-76.9673088108707));
#64846=CARTESIAN_POINT('',(31.7370454019089,83.8,-76.9673088108707));
#64847=CARTESIAN_POINT('',(32.1701802043176,83.8,-79.8213809151238));
#64848=CARTESIAN_POINT('Origin',(29.0487790541889,83.8,-75.9153785008933));
#64849=CARTESIAN_POINT('',(29.0487790541889,83.8,-75.9153785008933));
#64850=CARTESIAN_POINT('Origin',(26.7936475088776,83.8,-77.717520295169));
#64851=CARTESIAN_POINT('',(26.7936475088776,83.8,-77.717520295169));
#64852=CARTESIAN_POINT('Origin',(27.2267823112863,83.8,-80.571592399422));
#64853=CARTESIAN_POINT('',(27.2267823112863,83.8,-80.571592399422));
#64854=CARTESIAN_POINT('Origin',(29.9150486590063,83.8,-81.6235227093995));
#64855=CARTESIAN_POINT('',(29.9150486590063,83.8,-81.6235227093995));
#64856=CARTESIAN_POINT('Origin',(32.1701802043176,83.8,-79.8213809151238));
#64857=CARTESIAN_POINT('Origin',(-39.2314803024698,83.8,-42.2222608277847));
#64858=CARTESIAN_POINT('',(-39.2314803024698,83.8,-42.2222608277847));
#64859=CARTESIAN_POINT('',(-38.798345500061,83.8,-45.0763329320378));
#64860=CARTESIAN_POINT('Origin',(-41.9197466501898,83.8,-41.1703305178073));
#64861=CARTESIAN_POINT('',(-41.9197466501898,83.8,-41.1703305178073));
#64862=CARTESIAN_POINT('Origin',(-44.1748781955011,83.8,-42.972472312083));
#64863=CARTESIAN_POINT('',(-44.1748781955011,83.8,-42.972472312083));
#64864=CARTESIAN_POINT('Origin',(-43.7417433930924,83.8,-45.8265444163361));
#64865=CARTESIAN_POINT('',(-43.7417433930924,83.8,-45.8265444163361));
#64866=CARTESIAN_POINT('Origin',(-41.0534770453724,83.8,-46.8784747263135));
#64867=CARTESIAN_POINT('',(-41.0534770453724,83.8,-46.8784747263135));
#64868=CARTESIAN_POINT('Origin',(-38.798345500061,83.8,-45.0763329320378));
#64869=CARTESIAN_POINT('Origin',(52.6900079452883,83.8,-85.1662941539323));
#64870=CARTESIAN_POINT('',(52.6900079452883,83.8,-85.1662941539323));
#64871=CARTESIAN_POINT('',(53.123142747697,83.8,-88.0203662581854));
#64872=CARTESIAN_POINT('Origin',(50.0017415975683,83.8,-84.1143638439549));
#64873=CARTESIAN_POINT('',(50.0017415975683,83.8,-84.1143638439549));
#64874=CARTESIAN_POINT('Origin',(47.7466100522569,83.8,-85.9165056382306));
#64875=CARTESIAN_POINT('',(47.7466100522569,83.8,-85.9165056382306));
#64876=CARTESIAN_POINT('Origin',(48.1797448546657,83.8,-88.7705777424837));
#64877=CARTESIAN_POINT('',(48.1797448546657,83.8,-88.7705777424837));
#64878=CARTESIAN_POINT('Origin',(50.8680112023857,83.8,-89.8225080524611));
#64879=CARTESIAN_POINT('',(50.8680112023857,83.8,-89.8225080524611));
#64880=CARTESIAN_POINT('Origin',(53.123142747697,83.8,-88.0203662581854));
#64881=CARTESIAN_POINT('Origin',(45.7056870974952,83.8,-82.4332990395785));
#64882=CARTESIAN_POINT('',(45.7056870974952,83.8,-82.4332990395785));
#64883=CARTESIAN_POINT('',(46.1388218999039,83.8,-85.2873711438316));
#64884=CARTESIAN_POINT('Origin',(43.0174207497752,83.8,-81.381368729601));
#64885=CARTESIAN_POINT('',(43.0174207497752,83.8,-81.381368729601));
#64886=CARTESIAN_POINT('Origin',(40.7622892044638,83.8,-83.1835105238767));
#64887=CARTESIAN_POINT('',(40.7622892044638,83.8,-83.1835105238767));
#64888=CARTESIAN_POINT('Origin',(41.1954240068725,83.8,-86.0375826281298));
#64889=CARTESIAN_POINT('',(41.1954240068725,83.8,-86.0375826281298));
#64890=CARTESIAN_POINT('Origin',(43.8836903545926,83.8,-87.0895129381072));
#64891=CARTESIAN_POINT('',(43.8836903545926,83.8,-87.0895129381072));
#64892=CARTESIAN_POINT('Origin',(46.1388218999039,83.8,-85.2873711438316));
#64893=CARTESIAN_POINT('Origin',(38.721366249702,83.8,-79.7003039252246));
#64894=CARTESIAN_POINT('',(38.721366249702,83.8,-79.7003039252246));
#64895=CARTESIAN_POINT('',(39.1545010521108,83.8,-82.5543760294777));
#64896=CARTESIAN_POINT('Origin',(36.033099901982,83.8,-78.6483736152472));
#64897=CARTESIAN_POINT('',(36.033099901982,83.8,-78.6483736152472));
#64898=CARTESIAN_POINT('Origin',(33.7779683566707,83.8,-80.4505154095229));
#64899=CARTESIAN_POINT('',(33.7779683566707,83.8,-80.4505154095229));
#64900=CARTESIAN_POINT('Origin',(34.2111031590794,83.8,-83.3045875137759));
#64901=CARTESIAN_POINT('',(34.2111031590794,83.8,-83.3045875137759));
#64902=CARTESIAN_POINT('Origin',(36.8993695067994,83.8,-84.3565178237533));
#64903=CARTESIAN_POINT('',(36.8993695067994,83.8,-84.3565178237533));
#64904=CARTESIAN_POINT('Origin',(39.1545010521108,83.8,-82.5543760294777));
#64905=CARTESIAN_POINT('Origin',(14.1600345378716,83.8,-91.0136139864502));
#64906=CARTESIAN_POINT('',(14.1600345378716,83.8,-91.0136139864502));
#64907=CARTESIAN_POINT('',(14.5931693402804,83.8,-93.8676860907033));
#64908=CARTESIAN_POINT('Origin',(11.4717681901516,83.8,-89.9616836764728));
#64909=CARTESIAN_POINT('',(11.4717681901516,83.8,-89.9616836764728));
#64910=CARTESIAN_POINT('Origin',(9.21663664484028,83.8,-91.7638254707484));
#64911=CARTESIAN_POINT('',(9.21663664484028,83.8,-91.7638254707484));
#64912=CARTESIAN_POINT('Origin',(9.64977144724901,83.8,-94.6178975750015));
#64913=CARTESIAN_POINT('',(9.64977144724901,83.8,-94.6178975750015));
#64914=CARTESIAN_POINT('Origin',(12.338037794969,83.8,-95.6698278849789));
#64915=CARTESIAN_POINT('',(12.338037794969,83.8,-95.6698278849789));
#64916=CARTESIAN_POINT('Origin',(14.5931693402804,83.8,-93.8676860907033));
#64917=CARTESIAN_POINT('Origin',(21.1443553856648,83.8,-93.7466091008041));
#64918=CARTESIAN_POINT('',(21.1443553856648,83.8,-93.7466091008041));
#64919=CARTESIAN_POINT('',(21.5774901880735,83.8,-96.6006812050572));
#64920=CARTESIAN_POINT('Origin',(18.4560890379448,83.8,-92.6946787908267));
#64921=CARTESIAN_POINT('',(18.4560890379448,83.8,-92.6946787908267));
#64922=CARTESIAN_POINT('Origin',(16.2009574926334,83.8,-94.4968205851023));
#64923=CARTESIAN_POINT('',(16.2009574926334,83.8,-94.4968205851023));
#64924=CARTESIAN_POINT('Origin',(16.6340922950421,83.8,-97.3508926893554));
#64925=CARTESIAN_POINT('',(16.6340922950421,83.8,-97.3508926893554));
#64926=CARTESIAN_POINT('Origin',(19.3223586427622,83.8,-98.4028229993328));
#64927=CARTESIAN_POINT('',(19.3223586427622,83.8,-98.4028229993328));
#64928=CARTESIAN_POINT('Origin',(21.5774901880735,83.8,-96.6006812050572));
#64929=CARTESIAN_POINT('Origin',(28.1286762334579,83.8,-96.479604215158));
#64930=CARTESIAN_POINT('',(28.1286762334579,83.8,-96.479604215158));
#64931=CARTESIAN_POINT('',(28.5618110358666,83.8,-99.3336763194111));
#64932=CARTESIAN_POINT('Origin',(25.4404098857379,83.8,-95.4276739051805));
#64933=CARTESIAN_POINT('',(25.4404098857379,83.8,-95.4276739051805));
#64934=CARTESIAN_POINT('Origin',(23.1852783404265,83.8,-97.2298156994562));
#64935=CARTESIAN_POINT('',(23.1852783404265,83.8,-97.2298156994562));
#64936=CARTESIAN_POINT('Origin',(23.6184131428353,83.8,-100.083887803709));
#64937=CARTESIAN_POINT('',(23.6184131428353,83.8,-100.083887803709));
#64938=CARTESIAN_POINT('Origin',(26.3066794905553,83.8,-101.135818113687));
#64939=CARTESIAN_POINT('',(26.3066794905553,83.8,-101.135818113687));
#64940=CARTESIAN_POINT('Origin',(28.5618110358666,83.8,-99.3336763194111));
#64941=CARTESIAN_POINT('Origin',(35.112997081251,83.8,-99.2125993295118));
#64942=CARTESIAN_POINT('',(35.112997081251,83.8,-99.2125993295118));
#64943=CARTESIAN_POINT('',(35.5461318836598,83.8,-102.066671433765));
#64944=CARTESIAN_POINT('Origin',(32.424730733531,83.8,-98.1606690195344));
#64945=CARTESIAN_POINT('',(32.424730733531,83.8,-98.1606690195344));
#64946=CARTESIAN_POINT('Origin',(30.1695991882197,83.8,-99.9628108138101));
#64947=CARTESIAN_POINT('',(30.1695991882197,83.8,-99.9628108138101));
#64948=CARTESIAN_POINT('Origin',(30.6027339906284,83.8,-102.816882918063));
#64949=CARTESIAN_POINT('',(30.6027339906284,83.8,-102.816882918063));
#64950=CARTESIAN_POINT('Origin',(33.2910003383484,83.8,-103.868813228041));
#64951=CARTESIAN_POINT('',(33.2910003383484,83.8,-103.868813228041));
#64952=CARTESIAN_POINT('Origin',(35.5461318836598,83.8,-102.066671433765));
#64953=CARTESIAN_POINT('Origin',(-28.8712077753345,83.8,-67.2005464607798));
#64954=CARTESIAN_POINT('',(-28.8712077753345,83.8,-67.2005464607798));
#64955=CARTESIAN_POINT('',(-28.4380729729258,83.8,-70.0546185650329));
#64956=CARTESIAN_POINT('Origin',(-31.5594741230545,83.8,-66.1486161508024));
#64957=CARTESIAN_POINT('',(-31.5594741230545,83.8,-66.1486161508024));
#64958=CARTESIAN_POINT('Origin',(-33.8146056683659,83.8,-67.9507579450781));
#64959=CARTESIAN_POINT('',(-33.8146056683659,83.8,-67.9507579450781));
#64960=CARTESIAN_POINT('Origin',(-33.3814708659571,83.8,-70.8048300493311));
#64961=CARTESIAN_POINT('',(-33.3814708659571,83.8,-70.8048300493311));
#64962=CARTESIAN_POINT('Origin',(-30.6932045182371,83.8,-71.8567603593086));
#64963=CARTESIAN_POINT('',(-30.6932045182371,83.8,-71.8567603593086));
#64964=CARTESIAN_POINT('Origin',(-28.4380729729258,83.8,-70.0546185650329));
#64965=CARTESIAN_POINT('Origin',(-35.8555286231276,83.8,-64.4675513464259));
#64966=CARTESIAN_POINT('',(-35.8555286231276,83.8,-64.4675513464259));
#64967=CARTESIAN_POINT('',(-35.4223938207189,83.8,-67.321623450679));
#64968=CARTESIAN_POINT('Origin',(-38.5437949708476,83.8,-63.4156210364485));
#64969=CARTESIAN_POINT('',(-38.5437949708476,83.8,-63.4156210364485));
#64970=CARTESIAN_POINT('Origin',(-40.798926516159,83.8,-65.2177628307242));
#64971=CARTESIAN_POINT('',(-40.798926516159,83.8,-65.2177628307242));
#64972=CARTESIAN_POINT('Origin',(-40.3657917137503,83.8,-68.0718349349772));
#64973=CARTESIAN_POINT('',(-40.3657917137503,83.8,-68.0718349349772));
#64974=CARTESIAN_POINT('Origin',(-37.6775253660303,83.8,-69.1237652449547));
#64975=CARTESIAN_POINT('',(-37.6775253660303,83.8,-69.1237652449547));
#64976=CARTESIAN_POINT('Origin',(-35.4223938207189,83.8,-67.321623450679));
#64977=CARTESIAN_POINT('Origin',(-42.8398494709208,83.8,-61.734556232072));
#64978=CARTESIAN_POINT('',(-42.8398494709208,83.8,-61.734556232072));
#64979=CARTESIAN_POINT('',(-42.4067146685121,83.8,-64.5886283363251));
#64980=CARTESIAN_POINT('Origin',(-45.5281158186408,83.8,-60.6826259220946));
#64981=CARTESIAN_POINT('',(-45.5281158186408,83.8,-60.6826259220946));
#64982=CARTESIAN_POINT('Origin',(-47.7832473639521,83.8,-62.4847677163703));
#64983=CARTESIAN_POINT('',(-47.7832473639521,83.8,-62.4847677163703));
#64984=CARTESIAN_POINT('Origin',(-47.3501125615434,83.8,-65.3388398206233));
#64985=CARTESIAN_POINT('',(-47.3501125615434,83.8,-65.3388398206233));
#64986=CARTESIAN_POINT('Origin',(-44.6618462138234,83.8,-66.3907701306008));
#64987=CARTESIAN_POINT('',(-44.6618462138234,83.8,-66.3907701306008));
#64988=CARTESIAN_POINT('Origin',(-42.4067146685121,83.8,-64.5886283363251));
#64989=CARTESIAN_POINT('Origin',(42.0973179290442,83.8,-101.945594443866));
#64990=CARTESIAN_POINT('',(42.0973179290442,83.8,-101.945594443866));
#64991=CARTESIAN_POINT('',(42.5304527314529,83.8,-104.799666548119));
#64992=CARTESIAN_POINT('Origin',(39.4090515813242,83.8,-100.893664133888));
#64993=CARTESIAN_POINT('',(39.4090515813242,83.8,-100.893664133888));
#64994=CARTESIAN_POINT('Origin',(37.1539200360128,83.8,-102.695805928164));
#64995=CARTESIAN_POINT('',(37.1539200360128,83.8,-102.695805928164));
#64996=CARTESIAN_POINT('Origin',(37.5870548384215,83.8,-105.549878032417));
#64997=CARTESIAN_POINT('',(37.5870548384215,83.8,-105.549878032417));
#64998=CARTESIAN_POINT('Origin',(40.2753211861416,83.8,-106.601808342394));
#64999=CARTESIAN_POINT('',(40.2753211861416,83.8,-106.601808342394));
#65000=CARTESIAN_POINT('Origin',(42.5304527314529,83.8,-104.799666548119));
#65001=CARTESIAN_POINT('Origin',(7.17571369007852,83.8,-88.2806188720963));
#65002=CARTESIAN_POINT('',(7.17571369007852,83.8,-88.2806188720963));
#65003=CARTESIAN_POINT('',(7.60884849248723,83.8,-91.1346909763494));
#65004=CARTESIAN_POINT('Origin',(4.4874473423585,83.8,-87.2286885621189));
#65005=CARTESIAN_POINT('',(4.4874473423585,83.8,-87.2286885621189));
#65006=CARTESIAN_POINT('Origin',(2.23231579704715,83.8,-89.0308303563946));
#65007=CARTESIAN_POINT('',(2.23231579704715,83.8,-89.0308303563946));
#65008=CARTESIAN_POINT('Origin',(2.66545059945588,83.8,-91.8849024606476));
#65009=CARTESIAN_POINT('',(2.66545059945588,83.8,-91.8849024606476));
#65010=CARTESIAN_POINT('Origin',(5.35371694717591,83.8,-92.936832770625));
#65011=CARTESIAN_POINT('',(5.35371694717591,83.8,-92.936832770625));
#65012=CARTESIAN_POINT('Origin',(7.60884849248723,83.8,-91.1346909763494));
#65013=CARTESIAN_POINT('Origin',(0.191392842285382,83.8,-85.5476237577424));
#65014=CARTESIAN_POINT('',(0.191392842285382,83.8,-85.5476237577424));
#65015=CARTESIAN_POINT('',(0.6245276446941,83.8,-88.4016958619955));
#65016=CARTESIAN_POINT('Origin',(-2.49687350543463,83.8,-84.495693447765));
#65017=CARTESIAN_POINT('',(-2.49687350543463,83.8,-84.495693447765));
#65018=CARTESIAN_POINT('Origin',(-4.75200505074598,83.8,-86.2978352420407));
#65019=CARTESIAN_POINT('',(-4.75200505074598,83.8,-86.2978352420407));
#65020=CARTESIAN_POINT('Origin',(-4.31887024833725,83.8,-89.1519073462937));
#65021=CARTESIAN_POINT('',(-4.31887024833725,83.8,-89.1519073462937));
#65022=CARTESIAN_POINT('Origin',(-1.63060390061722,83.8,-90.2038376562712));
#65023=CARTESIAN_POINT('',(-1.63060390061722,83.8,-90.2038376562712));
#65024=CARTESIAN_POINT('Origin',(0.6245276446941,83.8,-88.4016958619955));
#65025=CARTESIAN_POINT('Origin',(-6.79292800550775,83.8,-82.8146286433885));
#65026=CARTESIAN_POINT('',(-6.79292800550775,83.8,-82.8146286433885));
#65027=CARTESIAN_POINT('',(-6.35979320309903,83.8,-85.6687007476416));
#65028=CARTESIAN_POINT('Origin',(-9.48119435322776,83.8,-81.7626983334111));
#65029=CARTESIAN_POINT('',(-9.48119435322776,83.8,-81.7626983334111));
#65030=CARTESIAN_POINT('Origin',(-11.7363258985391,83.8,-83.5648401276868));
#65031=CARTESIAN_POINT('',(-11.7363258985391,83.8,-83.5648401276868));
#65032=CARTESIAN_POINT('Origin',(-11.3031910961304,83.8,-86.4189122319399));
#65033=CARTESIAN_POINT('',(-11.3031910961304,83.8,-86.4189122319399));
#65034=CARTESIAN_POINT('Origin',(-8.61492474841036,83.8,-87.4708425419173));
#65035=CARTESIAN_POINT('',(-8.61492474841036,83.8,-87.4708425419173));
#65036=CARTESIAN_POINT('Origin',(-6.35979320309903,83.8,-85.6687007476416));
#65037=CARTESIAN_POINT('Origin',(-13.7772488533009,83.8,-80.0816335290346));
#65038=CARTESIAN_POINT('',(-13.7772488533009,83.8,-80.0816335290346));
#65039=CARTESIAN_POINT('',(-13.3441140508922,83.8,-82.9357056332877));
#65040=CARTESIAN_POINT('Origin',(-16.4655152010209,83.8,-79.0297032190572));
#65041=CARTESIAN_POINT('',(-16.4655152010209,83.8,-79.0297032190572));
#65042=CARTESIAN_POINT('Origin',(-18.7206467463322,83.8,-80.8318450133329));
#65043=CARTESIAN_POINT('',(-18.7206467463322,83.8,-80.8318450133329));
#65044=CARTESIAN_POINT('Origin',(-18.2875119439235,83.8,-83.685917117586));
#65045=CARTESIAN_POINT('',(-18.2875119439235,83.8,-83.685917117586));
#65046=CARTESIAN_POINT('Origin',(-15.5992455962035,83.8,-84.7378474275634));
#65047=CARTESIAN_POINT('',(-15.5992455962035,83.8,-84.7378474275634));
#65048=CARTESIAN_POINT('Origin',(-13.3441140508922,83.8,-82.9357056332877));
#65049=CARTESIAN_POINT('Origin',(-20.761569701094,83.8,-77.3486384146807));
#65050=CARTESIAN_POINT('',(-20.761569701094,83.8,-77.3486384146807));
#65051=CARTESIAN_POINT('',(-20.3284348986853,83.8,-80.2027105189338));
#65052=CARTESIAN_POINT('Origin',(-23.449836048814,83.8,-76.2967081047033));
#65053=CARTESIAN_POINT('',(-23.449836048814,83.8,-76.2967081047033));
#65054=CARTESIAN_POINT('Origin',(-25.7049675941254,83.8,-78.098849898979));
#65055=CARTESIAN_POINT('',(-25.7049675941254,83.8,-78.098849898979));
#65056=CARTESIAN_POINT('Origin',(-25.2718327917166,83.8,-80.9529220032321));
#65057=CARTESIAN_POINT('',(-25.2718327917166,83.8,-80.9529220032321));
#65058=CARTESIAN_POINT('Origin',(-22.5835664439966,83.8,-82.0048523132095));
#65059=CARTESIAN_POINT('',(-22.5835664439966,83.8,-82.0048523132095));
#65060=CARTESIAN_POINT('Origin',(-20.3284348986853,83.8,-80.2027105189338));
#65061=CARTESIAN_POINT('Origin',(-27.7458905488871,83.8,-74.6156433003268));
#65062=CARTESIAN_POINT('',(-27.7458905488871,83.8,-74.6156433003268));
#65063=CARTESIAN_POINT('',(-27.3127557464784,83.8,-77.4697154045799));
#65064=CARTESIAN_POINT('Origin',(-30.4341568966072,83.8,-73.5637129903494));
#65065=CARTESIAN_POINT('',(-30.4341568966072,83.8,-73.5637129903494));
#65066=CARTESIAN_POINT('Origin',(-32.6892884419185,83.8,-75.3658547846251));
#65067=CARTESIAN_POINT('',(-32.6892884419185,83.8,-75.3658547846251));
#65068=CARTESIAN_POINT('Origin',(-32.2561536395098,83.8,-78.2199268888782));
#65069=CARTESIAN_POINT('',(-32.2561536395098,83.8,-78.2199268888782));
#65070=CARTESIAN_POINT('Origin',(-29.5678872917897,83.8,-79.2718571988556));
#65071=CARTESIAN_POINT('',(-29.5678872917897,83.8,-79.2718571988556));
#65072=CARTESIAN_POINT('Origin',(-27.3127557464784,83.8,-77.4697154045799));
#65073=CARTESIAN_POINT('Origin',(-34.7302113966803,83.8,-71.8826481859729));
#65074=CARTESIAN_POINT('',(-34.7302113966803,83.8,-71.8826481859729));
#65075=CARTESIAN_POINT('',(-34.2970765942716,83.8,-74.7367202902261));
#65076=CARTESIAN_POINT('Origin',(-37.4184777444003,83.8,-70.8307178759955));
#65077=CARTESIAN_POINT('',(-37.4184777444003,83.8,-70.8307178759955));
#65078=CARTESIAN_POINT('Origin',(-39.6736092897116,83.8,-72.6328596702712));
#65079=CARTESIAN_POINT('',(-39.6736092897116,83.8,-72.6328596702712));
#65080=CARTESIAN_POINT('Origin',(-39.2404744873029,83.8,-75.4869317745243));
#65081=CARTESIAN_POINT('',(-39.2404744873029,83.8,-75.4869317745243));
#65082=CARTESIAN_POINT('Origin',(-36.5522081395829,83.8,-76.5388620845017));
#65083=CARTESIAN_POINT('',(-36.5522081395829,83.8,-76.5388620845017));
#65084=CARTESIAN_POINT('Origin',(-34.2970765942716,83.8,-74.7367202902261));
#65085=CARTESIAN_POINT('Origin',(-41.7145322444734,83.8,-69.1496530716191));
#65086=CARTESIAN_POINT('',(-41.7145322444734,83.8,-69.1496530716191));
#65087=CARTESIAN_POINT('',(-41.2813974420647,83.8,-72.0037251758721));
#65088=CARTESIAN_POINT('Origin',(-44.4027985921934,83.8,-68.0977227616416));
#65089=CARTESIAN_POINT('',(-44.4027985921934,83.8,-68.0977227616416));
#65090=CARTESIAN_POINT('Origin',(-46.6579301375048,83.8,-69.8998645559173));
#65091=CARTESIAN_POINT('',(-46.6579301375048,83.8,-69.8998645559173));
#65092=CARTESIAN_POINT('Origin',(-46.224795335096,83.8,-72.7539366601704));
#65093=CARTESIAN_POINT('',(-46.224795335096,83.8,-72.7539366601704));
#65094=CARTESIAN_POINT('Origin',(-43.536528987376,83.8,-73.8058669701478));
#65095=CARTESIAN_POINT('',(-43.536528987376,83.8,-73.8058669701478));
#65096=CARTESIAN_POINT('Origin',(-41.2813974420647,83.8,-72.0037251758721));
#65097=CARTESIAN_POINT('Origin',(-43.9651666973681,83.8,-54.3194593925249));
#65098=CARTESIAN_POINT('',(-43.9651666973681,83.8,-54.3194593925249));
#65099=CARTESIAN_POINT('',(-43.5320318949594,83.8,-57.1735314967781));
#65100=CARTESIAN_POINT('Origin',(-46.6534330450882,83.8,-53.2675290825475));
#65101=CARTESIAN_POINT('',(-46.6534330450882,83.8,-53.2675290825475));
#65102=CARTESIAN_POINT('Origin',(-48.9085645903995,83.8,-55.0696708768232));
#65103=CARTESIAN_POINT('',(-48.9085645903995,83.8,-55.0696708768232));
#65104=CARTESIAN_POINT('Origin',(-48.4754297879908,83.8,-57.9237429810763));
#65105=CARTESIAN_POINT('',(-48.4754297879908,83.8,-57.9237429810763));
#65106=CARTESIAN_POINT('Origin',(-45.7871634402707,83.8,-58.9756732910537));
#65107=CARTESIAN_POINT('',(-45.7871634402707,83.8,-58.9756732910537));
#65108=CARTESIAN_POINT('Origin',(-43.5320318949594,83.8,-57.1735314967781));
#65109=CARTESIAN_POINT('Origin',(47.9563215503899,83.8,-97.2634927186726));
#65110=CARTESIAN_POINT('',(47.9563215503899,83.8,-97.2634927186726));
#65111=CARTESIAN_POINT('',(48.3894563527986,83.8,-100.117564822926));
#65112=CARTESIAN_POINT('Origin',(45.2680552026699,83.8,-96.2115624086952));
#65113=CARTESIAN_POINT('',(45.2680552026699,83.8,-96.2115624086952));
#65114=CARTESIAN_POINT('Origin',(43.0129236573585,83.8,-98.0137042029708));
#65115=CARTESIAN_POINT('',(43.0129236573585,83.8,-98.0137042029708));
#65116=CARTESIAN_POINT('Origin',(43.4460584597673,83.8,-100.867776307224));
#65117=CARTESIAN_POINT('',(43.4460584597673,83.8,-100.867776307224));
#65118=CARTESIAN_POINT('Origin',(46.1343248074873,83.8,-101.919706617201));
#65119=CARTESIAN_POINT('',(46.1343248074873,83.8,-101.919706617201));
#65120=CARTESIAN_POINT('Origin',(48.3894563527986,83.8,-100.117564822926));
#65121=CARTESIAN_POINT('Origin',(40.9720007025968,83.8,-94.5304976043187));
#65122=CARTESIAN_POINT('',(40.9720007025968,83.8,-94.5304976043187));
#65123=CARTESIAN_POINT('',(41.4051355050055,83.8,-97.3845697085718));
#65124=CARTESIAN_POINT('Origin',(38.2837343548768,83.8,-93.4785672943413));
#65125=CARTESIAN_POINT('',(38.2837343548768,83.8,-93.4785672943413));
#65126=CARTESIAN_POINT('Origin',(36.0286028095654,83.8,-95.280709088617));
#65127=CARTESIAN_POINT('',(36.0286028095654,83.8,-95.280709088617));
#65128=CARTESIAN_POINT('Origin',(36.4617376119742,83.8,-98.13478119287));
#65129=CARTESIAN_POINT('',(36.4617376119742,83.8,-98.13478119287));
#65130=CARTESIAN_POINT('Origin',(39.1500039596942,83.8,-99.1867115028474));
#65131=CARTESIAN_POINT('',(39.1500039596942,83.8,-99.1867115028474));
#65132=CARTESIAN_POINT('Origin',(41.4051355050055,83.8,-97.3845697085718));
#65133=CARTESIAN_POINT('Origin',(33.9876798548037,83.8,-91.7975024899648));
#65134=CARTESIAN_POINT('',(33.9876798548037,83.8,-91.7975024899648));
#65135=CARTESIAN_POINT('',(34.4208146572124,83.8,-94.6515745942179));
#65136=CARTESIAN_POINT('Origin',(31.2994135070836,83.8,-90.7455721799874));
#65137=CARTESIAN_POINT('',(31.2994135070836,83.8,-90.7455721799874));
#65138=CARTESIAN_POINT('Origin',(29.0442819617723,83.8,-92.5477139742631));
#65139=CARTESIAN_POINT('',(29.0442819617723,83.8,-92.5477139742631));
#65140=CARTESIAN_POINT('Origin',(29.477416764181,83.8,-95.4017860785161));
#65141=CARTESIAN_POINT('',(29.477416764181,83.8,-95.4017860785161));
#65142=CARTESIAN_POINT('Origin',(32.1656831119011,83.8,-96.4537163884935));
#65143=CARTESIAN_POINT('',(32.1656831119011,83.8,-96.4537163884935));
#65144=CARTESIAN_POINT('Origin',(34.4208146572124,83.8,-94.6515745942179));
#65145=CARTESIAN_POINT('Origin',(-36.980845849575,83.8,-57.0524545068788));
#65146=CARTESIAN_POINT('',(-36.980845849575,83.8,-57.0524545068788));
#65147=CARTESIAN_POINT('',(-36.5477110471663,83.8,-59.9065266111319));
#65148=CARTESIAN_POINT('Origin',(-39.669112197295,83.8,-56.0005241969014));
#65149=CARTESIAN_POINT('',(-39.669112197295,83.8,-56.0005241969014));
#65150=CARTESIAN_POINT('Origin',(-41.9242437426064,83.8,-57.8026659911771));
#65151=CARTESIAN_POINT('',(-41.9242437426064,83.8,-57.8026659911771));
#65152=CARTESIAN_POINT('Origin',(-41.4911089401976,83.8,-60.6567380954302));
#65153=CARTESIAN_POINT('',(-41.4911089401976,83.8,-60.6567380954302));
#65154=CARTESIAN_POINT('Origin',(-38.8028425924776,83.8,-61.7086684054076));
#65155=CARTESIAN_POINT('',(-38.8028425924776,83.8,-61.7086684054076));
#65156=CARTESIAN_POINT('Origin',(-36.5477110471663,83.8,-59.9065266111319));
#65157=CARTESIAN_POINT('Origin',(-29.9965250017819,83.8,-59.7854496212327));
#65158=CARTESIAN_POINT('',(-29.9965250017819,83.8,-59.7854496212327));
#65159=CARTESIAN_POINT('',(-29.5633901993732,83.8,-62.6395217254858));
#65160=CARTESIAN_POINT('Origin',(-32.6847913495019,83.8,-58.7335193112553));
#65161=CARTESIAN_POINT('',(-32.6847913495019,83.8,-58.7335193112553));
#65162=CARTESIAN_POINT('Origin',(-34.9399228948133,83.8,-60.535661105531));
#65163=CARTESIAN_POINT('',(-34.9399228948133,83.8,-60.535661105531));
#65164=CARTESIAN_POINT('Origin',(-34.5067880924045,83.8,-63.3897332097841));
#65165=CARTESIAN_POINT('',(-34.5067880924045,83.8,-63.3897332097841));
#65166=CARTESIAN_POINT('Origin',(-31.8185217446845,83.8,-64.4416635197615));
#65167=CARTESIAN_POINT('',(-31.8185217446845,83.8,-64.4416635197615));
#65168=CARTESIAN_POINT('Origin',(-29.5633901993732,83.8,-62.6395217254858));
#65169=CARTESIAN_POINT('Origin',(-23.0122041539888,83.8,-62.5184447355866));
#65170=CARTESIAN_POINT('',(-23.0122041539888,83.8,-62.5184447355866));
#65171=CARTESIAN_POINT('',(-22.57906935158,83.8,-65.3725168398397));
#65172=CARTESIAN_POINT('Origin',(-25.7004705017088,83.8,-61.4665144256092));
#65173=CARTESIAN_POINT('',(-25.7004705017088,83.8,-61.4665144256092));
#65174=CARTESIAN_POINT('Origin',(-27.9556020470201,83.8,-63.2686562198849));
#65175=CARTESIAN_POINT('',(-27.9556020470201,83.8,-63.2686562198849));
#65176=CARTESIAN_POINT('Origin',(-27.5224672446114,83.8,-66.122728324138));
#65177=CARTESIAN_POINT('',(-27.5224672446114,83.8,-66.122728324138));
#65178=CARTESIAN_POINT('Origin',(-24.8342008968914,83.8,-67.1746586341154));
#65179=CARTESIAN_POINT('',(-24.8342008968914,83.8,-67.1746586341154));
#65180=CARTESIAN_POINT('Origin',(-22.57906935158,83.8,-65.3725168398397));
#65181=CARTESIAN_POINT('Origin',(-16.0278833061956,83.8,-65.2514398499405));
#65182=CARTESIAN_POINT('',(-16.0278833061956,83.8,-65.2514398499405));
#65183=CARTESIAN_POINT('',(-15.5947485037869,83.8,-68.1055119541936));
#65184=CARTESIAN_POINT('Origin',(-18.7161496539156,83.8,-64.1995095399631));
#65185=CARTESIAN_POINT('',(-18.7161496539156,83.8,-64.1995095399631));
#65186=CARTESIAN_POINT('Origin',(-20.971281199227,83.8,-66.0016513342388));
#65187=CARTESIAN_POINT('',(-20.971281199227,83.8,-66.0016513342388));
#65188=CARTESIAN_POINT('Origin',(-20.5381463968183,83.8,-68.8557234384919));
#65189=CARTESIAN_POINT('',(-20.5381463968183,83.8,-68.8557234384919));
#65190=CARTESIAN_POINT('Origin',(-17.8498800490982,83.8,-69.9076537484693));
#65191=CARTESIAN_POINT('',(-17.8498800490982,83.8,-69.9076537484693));
#65192=CARTESIAN_POINT('Origin',(-15.5947485037869,83.8,-68.1055119541936));
#65193=CARTESIAN_POINT('Origin',(27.0033590070105,83.8,-89.0645073756109));
#65194=CARTESIAN_POINT('',(27.0033590070105,83.8,-89.0645073756109));
#65195=CARTESIAN_POINT('',(27.4364938094193,83.8,-91.918579479864));
#65196=CARTESIAN_POINT('Origin',(24.3150926592905,83.8,-88.0125770656335));
#65197=CARTESIAN_POINT('',(24.3150926592905,83.8,-88.0125770656335));
#65198=CARTESIAN_POINT('Origin',(22.0599611139792,83.8,-89.8147188599092));
#65199=CARTESIAN_POINT('',(22.0599611139792,83.8,-89.8147188599092));
#65200=CARTESIAN_POINT('Origin',(22.4930959163879,83.8,-92.6687909641622));
#65201=CARTESIAN_POINT('',(22.4930959163879,83.8,-92.6687909641622));
#65202=CARTESIAN_POINT('Origin',(25.1813622641079,83.8,-93.7207212741397));
#65203=CARTESIAN_POINT('',(25.1813622641079,83.8,-93.7207212741397));
#65204=CARTESIAN_POINT('Origin',(27.4364938094193,83.8,-91.918579479864));
#65205=CARTESIAN_POINT('Origin',(20.0190381592174,83.8,-86.331512261257));
#65206=CARTESIAN_POINT('',(20.0190381592174,83.8,-86.331512261257));
#65207=CARTESIAN_POINT('',(20.4521729616261,83.8,-89.1855843655101));
#65208=CARTESIAN_POINT('Origin',(17.3307718114974,83.8,-85.2795819512796));
#65209=CARTESIAN_POINT('',(17.3307718114974,83.8,-85.2795819512796));
#65210=CARTESIAN_POINT('Origin',(15.075640266186,83.8,-87.0817237455553));
#65211=CARTESIAN_POINT('',(15.075640266186,83.8,-87.0817237455553));
#65212=CARTESIAN_POINT('Origin',(15.5087750685948,83.8,-89.9357958498083));
#65213=CARTESIAN_POINT('',(15.5087750685948,83.8,-89.9357958498083));
#65214=CARTESIAN_POINT('Origin',(18.1970414163148,83.8,-90.9877261597858));
#65215=CARTESIAN_POINT('',(18.1970414163148,83.8,-90.9877261597858));
#65216=CARTESIAN_POINT('Origin',(20.4521729616261,83.8,-89.1855843655101));
#65217=CARTESIAN_POINT('Origin',(13.0347173114243,83.8,-83.5985171469031));
#65218=CARTESIAN_POINT('',(13.0347173114243,83.8,-83.5985171469031));
#65219=CARTESIAN_POINT('',(13.467852113833,83.8,-86.4525892511562));
#65220=CARTESIAN_POINT('Origin',(10.3464509637043,83.8,-82.5465868369257));
#65221=CARTESIAN_POINT('',(10.3464509637043,83.8,-82.5465868369257));
#65222=CARTESIAN_POINT('Origin',(8.09131941839291,83.8,-84.3487286312014));
#65223=CARTESIAN_POINT('',(8.09131941839291,83.8,-84.3487286312014));
#65224=CARTESIAN_POINT('Origin',(8.52445422080164,83.8,-87.2028007354545));
#65225=CARTESIAN_POINT('',(8.52445422080164,83.8,-87.2028007354545));
#65226=CARTESIAN_POINT('Origin',(11.2127205685217,83.8,-88.2547310454319));
#65227=CARTESIAN_POINT('',(11.2127205685217,83.8,-88.2547310454319));
#65228=CARTESIAN_POINT('Origin',(13.467852113833,83.8,-86.4525892511562));
#65229=CARTESIAN_POINT('Origin',(6.05039646363115,83.8,-80.8655220325492));
#65230=CARTESIAN_POINT('',(6.05039646363115,83.8,-80.8655220325492));
#65231=CARTESIAN_POINT('',(6.48353126603986,83.8,-83.7195941368023));
#65232=CARTESIAN_POINT('Origin',(3.36213011591114,83.8,-79.8135917225718));
#65233=CARTESIAN_POINT('',(3.36213011591114,83.8,-79.8135917225718));
#65234=CARTESIAN_POINT('Origin',(1.10699857059978,83.8,-81.6157335168475));
#65235=CARTESIAN_POINT('',(1.10699857059978,83.8,-81.6157335168475));
#65236=CARTESIAN_POINT('Origin',(1.54013337300851,83.8,-84.4698056211006));
#65237=CARTESIAN_POINT('',(1.54013337300851,83.8,-84.4698056211006));
#65238=CARTESIAN_POINT('Origin',(4.22839972072854,83.8,-85.521735931078));
#65239=CARTESIAN_POINT('',(4.22839972072854,83.8,-85.521735931078));
#65240=CARTESIAN_POINT('Origin',(6.48353126603986,83.8,-83.7195941368023));
#65241=CARTESIAN_POINT('Origin',(-0.933924384161986,83.8,-78.1325269181953));
#65242=CARTESIAN_POINT('',(-0.933924384161986,83.8,-78.1325269181953));
#65243=CARTESIAN_POINT('',(-0.500789581753269,83.8,-80.9865990224485));
#65244=CARTESIAN_POINT('Origin',(-3.622190731882,83.8,-77.0805966082179));
#65245=CARTESIAN_POINT('',(-3.622190731882,83.8,-77.0805966082179));
#65246=CARTESIAN_POINT('Origin',(-5.87732227719335,83.8,-78.8827384024936));
#65247=CARTESIAN_POINT('',(-5.87732227719335,83.8,-78.8827384024936));
#65248=CARTESIAN_POINT('Origin',(-5.44418747478462,83.8,-81.7368105067467));
#65249=CARTESIAN_POINT('',(-5.44418747478462,83.8,-81.7368105067467));
#65250=CARTESIAN_POINT('Origin',(-2.75592112706459,83.8,-82.7887408167241));
#65251=CARTESIAN_POINT('',(-2.75592112706459,83.8,-82.7887408167241));
#65252=CARTESIAN_POINT('Origin',(-0.500789581753269,83.8,-80.9865990224485));
#65253=CARTESIAN_POINT('Origin',(-7.91824523195512,83.8,-75.3995318038414));
#65254=CARTESIAN_POINT('',(-7.91824523195512,83.8,-75.3995318038414));
#65255=CARTESIAN_POINT('',(-7.4851104295464,83.8,-78.2536039080945));
#65256=CARTESIAN_POINT('Origin',(-10.6065115796751,83.8,-74.347601493864));
#65257=CARTESIAN_POINT('',(-10.6065115796751,83.8,-74.347601493864));
#65258=CARTESIAN_POINT('Origin',(-12.8616431249865,83.8,-76.1497432881397));
#65259=CARTESIAN_POINT('',(-12.8616431249865,83.8,-76.1497432881397));
#65260=CARTESIAN_POINT('Origin',(-12.4285083225778,83.8,-79.0038153923928));
#65261=CARTESIAN_POINT('',(-12.4285083225778,83.8,-79.0038153923928));
#65262=CARTESIAN_POINT('Origin',(-9.74024197485773,83.8,-80.0557457023702));
#65263=CARTESIAN_POINT('',(-9.74024197485773,83.8,-80.0557457023702));
#65264=CARTESIAN_POINT('Origin',(-7.4851104295464,83.8,-78.2536039080945));
#65265=CARTESIAN_POINT('Origin',(-14.9025660797482,83.8,-72.6665366894876));
#65266=CARTESIAN_POINT('',(-14.9025660797482,83.8,-72.6665366894876));
#65267=CARTESIAN_POINT('',(-14.4694312773395,83.8,-75.5206087937407));
#65268=CARTESIAN_POINT('Origin',(-17.5908324274683,83.8,-71.6146063795101));
#65269=CARTESIAN_POINT('',(-17.5908324274683,83.8,-71.6146063795101));
#65270=CARTESIAN_POINT('Origin',(-19.8459639727796,83.8,-73.4167481737858));
#65271=CARTESIAN_POINT('',(-19.8459639727796,83.8,-73.4167481737858));
#65272=CARTESIAN_POINT('Origin',(-19.4128291703709,83.8,-76.2708202780389));
#65273=CARTESIAN_POINT('',(-19.4128291703709,83.8,-76.2708202780389));
#65274=CARTESIAN_POINT('Origin',(-16.7245628226509,83.8,-77.3227505880163));
#65275=CARTESIAN_POINT('',(-16.7245628226509,83.8,-77.3227505880163));
#65276=CARTESIAN_POINT('Origin',(-14.4694312773395,83.8,-75.5206087937407));
#65277=CARTESIAN_POINT('Origin',(-21.8868869275414,83.8,-69.9335415751337));
#65278=CARTESIAN_POINT('',(-21.8868869275414,83.8,-69.9335415751337));
#65279=CARTESIAN_POINT('',(-21.4537521251327,83.8,-72.7876136793868));
#65280=CARTESIAN_POINT('Origin',(-24.5751532752614,83.8,-68.8816112651563));
#65281=CARTESIAN_POINT('',(-24.5751532752614,83.8,-68.8816112651563));
#65282=CARTESIAN_POINT('Origin',(-26.8302848205727,83.8,-70.683753059432));
#65283=CARTESIAN_POINT('',(-26.8302848205727,83.8,-70.683753059432));
#65284=CARTESIAN_POINT('Origin',(-26.397150018164,83.8,-73.537825163685));
#65285=CARTESIAN_POINT('',(-26.397150018164,83.8,-73.537825163685));
#65286=CARTESIAN_POINT('Origin',(-23.708883670444,83.8,-74.5897554736624));
#65287=CARTESIAN_POINT('',(-23.708883670444,83.8,-74.5897554736624));
#65288=CARTESIAN_POINT('Origin',(-21.4537521251327,83.8,-72.7876136793868));
#65297=UNCERTAINTY_MEASURE_WITH_UNIT(LENGTH_MEASURE(0.01),#65305,
'DISTANCE_ACCURACY_VALUE',
'Maximum model space distance between geometric entities at asserted c
onnectivities');
#65298=UNCERTAINTY_MEASURE_WITH_UNIT(LENGTH_MEASURE(0.01),#65305,
'DISTANCE_ACCURACY_VALUE',
'Maximum model space distance between geometric entities at asserted c
onnectivities');
#65303=(
GEOMETRIC_REPRESENTATION_CONTEXT(3)
GLOBAL_UNCERTAINTY_ASSIGNED_CONTEXT((#65297))
GLOBAL_UNIT_ASSIGNED_CONTEXT((#65305,#65307,#65308))
REPRESENTATION_CONTEXT('','3D')
);
#65304=(
GEOMETRIC_REPRESENTATION_CONTEXT(3)
GLOBAL_UNCERTAINTY_ASSIGNED_CONTEXT((#65298))
GLOBAL_UNIT_ASSIGNED_CONTEXT((#65305,#65307,#65308))
REPRESENTATION_CONTEXT('','3D')
);
#65305=(
LENGTH_UNIT()
NAMED_UNIT(*)
SI_UNIT(.MILLI.,.METRE.)
);
#65307=(
NAMED_UNIT(*)
PLANE_ANGLE_UNIT()
SI_UNIT($,.RADIAN.)
);
#65308=(
NAMED_UNIT(*)
SI_UNIT($,.STERADIAN.)
SOLID_ANGLE_UNIT()
);
#65313=SHAPE_DEFINITION_REPRESENTATION(#65318,#65327);
#65318=PRODUCT_DEFINITION_SHAPE('',$,#65333);
#65327=SHAPE_REPRESENTATION('',(#41307),#65303);
#65328=PRODUCT_DEFINITION_CONTEXT('part definition',#65345,'design');
#65333=PRODUCT_DEFINITION('Sheet Metal Up','Sheet Metal Up',#65338,#65328);
#65338=PRODUCT_DEFINITION_FORMATION('',$,#65351);
#65345=APPLICATION_CONTEXT(
'Core Data for Automotive Mechanical Design Process');
#65346=PRODUCT_CONTEXT('part definition',#65345,'mechanical');
#65351=PRODUCT('Sheet Metal Up','Sheet Metal Up',$,(#65346));
#65356=PRESENTATION_STYLE_ASSIGNMENT((#65361));
#65361=SURFACE_STYLE_USAGE(.BOTH.,#65366);
#65366=SURFACE_SIDE_STYLE('',(#65371));
#65371=SURFACE_STYLE_FILL_AREA(#65376);
#65376=FILL_AREA_STYLE('Opaque(169,212,242)',(#65381));
#65381=FILL_AREA_STYLE_COLOUR('Opaque(169,212,242)',#65386);
#65386=COLOUR_RGB('Opaque(169,212,242)',0.662745098039216,0.831372549019608,
0.949019607843137);
ENDSEC;
END-ISO-10303-21;
